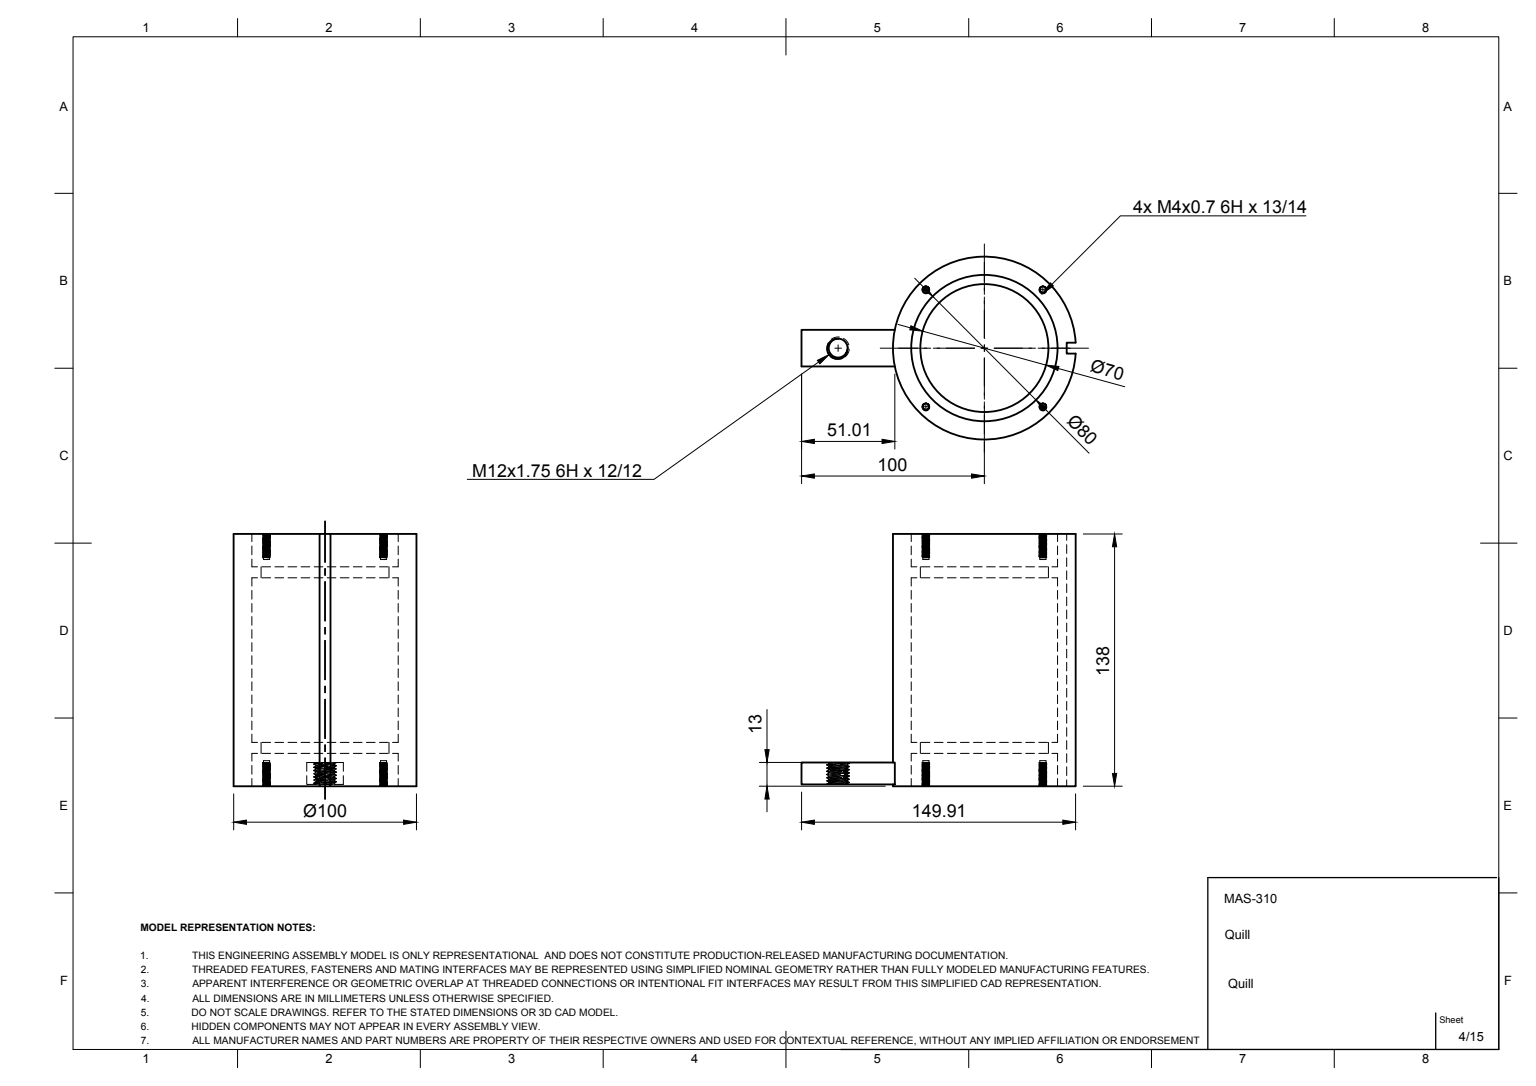
ISO-10303-21;
HEADER;
/* Generated by software containing ST-Developer
 * from STEP Tools, Inc. (www.steptools.com) 
 */

FILE_DESCRIPTION(
/* description */ ('Independent30mm screw-fed quill/spindle unit with16mm straight tool s
ocket, radial set screw, native reusable open ball bearings, retained 
inner/outer race stacks, keyed quill guide and M12x1.75 fine feed. Ext
ernal moving drive and tool not included. Ideal cage orbital links; in
dividual ball spin, force and preload not simulated. No drilling capac
ity, runout, speed, torque, load, life or machine safety rating.'),
/* implementation_level */ '2;1');

FILE_NAME(
/* name */ 'Quill.step',
/* time_stamp */ '2026-11-08T18:59:42-08:00',
/* author */ (''),
/* organization */ (''),
/* preprocessor_version */ 'ST-DEVELOPER v20.2',
/* originating_system */ 'Autodesk Translation Framework v15.17.0.0',
/* authorisation */ '');

FILE_SCHEMA (('AUTOMOTIVE_DESIGN { 1 0 10303 214 3 1 1 }'));
ENDSEC;

DATA;
#10=MECHANICAL_DESIGN_GEOMETRIC_PRESENTATION_REPRESENTATION('',(#1593),#63898);
#240=B_SPLINE_SURFACE_WITH_KNOTS('',3,3,((#31744,#31745,#31746,#31747,#31748,
#31749,#31750,#31751,#31752,#31753,#31754,#31755,#31756,#31757,#31758,#31759,
#31760,#31761,#31762,#31763,#31764,#31765,#31766,#31767,#31768,#31769,#31770,
#31771,#31772,#31773,#31774,#31775,#31776,#31777,#31778,#31779,#31780,#31781,
#31782,#31783,#31784,#31785,#31786,#31787,#31788,#31789,#31790,#31791,#31792,
#31793,#31794,#31795,#31796,#31797,#31798,#31799,#31800,#31801,#31802,#31803,
#31804,#31805,#31806,#31807,#31808,#31809,#31810,#31811,#31812,#31813,#31814,
#31815,#31816,#31817,#31818,#31819,#31820,#31821,#31822,#31823,#31824,#31825,
#31826,#31827,#31828,#31829,#31830,#31831,#31832,#31833,#31834,#31835,#31836,
#31837,#31838,#31839,#31840,#31841,#31842,#31843,#31844,#31845,#31846,#31847,
#31848,#31849,#31850,#31851,#31852,#31853,#31854,#31855,#31856,#31857,#31858,
#31859,#31860,#31861,#31862,#31863,#31864,#31865),(#31866,#31867,#31868,
#31869,#31870,#31871,#31872,#31873,#31874,#31875,#31876,#31877,#31878,#31879,
#31880,#31881,#31882,#31883,#31884,#31885,#31886,#31887,#31888,#31889,#31890,
#31891,#31892,#31893,#31894,#31895,#31896,#31897,#31898,#31899,#31900,#31901,
#31902,#31903,#31904,#31905,#31906,#31907,#31908,#31909,#31910,#31911,#31912,
#31913,#31914,#31915,#31916,#31917,#31918,#31919,#31920,#31921,#31922,#31923,
#31924,#31925,#31926,#31927,#31928,#31929,#31930,#31931,#31932,#31933,#31934,
#31935,#31936,#31937,#31938,#31939,#31940,#31941,#31942,#31943,#31944,#31945,
#31946,#31947,#31948,#31949,#31950,#31951,#31952,#31953,#31954,#31955,#31956,
#31957,#31958,#31959,#31960,#31961,#31962,#31963,#31964,#31965,#31966,#31967,
#31968,#31969,#31970,#31971,#31972,#31973,#31974,#31975,#31976,#31977,#31978,
#31979,#31980,#31981,#31982,#31983,#31984,#31985,#31986,#31987),(#31988,
#31989,#31990,#31991,#31992,#31993,#31994,#31995,#31996,#31997,#31998,#31999,
#32000,#32001,#32002,#32003,#32004,#32005,#32006,#32007,#32008,#32009,#32010,
#32011,#32012,#32013,#32014,#32015,#32016,#32017,#32018,#32019,#32020,#32021,
#32022,#32023,#32024,#32025,#32026,#32027,#32028,#32029,#32030,#32031,#32032,
#32033,#32034,#32035,#32036,#32037,#32038,#32039,#32040,#32041,#32042,#32043,
#32044,#32045,#32046,#32047,#32048,#32049,#32050,#32051,#32052,#32053,#32054,
#32055,#32056,#32057,#32058,#32059,#32060,#32061,#32062,#32063,#32064,#32065,
#32066,#32067,#32068,#32069,#32070,#32071,#32072,#32073,#32074,#32075,#32076,
#32077,#32078,#32079,#32080,#32081,#32082,#32083,#32084,#32085,#32086,#32087,
#32088,#32089,#32090,#32091,#32092,#32093,#32094,#32095,#32096,#32097,#32098,
#32099,#32100,#32101,#32102,#32103,#32104,#32105,#32106,#32107,#32108,#32109),
(#32110,#32111,#32112,#32113,#32114,#32115,#32116,#32117,#32118,#32119,
#32120,#32121,#32122,#32123,#32124,#32125,#32126,#32127,#32128,#32129,#32130,
#32131,#32132,#32133,#32134,#32135,#32136,#32137,#32138,#32139,#32140,#32141,
#32142,#32143,#32144,#32145,#32146,#32147,#32148,#32149,#32150,#32151,#32152,
#32153,#32154,#32155,#32156,#32157,#32158,#32159,#32160,#32161,#32162,#32163,
#32164,#32165,#32166,#32167,#32168,#32169,#32170,#32171,#32172,#32173,#32174,
#32175,#32176,#32177,#32178,#32179,#32180,#32181,#32182,#32183,#32184,#32185,
#32186,#32187,#32188,#32189,#32190,#32191,#32192,#32193,#32194,#32195,#32196,
#32197,#32198,#32199,#32200,#32201,#32202,#32203,#32204,#32205,#32206,#32207,
#32208,#32209,#32210,#32211,#32212,#32213,#32214,#32215,#32216,#32217,#32218,
#32219,#32220,#32221,#32222,#32223,#32224,#32225,#32226,#32227,#32228,#32229,
#32230,#32231)),.UNSPECIFIED.,.F.,.F.,.F.,(4,4),(4,1,1,1,1,1,1,1,1,1,1,
1,1,1,1,1,1,1,1,1,1,1,1,1,1,1,1,1,1,1,1,1,1,1,1,1,1,1,1,1,1,1,1,1,1,1,1,
1,1,1,1,1,1,1,1,1,1,1,1,1,1,1,1,1,1,1,1,1,1,1,1,1,1,1,1,1,1,1,1,1,1,1,1,
1,1,1,1,1,1,1,1,1,1,1,1,1,1,1,1,1,1,1,1,1,1,1,1,1,1,1,1,1,1,1,1,1,1,1,1,
4),(0.,0.0448889834294937),(11.8615800042573,12.8590786597078,13.8565773151583,
14.8540759706088,15.8515746260593,16.8490732815098,17.8465719369603,18.8440705924108,
19.8415692478613,20.8390679033118,21.8365665587623,22.8340652142128,23.8315638696633,
24.8290625251138,25.8265611805643,26.8240598360148,27.8215584914653,28.8190571469158,
29.8165558023663,30.8140544578168,31.8115531132673,32.8090517687178,33.8065504241683,
34.8040490796188,35.8015477350693,36.7990463905198,37.7965450459703,38.7940437014208,
39.7915423568713,40.7890410123218,41.7865396677723,42.7840383232228,43.7815369786733,
44.7790356341238,45.7765342895743,46.7740329450248,47.7715316004753,48.7690302559258,
49.7665289113763,50.7640275668268,51.7615262222773,52.7590248777278,53.7565235331783,
54.7540221886288,55.7515208440793,56.7490194995298,57.7465181549803,58.7440168104308,
59.7415154658813,60.7390141213318,61.7365127767823,62.7340114322328,63.7315100876833,
64.7290087431338,65.7265073985843,66.7240060540348,67.7215047094853,68.7190033649358,
69.7165020203863,70.7140006758368,71.7114993312873,72.7089979867378,73.7064966421883,
74.7039952976388,75.7014939530893,76.6989926085398,77.6964912639903,78.6939899194408,
79.6914885748913,80.6889872303418,81.6864858857923,82.6839845412428,83.6814831966933,
84.6789818521438,85.6764805075943,86.6739791630448,87.6714778184953,88.6689764739458,
89.6664751293963,90.6639737848468,91.6614724402973,92.6589710957478,93.6564697511983,
94.6539684066488,95.6514670620993,96.6489657175498,97.6464643730003,98.6439630284508,
99.6414616839013,100.638960339352,101.636458994802,102.633957650253,103.631456305703,
104.628954961154,105.626453616604,106.623952272055,107.621450927505,108.618949582956,
109.616448238406,110.613946893857,111.611445549307,112.608944204758,113.606442860208,
114.603941515659,115.601440171109,116.59893882656,117.59643748201,118.593936137461,
119.591434792911,120.588933448362,121.586432103812,122.583930759263,123.581429414713,
124.578928070164,125.576426725614,126.573925381065,127.571424036515,128.568922691966,
129.566421347416,130.563920002867),.UNSPECIFIED.);
#241=B_SPLINE_SURFACE_WITH_KNOTS('',3,3,((#32339,#32340,#32341,#32342,#32343,
#32344,#32345,#32346,#32347,#32348,#32349,#32350,#32351,#32352,#32353,#32354,
#32355,#32356,#32357,#32358,#32359,#32360,#32361,#32362,#32363,#32364,#32365,
#32366,#32367,#32368,#32369,#32370,#32371,#32372,#32373,#32374,#32375,#32376,
#32377,#32378,#32379,#32380,#32381,#32382,#32383,#32384,#32385,#32386,#32387,
#32388,#32389,#32390,#32391,#32392,#32393,#32394,#32395,#32396,#32397,#32398,
#32399,#32400,#32401,#32402,#32403,#32404,#32405,#32406,#32407,#32408,#32409,
#32410,#32411,#32412,#32413,#32414,#32415,#32416,#32417,#32418,#32419,#32420,
#32421,#32422,#32423,#32424,#32425,#32426,#32427,#32428,#32429,#32430,#32431,
#32432,#32433,#32434,#32435,#32436,#32437,#32438,#32439,#32440,#32441,#32442,
#32443,#32444,#32445,#32446,#32447,#32448,#32449,#32450,#32451,#32452,#32453,
#32454,#32455,#32456,#32457,#32458,#32459,#32460),(#32461,#32462,#32463,
#32464,#32465,#32466,#32467,#32468,#32469,#32470,#32471,#32472,#32473,#32474,
#32475,#32476,#32477,#32478,#32479,#32480,#32481,#32482,#32483,#32484,#32485,
#32486,#32487,#32488,#32489,#32490,#32491,#32492,#32493,#32494,#32495,#32496,
#32497,#32498,#32499,#32500,#32501,#32502,#32503,#32504,#32505,#32506,#32507,
#32508,#32509,#32510,#32511,#32512,#32513,#32514,#32515,#32516,#32517,#32518,
#32519,#32520,#32521,#32522,#32523,#32524,#32525,#32526,#32527,#32528,#32529,
#32530,#32531,#32532,#32533,#32534,#32535,#32536,#32537,#32538,#32539,#32540,
#32541,#32542,#32543,#32544,#32545,#32546,#32547,#32548,#32549,#32550,#32551,
#32552,#32553,#32554,#32555,#32556,#32557,#32558,#32559,#32560,#32561,#32562,
#32563,#32564,#32565,#32566,#32567,#32568,#32569,#32570,#32571,#32572,#32573,
#32574,#32575,#32576,#32577,#32578,#32579,#32580,#32581,#32582),(#32583,
#32584,#32585,#32586,#32587,#32588,#32589,#32590,#32591,#32592,#32593,#32594,
#32595,#32596,#32597,#32598,#32599,#32600,#32601,#32602,#32603,#32604,#32605,
#32606,#32607,#32608,#32609,#32610,#32611,#32612,#32613,#32614,#32615,#32616,
#32617,#32618,#32619,#32620,#32621,#32622,#32623,#32624,#32625,#32626,#32627,
#32628,#32629,#32630,#32631,#32632,#32633,#32634,#32635,#32636,#32637,#32638,
#32639,#32640,#32641,#32642,#32643,#32644,#32645,#32646,#32647,#32648,#32649,
#32650,#32651,#32652,#32653,#32654,#32655,#32656,#32657,#32658,#32659,#32660,
#32661,#32662,#32663,#32664,#32665,#32666,#32667,#32668,#32669,#32670,#32671,
#32672,#32673,#32674,#32675,#32676,#32677,#32678,#32679,#32680,#32681,#32682,
#32683,#32684,#32685,#32686,#32687,#32688,#32689,#32690,#32691,#32692,#32693,
#32694,#32695,#32696,#32697,#32698,#32699,#32700,#32701,#32702,#32703,#32704),
(#32705,#32706,#32707,#32708,#32709,#32710,#32711,#32712,#32713,#32714,
#32715,#32716,#32717,#32718,#32719,#32720,#32721,#32722,#32723,#32724,#32725,
#32726,#32727,#32728,#32729,#32730,#32731,#32732,#32733,#32734,#32735,#32736,
#32737,#32738,#32739,#32740,#32741,#32742,#32743,#32744,#32745,#32746,#32747,
#32748,#32749,#32750,#32751,#32752,#32753,#32754,#32755,#32756,#32757,#32758,
#32759,#32760,#32761,#32762,#32763,#32764,#32765,#32766,#32767,#32768,#32769,
#32770,#32771,#32772,#32773,#32774,#32775,#32776,#32777,#32778,#32779,#32780,
#32781,#32782,#32783,#32784,#32785,#32786,#32787,#32788,#32789,#32790,#32791,
#32792,#32793,#32794,#32795,#32796,#32797,#32798,#32799,#32800,#32801,#32802,
#32803,#32804,#32805,#32806,#32807,#32808,#32809,#32810,#32811,#32812,#32813,
#32814,#32815,#32816,#32817,#32818,#32819,#32820,#32821,#32822,#32823,#32824,
#32825,#32826)),.UNSPECIFIED.,.F.,.F.,.F.,(4,4),(4,1,1,1,1,1,1,1,1,1,1,
1,1,1,1,1,1,1,1,1,1,1,1,1,1,1,1,1,1,1,1,1,1,1,1,1,1,1,1,1,1,1,1,1,1,1,1,
1,1,1,1,1,1,1,1,1,1,1,1,1,1,1,1,1,1,1,1,1,1,1,1,1,1,1,1,1,1,1,1,1,1,1,1,
1,1,1,1,1,1,1,1,1,1,1,1,1,1,1,1,1,1,1,1,1,1,1,1,1,1,1,1,1,1,1,1,1,1,1,1,
4),(0.,0.0448889834294937),(14.3981410127776,15.3956396682281,16.3931383236786,
17.3906369791291,18.3881356345796,19.3856342900301,20.3831329454806,21.3806316009311,
22.3781302563816,23.3756289118321,24.3731275672826,25.3706262227331,26.3681248781836,
27.3656235336341,28.3631221890846,29.3606208445351,30.3581194999856,31.3556181554361,
32.3531168108866,33.3506154663371,34.3481141217876,35.3456127772381,36.3431114326886,
37.3406100881391,38.3381087435896,39.3356073990401,40.3331060544906,41.3306047099411,
42.3281033653916,43.3256020208421,44.3231006762926,45.3205993317431,46.3180979871936,
47.3155966426441,48.3130952980946,49.3105939535451,50.3080926089956,51.3055912644461,
52.3030899198966,53.3005885753471,54.2980872307976,55.2955858862481,56.2930845416986,
57.2905831971491,58.2880818525996,59.2855805080501,60.2830791635006,61.2805778189511,
62.2780764744016,63.2755751298521,64.2730737853026,65.2705724407531,66.2680710962036,
67.2655697516541,68.2630684071046,69.2605670625551,70.2580657180056,71.2555643734561,
72.2530630289066,73.2505616843571,74.2480603398076,75.2455589952581,76.2430576507086,
77.2405563061591,78.2380549616096,79.2355536170601,80.2330522725106,81.2305509279611,
82.2280495834116,83.2255482388621,84.2230468943126,85.2205455497631,86.2180442052136,
87.2155428606641,88.2130415161146,89.2105401715651,90.2080388270156,91.2055374824661,
92.2030361379166,93.2005347933671,94.1980334488176,95.1955321042681,96.1930307597186,
97.1905294151691,98.1880280706196,99.1855267260701,100.183025381521,101.180524036971,
102.178022692422,103.175521347872,104.173020003323,105.170518658773,106.168017314224,
107.165515969674,108.163014625125,109.160513280575,110.158011936026,111.155510591476,
112.153009246927,113.150507902377,114.148006557828,115.145505213278,116.143003868729,
117.140502524179,118.13800117963,119.13549983508,120.132998490531,121.130497145981,
122.127995801432,123.125494456882,124.122993112333,125.120491767783,126.117990423234,
127.115489078684,128.112987734135,129.110486389585,130.107985045036,131.105483700486,
132.102982355937,133.100481011387),.UNSPECIFIED.);
#242=B_SPLINE_SURFACE_WITH_KNOTS('',3,3,((#33131,#33132,#33133,#33134,#33135,
#33136,#33137,#33138,#33139,#33140,#33141,#33142,#33143,#33144,#33145,#33146,
#33147,#33148,#33149,#33150,#33151,#33152,#33153,#33154,#33155,#33156,#33157,
#33158,#33159,#33160,#33161,#33162,#33163,#33164,#33165,#33166,#33167,#33168,
#33169,#33170,#33171,#33172,#33173,#33174,#33175,#33176,#33177,#33178,#33179,
#33180,#33181,#33182,#33183,#33184,#33185,#33186,#33187,#33188,#33189,#33190,
#33191,#33192,#33193,#33194,#33195,#33196,#33197,#33198,#33199,#33200,#33201,
#33202,#33203,#33204,#33205,#33206,#33207,#33208,#33209,#33210,#33211,#33212,
#33213,#33214,#33215,#33216,#33217,#33218,#33219,#33220,#33221,#33222,#33223,
#33224,#33225,#33226,#33227,#33228,#33229,#33230,#33231,#33232,#33233,#33234,
#33235,#33236,#33237,#33238,#33239,#33240,#33241,#33242,#33243,#33244,#33245,
#33246,#33247,#33248,#33249,#33250,#33251,#33252),(#33253,#33254,#33255,
#33256,#33257,#33258,#33259,#33260,#33261,#33262,#33263,#33264,#33265,#33266,
#33267,#33268,#33269,#33270,#33271,#33272,#33273,#33274,#33275,#33276,#33277,
#33278,#33279,#33280,#33281,#33282,#33283,#33284,#33285,#33286,#33287,#33288,
#33289,#33290,#33291,#33292,#33293,#33294,#33295,#33296,#33297,#33298,#33299,
#33300,#33301,#33302,#33303,#33304,#33305,#33306,#33307,#33308,#33309,#33310,
#33311,#33312,#33313,#33314,#33315,#33316,#33317,#33318,#33319,#33320,#33321,
#33322,#33323,#33324,#33325,#33326,#33327,#33328,#33329,#33330,#33331,#33332,
#33333,#33334,#33335,#33336,#33337,#33338,#33339,#33340,#33341,#33342,#33343,
#33344,#33345,#33346,#33347,#33348,#33349,#33350,#33351,#33352,#33353,#33354,
#33355,#33356,#33357,#33358,#33359,#33360,#33361,#33362,#33363,#33364,#33365,
#33366,#33367,#33368,#33369,#33370,#33371,#33372,#33373,#33374),(#33375,
#33376,#33377,#33378,#33379,#33380,#33381,#33382,#33383,#33384,#33385,#33386,
#33387,#33388,#33389,#33390,#33391,#33392,#33393,#33394,#33395,#33396,#33397,
#33398,#33399,#33400,#33401,#33402,#33403,#33404,#33405,#33406,#33407,#33408,
#33409,#33410,#33411,#33412,#33413,#33414,#33415,#33416,#33417,#33418,#33419,
#33420,#33421,#33422,#33423,#33424,#33425,#33426,#33427,#33428,#33429,#33430,
#33431,#33432,#33433,#33434,#33435,#33436,#33437,#33438,#33439,#33440,#33441,
#33442,#33443,#33444,#33445,#33446,#33447,#33448,#33449,#33450,#33451,#33452,
#33453,#33454,#33455,#33456,#33457,#33458,#33459,#33460,#33461,#33462,#33463,
#33464,#33465,#33466,#33467,#33468,#33469,#33470,#33471,#33472,#33473,#33474,
#33475,#33476,#33477,#33478,#33479,#33480,#33481,#33482,#33483,#33484,#33485,
#33486,#33487,#33488,#33489,#33490,#33491,#33492,#33493,#33494,#33495,#33496),
(#33497,#33498,#33499,#33500,#33501,#33502,#33503,#33504,#33505,#33506,
#33507,#33508,#33509,#33510,#33511,#33512,#33513,#33514,#33515,#33516,#33517,
#33518,#33519,#33520,#33521,#33522,#33523,#33524,#33525,#33526,#33527,#33528,
#33529,#33530,#33531,#33532,#33533,#33534,#33535,#33536,#33537,#33538,#33539,
#33540,#33541,#33542,#33543,#33544,#33545,#33546,#33547,#33548,#33549,#33550,
#33551,#33552,#33553,#33554,#33555,#33556,#33557,#33558,#33559,#33560,#33561,
#33562,#33563,#33564,#33565,#33566,#33567,#33568,#33569,#33570,#33571,#33572,
#33573,#33574,#33575,#33576,#33577,#33578,#33579,#33580,#33581,#33582,#33583,
#33584,#33585,#33586,#33587,#33588,#33589,#33590,#33591,#33592,#33593,#33594,
#33595,#33596,#33597,#33598,#33599,#33600,#33601,#33602,#33603,#33604,#33605,
#33606,#33607,#33608,#33609,#33610,#33611,#33612,#33613,#33614,#33615,#33616,
#33617,#33618)),.UNSPECIFIED.,.F.,.F.,.F.,(4,4),(4,1,1,1,1,1,1,1,1,1,1,
1,1,1,1,1,1,1,1,1,1,1,1,1,1,1,1,1,1,1,1,1,1,1,1,1,1,1,1,1,1,1,1,1,1,1,1,
1,1,1,1,1,1,1,1,1,1,1,1,1,1,1,1,1,1,1,1,1,1,1,1,1,1,1,1,1,1,1,1,1,1,1,1,
1,1,1,1,1,1,1,1,1,1,1,1,1,1,1,1,1,1,1,1,1,1,1,1,1,1,1,1,1,1,1,1,1,1,1,1,
4),(0.,0.0448889834294937),(11.8615800042567,12.8590786597072,13.8565773151577,
14.8540759706082,15.8515746260587,16.8490732815092,17.8465719369597,18.8440705924102,
19.8415692478607,20.8390679033112,21.8365665587617,22.8340652142122,23.8315638696627,
24.8290625251132,25.8265611805637,26.8240598360142,27.8215584914647,28.8190571469152,
29.8165558023657,30.8140544578162,31.8115531132667,32.8090517687172,33.8065504241677,
34.8040490796182,35.8015477350687,36.7990463905192,37.7965450459697,38.7940437014202,
39.7915423568707,40.7890410123212,41.7865396677717,42.7840383232222,43.7815369786727,
44.7790356341232,45.7765342895737,46.7740329450242,47.7715316004747,48.7690302559252,
49.7665289113757,50.7640275668262,51.7615262222767,52.7590248777272,53.7565235331777,
54.7540221886282,55.7515208440787,56.7490194995292,57.7465181549797,58.7440168104302,
59.7415154658807,60.7390141213312,61.7365127767817,62.7340114322322,63.7315100876827,
64.7290087431332,65.7265073985837,66.7240060540342,67.7215047094847,68.7190033649352,
69.7165020203857,70.7140006758362,71.7114993312867,72.7089979867372,73.7064966421877,
74.7039952976382,75.7014939530887,76.6989926085392,77.6964912639897,78.6939899194402,
79.6914885748907,80.6889872303412,81.6864858857917,82.6839845412422,83.6814831966927,
84.6789818521432,85.6764805075937,86.6739791630442,87.6714778184947,88.6689764739452,
89.6664751293957,90.6639737848462,91.6614724402967,92.6589710957472,93.6564697511977,
94.6539684066482,95.6514670620987,96.6489657175492,97.6464643729997,98.6439630284502,
99.6414616839007,100.638960339351,101.636458994802,102.633957650252,103.631456305703,
104.628954961153,105.626453616604,106.623952272054,107.621450927505,108.618949582955,
109.616448238406,110.613946893856,111.611445549307,112.608944204757,113.606442860208,
114.603941515658,115.601440171109,116.598938826559,117.59643748201,118.59393613746,
119.591434792911,120.588933448361,121.586432103812,122.583930759262,123.581429414713,
124.578928070163,125.576426725614,126.573925381064,127.571424036515,128.568922691965,
129.566421347416,130.563920002866),.UNSPECIFIED.);
#243=B_SPLINE_SURFACE_WITH_KNOTS('',3,3,((#33726,#33727,#33728,#33729,#33730,
#33731,#33732,#33733,#33734,#33735,#33736,#33737,#33738,#33739,#33740,#33741,
#33742,#33743,#33744,#33745,#33746,#33747,#33748,#33749,#33750,#33751,#33752,
#33753,#33754,#33755,#33756,#33757,#33758,#33759,#33760,#33761,#33762,#33763,
#33764,#33765,#33766,#33767,#33768,#33769,#33770,#33771,#33772,#33773,#33774,
#33775,#33776,#33777,#33778,#33779,#33780,#33781,#33782,#33783,#33784,#33785,
#33786,#33787,#33788,#33789,#33790,#33791,#33792,#33793,#33794,#33795,#33796,
#33797,#33798,#33799,#33800,#33801,#33802,#33803,#33804,#33805,#33806,#33807,
#33808,#33809,#33810,#33811,#33812,#33813,#33814,#33815,#33816,#33817,#33818,
#33819,#33820,#33821,#33822,#33823,#33824,#33825,#33826,#33827,#33828,#33829,
#33830,#33831,#33832,#33833,#33834,#33835,#33836,#33837,#33838,#33839,#33840,
#33841,#33842,#33843,#33844,#33845,#33846,#33847),(#33848,#33849,#33850,
#33851,#33852,#33853,#33854,#33855,#33856,#33857,#33858,#33859,#33860,#33861,
#33862,#33863,#33864,#33865,#33866,#33867,#33868,#33869,#33870,#33871,#33872,
#33873,#33874,#33875,#33876,#33877,#33878,#33879,#33880,#33881,#33882,#33883,
#33884,#33885,#33886,#33887,#33888,#33889,#33890,#33891,#33892,#33893,#33894,
#33895,#33896,#33897,#33898,#33899,#33900,#33901,#33902,#33903,#33904,#33905,
#33906,#33907,#33908,#33909,#33910,#33911,#33912,#33913,#33914,#33915,#33916,
#33917,#33918,#33919,#33920,#33921,#33922,#33923,#33924,#33925,#33926,#33927,
#33928,#33929,#33930,#33931,#33932,#33933,#33934,#33935,#33936,#33937,#33938,
#33939,#33940,#33941,#33942,#33943,#33944,#33945,#33946,#33947,#33948,#33949,
#33950,#33951,#33952,#33953,#33954,#33955,#33956,#33957,#33958,#33959,#33960,
#33961,#33962,#33963,#33964,#33965,#33966,#33967,#33968,#33969),(#33970,
#33971,#33972,#33973,#33974,#33975,#33976,#33977,#33978,#33979,#33980,#33981,
#33982,#33983,#33984,#33985,#33986,#33987,#33988,#33989,#33990,#33991,#33992,
#33993,#33994,#33995,#33996,#33997,#33998,#33999,#34000,#34001,#34002,#34003,
#34004,#34005,#34006,#34007,#34008,#34009,#34010,#34011,#34012,#34013,#34014,
#34015,#34016,#34017,#34018,#34019,#34020,#34021,#34022,#34023,#34024,#34025,
#34026,#34027,#34028,#34029,#34030,#34031,#34032,#34033,#34034,#34035,#34036,
#34037,#34038,#34039,#34040,#34041,#34042,#34043,#34044,#34045,#34046,#34047,
#34048,#34049,#34050,#34051,#34052,#34053,#34054,#34055,#34056,#34057,#34058,
#34059,#34060,#34061,#34062,#34063,#34064,#34065,#34066,#34067,#34068,#34069,
#34070,#34071,#34072,#34073,#34074,#34075,#34076,#34077,#34078,#34079,#34080,
#34081,#34082,#34083,#34084,#34085,#34086,#34087,#34088,#34089,#34090,#34091),
(#34092,#34093,#34094,#34095,#34096,#34097,#34098,#34099,#34100,#34101,
#34102,#34103,#34104,#34105,#34106,#34107,#34108,#34109,#34110,#34111,#34112,
#34113,#34114,#34115,#34116,#34117,#34118,#34119,#34120,#34121,#34122,#34123,
#34124,#34125,#34126,#34127,#34128,#34129,#34130,#34131,#34132,#34133,#34134,
#34135,#34136,#34137,#34138,#34139,#34140,#34141,#34142,#34143,#34144,#34145,
#34146,#34147,#34148,#34149,#34150,#34151,#34152,#34153,#34154,#34155,#34156,
#34157,#34158,#34159,#34160,#34161,#34162,#34163,#34164,#34165,#34166,#34167,
#34168,#34169,#34170,#34171,#34172,#34173,#34174,#34175,#34176,#34177,#34178,
#34179,#34180,#34181,#34182,#34183,#34184,#34185,#34186,#34187,#34188,#34189,
#34190,#34191,#34192,#34193,#34194,#34195,#34196,#34197,#34198,#34199,#34200,
#34201,#34202,#34203,#34204,#34205,#34206,#34207,#34208,#34209,#34210,#34211,
#34212,#34213)),.UNSPECIFIED.,.F.,.F.,.F.,(4,4),(4,1,1,1,1,1,1,1,1,1,1,
1,1,1,1,1,1,1,1,1,1,1,1,1,1,1,1,1,1,1,1,1,1,1,1,1,1,1,1,1,1,1,1,1,1,1,1,
1,1,1,1,1,1,1,1,1,1,1,1,1,1,1,1,1,1,1,1,1,1,1,1,1,1,1,1,1,1,1,1,1,1,1,1,
1,1,1,1,1,1,1,1,1,1,1,1,1,1,1,1,1,1,1,1,1,1,1,1,1,1,1,1,1,1,1,1,1,1,1,1,
4),(0.,0.0448889834294937),(14.398141012777,15.3956396682275,16.393138323678,
17.3906369791285,18.388135634579,19.3856342900295,20.38313294548,21.3806316009305,
22.378130256381,23.3756289118315,24.373127567282,25.3706262227325,26.368124878183,
27.3656235336335,28.363122189084,29.3606208445345,30.358119499985,31.3556181554355,
32.353116810886,33.3506154663365,34.348114121787,35.3456127772375,36.343111432688,
37.3406100881385,38.338108743589,39.3356073990395,40.33310605449,41.3306047099405,
42.328103365391,43.3256020208415,44.323100676292,45.3205993317425,46.318097987193,
47.3155966426435,48.313095298094,49.3105939535445,50.308092608995,51.3055912644455,
52.303089919896,53.3005885753465,54.298087230797,55.2955858862475,56.293084541698,
57.2905831971485,58.288081852599,59.2855805080495,60.2830791635,61.2805778189505,
62.278076474401,63.2755751298515,64.273073785302,65.2705724407525,66.268071096203,
67.2655697516535,68.263068407104,69.2605670625545,70.258065718005,71.2555643734555,
72.253063028906,73.2505616843565,74.248060339807,75.2455589952575,76.243057650708,
77.2405563061585,78.238054961609,79.2355536170595,80.23305227251,81.2305509279605,
82.228049583411,83.2255482388615,84.223046894312,85.2205455497625,86.218044205213,
87.2155428606635,88.213041516114,89.2105401715645,90.208038827015,91.2055374824655,
92.203036137916,93.2005347933665,94.198033448817,95.1955321042675,96.193030759718,
97.1905294151685,98.1880280706191,99.1855267260696,100.18302538152,101.180524036971,
102.178022692421,103.175521347872,104.173020003322,105.170518658773,106.168017314223,
107.165515969674,108.163014625124,109.160513280575,110.158011936025,111.155510591476,
112.153009246926,113.150507902377,114.148006557827,115.145505213278,116.143003868728,
117.140502524179,118.138001179629,119.13549983508,120.13299849053,121.130497145981,
122.127995801431,123.125494456882,124.122993112332,125.120491767783,126.117990423233,
127.115489078684,128.112987734134,129.110486389585,130.107985045035,131.105483700486,
132.102982355936,133.100481011387),.UNSPECIFIED.);
#244=B_SPLINE_SURFACE_WITH_KNOTS('',3,3,((#34518,#34519,#34520,#34521,#34522,
#34523,#34524,#34525,#34526,#34527,#34528,#34529,#34530,#34531,#34532,#34533,
#34534,#34535,#34536,#34537,#34538,#34539,#34540,#34541,#34542,#34543,#34544,
#34545,#34546,#34547,#34548,#34549,#34550,#34551,#34552,#34553,#34554,#34555,
#34556,#34557,#34558,#34559,#34560,#34561,#34562,#34563,#34564,#34565,#34566,
#34567,#34568,#34569,#34570,#34571,#34572,#34573,#34574,#34575,#34576,#34577,
#34578,#34579,#34580,#34581,#34582,#34583,#34584,#34585,#34586,#34587,#34588,
#34589,#34590,#34591,#34592,#34593,#34594,#34595,#34596,#34597,#34598,#34599,
#34600,#34601,#34602,#34603,#34604,#34605,#34606,#34607,#34608,#34609,#34610,
#34611,#34612,#34613,#34614,#34615,#34616,#34617,#34618,#34619,#34620,#34621,
#34622,#34623,#34624,#34625,#34626,#34627,#34628,#34629,#34630,#34631,#34632,
#34633,#34634,#34635,#34636,#34637,#34638,#34639),(#34640,#34641,#34642,
#34643,#34644,#34645,#34646,#34647,#34648,#34649,#34650,#34651,#34652,#34653,
#34654,#34655,#34656,#34657,#34658,#34659,#34660,#34661,#34662,#34663,#34664,
#34665,#34666,#34667,#34668,#34669,#34670,#34671,#34672,#34673,#34674,#34675,
#34676,#34677,#34678,#34679,#34680,#34681,#34682,#34683,#34684,#34685,#34686,
#34687,#34688,#34689,#34690,#34691,#34692,#34693,#34694,#34695,#34696,#34697,
#34698,#34699,#34700,#34701,#34702,#34703,#34704,#34705,#34706,#34707,#34708,
#34709,#34710,#34711,#34712,#34713,#34714,#34715,#34716,#34717,#34718,#34719,
#34720,#34721,#34722,#34723,#34724,#34725,#34726,#34727,#34728,#34729,#34730,
#34731,#34732,#34733,#34734,#34735,#34736,#34737,#34738,#34739,#34740,#34741,
#34742,#34743,#34744,#34745,#34746,#34747,#34748,#34749,#34750,#34751,#34752,
#34753,#34754,#34755,#34756,#34757,#34758,#34759,#34760,#34761),(#34762,
#34763,#34764,#34765,#34766,#34767,#34768,#34769,#34770,#34771,#34772,#34773,
#34774,#34775,#34776,#34777,#34778,#34779,#34780,#34781,#34782,#34783,#34784,
#34785,#34786,#34787,#34788,#34789,#34790,#34791,#34792,#34793,#34794,#34795,
#34796,#34797,#34798,#34799,#34800,#34801,#34802,#34803,#34804,#34805,#34806,
#34807,#34808,#34809,#34810,#34811,#34812,#34813,#34814,#34815,#34816,#34817,
#34818,#34819,#34820,#34821,#34822,#34823,#34824,#34825,#34826,#34827,#34828,
#34829,#34830,#34831,#34832,#34833,#34834,#34835,#34836,#34837,#34838,#34839,
#34840,#34841,#34842,#34843,#34844,#34845,#34846,#34847,#34848,#34849,#34850,
#34851,#34852,#34853,#34854,#34855,#34856,#34857,#34858,#34859,#34860,#34861,
#34862,#34863,#34864,#34865,#34866,#34867,#34868,#34869,#34870,#34871,#34872,
#34873,#34874,#34875,#34876,#34877,#34878,#34879,#34880,#34881,#34882,#34883),
(#34884,#34885,#34886,#34887,#34888,#34889,#34890,#34891,#34892,#34893,
#34894,#34895,#34896,#34897,#34898,#34899,#34900,#34901,#34902,#34903,#34904,
#34905,#34906,#34907,#34908,#34909,#34910,#34911,#34912,#34913,#34914,#34915,
#34916,#34917,#34918,#34919,#34920,#34921,#34922,#34923,#34924,#34925,#34926,
#34927,#34928,#34929,#34930,#34931,#34932,#34933,#34934,#34935,#34936,#34937,
#34938,#34939,#34940,#34941,#34942,#34943,#34944,#34945,#34946,#34947,#34948,
#34949,#34950,#34951,#34952,#34953,#34954,#34955,#34956,#34957,#34958,#34959,
#34960,#34961,#34962,#34963,#34964,#34965,#34966,#34967,#34968,#34969,#34970,
#34971,#34972,#34973,#34974,#34975,#34976,#34977,#34978,#34979,#34980,#34981,
#34982,#34983,#34984,#34985,#34986,#34987,#34988,#34989,#34990,#34991,#34992,
#34993,#34994,#34995,#34996,#34997,#34998,#34999,#35000,#35001,#35002,#35003,
#35004,#35005)),.UNSPECIFIED.,.F.,.F.,.F.,(4,4),(4,1,1,1,1,1,1,1,1,1,1,
1,1,1,1,1,1,1,1,1,1,1,1,1,1,1,1,1,1,1,1,1,1,1,1,1,1,1,1,1,1,1,1,1,1,1,1,
1,1,1,1,1,1,1,1,1,1,1,1,1,1,1,1,1,1,1,1,1,1,1,1,1,1,1,1,1,1,1,1,1,1,1,1,
1,1,1,1,1,1,1,1,1,1,1,1,1,1,1,1,1,1,1,1,1,1,1,1,1,1,1,1,1,1,1,1,1,1,1,1,
4),(0.,0.0448889834294937),(11.861580004257,12.8590786597075,13.856577315158,
14.8540759706085,15.851574626059,16.8490732815095,17.84657193696,18.8440705924105,
19.841569247861,20.8390679033115,21.836566558762,22.8340652142125,23.831563869663,
24.8290625251135,25.826561180564,26.8240598360145,27.821558491465,28.8190571469155,
29.816555802366,30.8140544578165,31.811553113267,32.8090517687175,33.806550424168,
34.8040490796185,35.801547735069,36.7990463905195,37.79654504597,38.7940437014205,
39.791542356871,40.7890410123215,41.786539667772,42.7840383232225,43.781536978673,
44.7790356341235,45.776534289574,46.7740329450245,47.771531600475,48.7690302559255,
49.766528911376,50.7640275668265,51.761526222277,52.7590248777275,53.756523533178,
54.7540221886285,55.751520844079,56.7490194995295,57.74651815498,58.7440168104305,
59.741515465881,60.7390141213315,61.736512776782,62.7340114322325,63.731510087683,
64.7290087431335,65.726507398584,66.7240060540345,67.721504709485,68.7190033649355,
69.716502020386,70.7140006758365,71.711499331287,72.7089979867375,73.706496642188,
74.7039952976385,75.701493953089,76.6989926085395,77.69649126399,78.6939899194405,
79.691488574891,80.6889872303415,81.686485885792,82.6839845412425,83.681483196693,
84.6789818521435,85.676480507594,86.6739791630445,87.671477818495,88.6689764739455,
89.666475129396,90.6639737848465,91.661472440297,92.6589710957475,93.656469751198,
94.6539684066485,95.651467062099,96.6489657175495,97.646464373,98.6439630284505,
99.641461683901,100.638960339352,101.636458994802,102.633957650253,103.631456305703,
104.628954961154,105.626453616604,106.623952272055,107.621450927505,108.618949582956,
109.616448238406,110.613946893857,111.611445549307,112.608944204758,113.606442860208,
114.603941515659,115.601440171109,116.59893882656,117.59643748201,118.593936137461,
119.591434792911,120.588933448362,121.586432103812,122.583930759263,123.581429414713,
124.578928070164,125.576426725614,126.573925381065,127.571424036515,128.568922691966,
129.566421347416,130.563920002867),.UNSPECIFIED.);
#245=B_SPLINE_SURFACE_WITH_KNOTS('',3,3,((#35113,#35114,#35115,#35116,#35117,
#35118,#35119,#35120,#35121,#35122,#35123,#35124,#35125,#35126,#35127,#35128,
#35129,#35130,#35131,#35132,#35133,#35134,#35135,#35136,#35137,#35138,#35139,
#35140,#35141,#35142,#35143,#35144,#35145,#35146,#35147,#35148,#35149,#35150,
#35151,#35152,#35153,#35154,#35155,#35156,#35157,#35158,#35159,#35160,#35161,
#35162,#35163,#35164,#35165,#35166,#35167,#35168,#35169,#35170,#35171,#35172,
#35173,#35174,#35175,#35176,#35177,#35178,#35179,#35180,#35181,#35182,#35183,
#35184,#35185,#35186,#35187,#35188,#35189,#35190,#35191,#35192,#35193,#35194,
#35195,#35196,#35197,#35198,#35199,#35200,#35201,#35202,#35203,#35204,#35205,
#35206,#35207,#35208,#35209,#35210,#35211,#35212,#35213,#35214,#35215,#35216,
#35217,#35218,#35219,#35220,#35221,#35222,#35223,#35224,#35225,#35226,#35227,
#35228,#35229,#35230,#35231,#35232,#35233,#35234),(#35235,#35236,#35237,
#35238,#35239,#35240,#35241,#35242,#35243,#35244,#35245,#35246,#35247,#35248,
#35249,#35250,#35251,#35252,#35253,#35254,#35255,#35256,#35257,#35258,#35259,
#35260,#35261,#35262,#35263,#35264,#35265,#35266,#35267,#35268,#35269,#35270,
#35271,#35272,#35273,#35274,#35275,#35276,#35277,#35278,#35279,#35280,#35281,
#35282,#35283,#35284,#35285,#35286,#35287,#35288,#35289,#35290,#35291,#35292,
#35293,#35294,#35295,#35296,#35297,#35298,#35299,#35300,#35301,#35302,#35303,
#35304,#35305,#35306,#35307,#35308,#35309,#35310,#35311,#35312,#35313,#35314,
#35315,#35316,#35317,#35318,#35319,#35320,#35321,#35322,#35323,#35324,#35325,
#35326,#35327,#35328,#35329,#35330,#35331,#35332,#35333,#35334,#35335,#35336,
#35337,#35338,#35339,#35340,#35341,#35342,#35343,#35344,#35345,#35346,#35347,
#35348,#35349,#35350,#35351,#35352,#35353,#35354,#35355,#35356),(#35357,
#35358,#35359,#35360,#35361,#35362,#35363,#35364,#35365,#35366,#35367,#35368,
#35369,#35370,#35371,#35372,#35373,#35374,#35375,#35376,#35377,#35378,#35379,
#35380,#35381,#35382,#35383,#35384,#35385,#35386,#35387,#35388,#35389,#35390,
#35391,#35392,#35393,#35394,#35395,#35396,#35397,#35398,#35399,#35400,#35401,
#35402,#35403,#35404,#35405,#35406,#35407,#35408,#35409,#35410,#35411,#35412,
#35413,#35414,#35415,#35416,#35417,#35418,#35419,#35420,#35421,#35422,#35423,
#35424,#35425,#35426,#35427,#35428,#35429,#35430,#35431,#35432,#35433,#35434,
#35435,#35436,#35437,#35438,#35439,#35440,#35441,#35442,#35443,#35444,#35445,
#35446,#35447,#35448,#35449,#35450,#35451,#35452,#35453,#35454,#35455,#35456,
#35457,#35458,#35459,#35460,#35461,#35462,#35463,#35464,#35465,#35466,#35467,
#35468,#35469,#35470,#35471,#35472,#35473,#35474,#35475,#35476,#35477,#35478),
(#35479,#35480,#35481,#35482,#35483,#35484,#35485,#35486,#35487,#35488,
#35489,#35490,#35491,#35492,#35493,#35494,#35495,#35496,#35497,#35498,#35499,
#35500,#35501,#35502,#35503,#35504,#35505,#35506,#35507,#35508,#35509,#35510,
#35511,#35512,#35513,#35514,#35515,#35516,#35517,#35518,#35519,#35520,#35521,
#35522,#35523,#35524,#35525,#35526,#35527,#35528,#35529,#35530,#35531,#35532,
#35533,#35534,#35535,#35536,#35537,#35538,#35539,#35540,#35541,#35542,#35543,
#35544,#35545,#35546,#35547,#35548,#35549,#35550,#35551,#35552,#35553,#35554,
#35555,#35556,#35557,#35558,#35559,#35560,#35561,#35562,#35563,#35564,#35565,
#35566,#35567,#35568,#35569,#35570,#35571,#35572,#35573,#35574,#35575,#35576,
#35577,#35578,#35579,#35580,#35581,#35582,#35583,#35584,#35585,#35586,#35587,
#35588,#35589,#35590,#35591,#35592,#35593,#35594,#35595,#35596,#35597,#35598,
#35599,#35600)),.UNSPECIFIED.,.F.,.F.,.F.,(4,4),(4,1,1,1,1,1,1,1,1,1,1,
1,1,1,1,1,1,1,1,1,1,1,1,1,1,1,1,1,1,1,1,1,1,1,1,1,1,1,1,1,1,1,1,1,1,1,1,
1,1,1,1,1,1,1,1,1,1,1,1,1,1,1,1,1,1,1,1,1,1,1,1,1,1,1,1,1,1,1,1,1,1,1,1,
1,1,1,1,1,1,1,1,1,1,1,1,1,1,1,1,1,1,1,1,1,1,1,1,1,1,1,1,1,1,1,1,1,1,1,1,
4),(0.,0.0448889834294937),(14.3981410127773,15.3956396682278,16.3931383236783,
17.3906369791288,18.3881356345793,19.3856342900298,20.3831329454803,21.3806316009308,
22.3781302563813,23.3756289118318,24.3731275672823,25.3706262227328,26.3681248781833,
27.3656235336338,28.3631221890843,29.3606208445348,30.3581194999853,31.3556181554358,
32.3531168108863,33.3506154663368,34.3481141217873,35.3456127772378,36.3431114326883,
37.3406100881388,38.3381087435893,39.3356073990398,40.3331060544903,41.3306047099408,
42.3281033653913,43.3256020208418,44.3231006762923,45.3205993317428,46.3180979871933,
47.3155966426438,48.3130952980943,49.3105939535448,50.3080926089953,51.3055912644458,
52.3030899198963,53.3005885753468,54.2980872307973,55.2955858862478,56.2930845416983,
57.2905831971488,58.2880818525993,59.2855805080498,60.2830791635003,61.2805778189508,
62.2780764744013,63.2755751298518,64.2730737853023,65.2705724407528,66.2680710962033,
67.2655697516538,68.2630684071043,69.2605670625549,70.2580657180054,71.2555643734559,
72.2530630289064,73.2505616843569,74.2480603398074,75.2455589952579,76.2430576507084,
77.2405563061589,78.2380549616094,79.2355536170598,80.2330522725103,81.2305509279608,
82.2280495834113,83.2255482388618,84.2230468943123,85.2205455497629,86.2180442052134,
87.2155428606639,88.2130415161144,89.2105401715649,90.2080388270154,91.2055374824659,
92.2030361379164,93.2005347933669,94.1980334488174,95.1955321042679,96.1930307597184,
97.1905294151689,98.1880280706194,99.1855267260699,100.18302538152,101.180524036971,
102.178022692421,103.175521347872,104.173020003322,105.170518658773,106.168017314223,
107.165515969674,108.163014625124,109.160513280575,110.158011936025,111.155510591476,
112.153009246926,113.150507902377,114.148006557827,115.145505213278,116.143003868728,
117.140502524179,118.138001179629,119.13549983508,120.13299849053,121.130497145981,
122.127995801431,123.125494456882,124.122993112332,125.120491767783,126.117990423233,
127.115489078684,128.112987734134,129.110486389585,130.107985045035,131.105483700486,
132.102982355936,133.100481011387),.UNSPECIFIED.);
#246=B_SPLINE_SURFACE_WITH_KNOTS('',3,3,((#35905,#35906,#35907,#35908,#35909,
#35910,#35911,#35912,#35913,#35914,#35915,#35916,#35917,#35918,#35919,#35920,
#35921,#35922,#35923,#35924,#35925,#35926,#35927,#35928,#35929,#35930,#35931,
#35932,#35933,#35934,#35935,#35936,#35937,#35938,#35939,#35940,#35941,#35942,
#35943,#35944,#35945,#35946,#35947,#35948,#35949,#35950,#35951,#35952,#35953,
#35954,#35955,#35956,#35957,#35958,#35959,#35960,#35961,#35962,#35963,#35964,
#35965,#35966,#35967,#35968,#35969,#35970,#35971,#35972,#35973,#35974,#35975,
#35976,#35977,#35978,#35979,#35980,#35981,#35982,#35983,#35984,#35985,#35986,
#35987,#35988,#35989,#35990,#35991,#35992,#35993,#35994,#35995,#35996,#35997,
#35998,#35999,#36000,#36001,#36002,#36003,#36004,#36005,#36006,#36007,#36008,
#36009,#36010,#36011,#36012,#36013,#36014,#36015,#36016,#36017,#36018,#36019,
#36020,#36021,#36022,#36023,#36024,#36025,#36026),(#36027,#36028,#36029,
#36030,#36031,#36032,#36033,#36034,#36035,#36036,#36037,#36038,#36039,#36040,
#36041,#36042,#36043,#36044,#36045,#36046,#36047,#36048,#36049,#36050,#36051,
#36052,#36053,#36054,#36055,#36056,#36057,#36058,#36059,#36060,#36061,#36062,
#36063,#36064,#36065,#36066,#36067,#36068,#36069,#36070,#36071,#36072,#36073,
#36074,#36075,#36076,#36077,#36078,#36079,#36080,#36081,#36082,#36083,#36084,
#36085,#36086,#36087,#36088,#36089,#36090,#36091,#36092,#36093,#36094,#36095,
#36096,#36097,#36098,#36099,#36100,#36101,#36102,#36103,#36104,#36105,#36106,
#36107,#36108,#36109,#36110,#36111,#36112,#36113,#36114,#36115,#36116,#36117,
#36118,#36119,#36120,#36121,#36122,#36123,#36124,#36125,#36126,#36127,#36128,
#36129,#36130,#36131,#36132,#36133,#36134,#36135,#36136,#36137,#36138,#36139,
#36140,#36141,#36142,#36143,#36144,#36145,#36146,#36147,#36148),(#36149,
#36150,#36151,#36152,#36153,#36154,#36155,#36156,#36157,#36158,#36159,#36160,
#36161,#36162,#36163,#36164,#36165,#36166,#36167,#36168,#36169,#36170,#36171,
#36172,#36173,#36174,#36175,#36176,#36177,#36178,#36179,#36180,#36181,#36182,
#36183,#36184,#36185,#36186,#36187,#36188,#36189,#36190,#36191,#36192,#36193,
#36194,#36195,#36196,#36197,#36198,#36199,#36200,#36201,#36202,#36203,#36204,
#36205,#36206,#36207,#36208,#36209,#36210,#36211,#36212,#36213,#36214,#36215,
#36216,#36217,#36218,#36219,#36220,#36221,#36222,#36223,#36224,#36225,#36226,
#36227,#36228,#36229,#36230,#36231,#36232,#36233,#36234,#36235,#36236,#36237,
#36238,#36239,#36240,#36241,#36242,#36243,#36244,#36245,#36246,#36247,#36248,
#36249,#36250,#36251,#36252,#36253,#36254,#36255,#36256,#36257,#36258,#36259,
#36260,#36261,#36262,#36263,#36264,#36265,#36266,#36267,#36268,#36269,#36270),
(#36271,#36272,#36273,#36274,#36275,#36276,#36277,#36278,#36279,#36280,
#36281,#36282,#36283,#36284,#36285,#36286,#36287,#36288,#36289,#36290,#36291,
#36292,#36293,#36294,#36295,#36296,#36297,#36298,#36299,#36300,#36301,#36302,
#36303,#36304,#36305,#36306,#36307,#36308,#36309,#36310,#36311,#36312,#36313,
#36314,#36315,#36316,#36317,#36318,#36319,#36320,#36321,#36322,#36323,#36324,
#36325,#36326,#36327,#36328,#36329,#36330,#36331,#36332,#36333,#36334,#36335,
#36336,#36337,#36338,#36339,#36340,#36341,#36342,#36343,#36344,#36345,#36346,
#36347,#36348,#36349,#36350,#36351,#36352,#36353,#36354,#36355,#36356,#36357,
#36358,#36359,#36360,#36361,#36362,#36363,#36364,#36365,#36366,#36367,#36368,
#36369,#36370,#36371,#36372,#36373,#36374,#36375,#36376,#36377,#36378,#36379,
#36380,#36381,#36382,#36383,#36384,#36385,#36386,#36387,#36388,#36389,#36390,
#36391,#36392)),.UNSPECIFIED.,.F.,.F.,.F.,(4,4),(4,1,1,1,1,1,1,1,1,1,1,
1,1,1,1,1,1,1,1,1,1,1,1,1,1,1,1,1,1,1,1,1,1,1,1,1,1,1,1,1,1,1,1,1,1,1,1,
1,1,1,1,1,1,1,1,1,1,1,1,1,1,1,1,1,1,1,1,1,1,1,1,1,1,1,1,1,1,1,1,1,1,1,1,
1,1,1,1,1,1,1,1,1,1,1,1,1,1,1,1,1,1,1,1,1,1,1,1,1,1,1,1,1,1,1,1,1,1,1,1,
4),(0.,0.0448889834294937),(11.861580004257,12.8590786597075,13.856577315158,
14.8540759706085,15.851574626059,16.8490732815095,17.84657193696,18.8440705924105,
19.841569247861,20.8390679033115,21.836566558762,22.8340652142125,23.831563869663,
24.8290625251135,25.826561180564,26.8240598360145,27.821558491465,28.8190571469155,
29.816555802366,30.8140544578165,31.811553113267,32.8090517687175,33.806550424168,
34.8040490796185,35.801547735069,36.7990463905195,37.79654504597,38.7940437014205,
39.791542356871,40.7890410123215,41.786539667772,42.7840383232225,43.781536978673,
44.7790356341235,45.776534289574,46.7740329450245,47.771531600475,48.7690302559255,
49.766528911376,50.7640275668265,51.761526222277,52.7590248777275,53.756523533178,
54.7540221886285,55.751520844079,56.7490194995295,57.74651815498,58.7440168104305,
59.741515465881,60.7390141213315,61.736512776782,62.7340114322325,63.731510087683,
64.7290087431335,65.726507398584,66.7240060540345,67.721504709485,68.7190033649355,
69.716502020386,70.7140006758365,71.711499331287,72.7089979867375,73.706496642188,
74.7039952976385,75.701493953089,76.6989926085395,77.69649126399,78.6939899194405,
79.691488574891,80.6889872303415,81.686485885792,82.6839845412425,83.681483196693,
84.6789818521435,85.676480507594,86.6739791630445,87.671477818495,88.6689764739455,
89.666475129396,90.6639737848465,91.661472440297,92.6589710957475,93.656469751198,
94.6539684066485,95.651467062099,96.6489657175495,97.646464373,98.6439630284505,
99.641461683901,100.638960339352,101.636458994802,102.633957650253,103.631456305703,
104.628954961154,105.626453616604,106.623952272055,107.621450927505,108.618949582956,
109.616448238406,110.613946893857,111.611445549307,112.608944204758,113.606442860208,
114.603941515659,115.601440171109,116.59893882656,117.59643748201,118.593936137461,
119.591434792911,120.588933448362,121.586432103812,122.583930759263,123.581429414713,
124.578928070164,125.576426725614,126.573925381065,127.571424036515,128.568922691966,
129.566421347416,130.563920002867),.UNSPECIFIED.);
#247=B_SPLINE_SURFACE_WITH_KNOTS('',3,3,((#36500,#36501,#36502,#36503,#36504,
#36505,#36506,#36507,#36508,#36509,#36510,#36511,#36512,#36513,#36514,#36515,
#36516,#36517,#36518,#36519,#36520,#36521,#36522,#36523,#36524,#36525,#36526,
#36527,#36528,#36529,#36530,#36531,#36532,#36533,#36534,#36535,#36536,#36537,
#36538,#36539,#36540,#36541,#36542,#36543,#36544,#36545,#36546,#36547,#36548,
#36549,#36550,#36551,#36552,#36553,#36554,#36555,#36556,#36557,#36558,#36559,
#36560,#36561,#36562,#36563,#36564,#36565,#36566,#36567,#36568,#36569,#36570,
#36571,#36572,#36573,#36574,#36575,#36576,#36577,#36578,#36579,#36580,#36581,
#36582,#36583,#36584,#36585,#36586,#36587,#36588,#36589,#36590,#36591,#36592,
#36593,#36594,#36595,#36596,#36597,#36598,#36599,#36600,#36601,#36602,#36603,
#36604,#36605,#36606,#36607,#36608,#36609,#36610,#36611,#36612,#36613,#36614,
#36615,#36616,#36617,#36618,#36619,#36620,#36621),(#36622,#36623,#36624,
#36625,#36626,#36627,#36628,#36629,#36630,#36631,#36632,#36633,#36634,#36635,
#36636,#36637,#36638,#36639,#36640,#36641,#36642,#36643,#36644,#36645,#36646,
#36647,#36648,#36649,#36650,#36651,#36652,#36653,#36654,#36655,#36656,#36657,
#36658,#36659,#36660,#36661,#36662,#36663,#36664,#36665,#36666,#36667,#36668,
#36669,#36670,#36671,#36672,#36673,#36674,#36675,#36676,#36677,#36678,#36679,
#36680,#36681,#36682,#36683,#36684,#36685,#36686,#36687,#36688,#36689,#36690,
#36691,#36692,#36693,#36694,#36695,#36696,#36697,#36698,#36699,#36700,#36701,
#36702,#36703,#36704,#36705,#36706,#36707,#36708,#36709,#36710,#36711,#36712,
#36713,#36714,#36715,#36716,#36717,#36718,#36719,#36720,#36721,#36722,#36723,
#36724,#36725,#36726,#36727,#36728,#36729,#36730,#36731,#36732,#36733,#36734,
#36735,#36736,#36737,#36738,#36739,#36740,#36741,#36742,#36743),(#36744,
#36745,#36746,#36747,#36748,#36749,#36750,#36751,#36752,#36753,#36754,#36755,
#36756,#36757,#36758,#36759,#36760,#36761,#36762,#36763,#36764,#36765,#36766,
#36767,#36768,#36769,#36770,#36771,#36772,#36773,#36774,#36775,#36776,#36777,
#36778,#36779,#36780,#36781,#36782,#36783,#36784,#36785,#36786,#36787,#36788,
#36789,#36790,#36791,#36792,#36793,#36794,#36795,#36796,#36797,#36798,#36799,
#36800,#36801,#36802,#36803,#36804,#36805,#36806,#36807,#36808,#36809,#36810,
#36811,#36812,#36813,#36814,#36815,#36816,#36817,#36818,#36819,#36820,#36821,
#36822,#36823,#36824,#36825,#36826,#36827,#36828,#36829,#36830,#36831,#36832,
#36833,#36834,#36835,#36836,#36837,#36838,#36839,#36840,#36841,#36842,#36843,
#36844,#36845,#36846,#36847,#36848,#36849,#36850,#36851,#36852,#36853,#36854,
#36855,#36856,#36857,#36858,#36859,#36860,#36861,#36862,#36863,#36864,#36865),
(#36866,#36867,#36868,#36869,#36870,#36871,#36872,#36873,#36874,#36875,
#36876,#36877,#36878,#36879,#36880,#36881,#36882,#36883,#36884,#36885,#36886,
#36887,#36888,#36889,#36890,#36891,#36892,#36893,#36894,#36895,#36896,#36897,
#36898,#36899,#36900,#36901,#36902,#36903,#36904,#36905,#36906,#36907,#36908,
#36909,#36910,#36911,#36912,#36913,#36914,#36915,#36916,#36917,#36918,#36919,
#36920,#36921,#36922,#36923,#36924,#36925,#36926,#36927,#36928,#36929,#36930,
#36931,#36932,#36933,#36934,#36935,#36936,#36937,#36938,#36939,#36940,#36941,
#36942,#36943,#36944,#36945,#36946,#36947,#36948,#36949,#36950,#36951,#36952,
#36953,#36954,#36955,#36956,#36957,#36958,#36959,#36960,#36961,#36962,#36963,
#36964,#36965,#36966,#36967,#36968,#36969,#36970,#36971,#36972,#36973,#36974,
#36975,#36976,#36977,#36978,#36979,#36980,#36981,#36982,#36983,#36984,#36985,
#36986,#36987)),.UNSPECIFIED.,.F.,.F.,.F.,(4,4),(4,1,1,1,1,1,1,1,1,1,1,
1,1,1,1,1,1,1,1,1,1,1,1,1,1,1,1,1,1,1,1,1,1,1,1,1,1,1,1,1,1,1,1,1,1,1,1,
1,1,1,1,1,1,1,1,1,1,1,1,1,1,1,1,1,1,1,1,1,1,1,1,1,1,1,1,1,1,1,1,1,1,1,1,
1,1,1,1,1,1,1,1,1,1,1,1,1,1,1,1,1,1,1,1,1,1,1,1,1,1,1,1,1,1,1,1,1,1,1,1,
4),(0.,0.0448889834294937),(14.3981410127773,15.3956396682278,16.3931383236783,
17.3906369791288,18.3881356345793,19.3856342900298,20.3831329454803,21.3806316009308,
22.3781302563813,23.3756289118318,24.3731275672823,25.3706262227328,26.3681248781833,
27.3656235336338,28.3631221890843,29.3606208445348,30.3581194999853,31.3556181554358,
32.3531168108863,33.3506154663368,34.3481141217873,35.3456127772378,36.3431114326883,
37.3406100881388,38.3381087435893,39.3356073990398,40.3331060544903,41.3306047099408,
42.3281033653913,43.3256020208418,44.3231006762923,45.3205993317428,46.3180979871933,
47.3155966426438,48.3130952980943,49.3105939535448,50.3080926089953,51.3055912644458,
52.3030899198963,53.3005885753468,54.2980872307973,55.2955858862478,56.2930845416983,
57.2905831971488,58.2880818525993,59.2855805080498,60.2830791635003,61.2805778189508,
62.2780764744013,63.2755751298518,64.2730737853023,65.2705724407528,66.2680710962033,
67.2655697516538,68.2630684071043,69.2605670625549,70.2580657180054,71.2555643734559,
72.2530630289064,73.2505616843569,74.2480603398074,75.2455589952579,76.2430576507084,
77.2405563061589,78.2380549616094,79.2355536170598,80.2330522725103,81.2305509279608,
82.2280495834113,83.2255482388618,84.2230468943123,85.2205455497629,86.2180442052134,
87.2155428606639,88.2130415161144,89.2105401715649,90.2080388270154,91.2055374824659,
92.2030361379164,93.2005347933669,94.1980334488174,95.1955321042679,96.1930307597184,
97.1905294151689,98.1880280706194,99.1855267260699,100.18302538152,101.180524036971,
102.178022692421,103.175521347872,104.173020003322,105.170518658773,106.168017314223,
107.165515969674,108.163014625124,109.160513280575,110.158011936025,111.155510591476,
112.153009246926,113.150507902377,114.148006557827,115.145505213278,116.143003868728,
117.140502524179,118.138001179629,119.13549983508,120.13299849053,121.130497145981,
122.127995801431,123.125494456882,124.122993112332,125.120491767783,126.117990423233,
127.115489078684,128.112987734134,129.110486389585,130.107985045035,131.105483700486,
132.102982355936,133.100481011387),.UNSPECIFIED.);
#248=B_SPLINE_SURFACE_WITH_KNOTS('',3,3,((#37296,#37297,#37298,#37299,#37300,
#37301,#37302,#37303,#37304,#37305,#37306,#37307,#37308,#37309,#37310,#37311,
#37312,#37313,#37314,#37315,#37316,#37317,#37318,#37319,#37320,#37321,#37322,
#37323,#37324,#37325,#37326,#37327,#37328,#37329,#37330,#37331,#37332,#37333,
#37334,#37335,#37336,#37337,#37338,#37339,#37340,#37341,#37342,#37343,#37344,
#37345,#37346,#37347,#37348,#37349,#37350,#37351,#37352,#37353,#37354,#37355,
#37356,#37357,#37358,#37359,#37360,#37361,#37362,#37363,#37364,#37365,#37366,
#37367,#37368,#37369,#37370,#37371,#37372,#37373,#37374,#37375,#37376,#37377,
#37378,#37379,#37380,#37381,#37382,#37383,#37384,#37385,#37386,#37387,#37388,
#37389,#37390,#37391,#37392,#37393,#37394,#37395,#37396,#37397,#37398,#37399,
#37400,#37401,#37402,#37403,#37404,#37405,#37406,#37407,#37408,#37409,#37410,
#37411,#37412,#37413,#37414,#37415,#37416,#37417),(#37418,#37419,#37420,
#37421,#37422,#37423,#37424,#37425,#37426,#37427,#37428,#37429,#37430,#37431,
#37432,#37433,#37434,#37435,#37436,#37437,#37438,#37439,#37440,#37441,#37442,
#37443,#37444,#37445,#37446,#37447,#37448,#37449,#37450,#37451,#37452,#37453,
#37454,#37455,#37456,#37457,#37458,#37459,#37460,#37461,#37462,#37463,#37464,
#37465,#37466,#37467,#37468,#37469,#37470,#37471,#37472,#37473,#37474,#37475,
#37476,#37477,#37478,#37479,#37480,#37481,#37482,#37483,#37484,#37485,#37486,
#37487,#37488,#37489,#37490,#37491,#37492,#37493,#37494,#37495,#37496,#37497,
#37498,#37499,#37500,#37501,#37502,#37503,#37504,#37505,#37506,#37507,#37508,
#37509,#37510,#37511,#37512,#37513,#37514,#37515,#37516,#37517,#37518,#37519,
#37520,#37521,#37522,#37523,#37524,#37525,#37526,#37527,#37528,#37529,#37530,
#37531,#37532,#37533,#37534,#37535,#37536,#37537,#37538,#37539),(#37540,
#37541,#37542,#37543,#37544,#37545,#37546,#37547,#37548,#37549,#37550,#37551,
#37552,#37553,#37554,#37555,#37556,#37557,#37558,#37559,#37560,#37561,#37562,
#37563,#37564,#37565,#37566,#37567,#37568,#37569,#37570,#37571,#37572,#37573,
#37574,#37575,#37576,#37577,#37578,#37579,#37580,#37581,#37582,#37583,#37584,
#37585,#37586,#37587,#37588,#37589,#37590,#37591,#37592,#37593,#37594,#37595,
#37596,#37597,#37598,#37599,#37600,#37601,#37602,#37603,#37604,#37605,#37606,
#37607,#37608,#37609,#37610,#37611,#37612,#37613,#37614,#37615,#37616,#37617,
#37618,#37619,#37620,#37621,#37622,#37623,#37624,#37625,#37626,#37627,#37628,
#37629,#37630,#37631,#37632,#37633,#37634,#37635,#37636,#37637,#37638,#37639,
#37640,#37641,#37642,#37643,#37644,#37645,#37646,#37647,#37648,#37649,#37650,
#37651,#37652,#37653,#37654,#37655,#37656,#37657,#37658,#37659,#37660,#37661),
(#37662,#37663,#37664,#37665,#37666,#37667,#37668,#37669,#37670,#37671,
#37672,#37673,#37674,#37675,#37676,#37677,#37678,#37679,#37680,#37681,#37682,
#37683,#37684,#37685,#37686,#37687,#37688,#37689,#37690,#37691,#37692,#37693,
#37694,#37695,#37696,#37697,#37698,#37699,#37700,#37701,#37702,#37703,#37704,
#37705,#37706,#37707,#37708,#37709,#37710,#37711,#37712,#37713,#37714,#37715,
#37716,#37717,#37718,#37719,#37720,#37721,#37722,#37723,#37724,#37725,#37726,
#37727,#37728,#37729,#37730,#37731,#37732,#37733,#37734,#37735,#37736,#37737,
#37738,#37739,#37740,#37741,#37742,#37743,#37744,#37745,#37746,#37747,#37748,
#37749,#37750,#37751,#37752,#37753,#37754,#37755,#37756,#37757,#37758,#37759,
#37760,#37761,#37762,#37763,#37764,#37765,#37766,#37767,#37768,#37769,#37770,
#37771,#37772,#37773,#37774,#37775,#37776,#37777,#37778,#37779,#37780,#37781,
#37782,#37783)),.UNSPECIFIED.,.F.,.F.,.F.,(4,4),(4,1,1,1,1,1,1,1,1,1,1,
1,1,1,1,1,1,1,1,1,1,1,1,1,1,1,1,1,1,1,1,1,1,1,1,1,1,1,1,1,1,1,1,1,1,1,1,
1,1,1,1,1,1,1,1,1,1,1,1,1,1,1,1,1,1,1,1,1,1,1,1,1,1,1,1,1,1,1,1,1,1,1,1,
1,1,1,1,1,1,1,1,1,1,1,1,1,1,1,1,1,1,1,1,1,1,1,1,1,1,1,1,1,1,1,1,1,1,1,1,
4),(0.,0.0448889834294937),(11.8615800042567,12.8590786597072,13.8565773151577,
14.8540759706082,15.8515746260587,16.8490732815092,17.8465719369597,18.8440705924102,
19.8415692478607,20.8390679033112,21.8365665587617,22.8340652142122,23.8315638696627,
24.8290625251132,25.8265611805637,26.8240598360142,27.8215584914647,28.8190571469152,
29.8165558023657,30.8140544578162,31.8115531132667,32.8090517687172,33.8065504241677,
34.8040490796182,35.8015477350687,36.7990463905192,37.7965450459697,38.7940437014202,
39.7915423568707,40.7890410123212,41.7865396677717,42.7840383232222,43.7815369786727,
44.7790356341232,45.7765342895737,46.7740329450242,47.7715316004747,48.7690302559252,
49.7665289113757,50.7640275668262,51.7615262222767,52.7590248777272,53.7565235331777,
54.7540221886282,55.7515208440787,56.7490194995292,57.7465181549797,58.7440168104302,
59.7415154658807,60.7390141213312,61.7365127767817,62.7340114322322,63.7315100876827,
64.7290087431332,65.7265073985837,66.7240060540342,67.7215047094847,68.7190033649352,
69.7165020203857,70.7140006758362,71.7114993312867,72.7089979867372,73.7064966421877,
74.7039952976382,75.7014939530887,76.6989926085392,77.6964912639897,78.6939899194402,
79.6914885748908,80.6889872303413,81.6864858857918,82.6839845412423,83.6814831966928,
84.6789818521433,85.6764805075938,86.6739791630443,87.6714778184948,88.6689764739453,
89.6664751293958,90.6639737848463,91.6614724402968,92.6589710957473,93.6564697511978,
94.6539684066483,95.6514670620988,96.6489657175493,97.6464643729998,98.6439630284503,
99.6414616839008,100.638960339351,101.636458994802,102.633957650252,103.631456305703,
104.628954961153,105.626453616604,106.623952272054,107.621450927505,108.618949582955,
109.616448238406,110.613946893856,111.611445549307,112.608944204757,113.606442860208,
114.603941515658,115.601440171109,116.598938826559,117.59643748201,118.59393613746,
119.591434792911,120.588933448361,121.586432103812,122.583930759262,123.581429414713,
124.578928070163,125.576426725614,126.573925381064,127.571424036515,128.568922691965,
129.566421347416,130.563920002866),.UNSPECIFIED.);
#249=B_SPLINE_SURFACE_WITH_KNOTS('',3,3,((#37891,#37892,#37893,#37894,#37895,
#37896,#37897,#37898,#37899,#37900,#37901,#37902,#37903,#37904,#37905,#37906,
#37907,#37908,#37909,#37910,#37911,#37912,#37913,#37914,#37915,#37916,#37917,
#37918,#37919,#37920,#37921,#37922,#37923,#37924,#37925,#37926,#37927,#37928,
#37929,#37930,#37931,#37932,#37933,#37934,#37935,#37936,#37937,#37938,#37939,
#37940,#37941,#37942,#37943,#37944,#37945,#37946,#37947,#37948,#37949,#37950,
#37951,#37952,#37953,#37954,#37955,#37956,#37957,#37958,#37959,#37960,#37961,
#37962,#37963,#37964,#37965,#37966,#37967,#37968,#37969,#37970,#37971,#37972,
#37973,#37974,#37975,#37976,#37977,#37978,#37979,#37980,#37981,#37982,#37983,
#37984,#37985,#37986,#37987,#37988,#37989,#37990,#37991,#37992,#37993,#37994,
#37995,#37996,#37997,#37998,#37999,#38000,#38001,#38002,#38003,#38004,#38005,
#38006,#38007,#38008,#38009,#38010,#38011,#38012),(#38013,#38014,#38015,
#38016,#38017,#38018,#38019,#38020,#38021,#38022,#38023,#38024,#38025,#38026,
#38027,#38028,#38029,#38030,#38031,#38032,#38033,#38034,#38035,#38036,#38037,
#38038,#38039,#38040,#38041,#38042,#38043,#38044,#38045,#38046,#38047,#38048,
#38049,#38050,#38051,#38052,#38053,#38054,#38055,#38056,#38057,#38058,#38059,
#38060,#38061,#38062,#38063,#38064,#38065,#38066,#38067,#38068,#38069,#38070,
#38071,#38072,#38073,#38074,#38075,#38076,#38077,#38078,#38079,#38080,#38081,
#38082,#38083,#38084,#38085,#38086,#38087,#38088,#38089,#38090,#38091,#38092,
#38093,#38094,#38095,#38096,#38097,#38098,#38099,#38100,#38101,#38102,#38103,
#38104,#38105,#38106,#38107,#38108,#38109,#38110,#38111,#38112,#38113,#38114,
#38115,#38116,#38117,#38118,#38119,#38120,#38121,#38122,#38123,#38124,#38125,
#38126,#38127,#38128,#38129,#38130,#38131,#38132,#38133,#38134),(#38135,
#38136,#38137,#38138,#38139,#38140,#38141,#38142,#38143,#38144,#38145,#38146,
#38147,#38148,#38149,#38150,#38151,#38152,#38153,#38154,#38155,#38156,#38157,
#38158,#38159,#38160,#38161,#38162,#38163,#38164,#38165,#38166,#38167,#38168,
#38169,#38170,#38171,#38172,#38173,#38174,#38175,#38176,#38177,#38178,#38179,
#38180,#38181,#38182,#38183,#38184,#38185,#38186,#38187,#38188,#38189,#38190,
#38191,#38192,#38193,#38194,#38195,#38196,#38197,#38198,#38199,#38200,#38201,
#38202,#38203,#38204,#38205,#38206,#38207,#38208,#38209,#38210,#38211,#38212,
#38213,#38214,#38215,#38216,#38217,#38218,#38219,#38220,#38221,#38222,#38223,
#38224,#38225,#38226,#38227,#38228,#38229,#38230,#38231,#38232,#38233,#38234,
#38235,#38236,#38237,#38238,#38239,#38240,#38241,#38242,#38243,#38244,#38245,
#38246,#38247,#38248,#38249,#38250,#38251,#38252,#38253,#38254,#38255,#38256),
(#38257,#38258,#38259,#38260,#38261,#38262,#38263,#38264,#38265,#38266,
#38267,#38268,#38269,#38270,#38271,#38272,#38273,#38274,#38275,#38276,#38277,
#38278,#38279,#38280,#38281,#38282,#38283,#38284,#38285,#38286,#38287,#38288,
#38289,#38290,#38291,#38292,#38293,#38294,#38295,#38296,#38297,#38298,#38299,
#38300,#38301,#38302,#38303,#38304,#38305,#38306,#38307,#38308,#38309,#38310,
#38311,#38312,#38313,#38314,#38315,#38316,#38317,#38318,#38319,#38320,#38321,
#38322,#38323,#38324,#38325,#38326,#38327,#38328,#38329,#38330,#38331,#38332,
#38333,#38334,#38335,#38336,#38337,#38338,#38339,#38340,#38341,#38342,#38343,
#38344,#38345,#38346,#38347,#38348,#38349,#38350,#38351,#38352,#38353,#38354,
#38355,#38356,#38357,#38358,#38359,#38360,#38361,#38362,#38363,#38364,#38365,
#38366,#38367,#38368,#38369,#38370,#38371,#38372,#38373,#38374,#38375,#38376,
#38377,#38378)),.UNSPECIFIED.,.F.,.F.,.F.,(4,4),(4,1,1,1,1,1,1,1,1,1,1,
1,1,1,1,1,1,1,1,1,1,1,1,1,1,1,1,1,1,1,1,1,1,1,1,1,1,1,1,1,1,1,1,1,1,1,1,
1,1,1,1,1,1,1,1,1,1,1,1,1,1,1,1,1,1,1,1,1,1,1,1,1,1,1,1,1,1,1,1,1,1,1,1,
1,1,1,1,1,1,1,1,1,1,1,1,1,1,1,1,1,1,1,1,1,1,1,1,1,1,1,1,1,1,1,1,1,1,1,1,
4),(0.,0.0448889834294937),(14.3981410127769,15.3956396682274,16.3931383236779,
17.3906369791284,18.3881356345789,19.3856342900294,20.3831329454799,21.3806316009304,
22.3781302563809,23.3756289118314,24.3731275672819,25.3706262227324,26.3681248781829,
27.3656235336334,28.3631221890839,29.3606208445344,30.3581194999849,31.3556181554354,
32.3531168108859,33.3506154663364,34.3481141217869,35.3456127772374,36.3431114326879,
37.3406100881384,38.3381087435889,39.3356073990394,40.3331060544899,41.3306047099404,
42.3281033653909,43.3256020208414,44.3231006762919,45.3205993317424,46.3180979871929,
47.3155966426434,48.3130952980939,49.3105939535444,50.3080926089949,51.3055912644454,
52.3030899198959,53.3005885753464,54.2980872307969,55.2955858862474,56.2930845416979,
57.2905831971484,58.2880818525989,59.2855805080494,60.2830791634999,61.2805778189504,
62.2780764744009,63.2755751298514,64.2730737853019,65.2705724407524,66.2680710962029,
67.2655697516534,68.2630684071039,69.2605670625544,70.2580657180049,71.2555643734554,
72.2530630289059,73.2505616843565,74.248060339807,75.2455589952575,76.243057650708,
77.2405563061585,78.238054961609,79.2355536170595,80.23305227251,81.2305509279605,
82.228049583411,83.2255482388615,84.223046894312,85.2205455497625,86.218044205213,
87.2155428606635,88.213041516114,89.2105401715645,90.208038827015,91.2055374824655,
92.203036137916,93.2005347933665,94.198033448817,95.1955321042675,96.193030759718,
97.1905294151685,98.188028070619,99.1855267260695,100.18302538152,101.18052403697,
102.178022692421,103.175521347871,104.173020003322,105.170518658772,106.168017314223,
107.165515969673,108.163014625124,109.160513280574,110.158011936025,111.155510591476,
112.153009246926,113.150507902377,114.148006557827,115.145505213278,116.143003868728,
117.140502524179,118.138001179629,119.13549983508,120.13299849053,121.130497145981,
122.127995801431,123.125494456882,124.122993112332,125.120491767783,126.117990423233,
127.115489078684,128.112987734134,129.110486389585,130.107985045035,131.105483700486,
132.102982355936,133.100481011387),.UNSPECIFIED.);
#250=B_SPLINE_SURFACE_WITH_KNOTS('',3,3,((#38683,#38684,#38685,#38686,#38687,
#38688,#38689,#38690,#38691,#38692,#38693,#38694,#38695,#38696,#38697,#38698,
#38699,#38700,#38701,#38702,#38703,#38704,#38705,#38706,#38707,#38708,#38709,
#38710,#38711,#38712,#38713,#38714,#38715,#38716,#38717,#38718,#38719,#38720,
#38721,#38722,#38723,#38724,#38725,#38726,#38727,#38728,#38729,#38730,#38731,
#38732,#38733,#38734,#38735,#38736,#38737,#38738,#38739,#38740,#38741,#38742,
#38743,#38744,#38745,#38746,#38747,#38748,#38749,#38750,#38751,#38752,#38753,
#38754,#38755,#38756,#38757,#38758,#38759,#38760,#38761,#38762,#38763,#38764,
#38765,#38766,#38767,#38768,#38769,#38770,#38771,#38772,#38773,#38774,#38775,
#38776,#38777,#38778,#38779,#38780,#38781,#38782,#38783,#38784,#38785,#38786,
#38787,#38788,#38789,#38790,#38791,#38792,#38793,#38794,#38795,#38796,#38797,
#38798,#38799,#38800,#38801,#38802,#38803,#38804),(#38805,#38806,#38807,
#38808,#38809,#38810,#38811,#38812,#38813,#38814,#38815,#38816,#38817,#38818,
#38819,#38820,#38821,#38822,#38823,#38824,#38825,#38826,#38827,#38828,#38829,
#38830,#38831,#38832,#38833,#38834,#38835,#38836,#38837,#38838,#38839,#38840,
#38841,#38842,#38843,#38844,#38845,#38846,#38847,#38848,#38849,#38850,#38851,
#38852,#38853,#38854,#38855,#38856,#38857,#38858,#38859,#38860,#38861,#38862,
#38863,#38864,#38865,#38866,#38867,#38868,#38869,#38870,#38871,#38872,#38873,
#38874,#38875,#38876,#38877,#38878,#38879,#38880,#38881,#38882,#38883,#38884,
#38885,#38886,#38887,#38888,#38889,#38890,#38891,#38892,#38893,#38894,#38895,
#38896,#38897,#38898,#38899,#38900,#38901,#38902,#38903,#38904,#38905,#38906,
#38907,#38908,#38909,#38910,#38911,#38912,#38913,#38914,#38915,#38916,#38917,
#38918,#38919,#38920,#38921,#38922,#38923,#38924,#38925,#38926),(#38927,
#38928,#38929,#38930,#38931,#38932,#38933,#38934,#38935,#38936,#38937,#38938,
#38939,#38940,#38941,#38942,#38943,#38944,#38945,#38946,#38947,#38948,#38949,
#38950,#38951,#38952,#38953,#38954,#38955,#38956,#38957,#38958,#38959,#38960,
#38961,#38962,#38963,#38964,#38965,#38966,#38967,#38968,#38969,#38970,#38971,
#38972,#38973,#38974,#38975,#38976,#38977,#38978,#38979,#38980,#38981,#38982,
#38983,#38984,#38985,#38986,#38987,#38988,#38989,#38990,#38991,#38992,#38993,
#38994,#38995,#38996,#38997,#38998,#38999,#39000,#39001,#39002,#39003,#39004,
#39005,#39006,#39007,#39008,#39009,#39010,#39011,#39012,#39013,#39014,#39015,
#39016,#39017,#39018,#39019,#39020,#39021,#39022,#39023,#39024,#39025,#39026,
#39027,#39028,#39029,#39030,#39031,#39032,#39033,#39034,#39035,#39036,#39037,
#39038,#39039,#39040,#39041,#39042,#39043,#39044,#39045,#39046,#39047,#39048),
(#39049,#39050,#39051,#39052,#39053,#39054,#39055,#39056,#39057,#39058,
#39059,#39060,#39061,#39062,#39063,#39064,#39065,#39066,#39067,#39068,#39069,
#39070,#39071,#39072,#39073,#39074,#39075,#39076,#39077,#39078,#39079,#39080,
#39081,#39082,#39083,#39084,#39085,#39086,#39087,#39088,#39089,#39090,#39091,
#39092,#39093,#39094,#39095,#39096,#39097,#39098,#39099,#39100,#39101,#39102,
#39103,#39104,#39105,#39106,#39107,#39108,#39109,#39110,#39111,#39112,#39113,
#39114,#39115,#39116,#39117,#39118,#39119,#39120,#39121,#39122,#39123,#39124,
#39125,#39126,#39127,#39128,#39129,#39130,#39131,#39132,#39133,#39134,#39135,
#39136,#39137,#39138,#39139,#39140,#39141,#39142,#39143,#39144,#39145,#39146,
#39147,#39148,#39149,#39150,#39151,#39152,#39153,#39154,#39155,#39156,#39157,
#39158,#39159,#39160,#39161,#39162,#39163,#39164,#39165,#39166,#39167,#39168,
#39169,#39170)),.UNSPECIFIED.,.F.,.F.,.F.,(4,4),(4,1,1,1,1,1,1,1,1,1,1,
1,1,1,1,1,1,1,1,1,1,1,1,1,1,1,1,1,1,1,1,1,1,1,1,1,1,1,1,1,1,1,1,1,1,1,1,
1,1,1,1,1,1,1,1,1,1,1,1,1,1,1,1,1,1,1,1,1,1,1,1,1,1,1,1,1,1,1,1,1,1,1,1,
1,1,1,1,1,1,1,1,1,1,1,1,1,1,1,1,1,1,1,1,1,1,1,1,1,1,1,1,1,1,1,1,1,1,1,1,
4),(0.,0.0448889834294937),(11.8615800042567,12.8590786597072,13.8565773151577,
14.8540759706082,15.8515746260587,16.8490732815092,17.8465719369597,18.8440705924102,
19.8415692478607,20.8390679033112,21.8365665587617,22.8340652142122,23.8315638696627,
24.8290625251132,25.8265611805637,26.8240598360142,27.8215584914647,28.8190571469152,
29.8165558023657,30.8140544578162,31.8115531132667,32.8090517687172,33.8065504241677,
34.8040490796182,35.8015477350687,36.7990463905192,37.7965450459697,38.7940437014202,
39.7915423568707,40.7890410123212,41.7865396677717,42.7840383232222,43.7815369786727,
44.7790356341232,45.7765342895737,46.7740329450242,47.7715316004747,48.7690302559252,
49.7665289113757,50.7640275668262,51.7615262222767,52.7590248777272,53.7565235331777,
54.7540221886282,55.7515208440787,56.7490194995292,57.7465181549797,58.7440168104302,
59.7415154658807,60.7390141213312,61.7365127767817,62.7340114322322,63.7315100876827,
64.7290087431332,65.7265073985837,66.7240060540342,67.7215047094847,68.7190033649352,
69.7165020203857,70.7140006758362,71.7114993312867,72.7089979867372,73.7064966421877,
74.7039952976382,75.7014939530887,76.6989926085392,77.6964912639897,78.6939899194402,
79.6914885748908,80.6889872303413,81.6864858857918,82.6839845412423,83.6814831966928,
84.6789818521433,85.6764805075938,86.6739791630443,87.6714778184948,88.6689764739453,
89.6664751293958,90.6639737848463,91.6614724402968,92.6589710957473,93.6564697511978,
94.6539684066483,95.6514670620988,96.6489657175493,97.6464643729998,98.6439630284503,
99.6414616839008,100.638960339351,101.636458994802,102.633957650252,103.631456305703,
104.628954961153,105.626453616604,106.623952272054,107.621450927505,108.618949582955,
109.616448238406,110.613946893856,111.611445549307,112.608944204757,113.606442860208,
114.603941515658,115.601440171109,116.598938826559,117.59643748201,118.59393613746,
119.591434792911,120.588933448361,121.586432103812,122.583930759262,123.581429414713,
124.578928070163,125.576426725614,126.573925381064,127.571424036515,128.568922691965,
129.566421347416,130.563920002866),.UNSPECIFIED.);
#251=B_SPLINE_SURFACE_WITH_KNOTS('',3,3,((#39278,#39279,#39280,#39281,#39282,
#39283,#39284,#39285,#39286,#39287,#39288,#39289,#39290,#39291,#39292,#39293,
#39294,#39295,#39296,#39297,#39298,#39299,#39300,#39301,#39302,#39303,#39304,
#39305,#39306,#39307,#39308,#39309,#39310,#39311,#39312,#39313,#39314,#39315,
#39316,#39317,#39318,#39319,#39320,#39321,#39322,#39323,#39324,#39325,#39326,
#39327,#39328,#39329,#39330,#39331,#39332,#39333,#39334,#39335,#39336,#39337,
#39338,#39339,#39340,#39341,#39342,#39343,#39344,#39345,#39346,#39347,#39348,
#39349,#39350,#39351,#39352,#39353,#39354,#39355,#39356,#39357,#39358,#39359,
#39360,#39361,#39362,#39363,#39364,#39365,#39366,#39367,#39368,#39369,#39370,
#39371,#39372,#39373,#39374,#39375,#39376,#39377,#39378,#39379,#39380,#39381,
#39382,#39383,#39384,#39385,#39386,#39387,#39388,#39389,#39390,#39391,#39392,
#39393,#39394,#39395,#39396,#39397,#39398,#39399),(#39400,#39401,#39402,
#39403,#39404,#39405,#39406,#39407,#39408,#39409,#39410,#39411,#39412,#39413,
#39414,#39415,#39416,#39417,#39418,#39419,#39420,#39421,#39422,#39423,#39424,
#39425,#39426,#39427,#39428,#39429,#39430,#39431,#39432,#39433,#39434,#39435,
#39436,#39437,#39438,#39439,#39440,#39441,#39442,#39443,#39444,#39445,#39446,
#39447,#39448,#39449,#39450,#39451,#39452,#39453,#39454,#39455,#39456,#39457,
#39458,#39459,#39460,#39461,#39462,#39463,#39464,#39465,#39466,#39467,#39468,
#39469,#39470,#39471,#39472,#39473,#39474,#39475,#39476,#39477,#39478,#39479,
#39480,#39481,#39482,#39483,#39484,#39485,#39486,#39487,#39488,#39489,#39490,
#39491,#39492,#39493,#39494,#39495,#39496,#39497,#39498,#39499,#39500,#39501,
#39502,#39503,#39504,#39505,#39506,#39507,#39508,#39509,#39510,#39511,#39512,
#39513,#39514,#39515,#39516,#39517,#39518,#39519,#39520,#39521),(#39522,
#39523,#39524,#39525,#39526,#39527,#39528,#39529,#39530,#39531,#39532,#39533,
#39534,#39535,#39536,#39537,#39538,#39539,#39540,#39541,#39542,#39543,#39544,
#39545,#39546,#39547,#39548,#39549,#39550,#39551,#39552,#39553,#39554,#39555,
#39556,#39557,#39558,#39559,#39560,#39561,#39562,#39563,#39564,#39565,#39566,
#39567,#39568,#39569,#39570,#39571,#39572,#39573,#39574,#39575,#39576,#39577,
#39578,#39579,#39580,#39581,#39582,#39583,#39584,#39585,#39586,#39587,#39588,
#39589,#39590,#39591,#39592,#39593,#39594,#39595,#39596,#39597,#39598,#39599,
#39600,#39601,#39602,#39603,#39604,#39605,#39606,#39607,#39608,#39609,#39610,
#39611,#39612,#39613,#39614,#39615,#39616,#39617,#39618,#39619,#39620,#39621,
#39622,#39623,#39624,#39625,#39626,#39627,#39628,#39629,#39630,#39631,#39632,
#39633,#39634,#39635,#39636,#39637,#39638,#39639,#39640,#39641,#39642,#39643),
(#39644,#39645,#39646,#39647,#39648,#39649,#39650,#39651,#39652,#39653,
#39654,#39655,#39656,#39657,#39658,#39659,#39660,#39661,#39662,#39663,#39664,
#39665,#39666,#39667,#39668,#39669,#39670,#39671,#39672,#39673,#39674,#39675,
#39676,#39677,#39678,#39679,#39680,#39681,#39682,#39683,#39684,#39685,#39686,
#39687,#39688,#39689,#39690,#39691,#39692,#39693,#39694,#39695,#39696,#39697,
#39698,#39699,#39700,#39701,#39702,#39703,#39704,#39705,#39706,#39707,#39708,
#39709,#39710,#39711,#39712,#39713,#39714,#39715,#39716,#39717,#39718,#39719,
#39720,#39721,#39722,#39723,#39724,#39725,#39726,#39727,#39728,#39729,#39730,
#39731,#39732,#39733,#39734,#39735,#39736,#39737,#39738,#39739,#39740,#39741,
#39742,#39743,#39744,#39745,#39746,#39747,#39748,#39749,#39750,#39751,#39752,
#39753,#39754,#39755,#39756,#39757,#39758,#39759,#39760,#39761,#39762,#39763,
#39764,#39765)),.UNSPECIFIED.,.F.,.F.,.F.,(4,4),(4,1,1,1,1,1,1,1,1,1,1,
1,1,1,1,1,1,1,1,1,1,1,1,1,1,1,1,1,1,1,1,1,1,1,1,1,1,1,1,1,1,1,1,1,1,1,1,
1,1,1,1,1,1,1,1,1,1,1,1,1,1,1,1,1,1,1,1,1,1,1,1,1,1,1,1,1,1,1,1,1,1,1,1,
1,1,1,1,1,1,1,1,1,1,1,1,1,1,1,1,1,1,1,1,1,1,1,1,1,1,1,1,1,1,1,1,1,1,1,1,
4),(0.,0.0448889834294937),(14.3981410127769,15.3956396682274,16.3931383236779,
17.3906369791284,18.3881356345789,19.3856342900294,20.3831329454799,21.3806316009304,
22.3781302563809,23.3756289118314,24.3731275672819,25.3706262227324,26.3681248781829,
27.3656235336334,28.3631221890839,29.3606208445344,30.3581194999849,31.3556181554354,
32.3531168108859,33.3506154663364,34.3481141217869,35.3456127772374,36.3431114326879,
37.3406100881384,38.3381087435889,39.3356073990394,40.3331060544899,41.3306047099404,
42.3281033653909,43.3256020208414,44.3231006762919,45.3205993317424,46.3180979871929,
47.3155966426434,48.3130952980939,49.3105939535444,50.3080926089949,51.3055912644454,
52.3030899198959,53.3005885753464,54.2980872307969,55.2955858862474,56.2930845416979,
57.2905831971484,58.2880818525989,59.2855805080494,60.2830791634999,61.2805778189504,
62.2780764744009,63.2755751298514,64.2730737853019,65.2705724407524,66.2680710962029,
67.2655697516534,68.2630684071039,69.2605670625544,70.2580657180049,71.2555643734554,
72.2530630289059,73.2505616843565,74.248060339807,75.2455589952575,76.243057650708,
77.2405563061585,78.238054961609,79.2355536170595,80.23305227251,81.2305509279605,
82.228049583411,83.2255482388615,84.223046894312,85.2205455497625,86.218044205213,
87.2155428606635,88.213041516114,89.2105401715645,90.208038827015,91.2055374824655,
92.203036137916,93.2005347933665,94.198033448817,95.1955321042675,96.193030759718,
97.1905294151685,98.188028070619,99.1855267260695,100.18302538152,101.18052403697,
102.178022692421,103.175521347871,104.173020003322,105.170518658772,106.168017314223,
107.165515969673,108.163014625124,109.160513280574,110.158011936025,111.155510591476,
112.153009246926,113.150507902377,114.148006557827,115.145505213278,116.143003868728,
117.140502524179,118.138001179629,119.13549983508,120.13299849053,121.130497145981,
122.127995801431,123.125494456882,124.122993112332,125.120491767783,126.117990423233,
127.115489078684,128.112987734134,129.110486389585,130.107985045035,131.105483700486,
132.102982355936,133.100481011387),.UNSPECIFIED.);
#252=B_SPLINE_SURFACE_WITH_KNOTS('',3,3,((#40070,#40071,#40072,#40073,#40074,
#40075,#40076,#40077,#40078,#40079,#40080,#40081,#40082,#40083,#40084,#40085,
#40086,#40087,#40088,#40089,#40090,#40091,#40092,#40093,#40094,#40095,#40096,
#40097,#40098,#40099,#40100,#40101,#40102,#40103,#40104,#40105,#40106,#40107,
#40108,#40109,#40110,#40111,#40112,#40113,#40114,#40115,#40116,#40117,#40118,
#40119,#40120,#40121,#40122,#40123,#40124,#40125,#40126,#40127,#40128,#40129,
#40130,#40131,#40132,#40133,#40134,#40135,#40136,#40137,#40138,#40139,#40140,
#40141,#40142,#40143,#40144,#40145,#40146,#40147,#40148,#40149,#40150,#40151,
#40152,#40153,#40154,#40155,#40156,#40157,#40158,#40159,#40160,#40161,#40162,
#40163,#40164,#40165,#40166,#40167,#40168,#40169,#40170,#40171,#40172,#40173,
#40174,#40175,#40176,#40177,#40178,#40179,#40180,#40181,#40182,#40183,#40184,
#40185,#40186,#40187,#40188,#40189,#40190,#40191),(#40192,#40193,#40194,
#40195,#40196,#40197,#40198,#40199,#40200,#40201,#40202,#40203,#40204,#40205,
#40206,#40207,#40208,#40209,#40210,#40211,#40212,#40213,#40214,#40215,#40216,
#40217,#40218,#40219,#40220,#40221,#40222,#40223,#40224,#40225,#40226,#40227,
#40228,#40229,#40230,#40231,#40232,#40233,#40234,#40235,#40236,#40237,#40238,
#40239,#40240,#40241,#40242,#40243,#40244,#40245,#40246,#40247,#40248,#40249,
#40250,#40251,#40252,#40253,#40254,#40255,#40256,#40257,#40258,#40259,#40260,
#40261,#40262,#40263,#40264,#40265,#40266,#40267,#40268,#40269,#40270,#40271,
#40272,#40273,#40274,#40275,#40276,#40277,#40278,#40279,#40280,#40281,#40282,
#40283,#40284,#40285,#40286,#40287,#40288,#40289,#40290,#40291,#40292,#40293,
#40294,#40295,#40296,#40297,#40298,#40299,#40300,#40301,#40302,#40303,#40304,
#40305,#40306,#40307,#40308,#40309,#40310,#40311,#40312,#40313),(#40314,
#40315,#40316,#40317,#40318,#40319,#40320,#40321,#40322,#40323,#40324,#40325,
#40326,#40327,#40328,#40329,#40330,#40331,#40332,#40333,#40334,#40335,#40336,
#40337,#40338,#40339,#40340,#40341,#40342,#40343,#40344,#40345,#40346,#40347,
#40348,#40349,#40350,#40351,#40352,#40353,#40354,#40355,#40356,#40357,#40358,
#40359,#40360,#40361,#40362,#40363,#40364,#40365,#40366,#40367,#40368,#40369,
#40370,#40371,#40372,#40373,#40374,#40375,#40376,#40377,#40378,#40379,#40380,
#40381,#40382,#40383,#40384,#40385,#40386,#40387,#40388,#40389,#40390,#40391,
#40392,#40393,#40394,#40395,#40396,#40397,#40398,#40399,#40400,#40401,#40402,
#40403,#40404,#40405,#40406,#40407,#40408,#40409,#40410,#40411,#40412,#40413,
#40414,#40415,#40416,#40417,#40418,#40419,#40420,#40421,#40422,#40423,#40424,
#40425,#40426,#40427,#40428,#40429,#40430,#40431,#40432,#40433,#40434,#40435),
(#40436,#40437,#40438,#40439,#40440,#40441,#40442,#40443,#40444,#40445,
#40446,#40447,#40448,#40449,#40450,#40451,#40452,#40453,#40454,#40455,#40456,
#40457,#40458,#40459,#40460,#40461,#40462,#40463,#40464,#40465,#40466,#40467,
#40468,#40469,#40470,#40471,#40472,#40473,#40474,#40475,#40476,#40477,#40478,
#40479,#40480,#40481,#40482,#40483,#40484,#40485,#40486,#40487,#40488,#40489,
#40490,#40491,#40492,#40493,#40494,#40495,#40496,#40497,#40498,#40499,#40500,
#40501,#40502,#40503,#40504,#40505,#40506,#40507,#40508,#40509,#40510,#40511,
#40512,#40513,#40514,#40515,#40516,#40517,#40518,#40519,#40520,#40521,#40522,
#40523,#40524,#40525,#40526,#40527,#40528,#40529,#40530,#40531,#40532,#40533,
#40534,#40535,#40536,#40537,#40538,#40539,#40540,#40541,#40542,#40543,#40544,
#40545,#40546,#40547,#40548,#40549,#40550,#40551,#40552,#40553,#40554,#40555,
#40556,#40557)),.UNSPECIFIED.,.F.,.F.,.F.,(4,4),(4,1,1,1,1,1,1,1,1,1,1,
1,1,1,1,1,1,1,1,1,1,1,1,1,1,1,1,1,1,1,1,1,1,1,1,1,1,1,1,1,1,1,1,1,1,1,1,
1,1,1,1,1,1,1,1,1,1,1,1,1,1,1,1,1,1,1,1,1,1,1,1,1,1,1,1,1,1,1,1,1,1,1,1,
1,1,1,1,1,1,1,1,1,1,1,1,1,1,1,1,1,1,1,1,1,1,1,1,1,1,1,1,1,1,1,1,1,1,1,1,
4),(0.,0.0448889834294937),(11.8615800042567,12.8590786597072,13.8565773151577,
14.8540759706082,15.8515746260587,16.8490732815092,17.8465719369597,18.8440705924102,
19.8415692478607,20.8390679033112,21.8365665587617,22.8340652142122,23.8315638696627,
24.8290625251132,25.8265611805637,26.8240598360142,27.8215584914647,28.8190571469152,
29.8165558023657,30.8140544578162,31.8115531132667,32.8090517687172,33.8065504241677,
34.8040490796182,35.8015477350687,36.7990463905192,37.7965450459697,38.7940437014202,
39.7915423568707,40.7890410123212,41.7865396677717,42.7840383232222,43.7815369786727,
44.7790356341232,45.7765342895737,46.7740329450242,47.7715316004747,48.7690302559252,
49.7665289113757,50.7640275668262,51.7615262222767,52.7590248777272,53.7565235331777,
54.7540221886282,55.7515208440787,56.7490194995292,57.7465181549797,58.7440168104302,
59.7415154658807,60.7390141213312,61.7365127767817,62.7340114322322,63.7315100876827,
64.7290087431332,65.7265073985837,66.7240060540342,67.7215047094847,68.7190033649352,
69.7165020203857,70.7140006758362,71.7114993312867,72.7089979867372,73.7064966421877,
74.7039952976382,75.7014939530887,76.6989926085392,77.6964912639897,78.6939899194402,
79.6914885748908,80.6889872303413,81.6864858857918,82.6839845412423,83.6814831966928,
84.6789818521433,85.6764805075938,86.6739791630443,87.6714778184948,88.6689764739453,
89.6664751293958,90.6639737848463,91.6614724402968,92.6589710957473,93.6564697511978,
94.6539684066483,95.6514670620988,96.6489657175493,97.6464643729998,98.6439630284503,
99.6414616839008,100.638960339351,101.636458994802,102.633957650252,103.631456305703,
104.628954961153,105.626453616604,106.623952272054,107.621450927505,108.618949582955,
109.616448238406,110.613946893856,111.611445549307,112.608944204757,113.606442860208,
114.603941515658,115.601440171109,116.598938826559,117.59643748201,118.59393613746,
119.591434792911,120.588933448361,121.586432103812,122.583930759262,123.581429414713,
124.578928070163,125.576426725614,126.573925381064,127.571424036515,128.568922691965,
129.566421347416,130.563920002866),.UNSPECIFIED.);
#253=B_SPLINE_SURFACE_WITH_KNOTS('',3,3,((#40665,#40666,#40667,#40668,#40669,
#40670,#40671,#40672,#40673,#40674,#40675,#40676,#40677,#40678,#40679,#40680,
#40681,#40682,#40683,#40684,#40685,#40686,#40687,#40688,#40689,#40690,#40691,
#40692,#40693,#40694,#40695,#40696,#40697,#40698,#40699,#40700,#40701,#40702,
#40703,#40704,#40705,#40706,#40707,#40708,#40709,#40710,#40711,#40712,#40713,
#40714,#40715,#40716,#40717,#40718,#40719,#40720,#40721,#40722,#40723,#40724,
#40725,#40726,#40727,#40728,#40729,#40730,#40731,#40732,#40733,#40734,#40735,
#40736,#40737,#40738,#40739,#40740,#40741,#40742,#40743,#40744,#40745,#40746,
#40747,#40748,#40749,#40750,#40751,#40752,#40753,#40754,#40755,#40756,#40757,
#40758,#40759,#40760,#40761,#40762,#40763,#40764,#40765,#40766,#40767,#40768,
#40769,#40770,#40771,#40772,#40773,#40774,#40775,#40776,#40777,#40778,#40779,
#40780,#40781,#40782,#40783,#40784,#40785,#40786),(#40787,#40788,#40789,
#40790,#40791,#40792,#40793,#40794,#40795,#40796,#40797,#40798,#40799,#40800,
#40801,#40802,#40803,#40804,#40805,#40806,#40807,#40808,#40809,#40810,#40811,
#40812,#40813,#40814,#40815,#40816,#40817,#40818,#40819,#40820,#40821,#40822,
#40823,#40824,#40825,#40826,#40827,#40828,#40829,#40830,#40831,#40832,#40833,
#40834,#40835,#40836,#40837,#40838,#40839,#40840,#40841,#40842,#40843,#40844,
#40845,#40846,#40847,#40848,#40849,#40850,#40851,#40852,#40853,#40854,#40855,
#40856,#40857,#40858,#40859,#40860,#40861,#40862,#40863,#40864,#40865,#40866,
#40867,#40868,#40869,#40870,#40871,#40872,#40873,#40874,#40875,#40876,#40877,
#40878,#40879,#40880,#40881,#40882,#40883,#40884,#40885,#40886,#40887,#40888,
#40889,#40890,#40891,#40892,#40893,#40894,#40895,#40896,#40897,#40898,#40899,
#40900,#40901,#40902,#40903,#40904,#40905,#40906,#40907,#40908),(#40909,
#40910,#40911,#40912,#40913,#40914,#40915,#40916,#40917,#40918,#40919,#40920,
#40921,#40922,#40923,#40924,#40925,#40926,#40927,#40928,#40929,#40930,#40931,
#40932,#40933,#40934,#40935,#40936,#40937,#40938,#40939,#40940,#40941,#40942,
#40943,#40944,#40945,#40946,#40947,#40948,#40949,#40950,#40951,#40952,#40953,
#40954,#40955,#40956,#40957,#40958,#40959,#40960,#40961,#40962,#40963,#40964,
#40965,#40966,#40967,#40968,#40969,#40970,#40971,#40972,#40973,#40974,#40975,
#40976,#40977,#40978,#40979,#40980,#40981,#40982,#40983,#40984,#40985,#40986,
#40987,#40988,#40989,#40990,#40991,#40992,#40993,#40994,#40995,#40996,#40997,
#40998,#40999,#41000,#41001,#41002,#41003,#41004,#41005,#41006,#41007,#41008,
#41009,#41010,#41011,#41012,#41013,#41014,#41015,#41016,#41017,#41018,#41019,
#41020,#41021,#41022,#41023,#41024,#41025,#41026,#41027,#41028,#41029,#41030),
(#41031,#41032,#41033,#41034,#41035,#41036,#41037,#41038,#41039,#41040,
#41041,#41042,#41043,#41044,#41045,#41046,#41047,#41048,#41049,#41050,#41051,
#41052,#41053,#41054,#41055,#41056,#41057,#41058,#41059,#41060,#41061,#41062,
#41063,#41064,#41065,#41066,#41067,#41068,#41069,#41070,#41071,#41072,#41073,
#41074,#41075,#41076,#41077,#41078,#41079,#41080,#41081,#41082,#41083,#41084,
#41085,#41086,#41087,#41088,#41089,#41090,#41091,#41092,#41093,#41094,#41095,
#41096,#41097,#41098,#41099,#41100,#41101,#41102,#41103,#41104,#41105,#41106,
#41107,#41108,#41109,#41110,#41111,#41112,#41113,#41114,#41115,#41116,#41117,
#41118,#41119,#41120,#41121,#41122,#41123,#41124,#41125,#41126,#41127,#41128,
#41129,#41130,#41131,#41132,#41133,#41134,#41135,#41136,#41137,#41138,#41139,
#41140,#41141,#41142,#41143,#41144,#41145,#41146,#41147,#41148,#41149,#41150,
#41151,#41152)),.UNSPECIFIED.,.F.,.F.,.F.,(4,4),(4,1,1,1,1,1,1,1,1,1,1,
1,1,1,1,1,1,1,1,1,1,1,1,1,1,1,1,1,1,1,1,1,1,1,1,1,1,1,1,1,1,1,1,1,1,1,1,
1,1,1,1,1,1,1,1,1,1,1,1,1,1,1,1,1,1,1,1,1,1,1,1,1,1,1,1,1,1,1,1,1,1,1,1,
1,1,1,1,1,1,1,1,1,1,1,1,1,1,1,1,1,1,1,1,1,1,1,1,1,1,1,1,1,1,1,1,1,1,1,1,
4),(0.,0.0448889834294937),(14.3981410127769,15.3956396682274,16.3931383236779,
17.3906369791284,18.3881356345789,19.3856342900294,20.3831329454799,21.3806316009304,
22.3781302563809,23.3756289118314,24.3731275672819,25.3706262227324,26.3681248781829,
27.3656235336334,28.3631221890839,29.3606208445344,30.3581194999849,31.3556181554354,
32.3531168108859,33.3506154663364,34.3481141217869,35.3456127772374,36.3431114326879,
37.3406100881384,38.3381087435889,39.3356073990394,40.3331060544899,41.3306047099404,
42.3281033653909,43.3256020208414,44.3231006762919,45.3205993317424,46.3180979871929,
47.3155966426434,48.3130952980939,49.3105939535444,50.3080926089949,51.3055912644454,
52.3030899198959,53.3005885753464,54.2980872307969,55.2955858862474,56.2930845416979,
57.2905831971484,58.2880818525989,59.2855805080494,60.2830791634999,61.2805778189504,
62.2780764744009,63.2755751298514,64.2730737853019,65.2705724407524,66.2680710962029,
67.2655697516534,68.2630684071039,69.2605670625544,70.2580657180049,71.2555643734554,
72.2530630289059,73.2505616843565,74.248060339807,75.2455589952575,76.243057650708,
77.2405563061585,78.238054961609,79.2355536170595,80.23305227251,81.2305509279605,
82.228049583411,83.2255482388615,84.223046894312,85.2205455497625,86.218044205213,
87.2155428606635,88.213041516114,89.2105401715645,90.208038827015,91.2055374824655,
92.203036137916,93.2005347933665,94.198033448817,95.1955321042675,96.193030759718,
97.1905294151685,98.188028070619,99.1855267260695,100.18302538152,101.18052403697,
102.178022692421,103.175521347871,104.173020003322,105.170518658772,106.168017314223,
107.165515969673,108.163014625124,109.160513280574,110.158011936025,111.155510591476,
112.153009246926,113.150507902377,114.148006557827,115.145505213278,116.143003868728,
117.140502524179,118.138001179629,119.13549983508,120.13299849053,121.130497145981,
122.127995801431,123.125494456882,124.122993112332,125.120491767783,126.117990423233,
127.115489078684,128.112987734134,129.110486389585,130.107985045035,131.105483700486,
132.102982355936,133.100481011387),.UNSPECIFIED.);
#254=B_SPLINE_SURFACE_WITH_KNOTS('',3,3,((#41457,#41458,#41459,#41460,#41461,
#41462,#41463,#41464,#41465,#41466,#41467,#41468,#41469,#41470,#41471,#41472,
#41473,#41474,#41475,#41476,#41477,#41478,#41479,#41480,#41481,#41482,#41483,
#41484,#41485,#41486,#41487,#41488,#41489,#41490,#41491,#41492,#41493,#41494,
#41495,#41496,#41497,#41498,#41499,#41500,#41501,#41502,#41503,#41504,#41505,
#41506,#41507,#41508,#41509,#41510,#41511,#41512,#41513,#41514,#41515,#41516,
#41517,#41518,#41519,#41520,#41521,#41522,#41523,#41524,#41525,#41526,#41527,
#41528,#41529,#41530,#41531,#41532,#41533,#41534,#41535,#41536,#41537,#41538,
#41539,#41540,#41541,#41542,#41543,#41544,#41545,#41546,#41547,#41548,#41549,
#41550,#41551,#41552,#41553,#41554,#41555,#41556,#41557,#41558,#41559,#41560,
#41561,#41562,#41563,#41564,#41565,#41566,#41567,#41568,#41569,#41570,#41571,
#41572,#41573,#41574,#41575,#41576,#41577,#41578),(#41579,#41580,#41581,
#41582,#41583,#41584,#41585,#41586,#41587,#41588,#41589,#41590,#41591,#41592,
#41593,#41594,#41595,#41596,#41597,#41598,#41599,#41600,#41601,#41602,#41603,
#41604,#41605,#41606,#41607,#41608,#41609,#41610,#41611,#41612,#41613,#41614,
#41615,#41616,#41617,#41618,#41619,#41620,#41621,#41622,#41623,#41624,#41625,
#41626,#41627,#41628,#41629,#41630,#41631,#41632,#41633,#41634,#41635,#41636,
#41637,#41638,#41639,#41640,#41641,#41642,#41643,#41644,#41645,#41646,#41647,
#41648,#41649,#41650,#41651,#41652,#41653,#41654,#41655,#41656,#41657,#41658,
#41659,#41660,#41661,#41662,#41663,#41664,#41665,#41666,#41667,#41668,#41669,
#41670,#41671,#41672,#41673,#41674,#41675,#41676,#41677,#41678,#41679,#41680,
#41681,#41682,#41683,#41684,#41685,#41686,#41687,#41688,#41689,#41690,#41691,
#41692,#41693,#41694,#41695,#41696,#41697,#41698,#41699,#41700),(#41701,
#41702,#41703,#41704,#41705,#41706,#41707,#41708,#41709,#41710,#41711,#41712,
#41713,#41714,#41715,#41716,#41717,#41718,#41719,#41720,#41721,#41722,#41723,
#41724,#41725,#41726,#41727,#41728,#41729,#41730,#41731,#41732,#41733,#41734,
#41735,#41736,#41737,#41738,#41739,#41740,#41741,#41742,#41743,#41744,#41745,
#41746,#41747,#41748,#41749,#41750,#41751,#41752,#41753,#41754,#41755,#41756,
#41757,#41758,#41759,#41760,#41761,#41762,#41763,#41764,#41765,#41766,#41767,
#41768,#41769,#41770,#41771,#41772,#41773,#41774,#41775,#41776,#41777,#41778,
#41779,#41780,#41781,#41782,#41783,#41784,#41785,#41786,#41787,#41788,#41789,
#41790,#41791,#41792,#41793,#41794,#41795,#41796,#41797,#41798,#41799,#41800,
#41801,#41802,#41803,#41804,#41805,#41806,#41807,#41808,#41809,#41810,#41811,
#41812,#41813,#41814,#41815,#41816,#41817,#41818,#41819,#41820,#41821,#41822),
(#41823,#41824,#41825,#41826,#41827,#41828,#41829,#41830,#41831,#41832,
#41833,#41834,#41835,#41836,#41837,#41838,#41839,#41840,#41841,#41842,#41843,
#41844,#41845,#41846,#41847,#41848,#41849,#41850,#41851,#41852,#41853,#41854,
#41855,#41856,#41857,#41858,#41859,#41860,#41861,#41862,#41863,#41864,#41865,
#41866,#41867,#41868,#41869,#41870,#41871,#41872,#41873,#41874,#41875,#41876,
#41877,#41878,#41879,#41880,#41881,#41882,#41883,#41884,#41885,#41886,#41887,
#41888,#41889,#41890,#41891,#41892,#41893,#41894,#41895,#41896,#41897,#41898,
#41899,#41900,#41901,#41902,#41903,#41904,#41905,#41906,#41907,#41908,#41909,
#41910,#41911,#41912,#41913,#41914,#41915,#41916,#41917,#41918,#41919,#41920,
#41921,#41922,#41923,#41924,#41925,#41926,#41927,#41928,#41929,#41930,#41931,
#41932,#41933,#41934,#41935,#41936,#41937,#41938,#41939,#41940,#41941,#41942,
#41943,#41944)),.UNSPECIFIED.,.F.,.F.,.F.,(4,4),(4,1,1,1,1,1,1,1,1,1,1,
1,1,1,1,1,1,1,1,1,1,1,1,1,1,1,1,1,1,1,1,1,1,1,1,1,1,1,1,1,1,1,1,1,1,1,1,
1,1,1,1,1,1,1,1,1,1,1,1,1,1,1,1,1,1,1,1,1,1,1,1,1,1,1,1,1,1,1,1,1,1,1,1,
1,1,1,1,1,1,1,1,1,1,1,1,1,1,1,1,1,1,1,1,1,1,1,1,1,1,1,1,1,1,1,1,1,1,1,1,
4),(0.,0.0448889834294937),(11.8615800042567,12.8590786597072,13.8565773151577,
14.8540759706082,15.8515746260587,16.8490732815092,17.8465719369597,18.8440705924102,
19.8415692478607,20.8390679033112,21.8365665587617,22.8340652142122,23.8315638696627,
24.8290625251132,25.8265611805637,26.8240598360142,27.8215584914647,28.8190571469152,
29.8165558023657,30.8140544578162,31.8115531132667,32.8090517687172,33.8065504241677,
34.8040490796182,35.8015477350687,36.7990463905192,37.7965450459697,38.7940437014202,
39.7915423568707,40.7890410123212,41.7865396677717,42.7840383232222,43.7815369786727,
44.7790356341232,45.7765342895737,46.7740329450242,47.7715316004747,48.7690302559252,
49.7665289113757,50.7640275668262,51.7615262222767,52.7590248777272,53.7565235331777,
54.7540221886282,55.7515208440787,56.7490194995292,57.7465181549797,58.7440168104302,
59.7415154658807,60.7390141213312,61.7365127767817,62.7340114322322,63.7315100876827,
64.7290087431332,65.7265073985837,66.7240060540342,67.7215047094847,68.7190033649352,
69.7165020203857,70.7140006758362,71.7114993312867,72.7089979867372,73.7064966421877,
74.7039952976382,75.7014939530887,76.6989926085392,77.6964912639897,78.6939899194402,
79.6914885748908,80.6889872303413,81.6864858857918,82.6839845412423,83.6814831966928,
84.6789818521433,85.6764805075938,86.6739791630443,87.6714778184948,88.6689764739453,
89.6664751293958,90.6639737848463,91.6614724402968,92.6589710957473,93.6564697511978,
94.6539684066483,95.6514670620988,96.6489657175493,97.6464643729998,98.6439630284503,
99.6414616839008,100.638960339351,101.636458994802,102.633957650252,103.631456305703,
104.628954961153,105.626453616604,106.623952272054,107.621450927505,108.618949582955,
109.616448238406,110.613946893856,111.611445549307,112.608944204757,113.606442860208,
114.603941515658,115.601440171109,116.598938826559,117.59643748201,118.59393613746,
119.591434792911,120.588933448361,121.586432103812,122.583930759262,123.581429414713,
124.578928070163,125.576426725614,126.573925381064,127.571424036515,128.568922691965,
129.566421347416,130.563920002866),.UNSPECIFIED.);
#255=B_SPLINE_SURFACE_WITH_KNOTS('',3,3,((#42052,#42053,#42054,#42055,#42056,
#42057,#42058,#42059,#42060,#42061,#42062,#42063,#42064,#42065,#42066,#42067,
#42068,#42069,#42070,#42071,#42072,#42073,#42074,#42075,#42076,#42077,#42078,
#42079,#42080,#42081,#42082,#42083,#42084,#42085,#42086,#42087,#42088,#42089,
#42090,#42091,#42092,#42093,#42094,#42095,#42096,#42097,#42098,#42099,#42100,
#42101,#42102,#42103,#42104,#42105,#42106,#42107,#42108,#42109,#42110,#42111,
#42112,#42113,#42114,#42115,#42116,#42117,#42118,#42119,#42120,#42121,#42122,
#42123,#42124,#42125,#42126,#42127,#42128,#42129,#42130,#42131,#42132,#42133,
#42134,#42135,#42136,#42137,#42138,#42139,#42140,#42141,#42142,#42143,#42144,
#42145,#42146,#42147,#42148,#42149,#42150,#42151,#42152,#42153,#42154,#42155,
#42156,#42157,#42158,#42159,#42160,#42161,#42162,#42163,#42164,#42165,#42166,
#42167,#42168,#42169,#42170,#42171,#42172,#42173),(#42174,#42175,#42176,
#42177,#42178,#42179,#42180,#42181,#42182,#42183,#42184,#42185,#42186,#42187,
#42188,#42189,#42190,#42191,#42192,#42193,#42194,#42195,#42196,#42197,#42198,
#42199,#42200,#42201,#42202,#42203,#42204,#42205,#42206,#42207,#42208,#42209,
#42210,#42211,#42212,#42213,#42214,#42215,#42216,#42217,#42218,#42219,#42220,
#42221,#42222,#42223,#42224,#42225,#42226,#42227,#42228,#42229,#42230,#42231,
#42232,#42233,#42234,#42235,#42236,#42237,#42238,#42239,#42240,#42241,#42242,
#42243,#42244,#42245,#42246,#42247,#42248,#42249,#42250,#42251,#42252,#42253,
#42254,#42255,#42256,#42257,#42258,#42259,#42260,#42261,#42262,#42263,#42264,
#42265,#42266,#42267,#42268,#42269,#42270,#42271,#42272,#42273,#42274,#42275,
#42276,#42277,#42278,#42279,#42280,#42281,#42282,#42283,#42284,#42285,#42286,
#42287,#42288,#42289,#42290,#42291,#42292,#42293,#42294,#42295),(#42296,
#42297,#42298,#42299,#42300,#42301,#42302,#42303,#42304,#42305,#42306,#42307,
#42308,#42309,#42310,#42311,#42312,#42313,#42314,#42315,#42316,#42317,#42318,
#42319,#42320,#42321,#42322,#42323,#42324,#42325,#42326,#42327,#42328,#42329,
#42330,#42331,#42332,#42333,#42334,#42335,#42336,#42337,#42338,#42339,#42340,
#42341,#42342,#42343,#42344,#42345,#42346,#42347,#42348,#42349,#42350,#42351,
#42352,#42353,#42354,#42355,#42356,#42357,#42358,#42359,#42360,#42361,#42362,
#42363,#42364,#42365,#42366,#42367,#42368,#42369,#42370,#42371,#42372,#42373,
#42374,#42375,#42376,#42377,#42378,#42379,#42380,#42381,#42382,#42383,#42384,
#42385,#42386,#42387,#42388,#42389,#42390,#42391,#42392,#42393,#42394,#42395,
#42396,#42397,#42398,#42399,#42400,#42401,#42402,#42403,#42404,#42405,#42406,
#42407,#42408,#42409,#42410,#42411,#42412,#42413,#42414,#42415,#42416,#42417),
(#42418,#42419,#42420,#42421,#42422,#42423,#42424,#42425,#42426,#42427,
#42428,#42429,#42430,#42431,#42432,#42433,#42434,#42435,#42436,#42437,#42438,
#42439,#42440,#42441,#42442,#42443,#42444,#42445,#42446,#42447,#42448,#42449,
#42450,#42451,#42452,#42453,#42454,#42455,#42456,#42457,#42458,#42459,#42460,
#42461,#42462,#42463,#42464,#42465,#42466,#42467,#42468,#42469,#42470,#42471,
#42472,#42473,#42474,#42475,#42476,#42477,#42478,#42479,#42480,#42481,#42482,
#42483,#42484,#42485,#42486,#42487,#42488,#42489,#42490,#42491,#42492,#42493,
#42494,#42495,#42496,#42497,#42498,#42499,#42500,#42501,#42502,#42503,#42504,
#42505,#42506,#42507,#42508,#42509,#42510,#42511,#42512,#42513,#42514,#42515,
#42516,#42517,#42518,#42519,#42520,#42521,#42522,#42523,#42524,#42525,#42526,
#42527,#42528,#42529,#42530,#42531,#42532,#42533,#42534,#42535,#42536,#42537,
#42538,#42539)),.UNSPECIFIED.,.F.,.F.,.F.,(4,4),(4,1,1,1,1,1,1,1,1,1,1,
1,1,1,1,1,1,1,1,1,1,1,1,1,1,1,1,1,1,1,1,1,1,1,1,1,1,1,1,1,1,1,1,1,1,1,1,
1,1,1,1,1,1,1,1,1,1,1,1,1,1,1,1,1,1,1,1,1,1,1,1,1,1,1,1,1,1,1,1,1,1,1,1,
1,1,1,1,1,1,1,1,1,1,1,1,1,1,1,1,1,1,1,1,1,1,1,1,1,1,1,1,1,1,1,1,1,1,1,1,
4),(0.,0.0448889834294937),(14.3981410127769,15.3956396682274,16.3931383236779,
17.3906369791284,18.3881356345789,19.3856342900294,20.3831329454799,21.3806316009304,
22.3781302563809,23.3756289118314,24.3731275672819,25.3706262227324,26.3681248781829,
27.3656235336334,28.3631221890839,29.3606208445344,30.3581194999849,31.3556181554354,
32.3531168108859,33.3506154663364,34.3481141217869,35.3456127772374,36.3431114326879,
37.3406100881384,38.3381087435889,39.3356073990394,40.3331060544899,41.3306047099404,
42.3281033653909,43.3256020208414,44.3231006762919,45.3205993317424,46.3180979871929,
47.3155966426434,48.3130952980939,49.3105939535444,50.3080926089949,51.3055912644454,
52.3030899198959,53.3005885753464,54.2980872307969,55.2955858862474,56.2930845416979,
57.2905831971484,58.2880818525989,59.2855805080494,60.2830791634999,61.2805778189504,
62.2780764744009,63.2755751298514,64.2730737853019,65.2705724407524,66.2680710962029,
67.2655697516534,68.2630684071039,69.2605670625544,70.2580657180049,71.2555643734554,
72.2530630289059,73.2505616843565,74.248060339807,75.2455589952575,76.243057650708,
77.2405563061585,78.238054961609,79.2355536170595,80.23305227251,81.2305509279605,
82.228049583411,83.2255482388615,84.223046894312,85.2205455497625,86.218044205213,
87.2155428606635,88.213041516114,89.2105401715645,90.208038827015,91.2055374824655,
92.203036137916,93.2005347933665,94.198033448817,95.1955321042675,96.193030759718,
97.1905294151685,98.188028070619,99.1855267260695,100.18302538152,101.18052403697,
102.178022692421,103.175521347871,104.173020003322,105.170518658772,106.168017314223,
107.165515969673,108.163014625124,109.160513280574,110.158011936025,111.155510591476,
112.153009246926,113.150507902377,114.148006557827,115.145505213278,116.143003868728,
117.140502524179,118.138001179629,119.13549983508,120.13299849053,121.130497145981,
122.127995801431,123.125494456882,124.122993112332,125.120491767783,126.117990423233,
127.115489078684,128.112987734134,129.110486389585,130.107985045035,131.105483700486,
132.102982355936,133.100481011387),.UNSPECIFIED.);
#256=B_SPLINE_SURFACE_WITH_KNOTS('',3,3,((#42712,#42713,#42714,#42715,#42716,
#42717,#42718,#42719,#42720,#42721,#42722,#42723,#42724,#42725,#42726,#42727,
#42728,#42729,#42730,#42731,#42732,#42733,#42734,#42735,#42736,#42737,#42738,
#42739,#42740,#42741,#42742,#42743,#42744,#42745,#42746,#42747,#42748,#42749,
#42750,#42751,#42752,#42753,#42754,#42755,#42756,#42757,#42758,#42759,#42760,
#42761,#42762,#42763,#42764,#42765,#42766,#42767,#42768,#42769,#42770,#42771,
#42772,#42773,#42774,#42775,#42776,#42777,#42778,#42779,#42780,#42781,#42782,
#42783,#42784,#42785,#42786,#42787,#42788,#42789,#42790,#42791,#42792,#42793,
#42794,#42795,#42796,#42797,#42798,#42799,#42800,#42801,#42802,#42803,#42804,
#42805,#42806),(#42807,#42808,#42809,#42810,#42811,#42812,#42813,#42814,
#42815,#42816,#42817,#42818,#42819,#42820,#42821,#42822,#42823,#42824,#42825,
#42826,#42827,#42828,#42829,#42830,#42831,#42832,#42833,#42834,#42835,#42836,
#42837,#42838,#42839,#42840,#42841,#42842,#42843,#42844,#42845,#42846,#42847,
#42848,#42849,#42850,#42851,#42852,#42853,#42854,#42855,#42856,#42857,#42858,
#42859,#42860,#42861,#42862,#42863,#42864,#42865,#42866,#42867,#42868,#42869,
#42870,#42871,#42872,#42873,#42874,#42875,#42876,#42877,#42878,#42879,#42880,
#42881,#42882,#42883,#42884,#42885,#42886,#42887,#42888,#42889,#42890,#42891,
#42892,#42893,#42894,#42895,#42896,#42897,#42898,#42899,#42900,#42901),
(#42902,#42903,#42904,#42905,#42906,#42907,#42908,#42909,#42910,#42911,
#42912,#42913,#42914,#42915,#42916,#42917,#42918,#42919,#42920,#42921,#42922,
#42923,#42924,#42925,#42926,#42927,#42928,#42929,#42930,#42931,#42932,#42933,
#42934,#42935,#42936,#42937,#42938,#42939,#42940,#42941,#42942,#42943,#42944,
#42945,#42946,#42947,#42948,#42949,#42950,#42951,#42952,#42953,#42954,#42955,
#42956,#42957,#42958,#42959,#42960,#42961,#42962,#42963,#42964,#42965,#42966,
#42967,#42968,#42969,#42970,#42971,#42972,#42973,#42974,#42975,#42976,#42977,
#42978,#42979,#42980,#42981,#42982,#42983,#42984,#42985,#42986,#42987,#42988,
#42989,#42990,#42991,#42992,#42993,#42994,#42995,#42996),(#42997,#42998,
#42999,#43000,#43001,#43002,#43003,#43004,#43005,#43006,#43007,#43008,#43009,
#43010,#43011,#43012,#43013,#43014,#43015,#43016,#43017,#43018,#43019,#43020,
#43021,#43022,#43023,#43024,#43025,#43026,#43027,#43028,#43029,#43030,#43031,
#43032,#43033,#43034,#43035,#43036,#43037,#43038,#43039,#43040,#43041,#43042,
#43043,#43044,#43045,#43046,#43047,#43048,#43049,#43050,#43051,#43052,#43053,
#43054,#43055,#43056,#43057,#43058,#43059,#43060,#43061,#43062,#43063,#43064,
#43065,#43066,#43067,#43068,#43069,#43070,#43071,#43072,#43073,#43074,#43075,
#43076,#43077,#43078,#43079,#43080,#43081,#43082,#43083,#43084,#43085,#43086,
#43087,#43088,#43089,#43090,#43091)),.UNSPECIFIED.,.F.,.F.,.F.,(4,4),(4,
1,1,1,1,1,1,1,1,1,1,1,1,1,1,1,1,1,1,1,1,1,1,1,1,1,1,1,1,1,1,1,1,1,1,1,1,
1,1,1,1,1,1,1,1,1,1,1,1,1,1,1,1,1,1,1,1,1,1,1,1,1,1,1,1,1,1,1,1,1,1,1,1,
1,1,1,1,1,1,1,1,1,1,1,1,1,1,1,1,1,1,1,4),(0.,0.112756507572734),(11.8517336648509,
12.3420477881087,12.8323619113665,13.3226760346243,13.812990157882,14.3033042811398,
14.7936184043976,15.2839325276554,15.7742466509132,16.264560774171,16.7548748974288,
17.2451890206866,17.7355031439444,18.2258172672022,18.71613139046,19.2064455137178,
19.6967596369755,20.1870737602333,20.6773878834911,21.1677020067489,21.6580161300067,
22.1483302532645,22.6386443765223,23.1289584997801,23.6192726230379,24.1095867462957,
24.5999008695535,25.0902149928113,25.5805291160691,26.0708432393268,26.5611573625846,
27.0514714858424,27.5417856091002,28.032099732358,28.5224138556158,29.0127279788736,
29.5030421021314,29.9933562253892,30.483670348647,30.9739844719048,31.4642985951626,
31.9546127184203,32.4449268416781,32.9352409649359,33.4255550881937,33.9158692114515,
34.4061833347093,34.8964974579671,35.3868115812249,35.8771257044827,36.3674398277405,
36.8577539509983,37.3480680742561,37.8383821975139,38.3286963207716,38.8190104440294,
39.3093245672872,39.799638690545,40.2899528138028,40.7802669370606,41.2705810603184,
41.7608951835762,42.251209306834,42.7415234300918,43.2318375533496,43.7221516766074,
44.2124657998651,44.7027799231229,45.1930940463807,45.6834081696385,46.1737222928963,
46.6640364161541,47.1543505394119,47.6446646626697,48.1349787859275,48.6252929091853,
49.1156070324431,49.6059211557009,50.0962352789586,50.5865494022164,51.0768635254742,
51.567177648732,52.0574917719898,52.5478058952476,53.0381200185054,53.5284341417632,
54.018748265021,54.5090623882788,54.9993765115366,55.4896906347944,55.9800047580521,
56.4703188813099,56.9606330045677),.UNSPECIFIED.);
#257=B_SPLINE_SURFACE_WITH_KNOTS('',3,3,((#43365,#43366,#43367,#43368,#43369,
#43370,#43371,#43372,#43373,#43374,#43375,#43376,#43377,#43378,#43379,#43380,
#43381,#43382,#43383,#43384,#43385,#43386,#43387,#43388,#43389,#43390,#43391,
#43392,#43393,#43394,#43395,#43396,#43397,#43398,#43399,#43400,#43401,#43402,
#43403,#43404,#43405,#43406,#43407,#43408,#43409,#43410,#43411,#43412,#43413,
#43414,#43415,#43416,#43417,#43418,#43419,#43420,#43421,#43422,#43423,#43424,
#43425,#43426,#43427,#43428,#43429,#43430,#43431,#43432,#43433,#43434,#43435,
#43436,#43437,#43438,#43439,#43440,#43441,#43442,#43443,#43444,#43445,#43446,
#43447,#43448,#43449,#43450,#43451,#43452,#43453,#43454,#43455,#43456,#43457,
#43458,#43459),(#43460,#43461,#43462,#43463,#43464,#43465,#43466,#43467,
#43468,#43469,#43470,#43471,#43472,#43473,#43474,#43475,#43476,#43477,#43478,
#43479,#43480,#43481,#43482,#43483,#43484,#43485,#43486,#43487,#43488,#43489,
#43490,#43491,#43492,#43493,#43494,#43495,#43496,#43497,#43498,#43499,#43500,
#43501,#43502,#43503,#43504,#43505,#43506,#43507,#43508,#43509,#43510,#43511,
#43512,#43513,#43514,#43515,#43516,#43517,#43518,#43519,#43520,#43521,#43522,
#43523,#43524,#43525,#43526,#43527,#43528,#43529,#43530,#43531,#43532,#43533,
#43534,#43535,#43536,#43537,#43538,#43539,#43540,#43541,#43542,#43543,#43544,
#43545,#43546,#43547,#43548,#43549,#43550,#43551,#43552,#43553,#43554),
(#43555,#43556,#43557,#43558,#43559,#43560,#43561,#43562,#43563,#43564,
#43565,#43566,#43567,#43568,#43569,#43570,#43571,#43572,#43573,#43574,#43575,
#43576,#43577,#43578,#43579,#43580,#43581,#43582,#43583,#43584,#43585,#43586,
#43587,#43588,#43589,#43590,#43591,#43592,#43593,#43594,#43595,#43596,#43597,
#43598,#43599,#43600,#43601,#43602,#43603,#43604,#43605,#43606,#43607,#43608,
#43609,#43610,#43611,#43612,#43613,#43614,#43615,#43616,#43617,#43618,#43619,
#43620,#43621,#43622,#43623,#43624,#43625,#43626,#43627,#43628,#43629,#43630,
#43631,#43632,#43633,#43634,#43635,#43636,#43637,#43638,#43639,#43640,#43641,
#43642,#43643,#43644,#43645,#43646,#43647,#43648,#43649),(#43650,#43651,
#43652,#43653,#43654,#43655,#43656,#43657,#43658,#43659,#43660,#43661,#43662,
#43663,#43664,#43665,#43666,#43667,#43668,#43669,#43670,#43671,#43672,#43673,
#43674,#43675,#43676,#43677,#43678,#43679,#43680,#43681,#43682,#43683,#43684,
#43685,#43686,#43687,#43688,#43689,#43690,#43691,#43692,#43693,#43694,#43695,
#43696,#43697,#43698,#43699,#43700,#43701,#43702,#43703,#43704,#43705,#43706,
#43707,#43708,#43709,#43710,#43711,#43712,#43713,#43714,#43715,#43716,#43717,
#43718,#43719,#43720,#43721,#43722,#43723,#43724,#43725,#43726,#43727,#43728,
#43729,#43730,#43731,#43732,#43733,#43734,#43735,#43736,#43737,#43738,#43739,
#43740,#43741,#43742,#43743,#43744)),.UNSPECIFIED.,.F.,.F.,.F.,(4,4),(4,
1,1,1,1,1,1,1,1,1,1,1,1,1,1,1,1,1,1,1,1,1,1,1,1,1,1,1,1,1,1,1,1,1,1,1,1,
1,1,1,1,1,1,1,1,1,1,1,1,1,1,1,1,1,1,1,1,1,1,1,1,1,1,1,1,1,1,1,1,1,1,1,1,
1,1,1,1,1,1,1,1,1,1,1,1,1,1,1,1,1,1,1,4),(0.,0.112756507572734),(14.3984001269719,
14.8887142502297,15.3790283734874,15.8693424967452,16.359656620003,16.8499707432608,
17.3402848665186,17.8305989897764,18.3209131130342,18.811227236292,19.3015413595498,
19.7918554828076,20.2821696060654,20.7724837293232,21.2627978525809,21.7531119758387,
22.2434260990965,22.7337402223543,23.2240543456121,23.7143684688699,24.2046825921277,
24.6949967153855,25.1853108386433,25.6756249619011,26.1659390851589,26.6562532084167,
27.1465673316744,27.6368814549322,28.12719557819,28.6175097014478,29.1078238247056,
29.5981379479634,30.0884520712212,30.578766194479,31.0690803177368,31.5593944409946,
32.0497085642524,32.5400226875101,33.0303368107679,33.5206509340257,34.0109650572835,
34.5012791805413,34.9915933037991,35.4819074270569,35.9722215503147,36.4625356735725,
36.9528497968303,37.4431639200881,37.9334780433459,38.4237921666036,38.9141062898614,
39.4044204131192,39.894734536377,40.3850486596348,40.8753627828926,41.3656769061504,
41.8559910294082,42.346305152666,42.8366192759238,43.3269333991816,43.8172475224394,
44.3075616456971,44.7978757689549,45.2881898922127,45.7785040154705,46.2688181387283,
46.7591322619861,47.2494463852439,47.7397605085017,48.2300746317595,48.7203887550173,
49.2107028782751,49.7010170015329,50.1913311247907,50.6816452480484,51.1719593713062,
51.662273494564,52.1525876178218,52.6429017410796,53.1332158643374,53.6235299875952,
54.113844110853,54.6041582341108,55.0944723573686,55.5847864806264,56.0751006038842,
56.5654147271419,57.0557288503997,57.5460429736575,58.0363570969153,58.5266712201731,
59.0169853434309,59.5072994666887),.UNSPECIFIED.);
#266=B_SPLINE_CURVE_WITH_KNOTS('',3,(#20089,#20090,#20091,#20092,#20093,
#20094,#20095,#20096,#20097,#20098,#20099,#20100,#20101),.UNSPECIFIED.,
 .F.,.F.,(4,3,3,3,4),(-43.0846992492315,-42.6573287234279,-42.1670146001701,
-41.6767004769123,-41.5553414461756),.UNSPECIFIED.);
#267=B_SPLINE_CURVE_WITH_KNOTS('',3,(#20107,#20108,#20109,#20110,#20111,
#20112,#20113,#20114,#20115,#20116,#20117,#20118,#20119,#20120,#20121,#20122,
#20123,#20124,#20125,#20126,#20127,#20128,#20129,#20130,#20131,#20132,#20133,
#20134,#20135,#20136,#20137,#20138,#20139,#20140,#20141,#20142,#20143,#20144,
#20145,#20146),.UNSPECIFIED.,.F.,.F.,(4,3,3,3,3,3,3,3,3,3,3,3,3,4),(39.0086749840546,
39.2251298606233,39.7154439838811,40.2057581071389,40.6960722303967,41.1863863536545,
41.6767004769123,42.1670146001701,42.6573287234279,43.1476428466857,43.6379569699435,
44.1282710932012,44.618585216459,45.1088993397168),.UNSPECIFIED.);
#268=B_SPLINE_CURVE_WITH_KNOTS('',3,(#20148,#20149,#20150,#20151,#20152,
#20153,#20154,#20155,#20156,#20157,#20158,#20159,#20160,#20161,#20162,#20163,
#20164,#20165,#20166,#20167,#20168,#20169,#20170,#20171,#20172,#20173,#20174,
#20175,#20176,#20177,#20178,#20179,#20180,#20181,#20182,#20183,#20184,#20185,
#20186,#20187,#20188,#20189,#20190),.UNSPECIFIED.,.F.,.F.,(4,3,3,3,3,3,
3,3,3,3,3,3,3,3,4),(-41.5553414461756,-41.1863863536545,-40.6960722303967,
-40.2057581071389,-39.7154439838811,-39.2251298606233,-38.7348157373656,
-38.2445016141078,-37.75418749085,-37.2638733675922,-36.7735592443344,-36.2832451210766,
-35.7929309978188,-35.302616874561,-35.272156138996),.UNSPECIFIED.);
#269=B_SPLINE_CURVE_WITH_KNOTS('',3,(#20195,#20196,#20197,#20198,#20199,
#20200,#20201,#20202,#20203,#20204,#20205,#20206,#20207,#20208,#20209,#20210,
#20211,#20212,#20213,#20214,#20215,#20216,#20217,#20218,#20219,#20220,#20221,
#20222,#20223,#20224,#20225,#20226,#20227,#20228,#20229,#20230,#20231,#20232,
#20233,#20234,#20235,#20236,#20237),.UNSPECIFIED.,.F.,.F.,(4,3,3,3,3,3,
3,3,3,3,3,3,3,3,4),(32.725489676875,32.851046258272,33.3413603815298,33.8316745047876,
34.3219886280454,34.8123027513032,35.302616874561,35.7929309978188,36.2832451210766,
36.7735592443344,37.2638733675922,37.75418749085,38.2445016141078,38.7348157373655,
39.0086749840546),.UNSPECIFIED.);
#270=B_SPLINE_CURVE_WITH_KNOTS('',3,(#20238,#20239,#20240,#20241,#20242,
#20243,#20244,#20245,#20246,#20247,#20248,#20249,#20250,#20251,#20252,#20253,
#20254,#20255,#20256,#20257,#20258,#20259,#20260,#20261,#20262,#20263,#20264,
#20265,#20266,#20267,#20268,#20269,#20270,#20271,#20272,#20273,#20274,#20275,
#20276,#20277),.UNSPECIFIED.,.F.,.F.,(4,3,3,3,3,3,3,3,3,3,3,3,3,4),(-35.272156138996,
-34.8123027513032,-34.3219886280454,-33.8316745047876,-33.3413603815298,
-32.851046258272,-32.3607321350143,-31.8704180117565,-31.3801038884987,
-30.8897897652409,-30.3994756419831,-29.9091615187253,-29.4188473954675,
-28.9889708318164),.UNSPECIFIED.);
#271=B_SPLINE_CURVE_WITH_KNOTS('',3,(#20282,#20283,#20284,#20285,#20286,
#20287,#20288,#20289,#20290,#20291,#20292,#20293,#20294,#20295,#20296,#20297,
#20298,#20299,#20300,#20301,#20302,#20303,#20304,#20305,#20306,#20307,#20308,
#20309,#20310,#20311,#20312,#20313,#20314,#20315,#20316,#20317,#20318,#20319,
#20320,#20321,#20322,#20323,#20324),.UNSPECIFIED.,.F.,.F.,(4,3,3,3,3,3,
3,3,3,3,3,3,3,3,4),(26.4423043696954,26.4769626559207,26.9672767791785,
27.4575909024363,27.9479050256941,28.4382191489519,28.9285332722097,29.4188473954675,
29.9091615187253,30.3994756419831,30.8897897652409,31.3801038884987,31.8704180117565,
32.3607321350143,32.725489676875),.UNSPECIFIED.);
#272=B_SPLINE_CURVE_WITH_KNOTS('',3,(#20325,#20326,#20327,#20328,#20329,
#20330,#20331,#20332,#20333,#20334,#20335,#20336,#20337,#20338,#20339,#20340,
#20341,#20342,#20343,#20344,#20345,#20346,#20347,#20348,#20349,#20350,#20351,
#20352,#20353,#20354,#20355,#20356,#20357,#20358,#20359,#20360,#20361,#20362,
#20363,#20364,#20365,#20366,#20367),.UNSPECIFIED.,.F.,.F.,(4,3,3,3,3,3,
3,3,3,3,3,3,3,3,4),(-28.9889708318164,-28.9285332722097,-28.4382191489519,
-27.9479050256941,-27.4575909024363,-26.9672767791785,-26.4769626559208,
-25.986648532663,-25.4963344094052,-25.0060202861474,-24.5157061628896,
-24.0253920396318,-23.535077916374,-23.0447637931162,-22.7057855246369),
 .UNSPECIFIED.);
#273=B_SPLINE_CURVE_WITH_KNOTS('',3,(#20372,#20373,#20374,#20375,#20376,
#20377,#20378,#20379,#20380,#20381,#20382,#20383,#20384,#20385,#20386,#20387,
#20388,#20389,#20390,#20391,#20392,#20393,#20394,#20395,#20396,#20397,#20398,
#20399,#20400,#20401,#20402,#20403,#20404,#20405,#20406,#20407,#20408,#20409,
#20410,#20411),.UNSPECIFIED.,.F.,.F.,(4,3,3,3,3,3,3,3,3,3,3,3,3,4),(20.1591190625159,
20.5931931768272,21.083507300085,21.5738214233428,22.0641355466006,22.5544496698584,
23.0447637931162,23.535077916374,24.0253920396318,24.5157061628896,25.0060202861474,
25.4963344094052,25.986648532663,26.4423043696954),.UNSPECIFIED.);
#274=B_SPLINE_CURVE_WITH_KNOTS('',3,(#20412,#20413,#20414,#20415,#20416,
#20417,#20418,#20419,#20420,#20421,#20422,#20423,#20424,#20425,#20426,#20427,
#20428,#20429,#20430,#20431,#20432,#20433,#20434,#20435,#20436,#20437,#20438,
#20439,#20440,#20441,#20442,#20443,#20444,#20445,#20446,#20447,#20448,#20449,
#20450,#20451,#20452,#20453,#20454),.UNSPECIFIED.,.F.,.F.,(4,3,3,3,3,3,
3,3,3,3,3,3,3,3,4),(-22.7057855246369,-22.5544496698584,-22.0641355466006,
-21.5738214233428,-21.083507300085,-20.5931931768273,-20.1028790535695,
-19.6125649303117,-19.1222508070539,-18.6319366837961,-18.1416225605383,
-17.6513084372805,-17.1609943140227,-16.6706801907649,-16.4226002174572),
 .UNSPECIFIED.);
#275=B_SPLINE_CURVE_WITH_KNOTS('',3,(#20459,#20460,#20461,#20462,#20463,
#20464,#20465,#20466,#20467,#20468,#20469,#20470,#20471,#20472,#20473,#20474,
#20475,#20476,#20477,#20478,#20479,#20480,#20481,#20482,#20483,#20484,#20485,
#20486,#20487,#20488,#20489,#20490,#20491,#20492,#20493,#20494,#20495,#20496,
#20497,#20498,#20499,#20500,#20501),.UNSPECIFIED.,.F.,.F.,(4,3,3,3,3,3,
3,3,3,3,3,3,3,3,4),(13.8759337553363,14.219109574476,14.7094236977338,15.1997378209915,
15.6900519442493,16.1803660675071,16.6706801907649,17.1609943140227,17.6513084372805,
18.1416225605383,18.6319366837961,19.1222508070539,19.6125649303117,20.1028790535695,
20.1591190625159),.UNSPECIFIED.);
#276=B_SPLINE_CURVE_WITH_KNOTS('',3,(#20502,#20503,#20504,#20505,#20506,
#20507,#20508,#20509,#20510,#20511,#20512,#20513,#20514,#20515,#20516,#20517,
#20518,#20519,#20520,#20521,#20522,#20523,#20524,#20525,#20526,#20527,#20528,
#20529,#20530,#20531,#20532,#20533,#20534,#20535,#20536,#20537,#20538,#20539,
#20540,#20541,#20542,#20543,#20544),.UNSPECIFIED.,.F.,.F.,(4,3,3,3,3,3,
3,3,3,3,3,3,3,3,4),(-16.4226002174572,-16.1803660675071,-15.6900519442493,
-15.1997378209915,-14.7094236977338,-14.219109574476,-13.7287954512182,
-13.2384813279604,-12.7481672047026,-12.2578530814448,-11.767538958187,
-11.2772248349292,-10.7869107116714,-10.2965965884136,-10.1394149102777),
 .UNSPECIFIED.);
#277=B_SPLINE_CURVE_WITH_KNOTS('',3,(#20550,#20551,#20552,#20553,#20554,
#20555,#20556,#20557,#20558,#20559,#20560,#20561,#20562,#20563,#20564,#20565,
#20566,#20567,#20568,#20569,#20570,#20571,#20572,#20573,#20574),
 .UNSPECIFIED.,.F.,.F.,(4,3,3,3,3,3,3,3,4),(-3.85622960309808,-3.43219886280454,
-2.94188473954675,-2.45157061628896,-1.96125649303117,-1.47094236977338,
-0.980628246515584,-0.490314123257793,0.),.UNSPECIFIED.);
#278=B_SPLINE_CURVE_WITH_KNOTS('',3,(#20577,#20578,#20579,#20580,#20581,
#20582,#20583,#20584,#20585,#20586,#20587,#20588,#20589,#20590,#20591,#20592,
#20593,#20594,#20595,#20596,#20597,#20598,#20599,#20600,#20601,#20602,#20603,
#20604,#20605,#20606,#20607,#20608,#20609,#20610,#20611,#20612,#20613),
 .UNSPECIFIED.,.F.,.F.,(4,3,3,3,3,3,3,3,3,3,3,3,4),(2.02420009048538,2.45157061628896,
2.94188473954675,3.43219886280454,3.92251298606233,4.41282710932012,4.90314123257792,
5.39345535583571,5.8837694790935,6.37408360235129,6.86439772560908,7.35471184886687,
7.59274844815668),.UNSPECIFIED.);
#279=B_SPLINE_CURVE_WITH_KNOTS('',3,(#20619,#20620,#20621,#20622,#20623,
#20624,#20625,#20626,#20627,#20628,#20629),.UNSPECIFIED.,.F.,.F.,(4,1,1,
1,1,1,1,1,4),(53.4070751110265,53.5284341417632,54.018748265021,54.5090623882788,
54.9993765115366,55.4896906347944,55.9800047580521,56.4703188813099,56.9606330045677),
 .UNSPECIFIED.);
#280=B_SPLINE_CURVE_WITH_KNOTS('',3,(#20632,#20633,#20634,#20635,#20636,
#20637,#20638,#20639,#20640,#20641,#20642,#20643),.UNSPECIFIED.,.F.,.F.,
(4,1,1,1,1,1,1,1,1,4),(53.4070751110265,53.6235299875952,54.113844110853,
54.6041582341108,55.0944723573686,55.5847864806264,56.0751006038842,56.5654147271419,
57.0557288503997,57.4830993762033),.UNSPECIFIED.);
#281=B_SPLINE_CURVE_WITH_KNOTS('',3,(#20648,#20649,#20650,#20651,#20652,
#20653,#20654,#20655,#20656,#20657,#20658,#20659,#20660,#20661,#20662,#20663,
#20664),.UNSPECIFIED.,.F.,.F.,(4,1,1,1,1,1,1,1,1,1,1,1,1,1,4),(47.1238898038469,
47.1543505394119,47.6446646626697,48.1349787859275,48.6252929091853,49.1156070324431,
49.6059211557009,50.0962352789586,50.5865494022164,51.0768635254742,51.567177648732,
52.0574917719898,52.5478058952476,53.0381200185054,53.4070751110265),
 .UNSPECIFIED.);
#282=B_SPLINE_CURVE_WITH_KNOTS('',3,(#20665,#20666,#20667,#20668,#20669,
#20670,#20671,#20672,#20673,#20674,#20675,#20676,#20677,#20678,#20679,#20680,
#20681),.UNSPECIFIED.,.F.,.F.,(4,1,1,1,1,1,1,1,1,1,1,1,1,1,4),(47.1238898038469,
47.2494463852439,47.7397605085017,48.2300746317595,48.7203887550173,49.2107028782751,
49.7010170015329,50.1913311247907,50.6816452480484,51.1719593713062,51.662273494564,
52.1525876178218,52.6429017410796,53.1332158643374,53.4070751110265),
 .UNSPECIFIED.);
#283=B_SPLINE_CURVE_WITH_KNOTS('',3,(#20686,#20687,#20688,#20689,#20690,
#20691,#20692,#20693,#20694,#20695,#20696,#20697,#20698,#20699,#20700,#20701),
 .UNSPECIFIED.,.F.,.F.,(4,1,1,1,1,1,1,1,1,1,1,1,1,4),(40.8407044966673,
41.2705810603184,41.7608951835762,42.251209306834,42.7415234300918,43.2318375533496,
43.7221516766074,44.2124657998651,44.7027799231229,45.1930940463807,45.6834081696385,
46.1737222928963,46.6640364161541,47.1238898038469),.UNSPECIFIED.);
#284=B_SPLINE_CURVE_WITH_KNOTS('',3,(#20702,#20703,#20704,#20705,#20706,
#20707,#20708,#20709,#20710,#20711,#20712,#20713,#20714,#20715,#20716,#20717,
#20718),.UNSPECIFIED.,.F.,.F.,(4,1,1,1,1,1,1,1,1,1,1,1,1,1,4),(40.8407044966673,
40.8753627828926,41.3656769061504,41.8559910294082,42.346305152666,42.8366192759238,
43.3269333991816,43.8172475224394,44.3075616456971,44.7978757689549,45.2881898922127,
45.7785040154705,46.2688181387283,46.7591322619861,47.1238898038469),
 .UNSPECIFIED.);
#285=B_SPLINE_CURVE_WITH_KNOTS('',3,(#20723,#20724,#20725,#20726,#20727,
#20728,#20729,#20730,#20731,#20732,#20733,#20734,#20735,#20736,#20737,#20738,
#20739),.UNSPECIFIED.,.F.,.F.,(4,1,1,1,1,1,1,1,1,1,1,1,1,1,4),(34.5575191894877,
34.8964974579671,35.3868115812249,35.8771257044827,36.3674398277405,36.8577539509983,
37.3480680742561,37.8383821975139,38.3286963207716,38.8190104440294,39.3093245672872,
39.799638690545,40.2899528138028,40.7802669370606,40.8407044966673),
 .UNSPECIFIED.);
#286=B_SPLINE_CURVE_WITH_KNOTS('',3,(#20740,#20741,#20742,#20743,#20744,
#20745,#20746,#20747,#20748,#20749,#20750,#20751,#20752,#20753,#20754,#20755),
 .UNSPECIFIED.,.F.,.F.,(4,1,1,1,1,1,1,1,1,1,1,1,1,4),(34.5575191894877,
34.9915933037991,35.4819074270569,35.9722215503147,36.4625356735725,36.9528497968303,
37.4431639200881,37.9334780433459,38.4237921666036,38.9141062898614,39.4044204131192,
39.894734536377,40.3850486596348,40.8407044966673),.UNSPECIFIED.);
#287=B_SPLINE_CURVE_WITH_KNOTS('',3,(#20760,#20761,#20762,#20763,#20764,
#20765,#20766,#20767,#20768,#20769,#20770,#20771,#20772,#20773,#20774,#20775,
#20776),.UNSPECIFIED.,.F.,.F.,(4,1,1,1,1,1,1,1,1,1,1,1,1,1,4),(28.2743338823081,
28.5224138556158,29.0127279788736,29.5030421021314,29.9933562253892,30.483670348647,
30.9739844719048,31.4642985951626,31.9546127184203,32.4449268416781,32.9352409649359,
33.4255550881937,33.9158692114515,34.4061833347093,34.5575191894877),
 .UNSPECIFIED.);
#288=B_SPLINE_CURVE_WITH_KNOTS('',3,(#20777,#20778,#20779,#20780,#20781,
#20782,#20783,#20784,#20785,#20786,#20787,#20788,#20789,#20790,#20791,#20792,
#20793),.UNSPECIFIED.,.F.,.F.,(4,1,1,1,1,1,1,1,1,1,1,1,1,1,4),(28.2743338823081,
28.6175097014478,29.1078238247056,29.5981379479634,30.0884520712212,30.578766194479,
31.0690803177368,31.5593944409946,32.0497085642524,32.5400226875101,33.0303368107679,
33.5206509340257,34.0109650572835,34.5012791805413,34.5575191894877),
 .UNSPECIFIED.);
#289=B_SPLINE_CURVE_WITH_KNOTS('',3,(#20798,#20799,#20800,#20801,#20802,
#20803,#20804,#20805,#20806,#20807,#20808,#20809,#20810,#20811,#20812,#20813,
#20814),.UNSPECIFIED.,.F.,.F.,(4,1,1,1,1,1,1,1,1,1,1,1,1,1,4),(21.9911485751285,
22.1483302532645,22.6386443765223,23.1289584997801,23.6192726230379,24.1095867462957,
24.5999008695535,25.0902149928113,25.5805291160691,26.0708432393268,26.5611573625846,
27.0514714858424,27.5417856091002,28.032099732358,28.2743338823081),
 .UNSPECIFIED.);
#290=B_SPLINE_CURVE_WITH_KNOTS('',3,(#20815,#20816,#20817,#20818,#20819,
#20820,#20821,#20822,#20823,#20824,#20825,#20826,#20827,#20828,#20829,#20830,
#20831),.UNSPECIFIED.,.F.,.F.,(4,1,1,1,1,1,1,1,1,1,1,1,1,1,4),(21.9911485751285,
22.2434260990965,22.7337402223543,23.2240543456121,23.7143684688699,24.2046825921277,
24.6949967153855,25.1853108386433,25.6756249619011,26.1659390851589,26.6562532084167,
27.1465673316744,27.6368814549322,28.12719557819,28.2743338823081),
 .UNSPECIFIED.);
#291=B_SPLINE_CURVE_WITH_KNOTS('',3,(#20837,#20838,#20839,#20840,#20841,
#20842),.UNSPECIFIED.,.F.,.F.,(4,1,1,4),(14.3984001269719,14.8887142502297,
15.3790283734874,15.7079632679489),.UNSPECIFIED.);
#292=B_SPLINE_CURVE_WITH_KNOTS('',3,(#20845,#20846,#20847,#20848,#20849,
#20850,#20851),.UNSPECIFIED.,.F.,.F.,(4,1,1,1,4),(13.8759337553363,14.3033042811398,
14.7936184043976,15.2839325276554,15.7079632679489),.UNSPECIFIED.);
#293=B_SPLINE_CURVE_WITH_KNOTS('',3,(#20857,#20858,#20859,#20860,#20861,
#20862,#20863,#20864,#20865,#20866,#20867,#20868,#20869,#20870,#20871,#20872),
 .UNSPECIFIED.,.F.,.F.,(4,3,3,3,3,4),(114.407157784405,114.712345376808,
115.709844032258,116.707342687709,117.704841343159,118.70233999861),
 .UNSPECIFIED.);
#294=B_SPLINE_CURVE_WITH_KNOTS('',3,(#20880,#20881,#20882,#20883,#20884,
#20885,#20886,#20887,#20888,#20889,#20890,#20891,#20892,#20893,#20894,#20895,
#20896,#20897,#20898,#20899,#20900,#20901),.UNSPECIFIED.,.F.,.F.,(4,3,3,
3,3,3,3,4),(-116.687727133335,-115.709844032258,-114.712345376808,-113.714846721357,
-112.717348065907,-111.719849410456,-110.722350755006,-110.660533485745),
 .UNSPECIFIED.);
#295=B_SPLINE_CURVE_WITH_KNOTS('',3,(#20906,#20907,#20908,#20909,#20910,
#20911,#20912,#20913,#20914,#20915,#20916,#20917,#20918,#20919,#20920,#20921,
#20922,#20923,#20924,#20925,#20926,#20927),.UNSPECIFIED.,.F.,.F.,(4,3,3,
3,3,3,3,4),(108.123972477225,108.727353444105,109.724852099555,110.722350755006,
111.719849410456,112.717348065907,113.714846721357,114.407157784405),
 .UNSPECIFIED.);
#296=B_SPLINE_CURVE_WITH_KNOTS('',3,(#20928,#20929,#20930,#20931,#20932,
#20933,#20934,#20935,#20936,#20937,#20938,#20939,#20940,#20941,#20942,#20943,
#20944,#20945,#20946,#20947,#20948,#20949),.UNSPECIFIED.,.F.,.F.,(4,3,3,
3,3,3,3,4),(-110.660533485745,-109.724852099555,-108.727353444105,-107.729854788654,
-106.732356133204,-105.734857477753,-104.737358822303,-104.377348178566),
 .UNSPECIFIED.);
#297=B_SPLINE_CURVE_WITH_KNOTS('',3,(#20954,#20955,#20956,#20957,#20958,
#20959,#20960,#20961,#20962,#20963,#20964,#20965,#20966,#20967,#20968,#20969,
#20970,#20971,#20972,#20973,#20974,#20975),.UNSPECIFIED.,.F.,.F.,(4,3,3,
3,3,3,3,4),(101.840787170045,102.742361511402,103.739860166852,104.737358822303,
105.734857477753,106.732356133204,107.729854788654,108.123972477225),
 .UNSPECIFIED.);
#298=B_SPLINE_CURVE_WITH_KNOTS('',3,(#20976,#20977,#20978,#20979,#20980,
#20981,#20982,#20983,#20984,#20985,#20986,#20987,#20988,#20989,#20990,#20991,
#20992,#20993,#20994,#20995,#20996,#20997),.UNSPECIFIED.,.F.,.F.,(4,3,3,
3,3,3,3,4),(-104.377348178566,-103.739860166852,-102.742361511402,-101.744862855951,
-100.747364200501,-99.7498655450501,-98.7523668895996,-98.094162871386),
 .UNSPECIFIED.);
#299=B_SPLINE_CURVE_WITH_KNOTS('',3,(#21002,#21003,#21004,#21005,#21006,
#21007,#21008,#21009,#21010,#21011,#21012,#21013,#21014,#21015,#21016,#21017,
#21018,#21019,#21020,#21021,#21022,#21023,#21024,#21025,#21026),
 .UNSPECIFIED.,.F.,.F.,(4,3,3,3,3,3,3,3,4),(95.5576018628658,95.7598709232481,
96.7573695786986,97.7548682341491,98.7523668895996,99.7498655450502,100.747364200501,
101.744862855951,101.840787170045),.UNSPECIFIED.);
#300=B_SPLINE_CURVE_WITH_KNOTS('',3,(#21027,#21028,#21029,#21030,#21031,
#21032,#21033,#21034,#21035,#21036,#21037,#21038,#21039,#21040,#21041,#21042,
#21043,#21044,#21045,#21046,#21047,#21048),.UNSPECIFIED.,.F.,.F.,(4,3,3,
3,3,3,3,4),(-98.094162871386,-97.7548682341491,-96.7573695786986,-95.7598709232481,
-94.7623722677976,-93.7648736123471,-92.7673749568966,-91.8109775642064),
 .UNSPECIFIED.);
#301=B_SPLINE_CURVE_WITH_KNOTS('',3,(#21053,#21054,#21055,#21056,#21057,
#21058,#21059,#21060,#21061,#21062,#21063,#21064,#21065,#21066,#21067,#21068,
#21069,#21070,#21071,#21072,#21073,#21074),.UNSPECIFIED.,.F.,.F.,(4,3,3,
3,3,3,3,4),(89.2744165556862,89.7748789905451,90.7723776459956,91.7698763014461,
92.7673749568966,93.7648736123471,94.7623722677976,95.5576018628658),
 .UNSPECIFIED.);
#302=B_SPLINE_CURVE_WITH_KNOTS('',3,(#21075,#21076,#21077,#21078,#21079,
#21080,#21081,#21082,#21083,#21084,#21085,#21086,#21087,#21088,#21089,#21090,
#21091,#21092,#21093,#21094,#21095,#21096,#21097,#21098,#21099),
 .UNSPECIFIED.,.F.,.F.,(4,3,3,3,3,3,3,3,4),(-91.8109775642064,-91.7698763014461,
-90.7723776459956,-89.7748789905451,-88.7773803350946,-87.7798816796441,
-86.7823830241936,-85.7848843687431,-85.5277922570269),.UNSPECIFIED.);
#303=B_SPLINE_CURVE_WITH_KNOTS('',3,(#21104,#21105,#21106,#21107,#21108,
#21109,#21110,#21111,#21112,#21113,#21114,#21115,#21116,#21117,#21118,#21119,
#21120,#21121,#21122,#21123,#21124,#21125),.UNSPECIFIED.,.F.,.F.,(4,3,3,
3,3,3,3,4),(82.9912312485066,83.7898870578421,84.7873857132926,85.7848843687431,
86.7823830241936,87.7798816796441,88.7773803350946,89.2744165556862),
 .UNSPECIFIED.);
#304=B_SPLINE_CURVE_WITH_KNOTS('',3,(#21126,#21127,#21128,#21129,#21130,
#21131,#21132,#21133,#21134,#21135,#21136,#21137,#21138,#21139,#21140,#21141,
#21142,#21143,#21144,#21145,#21146,#21147),.UNSPECIFIED.,.F.,.F.,(4,3,3,
3,3,3,3,4),(-85.5277922570269,-84.7873857132926,-83.7898870578422,-82.7923884023916,
-81.7948897469411,-80.7973910914906,-79.7998924360401,-79.2446069498473),
 .UNSPECIFIED.);
#305=B_SPLINE_CURVE_WITH_KNOTS('',3,(#21152,#21153,#21154,#21155,#21156,
#21157,#21158,#21159,#21160,#21161,#21162,#21163,#21164,#21165,#21166,#21167,
#21168,#21169,#21170,#21171,#21172,#21173,#21174,#21175,#21176),
 .UNSPECIFIED.,.F.,.F.,(4,3,3,3,3,3,3,3,4),(76.708045941327,76.8073964696886,
77.8048951251391,78.8023937805896,79.7998924360401,80.7973910914906,81.7948897469411,
82.7923884023916,82.9912312485066),.UNSPECIFIED.);
#306=B_SPLINE_CURVE_WITH_KNOTS('',3,(#21177,#21178,#21179,#21180,#21181,
#21182,#21183,#21184,#21185,#21186,#21187,#21188,#21189,#21190,#21191,#21192,
#21193,#21194,#21195,#21196,#21197,#21198),.UNSPECIFIED.,.F.,.F.,(4,3,3,
3,3,3,3,4),(-79.2446069498473,-78.8023937805896,-77.8048951251391,-76.8073964696886,
-75.8098978142381,-74.8123991587876,-73.8149005033371,-72.9614216426677),
 .UNSPECIFIED.);
#307=B_SPLINE_CURVE_WITH_KNOTS('',3,(#21203,#21204,#21205,#21206,#21207,
#21208,#21209,#21210,#21211,#21212,#21213,#21214,#21215,#21216,#21217,#21218,
#21219,#21220,#21221,#21222,#21223,#21224),.UNSPECIFIED.,.F.,.F.,(4,3,3,
3,3,3,3,4),(70.4248606341474,70.8224045369856,71.8199031924361,72.8174018478866,
73.8149005033371,74.8123991587876,75.8098978142381,76.708045941327),
 .UNSPECIFIED.);
#308=B_SPLINE_CURVE_WITH_KNOTS('',3,(#21225,#21226,#21227,#21228,#21229,
#21230,#21231,#21232,#21233,#21234,#21235,#21236,#21237,#21238,#21239,#21240,
#21241,#21242,#21243,#21244,#21245,#21246,#21247,#21248,#21249),
 .UNSPECIFIED.,.F.,.F.,(4,3,3,3,3,3,3,3,4),(-72.9614216426677,-72.8174018478866,
-71.8199031924361,-70.8224045369856,-69.8249058815351,-68.8274072260846,
-67.8299085706341,-66.8324099151836,-66.6782363354882),.UNSPECIFIED.);
#309=B_SPLINE_CURVE_WITH_KNOTS('',3,(#21254,#21255,#21256,#21257,#21258,
#21259,#21260,#21261,#21262,#21263,#21264,#21265,#21266,#21267,#21268,#21269,
#21270,#21271,#21272,#21273,#21274,#21275),.UNSPECIFIED.,.F.,.F.,(4,3,3,
3,3,3,3,4),(64.1416753269678,64.8374126042826,65.8349112597331,66.8324099151836,
67.8299085706341,68.8274072260846,69.8249058815351,70.4248606341474),
 .UNSPECIFIED.);
#310=B_SPLINE_CURVE_WITH_KNOTS('',3,(#21276,#21277,#21278,#21279,#21280,
#21281,#21282,#21283,#21284,#21285,#21286,#21287,#21288,#21289,#21290,#21291,
#21292,#21293,#21294,#21295,#21296,#21297),.UNSPECIFIED.,.F.,.F.,(4,3,3,
3,3,3,3,4),(-66.6782363354882,-65.8349112597331,-64.8374126042826,-63.8399139488321,
-62.8424152933816,-61.8449166379311,-60.8474179824806,-60.3950510283085),
 .UNSPECIFIED.);
#311=B_SPLINE_CURVE_WITH_KNOTS('',3,(#21302,#21303,#21304,#21305,#21306,
#21307,#21308,#21309,#21310,#21311,#21312,#21313,#21314,#21315,#21316,#21317,
#21318,#21319,#21320,#21321,#21322,#21323),.UNSPECIFIED.,.F.,.F.,(4,3,3,
3,3,3,3,4),(57.8584900197882,58.8524206715796,59.8499193270301,60.8474179824806,
61.8449166379311,62.8424152933816,63.8399139488321,64.1416753269678),
 .UNSPECIFIED.);
#312=B_SPLINE_CURVE_WITH_KNOTS('',3,(#21324,#21325,#21326,#21327,#21328,
#21329,#21330,#21331,#21332,#21333,#21334,#21335,#21336,#21337,#21338,#21339,
#21340,#21341,#21342,#21343,#21344,#21345),.UNSPECIFIED.,.F.,.F.,(4,3,3,
3,3,3,3,4),(-60.3950510283085,-59.8499193270301,-58.8524206715796,-57.8549220161291,
-56.8574233606786,-55.8599247052281,-54.8624260497776,-54.1118657211289),
 .UNSPECIFIED.);
#313=B_SPLINE_CURVE_WITH_KNOTS('',3,(#21350,#21351,#21352,#21353,#21354,
#21355,#21356,#21357,#21358,#21359,#21360,#21361,#21362,#21363,#21364,#21365,
#21366,#21367,#21368,#21369,#21370,#21371,#21372,#21373,#21374),
 .UNSPECIFIED.,.F.,.F.,(4,3,3,3,3,3,3,3,4),(51.5753047126086,51.8699300834261,
52.8674287388766,53.8649273943271,54.8624260497776,55.8599247052281,56.8574233606786,
57.8549220161291,57.8584900197882),.UNSPECIFIED.);
#314=B_SPLINE_CURVE_WITH_KNOTS('',3,(#21375,#21376,#21377,#21378,#21379,
#21380,#21381,#21382,#21383,#21384,#21385,#21386,#21387,#21388,#21389,#21390,
#21391,#21392,#21393,#21394,#21395,#21396,#21397,#21398,#21399),
 .UNSPECIFIED.,.F.,.F.,(4,3,3,3,3,3,3,3,4),(-54.1118657211289,-53.8649273943271,
-52.8674287388766,-51.8699300834261,-50.8724314279756,-49.8749327725251,
-48.8774341170746,-47.8799354616241,-47.8286804139493),.UNSPECIFIED.);
#315=B_SPLINE_CURVE_WITH_KNOTS('',3,(#21404,#21405,#21406,#21407,#21408,
#21409,#21410,#21411,#21412,#21413,#21414,#21415,#21416,#21417,#21418,#21419,
#21420,#21421,#21422,#21423,#21424,#21425),.UNSPECIFIED.,.F.,.F.,(4,3,3,
3,3,3,3,4),(45.292119405429,45.8849381507231,46.8824368061736,47.8799354616241,
48.8774341170746,49.8749327725251,50.8724314279756,51.5753047126086),
 .UNSPECIFIED.);
#316=B_SPLINE_CURVE_WITH_KNOTS('',3,(#21426,#21427,#21428,#21429,#21430,
#21431,#21432,#21433,#21434,#21435,#21436,#21437,#21438,#21439,#21440,#21441,
#21442,#21443,#21444,#21445,#21446,#21447),.UNSPECIFIED.,.F.,.F.,(4,3,3,
3,3,3,3,4),(-47.8286804139493,-46.8824368061736,-45.8849381507231,-44.8874394952726,
-43.8899408398221,-42.8924421843716,-41.8949435289211,-41.5454951067697),
 .UNSPECIFIED.);
#317=B_SPLINE_CURVE_WITH_KNOTS('',3,(#21452,#21453,#21454,#21455,#21456,
#21457,#21458,#21459,#21460,#21461,#21462,#21463,#21464,#21465,#21466,#21467,
#21468,#21469,#21470,#21471,#21472,#21473),.UNSPECIFIED.,.F.,.F.,(4,3,3,
3,3,3,3,4),(39.0089340982495,39.8999462180201,40.8974448734706,41.8949435289211,
42.8924421843716,43.8899408398221,44.8874394952726,45.292119405429),
 .UNSPECIFIED.);
#318=B_SPLINE_CURVE_WITH_KNOTS('',3,(#21474,#21475,#21476,#21477,#21478,
#21479,#21480,#21481,#21482,#21483,#21484,#21485,#21486,#21487,#21488,#21489,
#21490,#21491,#21492,#21493,#21494,#21495),.UNSPECIFIED.,.F.,.F.,(4,3,3,
3,3,3,3,4),(-41.5454951067697,-40.8974448734706,-39.8999462180201,-38.9024475625696,
-37.9049489071191,-36.9074502516685,-35.909951596218,-35.2623097995902),
 .UNSPECIFIED.);
#319=B_SPLINE_CURVE_WITH_KNOTS('',3,(#21500,#21501,#21502,#21503,#21504,
#21505,#21506,#21507,#21508,#21509,#21510,#21511,#21512,#21513,#21514,#21515,
#21516,#21517,#21518,#21519,#21520,#21521,#21522,#21523,#21524),
 .UNSPECIFIED.,.F.,.F.,(4,3,3,3,3,3,3,3,4),(32.7257487910699,32.9174556298666,
33.9149542853171,34.9124529407676,35.9099515962181,36.9074502516685,37.9049489071191,
38.9024475625696,39.0089340982495),.UNSPECIFIED.);
#320=B_SPLINE_CURVE_WITH_KNOTS('',3,(#21525,#21526,#21527,#21528,#21529,
#21530,#21531,#21532,#21533,#21534,#21535,#21536,#21537,#21538,#21539,#21540,
#21541,#21542,#21543,#21544,#21545,#21546),.UNSPECIFIED.,.F.,.F.,(4,3,3,
3,3,3,3,4),(-35.2623097995902,-34.9124529407676,-33.9149542853171,-32.9174556298665,
-31.919956974416,-30.9224583189655,-29.9249596635151,-28.9791244924106),
 .UNSPECIFIED.);
#321=B_SPLINE_CURVE_WITH_KNOTS('',3,(#21551,#21552,#21553,#21554,#21555,
#21556,#21557,#21558,#21559,#21560,#21561,#21562,#21563,#21564,#21565,#21566,
#21567,#21568,#21569,#21570,#21571,#21572),.UNSPECIFIED.,.F.,.F.,(4,3,3,
3,3,3,3,4),(26.4425634838902,26.9324636971635,27.929962352614,28.9274610080645,
29.924959663515,30.9224583189655,31.9199569744161,32.7257487910699),
 .UNSPECIFIED.);
#322=B_SPLINE_CURVE_WITH_KNOTS('',3,(#21573,#21574,#21575,#21576,#21577,
#21578,#21579,#21580,#21581,#21582,#21583,#21584,#21585,#21586,#21587,#21588,
#21589,#21590,#21591,#21592,#21593,#21594,#21595,#21596,#21597),
 .UNSPECIFIED.,.F.,.F.,(4,3,3,3,3,3,3,3,4),(-28.9791244924106,-28.9274610080645,
-27.929962352614,-26.9324636971635,-25.934965041713,-24.9374663862625,-23.939967730812,
-22.9424690753615,-22.6959391852309),.UNSPECIFIED.);
#323=B_SPLINE_CURVE_WITH_KNOTS('',3,(#21602,#21603,#21604,#21605,#21606,
#21607,#21608,#21609,#21610,#21611,#21612,#21613,#21614,#21615,#21616,#21617,
#21618,#21619,#21620,#21621,#21622,#21623),.UNSPECIFIED.,.F.,.F.,(4,3,3,
3,3,3,3,4),(20.1593781767107,20.9474717644605,21.944970419911,22.9424690753615,
23.939967730812,24.9374663862625,25.934965041713,26.4425634838902),
 .UNSPECIFIED.);
#324=B_SPLINE_CURVE_WITH_KNOTS('',3,(#21624,#21625,#21626,#21627,#21628,
#21629,#21630,#21631,#21632,#21633,#21634,#21635,#21636,#21637,#21638,#21639,
#21640,#21641,#21642,#21643,#21644,#21645),.UNSPECIFIED.,.F.,.F.,(4,3,3,
3,3,3,3,4),(-22.6959391852309,-21.944970419911,-20.9474717644605,-19.94997310901,
-18.9524744535595,-17.954975798109,-16.9574771426585,-16.4127538780514),
 .UNSPECIFIED.);
#325=B_SPLINE_CURVE_WITH_KNOTS('',3,(#21650,#21651,#21652,#21653,#21654,
#21655,#21656,#21657,#21658,#21659,#21660,#21661,#21662,#21663,#21664,#21665,
#21666,#21667,#21668,#21669,#21670,#21671,#21672,#21673,#21674),
 .UNSPECIFIED.,.F.,.F.,(4,3,3,3,3,3,3,3,4),(13.8761928695311,13.964981176307,
14.9624798317575,15.959978487208,16.9574771426585,17.954975798109,18.9524744535595,
19.94997310901,20.1593781767107),.UNSPECIFIED.);
#326=B_SPLINE_CURVE_WITH_KNOTS('',3,(#21675,#21676,#21677,#21678,#21679,
#21680,#21681,#21682,#21683,#21684,#21685,#21686,#21687,#21688,#21689,#21690,
#21691,#21692,#21693,#21694,#21695,#21696),.UNSPECIFIED.,.F.,.F.,(4,3,3,
3,3,3,3,4),(-16.4127538780514,-15.959978487208,-14.9624798317575,-13.964981176307,
-12.9674825208565,-11.969983865406,-10.9724852099555,-10.1295685708718),
 .UNSPECIFIED.);
#327=B_SPLINE_CURVE_WITH_KNOTS('',3,(#21702,#21703,#21704,#21705,#21706,
#21707,#21708,#21709,#21710,#21711,#21712,#21713,#21714),.UNSPECIFIED.,
 .F.,.F.,(4,3,3,3,4),(-3.84638326369218,-2.9924959663515,-1.994997310901,
-0.997498655450501,0.),.UNSPECIFIED.);
#328=B_SPLINE_CURVE_WITH_KNOTS('',3,(#21717,#21718,#21719,#21720,#21721,
#21722,#21723,#21724,#21725,#21726,#21727,#21728,#21729,#21730,#21731,#21732,
#21733,#21734,#21735),.UNSPECIFIED.,.F.,.F.,(4,3,3,3,3,3,4),(2.01461286527449,
2.9924959663515,3.989994621802,4.98749327725251,5.98499193270301,6.98249058815351,
7.59300756235149),.UNSPECIFIED.);
#329=B_SPLINE_CURVE_WITH_KNOTS('',3,(#21741,#21742,#21743,#21744,#21745),
 .UNSPECIFIED.,.F.,.F.,(4,1,4),(128.805298797182,129.566421347416,130.563920002866),
 .UNSPECIFIED.);
#330=B_SPLINE_CURVE_WITH_KNOTS('',3,(#21748,#21749,#21750,#21751,#21752,
#21753),.UNSPECIFIED.,.F.,.F.,(4,1,1,4),(128.805298797182,129.110486389585,
130.107985045035,131.085868146112),.UNSPECIFIED.);
#331=B_SPLINE_CURVE_WITH_KNOTS('',3,(#21758,#21759,#21760,#21761,#21762,
#21763,#21764,#21765,#21766,#21767,#21768),.UNSPECIFIED.,.F.,.F.,(4,1,1,
1,1,1,1,1,4),(122.522113490002,122.583930759262,123.581429414713,124.578928070163,
125.576426725614,126.573925381064,127.571424036515,128.568922691965,128.805298797182),
 .UNSPECIFIED.);
#332=B_SPLINE_CURVE_WITH_KNOTS('',3,(#21769,#21770,#21771,#21772,#21773,
#21774,#21775,#21776,#21777,#21778),.UNSPECIFIED.,.F.,.F.,(4,1,1,1,1,1,
1,4),(122.522113490002,123.125494456882,124.122993112332,125.120491767783,
126.117990423233,127.115489078684,128.112987734134,128.805298797182),
 .UNSPECIFIED.);
#333=B_SPLINE_CURVE_WITH_KNOTS('',3,(#21783,#21784,#21785,#21786,#21787,
#21788,#21789,#21790,#21791,#21792),.UNSPECIFIED.,.F.,.F.,(4,1,1,1,1,1,
1,4),(116.238928182822,116.598938826559,117.59643748201,118.59393613746,
119.591434792911,120.588933448361,121.586432103812,122.522113490002),
 .UNSPECIFIED.);
#334=B_SPLINE_CURVE_WITH_KNOTS('',3,(#21793,#21794,#21795,#21796,#21797,
#21798,#21799,#21800,#21801,#21802),.UNSPECIFIED.,.F.,.F.,(4,1,1,1,1,1,
1,4),(116.238928182822,117.140502524179,118.138001179629,119.13549983508,
120.13299849053,121.130497145981,122.127995801431,122.522113490002),
 .UNSPECIFIED.);
#335=B_SPLINE_CURVE_WITH_KNOTS('',3,(#21807,#21808,#21809,#21810,#21811,
#21812,#21813,#21814,#21815,#21816),.UNSPECIFIED.,.F.,.F.,(4,1,1,1,1,1,
1,4),(109.955742875643,110.613946893856,111.611445549307,112.608944204757,
113.606442860208,114.603941515658,115.601440171109,116.238928182822),
 .UNSPECIFIED.);
#336=B_SPLINE_CURVE_WITH_KNOTS('',3,(#21817,#21818,#21819,#21820,#21821,
#21822,#21823,#21824,#21825,#21826,#21827),.UNSPECIFIED.,.F.,.F.,(4,1,1,
1,1,1,1,1,4),(109.955742875643,110.158011936025,111.155510591476,112.153009246926,
113.150507902377,114.148006557827,115.145505213278,116.143003868728,116.238928182822),
 .UNSPECIFIED.);
#337=B_SPLINE_CURVE_WITH_KNOTS('',3,(#21832,#21833,#21834,#21835,#21836,
#21837,#21838,#21839,#21840,#21841),.UNSPECIFIED.,.F.,.F.,(4,1,1,1,1,1,
1,4),(103.672557568463,104.628954961153,105.626453616604,106.623952272054,
107.621450927505,108.618949582955,109.616448238406,109.955742875643),
 .UNSPECIFIED.);
#338=B_SPLINE_CURVE_WITH_KNOTS('',3,(#21842,#21843,#21844,#21845,#21846,
#21847,#21848,#21849,#21850,#21851),.UNSPECIFIED.,.F.,.F.,(4,1,1,1,1,1,
1,4),(103.672557568463,104.173020003322,105.170518658772,106.168017314223,
107.165515969673,108.163014625124,109.160513280574,109.955742875643),
 .UNSPECIFIED.);
#339=B_SPLINE_CURVE_WITH_KNOTS('',3,(#21856,#21857,#21858,#21859,#21860,
#21861,#21862,#21863,#21864,#21865,#21866),.UNSPECIFIED.,.F.,.F.,(4,1,1,
1,1,1,1,1,4),(97.3893722612835,97.6464643729998,98.6439630284503,99.6414616839008,
100.638960339351,101.636458994802,102.633957650252,103.631456305703,103.672557568463),
 .UNSPECIFIED.);
#340=B_SPLINE_CURVE_WITH_KNOTS('',3,(#21867,#21868,#21869,#21870,#21871,
#21872,#21873,#21874,#21875,#21876),.UNSPECIFIED.,.F.,.F.,(4,1,1,1,1,1,
1,4),(97.3893722612835,98.188028070619,99.1855267260695,100.18302538152,
101.18052403697,102.178022692421,103.175521347871,103.672557568463),
 .UNSPECIFIED.);
#341=B_SPLINE_CURVE_WITH_KNOTS('',3,(#21881,#21882,#21883,#21884,#21885,
#21886,#21887,#21888,#21889,#21890),.UNSPECIFIED.,.F.,.F.,(4,1,1,1,1,1,
1,4),(91.106186954104,91.6614724402968,92.6589710957473,93.6564697511978,
94.6539684066483,95.6514670620988,96.6489657175493,97.3893722612835),
 .UNSPECIFIED.);
#342=B_SPLINE_CURVE_WITH_KNOTS('',3,(#21891,#21892,#21893,#21894,#21895,
#21896,#21897,#21898,#21899,#21900,#21901),.UNSPECIFIED.,.F.,.F.,(4,1,1,
1,1,1,1,1,4),(91.106186954104,91.2055374824655,92.203036137916,93.2005347933665,
94.198033448817,95.1955321042675,96.193030759718,97.1905294151685,97.3893722612835),
 .UNSPECIFIED.);
#343=B_SPLINE_CURVE_WITH_KNOTS('',3,(#21906,#21907,#21908,#21909,#21910,
#21911,#21912,#21913,#21914,#21915),.UNSPECIFIED.,.F.,.F.,(4,1,1,1,1,1,
1,4),(84.8230016469244,85.6764805075938,86.6739791630443,87.6714778184948,
88.6689764739453,89.6664751293958,90.6639737848463,91.106186954104),
 .UNSPECIFIED.);
#344=B_SPLINE_CURVE_WITH_KNOTS('',3,(#21916,#21917,#21918,#21919,#21920,
#21921,#21922,#21923,#21924,#21925),.UNSPECIFIED.,.F.,.F.,(4,1,1,1,1,1,
1,4),(84.8230016469244,85.2205455497625,86.218044205213,87.2155428606635,
88.213041516114,89.2105401715645,90.208038827015,91.106186954104),
 .UNSPECIFIED.);
#345=B_SPLINE_CURVE_WITH_KNOTS('',3,(#21930,#21931,#21932,#21933,#21934,
#21935,#21936,#21937,#21938,#21939,#21940),.UNSPECIFIED.,.F.,.F.,(4,1,1,
1,1,1,1,1,4),(78.5398163397448,78.6939899194402,79.6914885748908,80.6889872303413,
81.6864858857918,82.6839845412423,83.6814831966928,84.6789818521433,84.8230016469244),
 .UNSPECIFIED.);
#346=B_SPLINE_CURVE_WITH_KNOTS('',3,(#21941,#21942,#21943,#21944,#21945,
#21946,#21947,#21948,#21949,#21950),.UNSPECIFIED.,.F.,.F.,(4,1,1,1,1,1,
1,4),(78.5398163397448,79.2355536170595,80.23305227251,81.2305509279605,
82.228049583411,83.2255482388615,84.223046894312,84.8230016469244),
 .UNSPECIFIED.);
#347=B_SPLINE_CURVE_WITH_KNOTS('',3,(#21955,#21956,#21957,#21958,#21959,
#21960,#21961,#21962,#21963,#21964),.UNSPECIFIED.,.F.,.F.,(4,1,1,1,1,1,
1,4),(72.2566310325652,72.7089979867372,73.7064966421877,74.7039952976382,
75.7014939530887,76.6989926085392,77.6964912639897,78.5398163397448),
 .UNSPECIFIED.);
#348=B_SPLINE_CURVE_WITH_KNOTS('',3,(#21965,#21966,#21967,#21968,#21969,
#21970,#21971,#21972,#21973,#21974),.UNSPECIFIED.,.F.,.F.,(4,1,1,1,1,1,
1,4),(72.2566310325652,73.2505616843565,74.248060339807,75.2455589952575,
76.243057650708,77.2405563061585,78.238054961609,78.5398163397448),
 .UNSPECIFIED.);
#349=B_SPLINE_CURVE_WITH_KNOTS('',3,(#21979,#21980,#21981,#21982,#21983,
#21984,#21985,#21986,#21987,#21988),.UNSPECIFIED.,.F.,.F.,(4,1,1,1,1,1,
1,4),(65.9734457253856,66.7240060540342,67.7215047094847,68.7190033649352,
69.7165020203857,70.7140006758362,71.7114993312867,72.2566310325652),
 .UNSPECIFIED.);
#350=B_SPLINE_CURVE_WITH_KNOTS('',3,(#21989,#21990,#21991,#21992,#21993,
#21994,#21995,#21996,#21997,#21998,#21999),.UNSPECIFIED.,.F.,.F.,(4,1,1,
1,1,1,1,1,4),(65.9734457253856,66.2680710962029,67.2655697516534,68.2630684071039,
69.2605670625544,70.2580657180049,71.2555643734554,72.2530630289059,72.2566310325652),
 .UNSPECIFIED.);
#351=B_SPLINE_CURVE_WITH_KNOTS('',3,(#22004,#22005,#22006,#22007,#22008,
#22009,#22010,#22011,#22012,#22013,#22014),.UNSPECIFIED.,.F.,.F.,(4,1,1,
1,1,1,1,1,4),(59.690260418206,59.7415154658807,60.7390141213312,61.7365127767817,
62.7340114322322,63.7315100876827,64.7290087431332,65.7265073985837,65.9734457253856),
 .UNSPECIFIED.);
#352=B_SPLINE_CURVE_WITH_KNOTS('',3,(#22015,#22016,#22017,#22018,#22019,
#22020,#22021,#22022,#22023,#22024),.UNSPECIFIED.,.F.,.F.,(4,1,1,1,1,1,
1,4),(59.690260418206,60.2830791634999,61.2805778189504,62.2780764744009,
63.2755751298514,64.2730737853019,65.2705724407524,65.9734457253856),
 .UNSPECIFIED.);
#353=B_SPLINE_CURVE_WITH_KNOTS('',3,(#22029,#22030,#22031,#22032,#22033,
#22034,#22035,#22036,#22037,#22038),.UNSPECIFIED.,.F.,.F.,(4,1,1,1,1,1,
1,4),(53.4070751110264,53.7565235331777,54.7540221886282,55.7515208440787,
56.7490194995292,57.7465181549797,58.7440168104302,59.690260418206),
 .UNSPECIFIED.);
#354=B_SPLINE_CURVE_WITH_KNOTS('',3,(#22039,#22040,#22041,#22042,#22043,
#22044,#22045,#22046,#22047,#22048),.UNSPECIFIED.,.F.,.F.,(4,1,1,1,1,1,
1,4),(53.4070751110264,54.2980872307969,55.2955858862474,56.2930845416979,
57.2905831971484,58.2880818525989,59.2855805080494,59.690260418206),
 .UNSPECIFIED.);
#355=B_SPLINE_CURVE_WITH_KNOTS('',3,(#22053,#22054,#22055,#22056,#22057,
#22058,#22059,#22060,#22061,#22062),.UNSPECIFIED.,.F.,.F.,(4,1,1,1,1,1,
1,4),(47.1238898038468,47.7715316004747,48.7690302559252,49.7665289113757,
50.7640275668262,51.7615262222767,52.7590248777272,53.4070751110264),
 .UNSPECIFIED.);
#356=B_SPLINE_CURVE_WITH_KNOTS('',3,(#22063,#22064,#22065,#22066,#22067,
#22068,#22069,#22070,#22071,#22072,#22073),.UNSPECIFIED.,.F.,.F.,(4,1,1,
1,1,1,1,1,4),(47.1238898038468,47.3155966426434,48.3130952980939,49.3105939535444,
50.3080926089949,51.3055912644454,52.3030899198959,53.3005885753464,53.4070751110264),
 .UNSPECIFIED.);
#357=B_SPLINE_CURVE_WITH_KNOTS('',3,(#22078,#22079,#22080,#22081,#22082,
#22083,#22084,#22085,#22086,#22087),.UNSPECIFIED.,.F.,.F.,(4,1,1,1,1,1,
1,4),(40.8407044966672,41.7865396677717,42.7840383232222,43.7815369786727,
44.7790356341232,45.7765342895737,46.7740329450242,47.1238898038468),
 .UNSPECIFIED.);
#358=B_SPLINE_CURVE_WITH_KNOTS('',3,(#22088,#22089,#22090,#22091,#22092,
#22093,#22094,#22095,#22096,#22097),.UNSPECIFIED.,.F.,.F.,(4,1,1,1,1,1,
1,4),(40.8407044966672,41.3306047099404,42.3281033653909,43.3256020208414,
44.3231006762919,45.3205993317424,46.3180979871929,47.1238898038468),
 .UNSPECIFIED.);
#359=B_SPLINE_CURVE_WITH_KNOTS('',3,(#22102,#22103,#22104,#22105,#22106,
#22107,#22108,#22109,#22110,#22111,#22112),.UNSPECIFIED.,.F.,.F.,(4,1,1,
1,1,1,1,1,4),(34.5575191894877,34.8040490796182,35.8015477350687,36.7990463905192,
37.7965450459697,38.7940437014202,39.7915423568707,40.7890410123212,40.8407044966672),
 .UNSPECIFIED.);
#360=B_SPLINE_CURVE_WITH_KNOTS('',3,(#22113,#22114,#22115,#22116,#22117,
#22118,#22119,#22120,#22121,#22122),.UNSPECIFIED.,.F.,.F.,(4,1,1,1,1,1,
1,4),(34.5575191894877,35.3456127772374,36.3431114326879,37.3406100881384,
38.3381087435889,39.3356073990394,40.3331060544899,40.8407044966672),
 .UNSPECIFIED.);
#361=B_SPLINE_CURVE_WITH_KNOTS('',3,(#22127,#22128,#22129,#22130,#22131,
#22132,#22133,#22134,#22135,#22136),.UNSPECIFIED.,.F.,.F.,(4,1,1,1,1,1,
1,4),(28.2743338823081,28.8190571469152,29.8165558023657,30.8140544578162,
31.8115531132667,32.8090517687172,33.8065504241677,34.5575191894877),
 .UNSPECIFIED.);
#362=B_SPLINE_CURVE_WITH_KNOTS('',3,(#22137,#22138,#22139,#22140,#22141,
#22142,#22143,#22144,#22145,#22146,#22147),.UNSPECIFIED.,.F.,.F.,(4,1,1,
1,1,1,1,1,4),(28.2743338823081,28.3631221890839,29.3606208445344,30.3581194999849,
31.3556181554354,32.3531168108859,33.3506154663364,34.3481141217869,34.5575191894877),
 .UNSPECIFIED.);
#363=B_SPLINE_CURVE_WITH_KNOTS('',3,(#22152,#22153,#22154,#22155,#22156,
#22157,#22158,#22159,#22160,#22161),.UNSPECIFIED.,.F.,.F.,(4,1,1,1,1,1,
1,4),(21.9911485751284,22.8340652142122,23.8315638696627,24.8290625251132,
25.8265611805637,26.8240598360142,27.8215584914647,28.2743338823081),
 .UNSPECIFIED.);
#364=B_SPLINE_CURVE_WITH_KNOTS('',3,(#22162,#22163,#22164,#22165,#22166,
#22167,#22168,#22169,#22170,#22171),.UNSPECIFIED.,.F.,.F.,(4,1,1,1,1,1,
1,4),(21.9911485751284,22.3781302563809,23.3756289118314,24.3731275672819,
25.3706262227324,26.3681248781829,27.3656235336334,28.2743338823081),
 .UNSPECIFIED.);
#365=B_SPLINE_CURVE_WITH_KNOTS('',3,(#22177,#22178,#22179,#22180,#22181),
 .UNSPECIFIED.,.F.,.F.,(4,1,4),(14.3981410127769,15.3956396682274,15.7079632679489),
 .UNSPECIFIED.);
#366=B_SPLINE_CURVE_WITH_KNOTS('',3,(#22184,#22185,#22186,#22187,#22188),
 .UNSPECIFIED.,.F.,.F.,(4,1,4),(13.8761928695311,14.8540759706082,15.7079632679489),
 .UNSPECIFIED.);
#367=B_SPLINE_CURVE_WITH_KNOTS('',3,(#22194,#22195,#22196,#22197,#22198,
#22199,#22200,#22201,#22202,#22203,#22204,#22205,#22206,#22207,#22208,#22209),
 .UNSPECIFIED.,.F.,.F.,(4,3,3,3,3,4),(114.407157784405,114.712345376808,
115.709844032258,116.707342687709,117.704841343159,118.70233999861),
 .UNSPECIFIED.);
#368=B_SPLINE_CURVE_WITH_KNOTS('',3,(#22217,#22218,#22219,#22220,#22221,
#22222,#22223,#22224,#22225,#22226,#22227,#22228,#22229,#22230,#22231,#22232,
#22233,#22234,#22235,#22236,#22237,#22238),.UNSPECIFIED.,.F.,.F.,(4,3,3,
3,3,3,3,4),(-116.687727133335,-115.709844032258,-114.712345376808,-113.714846721357,
-112.717348065907,-111.719849410456,-110.722350755006,-110.660533485745),
 .UNSPECIFIED.);
#369=B_SPLINE_CURVE_WITH_KNOTS('',3,(#22243,#22244,#22245,#22246,#22247,
#22248,#22249,#22250,#22251,#22252,#22253,#22254,#22255,#22256,#22257,#22258,
#22259,#22260,#22261,#22262,#22263,#22264),.UNSPECIFIED.,.F.,.F.,(4,3,3,
3,3,3,3,4),(108.123972477225,108.727353444105,109.724852099555,110.722350755006,
111.719849410456,112.717348065907,113.714846721357,114.407157784405),
 .UNSPECIFIED.);
#370=B_SPLINE_CURVE_WITH_KNOTS('',3,(#22265,#22266,#22267,#22268,#22269,
#22270,#22271,#22272,#22273,#22274,#22275,#22276,#22277,#22278,#22279,#22280,
#22281,#22282,#22283,#22284,#22285,#22286),.UNSPECIFIED.,.F.,.F.,(4,3,3,
3,3,3,3,4),(-110.660533485745,-109.724852099555,-108.727353444105,-107.729854788654,
-106.732356133204,-105.734857477753,-104.737358822303,-104.377348178566),
 .UNSPECIFIED.);
#371=B_SPLINE_CURVE_WITH_KNOTS('',3,(#22291,#22292,#22293,#22294,#22295,
#22296,#22297,#22298,#22299,#22300,#22301,#22302,#22303,#22304,#22305,#22306,
#22307,#22308,#22309,#22310,#22311,#22312),.UNSPECIFIED.,.F.,.F.,(4,3,3,
3,3,3,3,4),(101.840787170045,102.742361511402,103.739860166852,104.737358822303,
105.734857477753,106.732356133204,107.729854788654,108.123972477225),
 .UNSPECIFIED.);
#372=B_SPLINE_CURVE_WITH_KNOTS('',3,(#22313,#22314,#22315,#22316,#22317,
#22318,#22319,#22320,#22321,#22322,#22323,#22324,#22325,#22326,#22327,#22328,
#22329,#22330,#22331,#22332,#22333,#22334),.UNSPECIFIED.,.F.,.F.,(4,3,3,
3,3,3,3,4),(-104.377348178566,-103.739860166852,-102.742361511402,-101.744862855951,
-100.747364200501,-99.7498655450501,-98.7523668895996,-98.094162871386),
 .UNSPECIFIED.);
#373=B_SPLINE_CURVE_WITH_KNOTS('',3,(#22339,#22340,#22341,#22342,#22343,
#22344,#22345,#22346,#22347,#22348,#22349,#22350,#22351,#22352,#22353,#22354,
#22355,#22356,#22357,#22358,#22359,#22360,#22361,#22362,#22363),
 .UNSPECIFIED.,.F.,.F.,(4,3,3,3,3,3,3,3,4),(95.5576018628657,95.7598709232481,
96.7573695786986,97.7548682341491,98.7523668895996,99.7498655450501,100.747364200501,
101.744862855951,101.840787170045),.UNSPECIFIED.);
#374=B_SPLINE_CURVE_WITH_KNOTS('',3,(#22364,#22365,#22366,#22367,#22368,
#22369,#22370,#22371,#22372,#22373,#22374,#22375,#22376,#22377,#22378,#22379,
#22380,#22381,#22382,#22383,#22384,#22385),.UNSPECIFIED.,.F.,.F.,(4,3,3,
3,3,3,3,4),(-98.094162871386,-97.7548682341491,-96.7573695786986,-95.7598709232481,
-94.7623722677976,-93.7648736123471,-92.7673749568966,-91.8109775642064),
 .UNSPECIFIED.);
#375=B_SPLINE_CURVE_WITH_KNOTS('',3,(#22390,#22391,#22392,#22393,#22394,
#22395,#22396,#22397,#22398,#22399,#22400,#22401,#22402,#22403,#22404,#22405,
#22406,#22407,#22408,#22409,#22410,#22411),.UNSPECIFIED.,.F.,.F.,(4,3,3,
3,3,3,3,4),(89.2744165556862,89.7748789905451,90.7723776459956,91.7698763014461,
92.7673749568966,93.7648736123471,94.7623722677976,95.5576018628657),
 .UNSPECIFIED.);
#376=B_SPLINE_CURVE_WITH_KNOTS('',3,(#22412,#22413,#22414,#22415,#22416,
#22417,#22418,#22419,#22420,#22421,#22422,#22423,#22424,#22425,#22426,#22427,
#22428,#22429,#22430,#22431,#22432,#22433,#22434,#22435,#22436),
 .UNSPECIFIED.,.F.,.F.,(4,3,3,3,3,3,3,3,4),(-91.8109775642064,-91.7698763014461,
-90.7723776459956,-89.7748789905451,-88.7773803350946,-87.7798816796441,
-86.7823830241936,-85.7848843687431,-85.5277922570269),.UNSPECIFIED.);
#377=B_SPLINE_CURVE_WITH_KNOTS('',3,(#22441,#22442,#22443,#22444,#22445,
#22446,#22447,#22448,#22449,#22450,#22451,#22452,#22453,#22454,#22455,#22456,
#22457,#22458,#22459,#22460,#22461,#22462),.UNSPECIFIED.,.F.,.F.,(4,3,3,
3,3,3,3,4),(82.9912312485066,83.7898870578421,84.7873857132926,85.7848843687431,
86.7823830241936,87.7798816796441,88.7773803350946,89.2744165556862),
 .UNSPECIFIED.);
#378=B_SPLINE_CURVE_WITH_KNOTS('',3,(#22463,#22464,#22465,#22466,#22467,
#22468,#22469,#22470,#22471,#22472,#22473,#22474,#22475,#22476,#22477,#22478,
#22479,#22480,#22481,#22482,#22483,#22484),.UNSPECIFIED.,.F.,.F.,(4,3,3,
3,3,3,3,4),(-85.5277922570269,-84.7873857132926,-83.7898870578422,-82.7923884023916,
-81.7948897469411,-80.7973910914906,-79.7998924360401,-79.2446069498473),
 .UNSPECIFIED.);
#379=B_SPLINE_CURVE_WITH_KNOTS('',3,(#22489,#22490,#22491,#22492,#22493,
#22494,#22495,#22496,#22497,#22498,#22499,#22500,#22501,#22502,#22503,#22504,
#22505,#22506,#22507,#22508,#22509,#22510,#22511,#22512,#22513),
 .UNSPECIFIED.,.F.,.F.,(4,3,3,3,3,3,3,3,4),(76.708045941327,76.8073964696886,
77.8048951251391,78.8023937805896,79.7998924360401,80.7973910914906,81.7948897469411,
82.7923884023916,82.9912312485066),.UNSPECIFIED.);
#380=B_SPLINE_CURVE_WITH_KNOTS('',3,(#22514,#22515,#22516,#22517,#22518,
#22519,#22520,#22521,#22522,#22523,#22524,#22525,#22526,#22527,#22528,#22529,
#22530,#22531,#22532,#22533,#22534,#22535),.UNSPECIFIED.,.F.,.F.,(4,3,3,
3,3,3,3,4),(-79.2446069498473,-78.8023937805896,-77.8048951251391,-76.8073964696886,
-75.8098978142381,-74.8123991587876,-73.8149005033371,-72.9614216426677),
 .UNSPECIFIED.);
#381=B_SPLINE_CURVE_WITH_KNOTS('',3,(#22540,#22541,#22542,#22543,#22544,
#22545,#22546,#22547,#22548,#22549,#22550,#22551,#22552,#22553,#22554,#22555,
#22556,#22557,#22558,#22559,#22560,#22561),.UNSPECIFIED.,.F.,.F.,(4,3,3,
3,3,3,3,4),(70.4248606341474,70.8224045369856,71.8199031924361,72.8174018478866,
73.8149005033371,74.8123991587876,75.8098978142381,76.708045941327),
 .UNSPECIFIED.);
#382=B_SPLINE_CURVE_WITH_KNOTS('',3,(#22562,#22563,#22564,#22565,#22566,
#22567,#22568,#22569,#22570,#22571,#22572,#22573,#22574,#22575,#22576,#22577,
#22578,#22579,#22580,#22581,#22582,#22583,#22584,#22585,#22586),
 .UNSPECIFIED.,.F.,.F.,(4,3,3,3,3,3,3,3,4),(-72.9614216426677,-72.8174018478866,
-71.8199031924361,-70.8224045369856,-69.8249058815351,-68.8274072260846,
-67.8299085706341,-66.8324099151836,-66.6782363354882),.UNSPECIFIED.);
#383=B_SPLINE_CURVE_WITH_KNOTS('',3,(#22591,#22592,#22593,#22594,#22595,
#22596,#22597,#22598,#22599,#22600,#22601,#22602,#22603,#22604,#22605,#22606,
#22607,#22608,#22609,#22610,#22611,#22612),.UNSPECIFIED.,.F.,.F.,(4,3,3,
3,3,3,3,4),(64.1416753269678,64.8374126042826,65.8349112597331,66.8324099151836,
67.8299085706341,68.8274072260846,69.8249058815351,70.4248606341474),
 .UNSPECIFIED.);
#384=B_SPLINE_CURVE_WITH_KNOTS('',3,(#22613,#22614,#22615,#22616,#22617,
#22618,#22619,#22620,#22621,#22622,#22623,#22624,#22625,#22626,#22627,#22628,
#22629,#22630,#22631,#22632,#22633,#22634),.UNSPECIFIED.,.F.,.F.,(4,3,3,
3,3,3,3,4),(-66.6782363354882,-65.8349112597331,-64.8374126042826,-63.8399139488321,
-62.8424152933816,-61.8449166379311,-60.8474179824806,-60.3950510283085),
 .UNSPECIFIED.);
#385=B_SPLINE_CURVE_WITH_KNOTS('',3,(#22639,#22640,#22641,#22642,#22643,
#22644,#22645,#22646,#22647,#22648,#22649,#22650,#22651,#22652,#22653,#22654,
#22655,#22656,#22657,#22658,#22659,#22660),.UNSPECIFIED.,.F.,.F.,(4,3,3,
3,3,3,3,4),(57.8584900197882,58.8524206715796,59.8499193270301,60.8474179824806,
61.8449166379311,62.8424152933816,63.8399139488321,64.1416753269678),
 .UNSPECIFIED.);
#386=B_SPLINE_CURVE_WITH_KNOTS('',3,(#22661,#22662,#22663,#22664,#22665,
#22666,#22667,#22668,#22669,#22670,#22671,#22672,#22673,#22674,#22675,#22676,
#22677,#22678,#22679,#22680,#22681,#22682),.UNSPECIFIED.,.F.,.F.,(4,3,3,
3,3,3,3,4),(-60.3950510283085,-59.8499193270301,-58.8524206715796,-57.8549220161291,
-56.8574233606786,-55.8599247052281,-54.8624260497776,-54.1118657211289),
 .UNSPECIFIED.);
#387=B_SPLINE_CURVE_WITH_KNOTS('',3,(#22687,#22688,#22689,#22690,#22691,
#22692,#22693,#22694,#22695,#22696,#22697,#22698,#22699,#22700,#22701,#22702,
#22703,#22704,#22705,#22706,#22707,#22708,#22709,#22710,#22711),
 .UNSPECIFIED.,.F.,.F.,(4,3,3,3,3,3,3,3,4),(51.5753047126086,51.8699300834261,
52.8674287388766,53.8649273943271,54.8624260497776,55.8599247052281,56.8574233606786,
57.8549220161291,57.8584900197882),.UNSPECIFIED.);
#388=B_SPLINE_CURVE_WITH_KNOTS('',3,(#22712,#22713,#22714,#22715,#22716,
#22717,#22718,#22719,#22720,#22721,#22722,#22723,#22724,#22725,#22726,#22727,
#22728,#22729,#22730,#22731,#22732,#22733,#22734,#22735,#22736),
 .UNSPECIFIED.,.F.,.F.,(4,3,3,3,3,3,3,3,4),(-54.1118657211289,-53.8649273943271,
-52.8674287388766,-51.8699300834261,-50.8724314279756,-49.8749327725251,
-48.8774341170746,-47.8799354616241,-47.8286804139493),.UNSPECIFIED.);
#389=B_SPLINE_CURVE_WITH_KNOTS('',3,(#22741,#22742,#22743,#22744,#22745,
#22746,#22747,#22748,#22749,#22750,#22751,#22752,#22753,#22754,#22755,#22756,
#22757,#22758,#22759,#22760,#22761,#22762),.UNSPECIFIED.,.F.,.F.,(4,3,3,
3,3,3,3,4),(45.292119405429,45.8849381507231,46.8824368061736,47.8799354616241,
48.8774341170746,49.8749327725251,50.8724314279756,51.5753047126086),
 .UNSPECIFIED.);
#390=B_SPLINE_CURVE_WITH_KNOTS('',3,(#22763,#22764,#22765,#22766,#22767,
#22768,#22769,#22770,#22771,#22772,#22773,#22774,#22775,#22776,#22777,#22778,
#22779,#22780,#22781,#22782,#22783,#22784),.UNSPECIFIED.,.F.,.F.,(4,3,3,
3,3,3,3,4),(-47.8286804139493,-46.8824368061736,-45.8849381507231,-44.8874394952726,
-43.8899408398221,-42.8924421843716,-41.8949435289211,-41.5454951067697),
 .UNSPECIFIED.);
#391=B_SPLINE_CURVE_WITH_KNOTS('',3,(#22789,#22790,#22791,#22792,#22793,
#22794,#22795,#22796,#22797,#22798,#22799,#22800,#22801,#22802,#22803,#22804,
#22805,#22806,#22807,#22808,#22809,#22810),.UNSPECIFIED.,.F.,.F.,(4,3,3,
3,3,3,3,4),(39.0089340982494,39.8999462180201,40.8974448734706,41.8949435289211,
42.8924421843716,43.8899408398221,44.8874394952726,45.292119405429),
 .UNSPECIFIED.);
#392=B_SPLINE_CURVE_WITH_KNOTS('',3,(#22811,#22812,#22813,#22814,#22815,
#22816,#22817,#22818,#22819,#22820,#22821,#22822,#22823,#22824,#22825,#22826,
#22827,#22828,#22829,#22830,#22831,#22832),.UNSPECIFIED.,.F.,.F.,(4,3,3,
3,3,3,3,4),(-41.5454951067697,-40.8974448734706,-39.8999462180201,-38.9024475625696,
-37.9049489071191,-36.9074502516685,-35.909951596218,-35.2623097995902),
 .UNSPECIFIED.);
#393=B_SPLINE_CURVE_WITH_KNOTS('',3,(#22837,#22838,#22839,#22840,#22841,
#22842,#22843,#22844,#22845,#22846,#22847,#22848,#22849,#22850,#22851,#22852,
#22853,#22854,#22855,#22856,#22857,#22858,#22859,#22860,#22861),
 .UNSPECIFIED.,.F.,.F.,(4,3,3,3,3,3,3,3,4),(32.7257487910699,32.9174556298666,
33.9149542853171,34.9124529407676,35.9099515962181,36.9074502516685,37.9049489071191,
38.9024475625696,39.0089340982494),.UNSPECIFIED.);
#394=B_SPLINE_CURVE_WITH_KNOTS('',3,(#22862,#22863,#22864,#22865,#22866,
#22867,#22868,#22869,#22870,#22871,#22872,#22873,#22874,#22875,#22876,#22877,
#22878,#22879,#22880,#22881,#22882,#22883),.UNSPECIFIED.,.F.,.F.,(4,3,3,
3,3,3,3,4),(-35.2623097995902,-34.9124529407676,-33.9149542853171,-32.9174556298665,
-31.919956974416,-30.9224583189655,-29.9249596635151,-28.9791244924106),
 .UNSPECIFIED.);
#395=B_SPLINE_CURVE_WITH_KNOTS('',3,(#22888,#22889,#22890,#22891,#22892,
#22893,#22894,#22895,#22896,#22897,#22898,#22899,#22900,#22901,#22902,#22903,
#22904,#22905,#22906,#22907,#22908,#22909),.UNSPECIFIED.,.F.,.F.,(4,3,3,
3,3,3,3,4),(26.4425634838902,26.9324636971635,27.929962352614,28.9274610080645,
29.924959663515,30.9224583189655,31.9199569744161,32.7257487910699),
 .UNSPECIFIED.);
#396=B_SPLINE_CURVE_WITH_KNOTS('',3,(#22910,#22911,#22912,#22913,#22914,
#22915,#22916,#22917,#22918,#22919,#22920,#22921,#22922,#22923,#22924,#22925,
#22926,#22927,#22928,#22929,#22930,#22931,#22932,#22933,#22934),
 .UNSPECIFIED.,.F.,.F.,(4,3,3,3,3,3,3,3,4),(-28.9791244924106,-28.9274610080645,
-27.929962352614,-26.9324636971635,-25.934965041713,-24.9374663862625,-23.939967730812,
-22.9424690753615,-22.6959391852309),.UNSPECIFIED.);
#397=B_SPLINE_CURVE_WITH_KNOTS('',3,(#22939,#22940,#22941,#22942,#22943,
#22944,#22945,#22946,#22947,#22948,#22949,#22950,#22951,#22952,#22953,#22954,
#22955,#22956,#22957,#22958,#22959,#22960),.UNSPECIFIED.,.F.,.F.,(4,3,3,
3,3,3,3,4),(20.1593781767106,20.9474717644605,21.944970419911,22.9424690753615,
23.939967730812,24.9374663862625,25.934965041713,26.4425634838902),
 .UNSPECIFIED.);
#398=B_SPLINE_CURVE_WITH_KNOTS('',3,(#22961,#22962,#22963,#22964,#22965,
#22966,#22967,#22968,#22969,#22970,#22971,#22972,#22973,#22974,#22975,#22976,
#22977,#22978,#22979,#22980,#22981,#22982),.UNSPECIFIED.,.F.,.F.,(4,3,3,
3,3,3,3,4),(-22.6959391852309,-21.944970419911,-20.9474717644605,-19.94997310901,
-18.9524744535595,-17.954975798109,-16.9574771426585,-16.4127538780514),
 .UNSPECIFIED.);
#399=B_SPLINE_CURVE_WITH_KNOTS('',3,(#22987,#22988,#22989,#22990,#22991,
#22992,#22993,#22994,#22995,#22996,#22997,#22998,#22999,#23000,#23001,#23002,
#23003,#23004,#23005,#23006,#23007,#23008,#23009,#23010,#23011),
 .UNSPECIFIED.,.F.,.F.,(4,3,3,3,3,3,3,3,4),(13.8761928695311,13.964981176307,
14.9624798317575,15.959978487208,16.9574771426585,17.954975798109,18.9524744535595,
19.94997310901,20.1593781767106),.UNSPECIFIED.);
#400=B_SPLINE_CURVE_WITH_KNOTS('',3,(#23012,#23013,#23014,#23015,#23016,
#23017,#23018,#23019,#23020,#23021,#23022,#23023,#23024,#23025,#23026,#23027,
#23028,#23029,#23030,#23031,#23032,#23033),.UNSPECIFIED.,.F.,.F.,(4,3,3,
3,3,3,3,4),(-16.4127538780514,-15.959978487208,-14.9624798317575,-13.964981176307,
-12.9674825208565,-11.969983865406,-10.9724852099555,-10.1295685708718),
 .UNSPECIFIED.);
#401=B_SPLINE_CURVE_WITH_KNOTS('',3,(#23039,#23040,#23041,#23042,#23043,
#23044,#23045,#23046,#23047,#23048,#23049,#23050,#23051),.UNSPECIFIED.,
 .F.,.F.,(4,3,3,3,4),(-3.84638326369218,-2.9924959663515,-1.994997310901,
-0.997498655450501,0.),.UNSPECIFIED.);
#402=B_SPLINE_CURVE_WITH_KNOTS('',3,(#23054,#23055,#23056,#23057,#23058,
#23059,#23060,#23061,#23062,#23063,#23064,#23065,#23066,#23067,#23068,#23069,
#23070,#23071,#23072),.UNSPECIFIED.,.F.,.F.,(4,3,3,3,3,3,4),(2.01461286527449,
2.99249596635151,3.98999462180201,4.98749327725251,5.98499193270301,6.98249058815351,
7.59300756235149),.UNSPECIFIED.);
#403=B_SPLINE_CURVE_WITH_KNOTS('',3,(#23078,#23079,#23080,#23081,#23082),
 .UNSPECIFIED.,.F.,.F.,(4,1,4),(128.805298797182,129.566421347416,130.563920002866),
 .UNSPECIFIED.);
#404=B_SPLINE_CURVE_WITH_KNOTS('',3,(#23085,#23086,#23087,#23088,#23089,
#23090),.UNSPECIFIED.,.F.,.F.,(4,1,1,4),(128.805298797182,129.110486389585,
130.107985045035,131.085868146112),.UNSPECIFIED.);
#405=B_SPLINE_CURVE_WITH_KNOTS('',3,(#23095,#23096,#23097,#23098,#23099,
#23100,#23101,#23102,#23103,#23104,#23105),.UNSPECIFIED.,.F.,.F.,(4,1,1,
1,1,1,1,1,4),(122.522113490002,122.583930759262,123.581429414713,124.578928070163,
125.576426725614,126.573925381064,127.571424036515,128.568922691965,128.805298797182),
 .UNSPECIFIED.);
#406=B_SPLINE_CURVE_WITH_KNOTS('',3,(#23106,#23107,#23108,#23109,#23110,
#23111,#23112,#23113,#23114,#23115),.UNSPECIFIED.,.F.,.F.,(4,1,1,1,1,1,
1,4),(122.522113490002,123.125494456882,124.122993112332,125.120491767783,
126.117990423233,127.115489078684,128.112987734134,128.805298797182),
 .UNSPECIFIED.);
#407=B_SPLINE_CURVE_WITH_KNOTS('',3,(#23120,#23121,#23122,#23123,#23124,
#23125,#23126,#23127,#23128,#23129),.UNSPECIFIED.,.F.,.F.,(4,1,1,1,1,1,
1,4),(116.238928182822,116.598938826559,117.59643748201,118.59393613746,
119.591434792911,120.588933448361,121.586432103812,122.522113490002),
 .UNSPECIFIED.);
#408=B_SPLINE_CURVE_WITH_KNOTS('',3,(#23130,#23131,#23132,#23133,#23134,
#23135,#23136,#23137,#23138,#23139),.UNSPECIFIED.,.F.,.F.,(4,1,1,1,1,1,
1,4),(116.238928182822,117.140502524179,118.138001179629,119.13549983508,
120.13299849053,121.130497145981,122.127995801431,122.522113490002),
 .UNSPECIFIED.);
#409=B_SPLINE_CURVE_WITH_KNOTS('',3,(#23144,#23145,#23146,#23147,#23148,
#23149,#23150,#23151,#23152,#23153),.UNSPECIFIED.,.F.,.F.,(4,1,1,1,1,1,
1,4),(109.955742875643,110.613946893856,111.611445549307,112.608944204757,
113.606442860208,114.603941515658,115.601440171109,116.238928182822),
 .UNSPECIFIED.);
#410=B_SPLINE_CURVE_WITH_KNOTS('',3,(#23154,#23155,#23156,#23157,#23158,
#23159,#23160,#23161,#23162,#23163,#23164),.UNSPECIFIED.,.F.,.F.,(4,1,1,
1,1,1,1,1,4),(109.955742875643,110.158011936025,111.155510591476,112.153009246926,
113.150507902377,114.148006557827,115.145505213278,116.143003868728,116.238928182822),
 .UNSPECIFIED.);
#411=B_SPLINE_CURVE_WITH_KNOTS('',3,(#23169,#23170,#23171,#23172,#23173,
#23174,#23175,#23176,#23177,#23178),.UNSPECIFIED.,.F.,.F.,(4,1,1,1,1,1,
1,4),(103.672557568463,104.628954961153,105.626453616604,106.623952272054,
107.621450927505,108.618949582955,109.616448238406,109.955742875643),
 .UNSPECIFIED.);
#412=B_SPLINE_CURVE_WITH_KNOTS('',3,(#23179,#23180,#23181,#23182,#23183,
#23184,#23185,#23186,#23187,#23188),.UNSPECIFIED.,.F.,.F.,(4,1,1,1,1,1,
1,4),(103.672557568463,104.173020003322,105.170518658772,106.168017314223,
107.165515969673,108.163014625124,109.160513280574,109.955742875643),
 .UNSPECIFIED.);
#413=B_SPLINE_CURVE_WITH_KNOTS('',3,(#23193,#23194,#23195,#23196,#23197,
#23198,#23199,#23200,#23201,#23202,#23203),.UNSPECIFIED.,.F.,.F.,(4,1,1,
1,1,1,1,1,4),(97.3893722612835,97.6464643729998,98.6439630284503,99.6414616839008,
100.638960339351,101.636458994802,102.633957650252,103.631456305703,103.672557568463),
 .UNSPECIFIED.);
#414=B_SPLINE_CURVE_WITH_KNOTS('',3,(#23204,#23205,#23206,#23207,#23208,
#23209,#23210,#23211,#23212,#23213),.UNSPECIFIED.,.F.,.F.,(4,1,1,1,1,1,
1,4),(97.3893722612835,98.188028070619,99.1855267260695,100.18302538152,
101.18052403697,102.178022692421,103.175521347871,103.672557568463),
 .UNSPECIFIED.);
#415=B_SPLINE_CURVE_WITH_KNOTS('',3,(#23218,#23219,#23220,#23221,#23222,
#23223,#23224,#23225,#23226,#23227),.UNSPECIFIED.,.F.,.F.,(4,1,1,1,1,1,
1,4),(91.1061869541039,91.6614724402968,92.6589710957473,93.6564697511978,
94.6539684066483,95.6514670620988,96.6489657175493,97.3893722612835),
 .UNSPECIFIED.);
#416=B_SPLINE_CURVE_WITH_KNOTS('',3,(#23228,#23229,#23230,#23231,#23232,
#23233,#23234,#23235,#23236,#23237,#23238),.UNSPECIFIED.,.F.,.F.,(4,1,1,
1,1,1,1,1,4),(91.106186954104,91.2055374824655,92.203036137916,93.2005347933665,
94.198033448817,95.1955321042675,96.193030759718,97.1905294151685,97.3893722612835),
 .UNSPECIFIED.);
#417=B_SPLINE_CURVE_WITH_KNOTS('',3,(#23243,#23244,#23245,#23246,#23247,
#23248,#23249,#23250,#23251,#23252),.UNSPECIFIED.,.F.,.F.,(4,1,1,1,1,1,
1,4),(84.8230016469243,85.6764805075938,86.6739791630443,87.6714778184948,
88.6689764739453,89.6664751293958,90.6639737848463,91.1061869541039),
 .UNSPECIFIED.);
#418=B_SPLINE_CURVE_WITH_KNOTS('',3,(#23253,#23254,#23255,#23256,#23257,
#23258,#23259,#23260,#23261,#23262),.UNSPECIFIED.,.F.,.F.,(4,1,1,1,1,1,
1,4),(84.8230016469244,85.2205455497625,86.218044205213,87.2155428606635,
88.213041516114,89.2105401715645,90.208038827015,91.106186954104),
 .UNSPECIFIED.);
#419=B_SPLINE_CURVE_WITH_KNOTS('',3,(#23267,#23268,#23269,#23270,#23271,
#23272,#23273,#23274,#23275,#23276,#23277),.UNSPECIFIED.,.F.,.F.,(4,1,1,
1,1,1,1,1,4),(78.5398163397448,78.6939899194402,79.6914885748908,80.6889872303413,
81.6864858857918,82.6839845412423,83.6814831966928,84.6789818521433,84.8230016469243),
 .UNSPECIFIED.);
#420=B_SPLINE_CURVE_WITH_KNOTS('',3,(#23278,#23279,#23280,#23281,#23282,
#23283,#23284,#23285,#23286,#23287),.UNSPECIFIED.,.F.,.F.,(4,1,1,1,1,1,
1,4),(78.5398163397448,79.2355536170595,80.23305227251,81.2305509279605,
82.228049583411,83.2255482388615,84.223046894312,84.8230016469244),
 .UNSPECIFIED.);
#421=B_SPLINE_CURVE_WITH_KNOTS('',3,(#23292,#23293,#23294,#23295,#23296,
#23297,#23298,#23299,#23300,#23301),.UNSPECIFIED.,.F.,.F.,(4,1,1,1,1,1,
1,4),(72.2566310325652,72.7089979867372,73.7064966421877,74.7039952976382,
75.7014939530887,76.6989926085392,77.6964912639897,78.5398163397448),
 .UNSPECIFIED.);
#422=B_SPLINE_CURVE_WITH_KNOTS('',3,(#23302,#23303,#23304,#23305,#23306,
#23307,#23308,#23309,#23310,#23311),.UNSPECIFIED.,.F.,.F.,(4,1,1,1,1,1,
1,4),(72.2566310325652,73.2505616843565,74.248060339807,75.2455589952575,
76.243057650708,77.2405563061585,78.238054961609,78.5398163397448),
 .UNSPECIFIED.);
#423=B_SPLINE_CURVE_WITH_KNOTS('',3,(#23316,#23317,#23318,#23319,#23320,
#23321,#23322,#23323,#23324,#23325),.UNSPECIFIED.,.F.,.F.,(4,1,1,1,1,1,
1,4),(65.9734457253856,66.7240060540342,67.7215047094847,68.7190033649352,
69.7165020203857,70.7140006758362,71.7114993312867,72.2566310325652),
 .UNSPECIFIED.);
#424=B_SPLINE_CURVE_WITH_KNOTS('',3,(#23326,#23327,#23328,#23329,#23330,
#23331,#23332,#23333,#23334,#23335,#23336),.UNSPECIFIED.,.F.,.F.,(4,1,1,
1,1,1,1,1,4),(65.9734457253856,66.2680710962029,67.2655697516534,68.2630684071039,
69.2605670625544,70.2580657180049,71.2555643734554,72.2530630289059,72.2566310325652),
 .UNSPECIFIED.);
#425=B_SPLINE_CURVE_WITH_KNOTS('',3,(#23341,#23342,#23343,#23344,#23345,
#23346,#23347,#23348,#23349,#23350,#23351),.UNSPECIFIED.,.F.,.F.,(4,1,1,
1,1,1,1,1,4),(59.690260418206,59.7415154658807,60.7390141213312,61.7365127767817,
62.7340114322322,63.7315100876827,64.7290087431332,65.7265073985837,65.9734457253856),
 .UNSPECIFIED.);
#426=B_SPLINE_CURVE_WITH_KNOTS('',3,(#23352,#23353,#23354,#23355,#23356,
#23357,#23358,#23359,#23360,#23361),.UNSPECIFIED.,.F.,.F.,(4,1,1,1,1,1,
1,4),(59.690260418206,60.2830791634999,61.2805778189504,62.2780764744009,
63.2755751298514,64.2730737853019,65.2705724407524,65.9734457253856),
 .UNSPECIFIED.);
#427=B_SPLINE_CURVE_WITH_KNOTS('',3,(#23366,#23367,#23368,#23369,#23370,
#23371,#23372,#23373,#23374,#23375),.UNSPECIFIED.,.F.,.F.,(4,1,1,1,1,1,
1,4),(53.4070751110263,53.7565235331777,54.7540221886282,55.7515208440787,
56.7490194995292,57.7465181549797,58.7440168104302,59.690260418206),
 .UNSPECIFIED.);
#428=B_SPLINE_CURVE_WITH_KNOTS('',3,(#23376,#23377,#23378,#23379,#23380,
#23381,#23382,#23383,#23384,#23385),.UNSPECIFIED.,.F.,.F.,(4,1,1,1,1,1,
1,4),(53.4070751110264,54.2980872307969,55.2955858862474,56.2930845416979,
57.2905831971484,58.2880818525989,59.2855805080494,59.690260418206),
 .UNSPECIFIED.);
#429=B_SPLINE_CURVE_WITH_KNOTS('',3,(#23390,#23391,#23392,#23393,#23394,
#23395,#23396,#23397,#23398,#23399),.UNSPECIFIED.,.F.,.F.,(4,1,1,1,1,1,
1,4),(47.1238898038468,47.7715316004747,48.7690302559252,49.7665289113757,
50.7640275668262,51.7615262222767,52.7590248777272,53.4070751110263),
 .UNSPECIFIED.);
#430=B_SPLINE_CURVE_WITH_KNOTS('',3,(#23400,#23401,#23402,#23403,#23404,
#23405,#23406,#23407,#23408,#23409,#23410),.UNSPECIFIED.,.F.,.F.,(4,1,1,
1,1,1,1,1,4),(47.1238898038468,47.3155966426434,48.3130952980939,49.3105939535444,
50.3080926089949,51.3055912644454,52.3030899198959,53.3005885753464,53.4070751110264),
 .UNSPECIFIED.);
#431=B_SPLINE_CURVE_WITH_KNOTS('',3,(#23415,#23416,#23417,#23418,#23419,
#23420,#23421,#23422,#23423,#23424),.UNSPECIFIED.,.F.,.F.,(4,1,1,1,1,1,
1,4),(40.8407044966672,41.7865396677717,42.7840383232222,43.7815369786727,
44.7790356341232,45.7765342895737,46.7740329450242,47.1238898038468),
 .UNSPECIFIED.);
#432=B_SPLINE_CURVE_WITH_KNOTS('',3,(#23425,#23426,#23427,#23428,#23429,
#23430,#23431,#23432,#23433,#23434),.UNSPECIFIED.,.F.,.F.,(4,1,1,1,1,1,
1,4),(40.8407044966672,41.3306047099404,42.3281033653909,43.3256020208414,
44.3231006762919,45.3205993317424,46.3180979871929,47.1238898038468),
 .UNSPECIFIED.);
#433=B_SPLINE_CURVE_WITH_KNOTS('',3,(#23439,#23440,#23441,#23442,#23443,
#23444,#23445,#23446,#23447,#23448,#23449),.UNSPECIFIED.,.F.,.F.,(4,1,1,
1,1,1,1,1,4),(34.5575191894876,34.8040490796182,35.8015477350687,36.7990463905192,
37.7965450459697,38.7940437014202,39.7915423568707,40.7890410123212,40.8407044966672),
 .UNSPECIFIED.);
#434=B_SPLINE_CURVE_WITH_KNOTS('',3,(#23450,#23451,#23452,#23453,#23454,
#23455,#23456,#23457,#23458,#23459),.UNSPECIFIED.,.F.,.F.,(4,1,1,1,1,1,
1,4),(34.5575191894877,35.3456127772374,36.3431114326879,37.3406100881384,
38.3381087435889,39.3356073990394,40.3331060544899,40.8407044966672),
 .UNSPECIFIED.);
#435=B_SPLINE_CURVE_WITH_KNOTS('',3,(#23464,#23465,#23466,#23467,#23468,
#23469,#23470,#23471,#23472,#23473),.UNSPECIFIED.,.F.,.F.,(4,1,1,1,1,1,
1,4),(28.2743338823081,28.8190571469152,29.8165558023657,30.8140544578162,
31.8115531132667,32.8090517687172,33.8065504241677,34.5575191894876),
 .UNSPECIFIED.);
#436=B_SPLINE_CURVE_WITH_KNOTS('',3,(#23474,#23475,#23476,#23477,#23478,
#23479,#23480,#23481,#23482,#23483,#23484),.UNSPECIFIED.,.F.,.F.,(4,1,1,
1,1,1,1,1,4),(28.2743338823081,28.3631221890839,29.3606208445344,30.3581194999849,
31.3556181554354,32.3531168108859,33.3506154663364,34.3481141217869,34.5575191894877),
 .UNSPECIFIED.);
#437=B_SPLINE_CURVE_WITH_KNOTS('',3,(#23489,#23490,#23491,#23492,#23493,
#23494,#23495,#23496,#23497,#23498),.UNSPECIFIED.,.F.,.F.,(4,1,1,1,1,1,
1,4),(21.9911485751284,22.8340652142122,23.8315638696627,24.8290625251132,
25.8265611805637,26.8240598360142,27.8215584914647,28.2743338823081),
 .UNSPECIFIED.);
#438=B_SPLINE_CURVE_WITH_KNOTS('',3,(#23499,#23500,#23501,#23502,#23503,
#23504,#23505,#23506,#23507,#23508),.UNSPECIFIED.,.F.,.F.,(4,1,1,1,1,1,
1,4),(21.9911485751284,22.3781302563809,23.3756289118314,24.3731275672819,
25.3706262227324,26.3681248781829,27.3656235336334,28.2743338823081),
 .UNSPECIFIED.);
#439=B_SPLINE_CURVE_WITH_KNOTS('',3,(#23514,#23515,#23516,#23517,#23518),
 .UNSPECIFIED.,.F.,.F.,(4,1,4),(14.3981410127769,15.3956396682274,15.7079632679489),
 .UNSPECIFIED.);
#440=B_SPLINE_CURVE_WITH_KNOTS('',3,(#23521,#23522,#23523,#23524,#23525),
 .UNSPECIFIED.,.F.,.F.,(4,1,4),(13.8761928695311,14.8540759706082,15.7079632679488),
 .UNSPECIFIED.);
#441=B_SPLINE_CURVE_WITH_KNOTS('',3,(#23531,#23532,#23533,#23534,#23535,
#23536,#23537,#23538,#23539,#23540,#23541,#23542,#23543,#23544,#23545,#23546),
 .UNSPECIFIED.,.F.,.F.,(4,3,3,3,3,4),(114.407157784405,114.712345376808,
115.709844032258,116.707342687709,117.704841343159,118.70233999861),
 .UNSPECIFIED.);
#442=B_SPLINE_CURVE_WITH_KNOTS('',3,(#23554,#23555,#23556,#23557,#23558,
#23559,#23560,#23561,#23562,#23563,#23564,#23565,#23566,#23567,#23568,#23569,
#23570,#23571,#23572,#23573,#23574,#23575),.UNSPECIFIED.,.F.,.F.,(4,3,3,
3,3,3,3,4),(-116.687727133335,-115.709844032258,-114.712345376808,-113.714846721357,
-112.717348065907,-111.719849410456,-110.722350755006,-110.660533485745),
 .UNSPECIFIED.);
#443=B_SPLINE_CURVE_WITH_KNOTS('',3,(#23580,#23581,#23582,#23583,#23584,
#23585,#23586,#23587,#23588,#23589,#23590,#23591,#23592,#23593,#23594,#23595,
#23596,#23597,#23598,#23599,#23600,#23601),.UNSPECIFIED.,.F.,.F.,(4,3,3,
3,3,3,3,4),(108.123972477225,108.727353444105,109.724852099555,110.722350755006,
111.719849410456,112.717348065907,113.714846721357,114.407157784405),
 .UNSPECIFIED.);
#444=B_SPLINE_CURVE_WITH_KNOTS('',3,(#23602,#23603,#23604,#23605,#23606,
#23607,#23608,#23609,#23610,#23611,#23612,#23613,#23614,#23615,#23616,#23617,
#23618,#23619,#23620,#23621,#23622,#23623),.UNSPECIFIED.,.F.,.F.,(4,3,3,
3,3,3,3,4),(-110.660533485745,-109.724852099555,-108.727353444105,-107.729854788654,
-106.732356133204,-105.734857477753,-104.737358822303,-104.377348178566),
 .UNSPECIFIED.);
#445=B_SPLINE_CURVE_WITH_KNOTS('',3,(#23628,#23629,#23630,#23631,#23632,
#23633,#23634,#23635,#23636,#23637,#23638,#23639,#23640,#23641,#23642,#23643,
#23644,#23645,#23646,#23647,#23648,#23649),.UNSPECIFIED.,.F.,.F.,(4,3,3,
3,3,3,3,4),(101.840787170045,102.742361511402,103.739860166852,104.737358822303,
105.734857477753,106.732356133204,107.729854788654,108.123972477225),
 .UNSPECIFIED.);
#446=B_SPLINE_CURVE_WITH_KNOTS('',3,(#23650,#23651,#23652,#23653,#23654,
#23655,#23656,#23657,#23658,#23659,#23660,#23661,#23662,#23663,#23664,#23665,
#23666,#23667,#23668,#23669,#23670,#23671),.UNSPECIFIED.,.F.,.F.,(4,3,3,
3,3,3,3,4),(-104.377348178566,-103.739860166852,-102.742361511402,-101.744862855951,
-100.747364200501,-99.7498655450501,-98.7523668895996,-98.094162871386),
 .UNSPECIFIED.);
#447=B_SPLINE_CURVE_WITH_KNOTS('',3,(#23676,#23677,#23678,#23679,#23680,
#23681,#23682,#23683,#23684,#23685,#23686,#23687,#23688,#23689,#23690,#23691,
#23692,#23693,#23694,#23695,#23696,#23697,#23698,#23699,#23700),
 .UNSPECIFIED.,.F.,.F.,(4,3,3,3,3,3,3,3,4),(95.5576018628657,95.7598709232481,
96.7573695786986,97.7548682341491,98.7523668895996,99.7498655450501,100.747364200501,
101.744862855951,101.840787170045),.UNSPECIFIED.);
#448=B_SPLINE_CURVE_WITH_KNOTS('',3,(#23701,#23702,#23703,#23704,#23705,
#23706,#23707,#23708,#23709,#23710,#23711,#23712,#23713,#23714,#23715,#23716,
#23717,#23718,#23719,#23720,#23721,#23722),.UNSPECIFIED.,.F.,.F.,(4,3,3,
3,3,3,3,4),(-98.094162871386,-97.7548682341491,-96.7573695786986,-95.7598709232481,
-94.7623722677976,-93.7648736123471,-92.7673749568966,-91.8109775642064),
 .UNSPECIFIED.);
#449=B_SPLINE_CURVE_WITH_KNOTS('',3,(#23727,#23728,#23729,#23730,#23731,
#23732,#23733,#23734,#23735,#23736,#23737,#23738,#23739,#23740,#23741,#23742,
#23743,#23744,#23745,#23746,#23747,#23748),.UNSPECIFIED.,.F.,.F.,(4,3,3,
3,3,3,3,4),(89.2744165556862,89.7748789905451,90.7723776459956,91.7698763014461,
92.7673749568966,93.7648736123471,94.7623722677976,95.5576018628657),
 .UNSPECIFIED.);
#450=B_SPLINE_CURVE_WITH_KNOTS('',3,(#23749,#23750,#23751,#23752,#23753,
#23754,#23755,#23756,#23757,#23758,#23759,#23760,#23761,#23762,#23763,#23764,
#23765,#23766,#23767,#23768,#23769,#23770,#23771,#23772,#23773),
 .UNSPECIFIED.,.F.,.F.,(4,3,3,3,3,3,3,3,4),(-91.8109775642064,-91.7698763014461,
-90.7723776459956,-89.7748789905451,-88.7773803350946,-87.7798816796441,
-86.7823830241936,-85.7848843687431,-85.5277922570269),.UNSPECIFIED.);
#451=B_SPLINE_CURVE_WITH_KNOTS('',3,(#23778,#23779,#23780,#23781,#23782,
#23783,#23784,#23785,#23786,#23787,#23788,#23789,#23790,#23791,#23792,#23793,
#23794,#23795,#23796,#23797,#23798,#23799),.UNSPECIFIED.,.F.,.F.,(4,3,3,
3,3,3,3,4),(82.9912312485066,83.7898870578421,84.7873857132926,85.7848843687431,
86.7823830241936,87.7798816796441,88.7773803350946,89.2744165556862),
 .UNSPECIFIED.);
#452=B_SPLINE_CURVE_WITH_KNOTS('',3,(#23800,#23801,#23802,#23803,#23804,
#23805,#23806,#23807,#23808,#23809,#23810,#23811,#23812,#23813,#23814,#23815,
#23816,#23817,#23818,#23819,#23820,#23821),.UNSPECIFIED.,.F.,.F.,(4,3,3,
3,3,3,3,4),(-85.5277922570269,-84.7873857132926,-83.7898870578422,-82.7923884023916,
-81.7948897469411,-80.7973910914906,-79.7998924360401,-79.2446069498473),
 .UNSPECIFIED.);
#453=B_SPLINE_CURVE_WITH_KNOTS('',3,(#23826,#23827,#23828,#23829,#23830,
#23831,#23832,#23833,#23834,#23835,#23836,#23837,#23838,#23839,#23840,#23841,
#23842,#23843,#23844,#23845,#23846,#23847,#23848,#23849,#23850),
 .UNSPECIFIED.,.F.,.F.,(4,3,3,3,3,3,3,3,4),(76.708045941327,76.8073964696886,
77.8048951251391,78.8023937805896,79.7998924360401,80.7973910914906,81.7948897469411,
82.7923884023916,82.9912312485066),.UNSPECIFIED.);
#454=B_SPLINE_CURVE_WITH_KNOTS('',3,(#23851,#23852,#23853,#23854,#23855,
#23856,#23857,#23858,#23859,#23860,#23861,#23862,#23863,#23864,#23865,#23866,
#23867,#23868,#23869,#23870,#23871,#23872),.UNSPECIFIED.,.F.,.F.,(4,3,3,
3,3,3,3,4),(-79.2446069498473,-78.8023937805896,-77.8048951251391,-76.8073964696886,
-75.8098978142381,-74.8123991587876,-73.8149005033371,-72.9614216426677),
 .UNSPECIFIED.);
#455=B_SPLINE_CURVE_WITH_KNOTS('',3,(#23877,#23878,#23879,#23880,#23881,
#23882,#23883,#23884,#23885,#23886,#23887,#23888,#23889,#23890,#23891,#23892,
#23893,#23894,#23895,#23896,#23897,#23898),.UNSPECIFIED.,.F.,.F.,(4,3,3,
3,3,3,3,4),(70.4248606341474,70.8224045369856,71.8199031924361,72.8174018478866,
73.8149005033371,74.8123991587876,75.8098978142381,76.708045941327),
 .UNSPECIFIED.);
#456=B_SPLINE_CURVE_WITH_KNOTS('',3,(#23899,#23900,#23901,#23902,#23903,
#23904,#23905,#23906,#23907,#23908,#23909,#23910,#23911,#23912,#23913,#23914,
#23915,#23916,#23917,#23918,#23919,#23920,#23921,#23922,#23923),
 .UNSPECIFIED.,.F.,.F.,(4,3,3,3,3,3,3,3,4),(-72.9614216426677,-72.8174018478866,
-71.8199031924361,-70.8224045369856,-69.8249058815351,-68.8274072260846,
-67.8299085706341,-66.8324099151836,-66.6782363354882),.UNSPECIFIED.);
#457=B_SPLINE_CURVE_WITH_KNOTS('',3,(#23928,#23929,#23930,#23931,#23932,
#23933,#23934,#23935,#23936,#23937,#23938,#23939,#23940,#23941,#23942,#23943,
#23944,#23945,#23946,#23947,#23948,#23949),.UNSPECIFIED.,.F.,.F.,(4,3,3,
3,3,3,3,4),(64.1416753269678,64.8374126042826,65.8349112597331,66.8324099151836,
67.8299085706341,68.8274072260846,69.8249058815351,70.4248606341474),
 .UNSPECIFIED.);
#458=B_SPLINE_CURVE_WITH_KNOTS('',3,(#23950,#23951,#23952,#23953,#23954,
#23955,#23956,#23957,#23958,#23959,#23960,#23961,#23962,#23963,#23964,#23965,
#23966,#23967,#23968,#23969,#23970,#23971),.UNSPECIFIED.,.F.,.F.,(4,3,3,
3,3,3,3,4),(-66.6782363354882,-65.8349112597331,-64.8374126042826,-63.8399139488321,
-62.8424152933816,-61.8449166379311,-60.8474179824806,-60.3950510283085),
 .UNSPECIFIED.);
#459=B_SPLINE_CURVE_WITH_KNOTS('',3,(#23976,#23977,#23978,#23979,#23980,
#23981,#23982,#23983,#23984,#23985,#23986,#23987,#23988,#23989,#23990,#23991,
#23992,#23993,#23994,#23995,#23996,#23997),.UNSPECIFIED.,.F.,.F.,(4,3,3,
3,3,3,3,4),(57.8584900197882,58.8524206715796,59.8499193270301,60.8474179824806,
61.8449166379311,62.8424152933816,63.8399139488321,64.1416753269678),
 .UNSPECIFIED.);
#460=B_SPLINE_CURVE_WITH_KNOTS('',3,(#23998,#23999,#24000,#24001,#24002,
#24003,#24004,#24005,#24006,#24007,#24008,#24009,#24010,#24011,#24012,#24013,
#24014,#24015,#24016,#24017,#24018,#24019),.UNSPECIFIED.,.F.,.F.,(4,3,3,
3,3,3,3,4),(-60.3950510283085,-59.8499193270301,-58.8524206715796,-57.8549220161291,
-56.8574233606786,-55.8599247052281,-54.8624260497776,-54.1118657211289),
 .UNSPECIFIED.);
#461=B_SPLINE_CURVE_WITH_KNOTS('',3,(#24024,#24025,#24026,#24027,#24028,
#24029,#24030,#24031,#24032,#24033,#24034,#24035,#24036,#24037,#24038,#24039,
#24040,#24041,#24042,#24043,#24044,#24045,#24046,#24047,#24048),
 .UNSPECIFIED.,.F.,.F.,(4,3,3,3,3,3,3,3,4),(51.5753047126086,51.8699300834261,
52.8674287388766,53.8649273943271,54.8624260497776,55.8599247052281,56.8574233606786,
57.8549220161291,57.8584900197882),.UNSPECIFIED.);
#462=B_SPLINE_CURVE_WITH_KNOTS('',3,(#24049,#24050,#24051,#24052,#24053,
#24054,#24055,#24056,#24057,#24058,#24059,#24060,#24061,#24062,#24063,#24064,
#24065,#24066,#24067,#24068,#24069,#24070,#24071,#24072,#24073),
 .UNSPECIFIED.,.F.,.F.,(4,3,3,3,3,3,3,3,4),(-54.1118657211289,-53.8649273943271,
-52.8674287388766,-51.8699300834261,-50.8724314279756,-49.8749327725251,
-48.8774341170746,-47.8799354616241,-47.8286804139493),.UNSPECIFIED.);
#463=B_SPLINE_CURVE_WITH_KNOTS('',3,(#24078,#24079,#24080,#24081,#24082,
#24083,#24084,#24085,#24086,#24087,#24088,#24089,#24090,#24091,#24092,#24093,
#24094,#24095,#24096,#24097,#24098,#24099),.UNSPECIFIED.,.F.,.F.,(4,3,3,
3,3,3,3,4),(45.292119405429,45.8849381507231,46.8824368061736,47.8799354616241,
48.8774341170746,49.8749327725251,50.8724314279756,51.5753047126086),
 .UNSPECIFIED.);
#464=B_SPLINE_CURVE_WITH_KNOTS('',3,(#24100,#24101,#24102,#24103,#24104,
#24105,#24106,#24107,#24108,#24109,#24110,#24111,#24112,#24113,#24114,#24115,
#24116,#24117,#24118,#24119,#24120,#24121),.UNSPECIFIED.,.F.,.F.,(4,3,3,
3,3,3,3,4),(-47.8286804139493,-46.8824368061736,-45.8849381507231,-44.8874394952726,
-43.8899408398221,-42.8924421843716,-41.8949435289211,-41.5454951067697),
 .UNSPECIFIED.);
#465=B_SPLINE_CURVE_WITH_KNOTS('',3,(#24126,#24127,#24128,#24129,#24130,
#24131,#24132,#24133,#24134,#24135,#24136,#24137,#24138,#24139,#24140,#24141,
#24142,#24143,#24144,#24145,#24146,#24147),.UNSPECIFIED.,.F.,.F.,(4,3,3,
3,3,3,3,4),(39.0089340982494,39.8999462180201,40.8974448734706,41.8949435289211,
42.8924421843716,43.8899408398221,44.8874394952726,45.292119405429),
 .UNSPECIFIED.);
#466=B_SPLINE_CURVE_WITH_KNOTS('',3,(#24148,#24149,#24150,#24151,#24152,
#24153,#24154,#24155,#24156,#24157,#24158,#24159,#24160,#24161,#24162,#24163,
#24164,#24165,#24166,#24167,#24168,#24169),.UNSPECIFIED.,.F.,.F.,(4,3,3,
3,3,3,3,4),(-41.5454951067697,-40.8974448734706,-39.8999462180201,-38.9024475625696,
-37.9049489071191,-36.9074502516685,-35.909951596218,-35.2623097995902),
 .UNSPECIFIED.);
#467=B_SPLINE_CURVE_WITH_KNOTS('',3,(#24174,#24175,#24176,#24177,#24178,
#24179,#24180,#24181,#24182,#24183,#24184,#24185,#24186,#24187,#24188,#24189,
#24190,#24191,#24192,#24193,#24194,#24195,#24196,#24197,#24198),
 .UNSPECIFIED.,.F.,.F.,(4,3,3,3,3,3,3,3,4),(32.7257487910699,32.9174556298665,
33.9149542853171,34.9124529407676,35.9099515962181,36.9074502516685,37.904948907119,
38.9024475625696,39.0089340982494),.UNSPECIFIED.);
#468=B_SPLINE_CURVE_WITH_KNOTS('',3,(#24199,#24200,#24201,#24202,#24203,
#24204,#24205,#24206,#24207,#24208,#24209,#24210,#24211,#24212,#24213,#24214,
#24215,#24216,#24217,#24218,#24219,#24220),.UNSPECIFIED.,.F.,.F.,(4,3,3,
3,3,3,3,4),(-35.2623097995902,-34.9124529407676,-33.9149542853171,-32.9174556298665,
-31.919956974416,-30.9224583189655,-29.9249596635151,-28.9791244924106),
 .UNSPECIFIED.);
#469=B_SPLINE_CURVE_WITH_KNOTS('',3,(#24225,#24226,#24227,#24228,#24229,
#24230,#24231,#24232,#24233,#24234,#24235,#24236,#24237,#24238,#24239,#24240,
#24241,#24242,#24243,#24244,#24245,#24246),.UNSPECIFIED.,.F.,.F.,(4,3,3,
3,3,3,3,4),(26.4425634838902,26.9324636971635,27.929962352614,28.9274610080645,
29.924959663515,30.9224583189655,31.919956974416,32.7257487910699),
 .UNSPECIFIED.);
#470=B_SPLINE_CURVE_WITH_KNOTS('',3,(#24247,#24248,#24249,#24250,#24251,
#24252,#24253,#24254,#24255,#24256,#24257,#24258,#24259,#24260,#24261,#24262,
#24263,#24264,#24265,#24266,#24267,#24268,#24269,#24270,#24271),
 .UNSPECIFIED.,.F.,.F.,(4,3,3,3,3,3,3,3,4),(-28.9791244924106,-28.9274610080645,
-27.929962352614,-26.9324636971635,-25.934965041713,-24.9374663862625,-23.939967730812,
-22.9424690753615,-22.6959391852309),.UNSPECIFIED.);
#471=B_SPLINE_CURVE_WITH_KNOTS('',3,(#24276,#24277,#24278,#24279,#24280,
#24281,#24282,#24283,#24284,#24285,#24286,#24287,#24288,#24289,#24290,#24291,
#24292,#24293,#24294,#24295,#24296,#24297),.UNSPECIFIED.,.F.,.F.,(4,3,3,
3,3,3,3,4),(20.1593781767106,20.9474717644605,21.944970419911,22.9424690753615,
23.939967730812,24.9374663862625,25.934965041713,26.4425634838902),
 .UNSPECIFIED.);
#472=B_SPLINE_CURVE_WITH_KNOTS('',3,(#24298,#24299,#24300,#24301,#24302,
#24303,#24304,#24305,#24306,#24307,#24308,#24309,#24310,#24311,#24312,#24313,
#24314,#24315,#24316,#24317,#24318,#24319),.UNSPECIFIED.,.F.,.F.,(4,3,3,
3,3,3,3,4),(-22.6959391852309,-21.944970419911,-20.9474717644605,-19.94997310901,
-18.9524744535595,-17.954975798109,-16.9574771426585,-16.4127538780514),
 .UNSPECIFIED.);
#473=B_SPLINE_CURVE_WITH_KNOTS('',3,(#24324,#24325,#24326,#24327,#24328,
#24329,#24330,#24331,#24332,#24333,#24334,#24335,#24336,#24337,#24338,#24339,
#24340,#24341,#24342,#24343,#24344,#24345,#24346,#24347,#24348),
 .UNSPECIFIED.,.F.,.F.,(4,3,3,3,3,3,3,3,4),(13.8761928695311,13.964981176307,
14.9624798317575,15.959978487208,16.9574771426585,17.954975798109,18.9524744535595,
19.94997310901,20.1593781767106),.UNSPECIFIED.);
#474=B_SPLINE_CURVE_WITH_KNOTS('',3,(#24349,#24350,#24351,#24352,#24353,
#24354,#24355,#24356,#24357,#24358,#24359,#24360,#24361,#24362,#24363,#24364,
#24365,#24366,#24367,#24368,#24369,#24370),.UNSPECIFIED.,.F.,.F.,(4,3,3,
3,3,3,3,4),(-16.4127538780514,-15.959978487208,-14.9624798317575,-13.964981176307,
-12.9674825208565,-11.969983865406,-10.9724852099555,-10.1295685708718),
 .UNSPECIFIED.);
#475=B_SPLINE_CURVE_WITH_KNOTS('',3,(#24376,#24377,#24378,#24379,#24380,
#24381,#24382,#24383,#24384,#24385,#24386,#24387,#24388),.UNSPECIFIED.,
 .F.,.F.,(4,3,3,3,4),(-3.84638326369218,-2.9924959663515,-1.994997310901,
-0.997498655450501,0.),.UNSPECIFIED.);
#476=B_SPLINE_CURVE_WITH_KNOTS('',3,(#24391,#24392,#24393,#24394,#24395,
#24396,#24397,#24398,#24399,#24400,#24401,#24402,#24403,#24404,#24405,#24406,
#24407,#24408,#24409),.UNSPECIFIED.,.F.,.F.,(4,3,3,3,3,3,4),(2.01461286527449,
2.99249596635151,3.98999462180201,4.98749327725251,5.98499193270301,6.98249058815351,
7.59300756235149),.UNSPECIFIED.);
#477=B_SPLINE_CURVE_WITH_KNOTS('',3,(#24415,#24416,#24417,#24418,#24419),
 .UNSPECIFIED.,.F.,.F.,(4,1,4),(128.805298797182,129.566421347416,130.563920002866),
 .UNSPECIFIED.);
#478=B_SPLINE_CURVE_WITH_KNOTS('',3,(#24422,#24423,#24424,#24425,#24426,
#24427),.UNSPECIFIED.,.F.,.F.,(4,1,1,4),(128.805298797182,129.110486389585,
130.107985045035,131.085868146112),.UNSPECIFIED.);
#479=B_SPLINE_CURVE_WITH_KNOTS('',3,(#24432,#24433,#24434,#24435,#24436,
#24437,#24438,#24439,#24440,#24441,#24442),.UNSPECIFIED.,.F.,.F.,(4,1,1,
1,1,1,1,1,4),(122.522113490002,122.583930759262,123.581429414713,124.578928070163,
125.576426725614,126.573925381064,127.571424036515,128.568922691965,128.805298797182),
 .UNSPECIFIED.);
#480=B_SPLINE_CURVE_WITH_KNOTS('',3,(#24443,#24444,#24445,#24446,#24447,
#24448,#24449,#24450,#24451,#24452),.UNSPECIFIED.,.F.,.F.,(4,1,1,1,1,1,
1,4),(122.522113490002,123.125494456882,124.122993112332,125.120491767783,
126.117990423233,127.115489078684,128.112987734134,128.805298797182),
 .UNSPECIFIED.);
#481=B_SPLINE_CURVE_WITH_KNOTS('',3,(#24457,#24458,#24459,#24460,#24461,
#24462,#24463,#24464,#24465,#24466),.UNSPECIFIED.,.F.,.F.,(4,1,1,1,1,1,
1,4),(116.238928182822,116.598938826559,117.59643748201,118.59393613746,
119.591434792911,120.588933448361,121.586432103812,122.522113490002),
 .UNSPECIFIED.);
#482=B_SPLINE_CURVE_WITH_KNOTS('',3,(#24467,#24468,#24469,#24470,#24471,
#24472,#24473,#24474,#24475,#24476),.UNSPECIFIED.,.F.,.F.,(4,1,1,1,1,1,
1,4),(116.238928182822,117.140502524179,118.138001179629,119.13549983508,
120.13299849053,121.130497145981,122.127995801431,122.522113490002),
 .UNSPECIFIED.);
#483=B_SPLINE_CURVE_WITH_KNOTS('',3,(#24481,#24482,#24483,#24484,#24485,
#24486,#24487,#24488,#24489,#24490),.UNSPECIFIED.,.F.,.F.,(4,1,1,1,1,1,
1,4),(109.955742875643,110.613946893856,111.611445549307,112.608944204757,
113.606442860208,114.603941515658,115.601440171109,116.238928182822),
 .UNSPECIFIED.);
#484=B_SPLINE_CURVE_WITH_KNOTS('',3,(#24491,#24492,#24493,#24494,#24495,
#24496,#24497,#24498,#24499,#24500,#24501),.UNSPECIFIED.,.F.,.F.,(4,1,1,
1,1,1,1,1,4),(109.955742875643,110.158011936025,111.155510591476,112.153009246926,
113.150507902377,114.148006557827,115.145505213278,116.143003868728,116.238928182822),
 .UNSPECIFIED.);
#485=B_SPLINE_CURVE_WITH_KNOTS('',3,(#24506,#24507,#24508,#24509,#24510,
#24511,#24512,#24513,#24514,#24515),.UNSPECIFIED.,.F.,.F.,(4,1,1,1,1,1,
1,4),(103.672557568463,104.628954961153,105.626453616604,106.623952272054,
107.621450927505,108.618949582955,109.616448238406,109.955742875643),
 .UNSPECIFIED.);
#486=B_SPLINE_CURVE_WITH_KNOTS('',3,(#24516,#24517,#24518,#24519,#24520,
#24521,#24522,#24523,#24524,#24525),.UNSPECIFIED.,.F.,.F.,(4,1,1,1,1,1,
1,4),(103.672557568463,104.173020003322,105.170518658772,106.168017314223,
107.165515969673,108.163014625124,109.160513280574,109.955742875643),
 .UNSPECIFIED.);
#487=B_SPLINE_CURVE_WITH_KNOTS('',3,(#24530,#24531,#24532,#24533,#24534,
#24535,#24536,#24537,#24538,#24539,#24540),.UNSPECIFIED.,.F.,.F.,(4,1,1,
1,1,1,1,1,4),(97.3893722612835,97.6464643729998,98.6439630284503,99.6414616839008,
100.638960339351,101.636458994802,102.633957650252,103.631456305703,103.672557568463),
 .UNSPECIFIED.);
#488=B_SPLINE_CURVE_WITH_KNOTS('',3,(#24541,#24542,#24543,#24544,#24545,
#24546,#24547,#24548,#24549,#24550),.UNSPECIFIED.,.F.,.F.,(4,1,1,1,1,1,
1,4),(97.3893722612835,98.188028070619,99.1855267260695,100.18302538152,
101.18052403697,102.178022692421,103.175521347871,103.672557568463),
 .UNSPECIFIED.);
#489=B_SPLINE_CURVE_WITH_KNOTS('',3,(#24555,#24556,#24557,#24558,#24559,
#24560,#24561,#24562,#24563,#24564),.UNSPECIFIED.,.F.,.F.,(4,1,1,1,1,1,
1,4),(91.1061869541039,91.6614724402968,92.6589710957473,93.6564697511978,
94.6539684066483,95.6514670620988,96.6489657175493,97.3893722612835),
 .UNSPECIFIED.);
#490=B_SPLINE_CURVE_WITH_KNOTS('',3,(#24565,#24566,#24567,#24568,#24569,
#24570,#24571,#24572,#24573,#24574,#24575),.UNSPECIFIED.,.F.,.F.,(4,1,1,
1,1,1,1,1,4),(91.106186954104,91.2055374824655,92.203036137916,93.2005347933665,
94.198033448817,95.1955321042675,96.193030759718,97.1905294151685,97.3893722612835),
 .UNSPECIFIED.);
#491=B_SPLINE_CURVE_WITH_KNOTS('',3,(#24580,#24581,#24582,#24583,#24584,
#24585,#24586,#24587,#24588,#24589),.UNSPECIFIED.,.F.,.F.,(4,1,1,1,1,1,
1,4),(84.8230016469243,85.6764805075938,86.6739791630443,87.6714778184948,
88.6689764739453,89.6664751293958,90.6639737848463,91.1061869541039),
 .UNSPECIFIED.);
#492=B_SPLINE_CURVE_WITH_KNOTS('',3,(#24590,#24591,#24592,#24593,#24594,
#24595,#24596,#24597,#24598,#24599),.UNSPECIFIED.,.F.,.F.,(4,1,1,1,1,1,
1,4),(84.8230016469244,85.2205455497625,86.218044205213,87.2155428606635,
88.213041516114,89.2105401715645,90.208038827015,91.106186954104),
 .UNSPECIFIED.);
#493=B_SPLINE_CURVE_WITH_KNOTS('',3,(#24604,#24605,#24606,#24607,#24608,
#24609,#24610,#24611,#24612,#24613,#24614),.UNSPECIFIED.,.F.,.F.,(4,1,1,
1,1,1,1,1,4),(78.5398163397448,78.6939899194402,79.6914885748908,80.6889872303413,
81.6864858857918,82.6839845412423,83.6814831966928,84.6789818521433,84.8230016469243),
 .UNSPECIFIED.);
#494=B_SPLINE_CURVE_WITH_KNOTS('',3,(#24615,#24616,#24617,#24618,#24619,
#24620,#24621,#24622,#24623,#24624),.UNSPECIFIED.,.F.,.F.,(4,1,1,1,1,1,
1,4),(78.5398163397448,79.2355536170595,80.23305227251,81.2305509279605,
82.228049583411,83.2255482388615,84.223046894312,84.8230016469244),
 .UNSPECIFIED.);
#495=B_SPLINE_CURVE_WITH_KNOTS('',3,(#24629,#24630,#24631,#24632,#24633,
#24634,#24635,#24636,#24637,#24638),.UNSPECIFIED.,.F.,.F.,(4,1,1,1,1,1,
1,4),(72.2566310325652,72.7089979867372,73.7064966421877,74.7039952976382,
75.7014939530887,76.6989926085392,77.6964912639897,78.5398163397448),
 .UNSPECIFIED.);
#496=B_SPLINE_CURVE_WITH_KNOTS('',3,(#24639,#24640,#24641,#24642,#24643,
#24644,#24645,#24646,#24647,#24648),.UNSPECIFIED.,.F.,.F.,(4,1,1,1,1,1,
1,4),(72.2566310325652,73.2505616843565,74.248060339807,75.2455589952575,
76.243057650708,77.2405563061585,78.238054961609,78.5398163397448),
 .UNSPECIFIED.);
#497=B_SPLINE_CURVE_WITH_KNOTS('',3,(#24653,#24654,#24655,#24656,#24657,
#24658,#24659,#24660,#24661,#24662),.UNSPECIFIED.,.F.,.F.,(4,1,1,1,1,1,
1,4),(65.9734457253856,66.7240060540342,67.7215047094847,68.7190033649352,
69.7165020203857,70.7140006758362,71.7114993312867,72.2566310325652),
 .UNSPECIFIED.);
#498=B_SPLINE_CURVE_WITH_KNOTS('',3,(#24663,#24664,#24665,#24666,#24667,
#24668,#24669,#24670,#24671,#24672,#24673),.UNSPECIFIED.,.F.,.F.,(4,1,1,
1,1,1,1,1,4),(65.9734457253856,66.2680710962029,67.2655697516534,68.2630684071039,
69.2605670625544,70.2580657180049,71.2555643734554,72.2530630289059,72.2566310325652),
 .UNSPECIFIED.);
#499=B_SPLINE_CURVE_WITH_KNOTS('',3,(#24678,#24679,#24680,#24681,#24682,
#24683,#24684,#24685,#24686,#24687,#24688),.UNSPECIFIED.,.F.,.F.,(4,1,1,
1,1,1,1,1,4),(59.690260418206,59.7415154658807,60.7390141213312,61.7365127767817,
62.7340114322322,63.7315100876827,64.7290087431332,65.7265073985837,65.9734457253856),
 .UNSPECIFIED.);
#500=B_SPLINE_CURVE_WITH_KNOTS('',3,(#24689,#24690,#24691,#24692,#24693,
#24694,#24695,#24696,#24697,#24698),.UNSPECIFIED.,.F.,.F.,(4,1,1,1,1,1,
1,4),(59.690260418206,60.2830791634999,61.2805778189504,62.2780764744009,
63.2755751298514,64.2730737853019,65.2705724407524,65.9734457253856),
 .UNSPECIFIED.);
#501=B_SPLINE_CURVE_WITH_KNOTS('',3,(#24703,#24704,#24705,#24706,#24707,
#24708,#24709,#24710,#24711,#24712),.UNSPECIFIED.,.F.,.F.,(4,1,1,1,1,1,
1,4),(53.4070751110263,53.7565235331777,54.7540221886282,55.7515208440787,
56.7490194995292,57.7465181549797,58.7440168104302,59.690260418206),
 .UNSPECIFIED.);
#502=B_SPLINE_CURVE_WITH_KNOTS('',3,(#24713,#24714,#24715,#24716,#24717,
#24718,#24719,#24720,#24721,#24722),.UNSPECIFIED.,.F.,.F.,(4,1,1,1,1,1,
1,4),(53.4070751110264,54.2980872307969,55.2955858862474,56.2930845416979,
57.2905831971484,58.2880818525989,59.2855805080494,59.690260418206),
 .UNSPECIFIED.);
#503=B_SPLINE_CURVE_WITH_KNOTS('',3,(#24727,#24728,#24729,#24730,#24731,
#24732,#24733,#24734,#24735,#24736),.UNSPECIFIED.,.F.,.F.,(4,1,1,1,1,1,
1,4),(47.1238898038468,47.7715316004747,48.7690302559252,49.7665289113757,
50.7640275668262,51.7615262222767,52.7590248777272,53.4070751110263),
 .UNSPECIFIED.);
#504=B_SPLINE_CURVE_WITH_KNOTS('',3,(#24737,#24738,#24739,#24740,#24741,
#24742,#24743,#24744,#24745,#24746,#24747),.UNSPECIFIED.,.F.,.F.,(4,1,1,
1,1,1,1,1,4),(47.1238898038468,47.3155966426434,48.3130952980939,49.3105939535444,
50.3080926089949,51.3055912644454,52.3030899198959,53.3005885753464,53.4070751110264),
 .UNSPECIFIED.);
#505=B_SPLINE_CURVE_WITH_KNOTS('',3,(#24752,#24753,#24754,#24755,#24756,
#24757,#24758,#24759,#24760,#24761),.UNSPECIFIED.,.F.,.F.,(4,1,1,1,1,1,
1,4),(40.8407044966672,41.7865396677717,42.7840383232222,43.7815369786727,
44.7790356341232,45.7765342895737,46.7740329450242,47.1238898038468),
 .UNSPECIFIED.);
#506=B_SPLINE_CURVE_WITH_KNOTS('',3,(#24762,#24763,#24764,#24765,#24766,
#24767,#24768,#24769,#24770,#24771),.UNSPECIFIED.,.F.,.F.,(4,1,1,1,1,1,
1,4),(40.8407044966672,41.3306047099404,42.3281033653909,43.3256020208414,
44.3231006762919,45.3205993317424,46.3180979871929,47.1238898038468),
 .UNSPECIFIED.);
#507=B_SPLINE_CURVE_WITH_KNOTS('',3,(#24776,#24777,#24778,#24779,#24780,
#24781,#24782,#24783,#24784,#24785,#24786),.UNSPECIFIED.,.F.,.F.,(4,1,1,
1,1,1,1,1,4),(34.5575191894876,34.8040490796182,35.8015477350687,36.7990463905192,
37.7965450459697,38.7940437014202,39.7915423568707,40.7890410123212,40.8407044966672),
 .UNSPECIFIED.);
#508=B_SPLINE_CURVE_WITH_KNOTS('',3,(#24787,#24788,#24789,#24790,#24791,
#24792,#24793,#24794,#24795,#24796),.UNSPECIFIED.,.F.,.F.,(4,1,1,1,1,1,
1,4),(34.5575191894877,35.3456127772374,36.3431114326879,37.3406100881384,
38.3381087435889,39.3356073990394,40.3331060544899,40.8407044966672),
 .UNSPECIFIED.);
#509=B_SPLINE_CURVE_WITH_KNOTS('',3,(#24801,#24802,#24803,#24804,#24805,
#24806,#24807,#24808,#24809,#24810),.UNSPECIFIED.,.F.,.F.,(4,1,1,1,1,1,
1,4),(28.2743338823081,28.8190571469152,29.8165558023657,30.8140544578162,
31.8115531132667,32.8090517687172,33.8065504241677,34.5575191894876),
 .UNSPECIFIED.);
#510=B_SPLINE_CURVE_WITH_KNOTS('',3,(#24811,#24812,#24813,#24814,#24815,
#24816,#24817,#24818,#24819,#24820,#24821),.UNSPECIFIED.,.F.,.F.,(4,1,1,
1,1,1,1,1,4),(28.2743338823081,28.3631221890839,29.3606208445344,30.3581194999849,
31.3556181554354,32.3531168108859,33.3506154663364,34.3481141217869,34.5575191894877),
 .UNSPECIFIED.);
#511=B_SPLINE_CURVE_WITH_KNOTS('',3,(#24826,#24827,#24828,#24829,#24830,
#24831,#24832,#24833,#24834,#24835),.UNSPECIFIED.,.F.,.F.,(4,1,1,1,1,1,
1,4),(21.9911485751284,22.8340652142122,23.8315638696627,24.8290625251132,
25.8265611805637,26.8240598360142,27.8215584914647,28.2743338823081),
 .UNSPECIFIED.);
#512=B_SPLINE_CURVE_WITH_KNOTS('',3,(#24836,#24837,#24838,#24839,#24840,
#24841,#24842,#24843,#24844,#24845),.UNSPECIFIED.,.F.,.F.,(4,1,1,1,1,1,
1,4),(21.9911485751284,22.3781302563809,23.3756289118314,24.3731275672819,
25.3706262227324,26.3681248781829,27.3656235336334,28.2743338823081),
 .UNSPECIFIED.);
#513=B_SPLINE_CURVE_WITH_KNOTS('',3,(#24851,#24852,#24853,#24854,#24855),
 .UNSPECIFIED.,.F.,.F.,(4,1,4),(14.3981410127769,15.3956396682274,15.7079632679489),
 .UNSPECIFIED.);
#514=B_SPLINE_CURVE_WITH_KNOTS('',3,(#24858,#24859,#24860,#24861,#24862),
 .UNSPECIFIED.,.F.,.F.,(4,1,4),(13.8761928695311,14.8540759706082,15.7079632679488),
 .UNSPECIFIED.);
#515=B_SPLINE_CURVE_WITH_KNOTS('',3,(#24868,#24869,#24870,#24871,#24872,
#24873,#24874,#24875,#24876,#24877,#24878,#24879,#24880,#24881,#24882,#24883),
 .UNSPECIFIED.,.F.,.F.,(4,3,3,3,3,4),(114.407157784405,114.712345376808,
115.709844032258,116.707342687709,117.704841343159,118.70233999861),
 .UNSPECIFIED.);
#516=B_SPLINE_CURVE_WITH_KNOTS('',3,(#24891,#24892,#24893,#24894,#24895,
#24896,#24897,#24898,#24899,#24900,#24901,#24902,#24903,#24904,#24905,#24906,
#24907,#24908,#24909,#24910,#24911,#24912),.UNSPECIFIED.,.F.,.F.,(4,3,3,
3,3,3,3,4),(-116.687727133335,-115.709844032258,-114.712345376808,-113.714846721357,
-112.717348065907,-111.719849410456,-110.722350755006,-110.660533485745),
 .UNSPECIFIED.);
#517=B_SPLINE_CURVE_WITH_KNOTS('',3,(#24917,#24918,#24919,#24920,#24921,
#24922,#24923,#24924,#24925,#24926,#24927,#24928,#24929,#24930,#24931,#24932,
#24933,#24934,#24935,#24936,#24937,#24938),.UNSPECIFIED.,.F.,.F.,(4,3,3,
3,3,3,3,4),(108.123972477225,108.727353444105,109.724852099555,110.722350755006,
111.719849410456,112.717348065907,113.714846721357,114.407157784405),
 .UNSPECIFIED.);
#518=B_SPLINE_CURVE_WITH_KNOTS('',3,(#24939,#24940,#24941,#24942,#24943,
#24944,#24945,#24946,#24947,#24948,#24949,#24950,#24951,#24952,#24953,#24954,
#24955,#24956,#24957,#24958,#24959,#24960),.UNSPECIFIED.,.F.,.F.,(4,3,3,
3,3,3,3,4),(-110.660533485745,-109.724852099555,-108.727353444105,-107.729854788654,
-106.732356133204,-105.734857477753,-104.737358822303,-104.377348178566),
 .UNSPECIFIED.);
#519=B_SPLINE_CURVE_WITH_KNOTS('',3,(#24965,#24966,#24967,#24968,#24969,
#24970,#24971,#24972,#24973,#24974,#24975,#24976,#24977,#24978,#24979,#24980,
#24981,#24982,#24983,#24984,#24985,#24986),.UNSPECIFIED.,.F.,.F.,(4,3,3,
3,3,3,3,4),(101.840787170045,102.742361511402,103.739860166852,104.737358822303,
105.734857477753,106.732356133204,107.729854788654,108.123972477225),
 .UNSPECIFIED.);
#520=B_SPLINE_CURVE_WITH_KNOTS('',3,(#24987,#24988,#24989,#24990,#24991,
#24992,#24993,#24994,#24995,#24996,#24997,#24998,#24999,#25000,#25001,#25002,
#25003,#25004,#25005,#25006,#25007,#25008),.UNSPECIFIED.,.F.,.F.,(4,3,3,
3,3,3,3,4),(-104.377348178566,-103.739860166852,-102.742361511402,-101.744862855951,
-100.747364200501,-99.7498655450501,-98.7523668895996,-98.094162871386),
 .UNSPECIFIED.);
#521=B_SPLINE_CURVE_WITH_KNOTS('',3,(#25013,#25014,#25015,#25016,#25017,
#25018,#25019,#25020,#25021,#25022,#25023,#25024,#25025,#25026,#25027,#25028,
#25029,#25030,#25031,#25032,#25033,#25034,#25035,#25036,#25037),
 .UNSPECIFIED.,.F.,.F.,(4,3,3,3,3,3,3,3,4),(95.5576018628657,95.7598709232481,
96.7573695786986,97.7548682341491,98.7523668895996,99.7498655450501,100.747364200501,
101.744862855951,101.840787170045),.UNSPECIFIED.);
#522=B_SPLINE_CURVE_WITH_KNOTS('',3,(#25038,#25039,#25040,#25041,#25042,
#25043,#25044,#25045,#25046,#25047,#25048,#25049,#25050,#25051,#25052,#25053,
#25054,#25055,#25056,#25057,#25058,#25059),.UNSPECIFIED.,.F.,.F.,(4,3,3,
3,3,3,3,4),(-98.094162871386,-97.7548682341491,-96.7573695786986,-95.7598709232481,
-94.7623722677976,-93.7648736123471,-92.7673749568966,-91.8109775642064),
 .UNSPECIFIED.);
#523=B_SPLINE_CURVE_WITH_KNOTS('',3,(#25064,#25065,#25066,#25067,#25068,
#25069,#25070,#25071,#25072,#25073,#25074,#25075,#25076,#25077,#25078,#25079,
#25080,#25081,#25082,#25083,#25084,#25085),.UNSPECIFIED.,.F.,.F.,(4,3,3,
3,3,3,3,4),(89.2744165556862,89.7748789905451,90.7723776459956,91.7698763014461,
92.7673749568966,93.7648736123471,94.7623722677976,95.5576018628657),
 .UNSPECIFIED.);
#524=B_SPLINE_CURVE_WITH_KNOTS('',3,(#25086,#25087,#25088,#25089,#25090,
#25091,#25092,#25093,#25094,#25095,#25096,#25097,#25098,#25099,#25100,#25101,
#25102,#25103,#25104,#25105,#25106,#25107,#25108,#25109,#25110),
 .UNSPECIFIED.,.F.,.F.,(4,3,3,3,3,3,3,3,4),(-91.8109775642064,-91.7698763014461,
-90.7723776459956,-89.7748789905451,-88.7773803350946,-87.7798816796441,
-86.7823830241936,-85.7848843687431,-85.5277922570269),.UNSPECIFIED.);
#525=B_SPLINE_CURVE_WITH_KNOTS('',3,(#25115,#25116,#25117,#25118,#25119,
#25120,#25121,#25122,#25123,#25124,#25125,#25126,#25127,#25128,#25129,#25130,
#25131,#25132,#25133,#25134,#25135,#25136),.UNSPECIFIED.,.F.,.F.,(4,3,3,
3,3,3,3,4),(82.9912312485066,83.7898870578421,84.7873857132926,85.7848843687431,
86.7823830241936,87.7798816796441,88.7773803350946,89.2744165556862),
 .UNSPECIFIED.);
#526=B_SPLINE_CURVE_WITH_KNOTS('',3,(#25137,#25138,#25139,#25140,#25141,
#25142,#25143,#25144,#25145,#25146,#25147,#25148,#25149,#25150,#25151,#25152,
#25153,#25154,#25155,#25156,#25157,#25158),.UNSPECIFIED.,.F.,.F.,(4,3,3,
3,3,3,3,4),(-85.5277922570269,-84.7873857132926,-83.7898870578422,-82.7923884023916,
-81.7948897469411,-80.7973910914906,-79.7998924360401,-79.2446069498473),
 .UNSPECIFIED.);
#527=B_SPLINE_CURVE_WITH_KNOTS('',3,(#25163,#25164,#25165,#25166,#25167,
#25168,#25169,#25170,#25171,#25172,#25173,#25174,#25175,#25176,#25177,#25178,
#25179,#25180,#25181,#25182,#25183,#25184,#25185,#25186,#25187),
 .UNSPECIFIED.,.F.,.F.,(4,3,3,3,3,3,3,3,4),(76.708045941327,76.8073964696886,
77.8048951251391,78.8023937805896,79.7998924360401,80.7973910914906,81.7948897469411,
82.7923884023916,82.9912312485066),.UNSPECIFIED.);
#528=B_SPLINE_CURVE_WITH_KNOTS('',3,(#25188,#25189,#25190,#25191,#25192,
#25193,#25194,#25195,#25196,#25197,#25198,#25199,#25200,#25201,#25202,#25203,
#25204,#25205,#25206,#25207,#25208,#25209),.UNSPECIFIED.,.F.,.F.,(4,3,3,
3,3,3,3,4),(-79.2446069498473,-78.8023937805896,-77.8048951251391,-76.8073964696886,
-75.8098978142381,-74.8123991587876,-73.8149005033371,-72.9614216426677),
 .UNSPECIFIED.);
#529=B_SPLINE_CURVE_WITH_KNOTS('',3,(#25214,#25215,#25216,#25217,#25218,
#25219,#25220,#25221,#25222,#25223,#25224,#25225,#25226,#25227,#25228,#25229,
#25230,#25231,#25232,#25233,#25234,#25235),.UNSPECIFIED.,.F.,.F.,(4,3,3,
3,3,3,3,4),(70.4248606341474,70.8224045369856,71.8199031924361,72.8174018478866,
73.8149005033371,74.8123991587876,75.8098978142381,76.708045941327),
 .UNSPECIFIED.);
#530=B_SPLINE_CURVE_WITH_KNOTS('',3,(#25236,#25237,#25238,#25239,#25240,
#25241,#25242,#25243,#25244,#25245,#25246,#25247,#25248,#25249,#25250,#25251,
#25252,#25253,#25254,#25255,#25256,#25257,#25258,#25259,#25260),
 .UNSPECIFIED.,.F.,.F.,(4,3,3,3,3,3,3,3,4),(-72.9614216426677,-72.8174018478866,
-71.8199031924361,-70.8224045369856,-69.8249058815351,-68.8274072260846,
-67.8299085706341,-66.8324099151836,-66.6782363354882),.UNSPECIFIED.);
#531=B_SPLINE_CURVE_WITH_KNOTS('',3,(#25265,#25266,#25267,#25268,#25269,
#25270,#25271,#25272,#25273,#25274,#25275,#25276,#25277,#25278,#25279,#25280,
#25281,#25282,#25283,#25284,#25285,#25286),.UNSPECIFIED.,.F.,.F.,(4,3,3,
3,3,3,3,4),(64.1416753269678,64.8374126042826,65.8349112597331,66.8324099151836,
67.8299085706341,68.8274072260846,69.8249058815351,70.4248606341474),
 .UNSPECIFIED.);
#532=B_SPLINE_CURVE_WITH_KNOTS('',3,(#25287,#25288,#25289,#25290,#25291,
#25292,#25293,#25294,#25295,#25296,#25297,#25298,#25299,#25300,#25301,#25302,
#25303,#25304,#25305,#25306,#25307,#25308),.UNSPECIFIED.,.F.,.F.,(4,3,3,
3,3,3,3,4),(-66.6782363354882,-65.8349112597331,-64.8374126042826,-63.8399139488321,
-62.8424152933816,-61.8449166379311,-60.8474179824806,-60.3950510283085),
 .UNSPECIFIED.);
#533=B_SPLINE_CURVE_WITH_KNOTS('',3,(#25313,#25314,#25315,#25316,#25317,
#25318,#25319,#25320,#25321,#25322,#25323,#25324,#25325,#25326,#25327,#25328,
#25329,#25330,#25331,#25332,#25333,#25334),.UNSPECIFIED.,.F.,.F.,(4,3,3,
3,3,3,3,4),(57.8584900197882,58.8524206715796,59.8499193270301,60.8474179824806,
61.8449166379311,62.8424152933816,63.8399139488321,64.1416753269678),
 .UNSPECIFIED.);
#534=B_SPLINE_CURVE_WITH_KNOTS('',3,(#25335,#25336,#25337,#25338,#25339,
#25340,#25341,#25342,#25343,#25344,#25345,#25346,#25347,#25348,#25349,#25350,
#25351,#25352,#25353,#25354,#25355,#25356),.UNSPECIFIED.,.F.,.F.,(4,3,3,
3,3,3,3,4),(-60.3950510283085,-59.8499193270301,-58.8524206715796,-57.8549220161291,
-56.8574233606786,-55.8599247052281,-54.8624260497776,-54.1118657211289),
 .UNSPECIFIED.);
#535=B_SPLINE_CURVE_WITH_KNOTS('',3,(#25361,#25362,#25363,#25364,#25365,
#25366,#25367,#25368,#25369,#25370,#25371,#25372,#25373,#25374,#25375,#25376,
#25377,#25378,#25379,#25380,#25381,#25382,#25383,#25384,#25385),
 .UNSPECIFIED.,.F.,.F.,(4,3,3,3,3,3,3,3,4),(51.5753047126086,51.8699300834261,
52.8674287388766,53.8649273943271,54.8624260497776,55.8599247052281,56.8574233606786,
57.8549220161291,57.8584900197882),.UNSPECIFIED.);
#536=B_SPLINE_CURVE_WITH_KNOTS('',3,(#25386,#25387,#25388,#25389,#25390,
#25391,#25392,#25393,#25394,#25395,#25396,#25397,#25398,#25399,#25400,#25401,
#25402,#25403,#25404,#25405,#25406,#25407,#25408,#25409,#25410),
 .UNSPECIFIED.,.F.,.F.,(4,3,3,3,3,3,3,3,4),(-54.1118657211289,-53.8649273943271,
-52.8674287388766,-51.8699300834261,-50.8724314279756,-49.8749327725251,
-48.8774341170746,-47.8799354616241,-47.8286804139493),.UNSPECIFIED.);
#537=B_SPLINE_CURVE_WITH_KNOTS('',3,(#25415,#25416,#25417,#25418,#25419,
#25420,#25421,#25422,#25423,#25424,#25425,#25426,#25427,#25428,#25429,#25430,
#25431,#25432,#25433,#25434,#25435,#25436),.UNSPECIFIED.,.F.,.F.,(4,3,3,
3,3,3,3,4),(45.292119405429,45.8849381507231,46.8824368061736,47.8799354616241,
48.8774341170746,49.8749327725251,50.8724314279756,51.5753047126086),
 .UNSPECIFIED.);
#538=B_SPLINE_CURVE_WITH_KNOTS('',3,(#25437,#25438,#25439,#25440,#25441,
#25442,#25443,#25444,#25445,#25446,#25447,#25448,#25449,#25450,#25451,#25452,
#25453,#25454,#25455,#25456,#25457,#25458),.UNSPECIFIED.,.F.,.F.,(4,3,3,
3,3,3,3,4),(-47.8286804139493,-46.8824368061736,-45.8849381507231,-44.8874394952726,
-43.8899408398221,-42.8924421843716,-41.8949435289211,-41.5454951067697),
 .UNSPECIFIED.);
#539=B_SPLINE_CURVE_WITH_KNOTS('',3,(#25463,#25464,#25465,#25466,#25467,
#25468,#25469,#25470,#25471,#25472,#25473,#25474,#25475,#25476,#25477,#25478,
#25479,#25480,#25481,#25482,#25483,#25484),.UNSPECIFIED.,.F.,.F.,(4,3,3,
3,3,3,3,4),(39.0089340982494,39.8999462180201,40.8974448734706,41.8949435289211,
42.8924421843716,43.8899408398221,44.8874394952726,45.292119405429),
 .UNSPECIFIED.);
#540=B_SPLINE_CURVE_WITH_KNOTS('',3,(#25485,#25486,#25487,#25488,#25489,
#25490,#25491,#25492,#25493,#25494,#25495,#25496,#25497,#25498,#25499,#25500,
#25501,#25502,#25503,#25504,#25505,#25506),.UNSPECIFIED.,.F.,.F.,(4,3,3,
3,3,3,3,4),(-41.5454951067697,-40.8974448734706,-39.8999462180201,-38.9024475625696,
-37.9049489071191,-36.9074502516685,-35.909951596218,-35.2623097995902),
 .UNSPECIFIED.);
#541=B_SPLINE_CURVE_WITH_KNOTS('',3,(#25511,#25512,#25513,#25514,#25515,
#25516,#25517,#25518,#25519,#25520,#25521,#25522,#25523,#25524,#25525,#25526,
#25527,#25528,#25529,#25530,#25531,#25532,#25533,#25534,#25535),
 .UNSPECIFIED.,.F.,.F.,(4,3,3,3,3,3,3,3,4),(32.7257487910699,32.9174556298665,
33.9149542853171,34.9124529407676,35.9099515962181,36.9074502516685,37.904948907119,
38.9024475625696,39.0089340982494),.UNSPECIFIED.);
#542=B_SPLINE_CURVE_WITH_KNOTS('',3,(#25536,#25537,#25538,#25539,#25540,
#25541,#25542,#25543,#25544,#25545,#25546,#25547,#25548,#25549,#25550,#25551,
#25552,#25553,#25554,#25555,#25556,#25557),.UNSPECIFIED.,.F.,.F.,(4,3,3,
3,3,3,3,4),(-35.2623097995902,-34.9124529407676,-33.9149542853171,-32.9174556298665,
-31.919956974416,-30.9224583189655,-29.9249596635151,-28.9791244924106),
 .UNSPECIFIED.);
#543=B_SPLINE_CURVE_WITH_KNOTS('',3,(#25562,#25563,#25564,#25565,#25566,
#25567,#25568,#25569,#25570,#25571,#25572,#25573,#25574,#25575,#25576,#25577,
#25578,#25579,#25580,#25581,#25582,#25583),.UNSPECIFIED.,.F.,.F.,(4,3,3,
3,3,3,3,4),(26.4425634838902,26.9324636971635,27.929962352614,28.9274610080645,
29.924959663515,30.9224583189655,31.919956974416,32.7257487910699),
 .UNSPECIFIED.);
#544=B_SPLINE_CURVE_WITH_KNOTS('',3,(#25584,#25585,#25586,#25587,#25588,
#25589,#25590,#25591,#25592,#25593,#25594,#25595,#25596,#25597,#25598,#25599,
#25600,#25601,#25602,#25603,#25604,#25605,#25606,#25607,#25608),
 .UNSPECIFIED.,.F.,.F.,(4,3,3,3,3,3,3,3,4),(-28.9791244924106,-28.9274610080645,
-27.929962352614,-26.9324636971635,-25.934965041713,-24.9374663862625,-23.939967730812,
-22.9424690753615,-22.6959391852309),.UNSPECIFIED.);
#545=B_SPLINE_CURVE_WITH_KNOTS('',3,(#25613,#25614,#25615,#25616,#25617,
#25618,#25619,#25620,#25621,#25622,#25623,#25624,#25625,#25626,#25627,#25628,
#25629,#25630,#25631,#25632,#25633,#25634),.UNSPECIFIED.,.F.,.F.,(4,3,3,
3,3,3,3,4),(20.1593781767106,20.9474717644605,21.944970419911,22.9424690753615,
23.939967730812,24.9374663862625,25.934965041713,26.4425634838902),
 .UNSPECIFIED.);
#546=B_SPLINE_CURVE_WITH_KNOTS('',3,(#25635,#25636,#25637,#25638,#25639,
#25640,#25641,#25642,#25643,#25644,#25645,#25646,#25647,#25648,#25649,#25650,
#25651,#25652,#25653,#25654,#25655,#25656),.UNSPECIFIED.,.F.,.F.,(4,3,3,
3,3,3,3,4),(-22.6959391852309,-21.944970419911,-20.9474717644605,-19.94997310901,
-18.9524744535595,-17.954975798109,-16.9574771426585,-16.4127538780514),
 .UNSPECIFIED.);
#547=B_SPLINE_CURVE_WITH_KNOTS('',3,(#25661,#25662,#25663,#25664,#25665,
#25666,#25667,#25668,#25669,#25670,#25671,#25672,#25673,#25674,#25675,#25676,
#25677,#25678,#25679,#25680,#25681,#25682,#25683,#25684,#25685),
 .UNSPECIFIED.,.F.,.F.,(4,3,3,3,3,3,3,3,4),(13.8761928695311,13.964981176307,
14.9624798317575,15.959978487208,16.9574771426585,17.954975798109,18.9524744535595,
19.94997310901,20.1593781767106),.UNSPECIFIED.);
#548=B_SPLINE_CURVE_WITH_KNOTS('',3,(#25686,#25687,#25688,#25689,#25690,
#25691,#25692,#25693,#25694,#25695,#25696,#25697,#25698,#25699,#25700,#25701,
#25702,#25703,#25704,#25705,#25706,#25707),.UNSPECIFIED.,.F.,.F.,(4,3,3,
3,3,3,3,4),(-16.4127538780514,-15.959978487208,-14.9624798317575,-13.964981176307,
-12.9674825208565,-11.969983865406,-10.9724852099555,-10.1295685708718),
 .UNSPECIFIED.);
#549=B_SPLINE_CURVE_WITH_KNOTS('',3,(#25713,#25714,#25715,#25716,#25717,
#25718,#25719,#25720,#25721,#25722,#25723,#25724,#25725),.UNSPECIFIED.,
 .F.,.F.,(4,3,3,3,4),(-3.84638326369218,-2.9924959663515,-1.994997310901,
-0.997498655450501,0.),.UNSPECIFIED.);
#550=B_SPLINE_CURVE_WITH_KNOTS('',3,(#25728,#25729,#25730,#25731,#25732,
#25733,#25734,#25735,#25736,#25737,#25738,#25739,#25740,#25741,#25742,#25743,
#25744,#25745,#25746),.UNSPECIFIED.,.F.,.F.,(4,3,3,3,3,3,4),(2.01461286527449,
2.99249596635151,3.98999462180201,4.98749327725251,5.98499193270301,6.98249058815351,
7.59300756235149),.UNSPECIFIED.);
#551=B_SPLINE_CURVE_WITH_KNOTS('',3,(#25752,#25753,#25754,#25755,#25756),
 .UNSPECIFIED.,.F.,.F.,(4,1,4),(128.805298797182,129.566421347416,130.563920002866),
 .UNSPECIFIED.);
#552=B_SPLINE_CURVE_WITH_KNOTS('',3,(#25759,#25760,#25761,#25762,#25763,
#25764),.UNSPECIFIED.,.F.,.F.,(4,1,1,4),(128.805298797182,129.110486389585,
130.107985045035,131.085868146112),.UNSPECIFIED.);
#553=B_SPLINE_CURVE_WITH_KNOTS('',3,(#25769,#25770,#25771,#25772,#25773,
#25774,#25775,#25776,#25777,#25778,#25779),.UNSPECIFIED.,.F.,.F.,(4,1,1,
1,1,1,1,1,4),(122.522113490002,122.583930759262,123.581429414713,124.578928070163,
125.576426725614,126.573925381064,127.571424036515,128.568922691965,128.805298797182),
 .UNSPECIFIED.);
#554=B_SPLINE_CURVE_WITH_KNOTS('',3,(#25780,#25781,#25782,#25783,#25784,
#25785,#25786,#25787,#25788,#25789),.UNSPECIFIED.,.F.,.F.,(4,1,1,1,1,1,
1,4),(122.522113490002,123.125494456882,124.122993112332,125.120491767783,
126.117990423233,127.115489078684,128.112987734134,128.805298797182),
 .UNSPECIFIED.);
#555=B_SPLINE_CURVE_WITH_KNOTS('',3,(#25794,#25795,#25796,#25797,#25798,
#25799,#25800,#25801,#25802,#25803),.UNSPECIFIED.,.F.,.F.,(4,1,1,1,1,1,
1,4),(116.238928182822,116.598938826559,117.59643748201,118.59393613746,
119.591434792911,120.588933448361,121.586432103812,122.522113490002),
 .UNSPECIFIED.);
#556=B_SPLINE_CURVE_WITH_KNOTS('',3,(#25804,#25805,#25806,#25807,#25808,
#25809,#25810,#25811,#25812,#25813),.UNSPECIFIED.,.F.,.F.,(4,1,1,1,1,1,
1,4),(116.238928182822,117.140502524179,118.138001179629,119.13549983508,
120.13299849053,121.130497145981,122.127995801431,122.522113490002),
 .UNSPECIFIED.);
#557=B_SPLINE_CURVE_WITH_KNOTS('',3,(#25818,#25819,#25820,#25821,#25822,
#25823,#25824,#25825,#25826,#25827),.UNSPECIFIED.,.F.,.F.,(4,1,1,1,1,1,
1,4),(109.955742875643,110.613946893856,111.611445549307,112.608944204757,
113.606442860208,114.603941515658,115.601440171109,116.238928182822),
 .UNSPECIFIED.);
#558=B_SPLINE_CURVE_WITH_KNOTS('',3,(#25828,#25829,#25830,#25831,#25832,
#25833,#25834,#25835,#25836,#25837,#25838),.UNSPECIFIED.,.F.,.F.,(4,1,1,
1,1,1,1,1,4),(109.955742875643,110.158011936025,111.155510591476,112.153009246926,
113.150507902377,114.148006557827,115.145505213278,116.143003868728,116.238928182822),
 .UNSPECIFIED.);
#559=B_SPLINE_CURVE_WITH_KNOTS('',3,(#25843,#25844,#25845,#25846,#25847,
#25848,#25849,#25850,#25851,#25852),.UNSPECIFIED.,.F.,.F.,(4,1,1,1,1,1,
1,4),(103.672557568463,104.628954961153,105.626453616604,106.623952272054,
107.621450927505,108.618949582955,109.616448238406,109.955742875643),
 .UNSPECIFIED.);
#560=B_SPLINE_CURVE_WITH_KNOTS('',3,(#25853,#25854,#25855,#25856,#25857,
#25858,#25859,#25860,#25861,#25862),.UNSPECIFIED.,.F.,.F.,(4,1,1,1,1,1,
1,4),(103.672557568463,104.173020003322,105.170518658772,106.168017314223,
107.165515969673,108.163014625124,109.160513280574,109.955742875643),
 .UNSPECIFIED.);
#561=B_SPLINE_CURVE_WITH_KNOTS('',3,(#25867,#25868,#25869,#25870,#25871,
#25872,#25873,#25874,#25875,#25876,#25877),.UNSPECIFIED.,.F.,.F.,(4,1,1,
1,1,1,1,1,4),(97.3893722612835,97.6464643729998,98.6439630284503,99.6414616839008,
100.638960339351,101.636458994802,102.633957650252,103.631456305703,103.672557568463),
 .UNSPECIFIED.);
#562=B_SPLINE_CURVE_WITH_KNOTS('',3,(#25878,#25879,#25880,#25881,#25882,
#25883,#25884,#25885,#25886,#25887),.UNSPECIFIED.,.F.,.F.,(4,1,1,1,1,1,
1,4),(97.3893722612835,98.188028070619,99.1855267260695,100.18302538152,
101.18052403697,102.178022692421,103.175521347871,103.672557568463),
 .UNSPECIFIED.);
#563=B_SPLINE_CURVE_WITH_KNOTS('',3,(#25892,#25893,#25894,#25895,#25896,
#25897,#25898,#25899,#25900,#25901),.UNSPECIFIED.,.F.,.F.,(4,1,1,1,1,1,
1,4),(91.1061869541039,91.6614724402968,92.6589710957473,93.6564697511978,
94.6539684066483,95.6514670620988,96.6489657175493,97.3893722612835),
 .UNSPECIFIED.);
#564=B_SPLINE_CURVE_WITH_KNOTS('',3,(#25902,#25903,#25904,#25905,#25906,
#25907,#25908,#25909,#25910,#25911,#25912),.UNSPECIFIED.,.F.,.F.,(4,1,1,
1,1,1,1,1,4),(91.106186954104,91.2055374824655,92.203036137916,93.2005347933665,
94.198033448817,95.1955321042675,96.193030759718,97.1905294151685,97.3893722612835),
 .UNSPECIFIED.);
#565=B_SPLINE_CURVE_WITH_KNOTS('',3,(#25917,#25918,#25919,#25920,#25921,
#25922,#25923,#25924,#25925,#25926),.UNSPECIFIED.,.F.,.F.,(4,1,1,1,1,1,
1,4),(84.8230016469243,85.6764805075938,86.6739791630443,87.6714778184948,
88.6689764739453,89.6664751293958,90.6639737848463,91.1061869541039),
 .UNSPECIFIED.);
#566=B_SPLINE_CURVE_WITH_KNOTS('',3,(#25927,#25928,#25929,#25930,#25931,
#25932,#25933,#25934,#25935,#25936),.UNSPECIFIED.,.F.,.F.,(4,1,1,1,1,1,
1,4),(84.8230016469244,85.2205455497625,86.218044205213,87.2155428606635,
88.213041516114,89.2105401715645,90.208038827015,91.106186954104),
 .UNSPECIFIED.);
#567=B_SPLINE_CURVE_WITH_KNOTS('',3,(#25941,#25942,#25943,#25944,#25945,
#25946,#25947,#25948,#25949,#25950,#25951),.UNSPECIFIED.,.F.,.F.,(4,1,1,
1,1,1,1,1,4),(78.5398163397448,78.6939899194402,79.6914885748908,80.6889872303413,
81.6864858857918,82.6839845412423,83.6814831966928,84.6789818521433,84.8230016469243),
 .UNSPECIFIED.);
#568=B_SPLINE_CURVE_WITH_KNOTS('',3,(#25952,#25953,#25954,#25955,#25956,
#25957,#25958,#25959,#25960,#25961),.UNSPECIFIED.,.F.,.F.,(4,1,1,1,1,1,
1,4),(78.5398163397448,79.2355536170595,80.23305227251,81.2305509279605,
82.228049583411,83.2255482388615,84.223046894312,84.8230016469244),
 .UNSPECIFIED.);
#569=B_SPLINE_CURVE_WITH_KNOTS('',3,(#25966,#25967,#25968,#25969,#25970,
#25971,#25972,#25973,#25974,#25975),.UNSPECIFIED.,.F.,.F.,(4,1,1,1,1,1,
1,4),(72.2566310325652,72.7089979867372,73.7064966421877,74.7039952976382,
75.7014939530887,76.6989926085392,77.6964912639897,78.5398163397448),
 .UNSPECIFIED.);
#570=B_SPLINE_CURVE_WITH_KNOTS('',3,(#25976,#25977,#25978,#25979,#25980,
#25981,#25982,#25983,#25984,#25985),.UNSPECIFIED.,.F.,.F.,(4,1,1,1,1,1,
1,4),(72.2566310325652,73.2505616843565,74.248060339807,75.2455589952575,
76.243057650708,77.2405563061585,78.238054961609,78.5398163397448),
 .UNSPECIFIED.);
#571=B_SPLINE_CURVE_WITH_KNOTS('',3,(#25990,#25991,#25992,#25993,#25994,
#25995,#25996,#25997,#25998,#25999),.UNSPECIFIED.,.F.,.F.,(4,1,1,1,1,1,
1,4),(65.9734457253856,66.7240060540342,67.7215047094847,68.7190033649352,
69.7165020203857,70.7140006758362,71.7114993312867,72.2566310325652),
 .UNSPECIFIED.);
#572=B_SPLINE_CURVE_WITH_KNOTS('',3,(#26000,#26001,#26002,#26003,#26004,
#26005,#26006,#26007,#26008,#26009,#26010),.UNSPECIFIED.,.F.,.F.,(4,1,1,
1,1,1,1,1,4),(65.9734457253856,66.2680710962029,67.2655697516534,68.2630684071039,
69.2605670625544,70.2580657180049,71.2555643734554,72.2530630289059,72.2566310325652),
 .UNSPECIFIED.);
#573=B_SPLINE_CURVE_WITH_KNOTS('',3,(#26015,#26016,#26017,#26018,#26019,
#26020,#26021,#26022,#26023,#26024,#26025),.UNSPECIFIED.,.F.,.F.,(4,1,1,
1,1,1,1,1,4),(59.690260418206,59.7415154658807,60.7390141213312,61.7365127767817,
62.7340114322322,63.7315100876827,64.7290087431332,65.7265073985837,65.9734457253856),
 .UNSPECIFIED.);
#574=B_SPLINE_CURVE_WITH_KNOTS('',3,(#26026,#26027,#26028,#26029,#26030,
#26031,#26032,#26033,#26034,#26035),.UNSPECIFIED.,.F.,.F.,(4,1,1,1,1,1,
1,4),(59.690260418206,60.2830791634999,61.2805778189504,62.2780764744009,
63.2755751298514,64.2730737853019,65.2705724407524,65.9734457253856),
 .UNSPECIFIED.);
#575=B_SPLINE_CURVE_WITH_KNOTS('',3,(#26040,#26041,#26042,#26043,#26044,
#26045,#26046,#26047,#26048,#26049),.UNSPECIFIED.,.F.,.F.,(4,1,1,1,1,1,
1,4),(53.4070751110263,53.7565235331777,54.7540221886282,55.7515208440787,
56.7490194995292,57.7465181549797,58.7440168104302,59.690260418206),
 .UNSPECIFIED.);
#576=B_SPLINE_CURVE_WITH_KNOTS('',3,(#26050,#26051,#26052,#26053,#26054,
#26055,#26056,#26057,#26058,#26059),.UNSPECIFIED.,.F.,.F.,(4,1,1,1,1,1,
1,4),(53.4070751110264,54.2980872307969,55.2955858862474,56.2930845416979,
57.2905831971484,58.2880818525989,59.2855805080494,59.690260418206),
 .UNSPECIFIED.);
#577=B_SPLINE_CURVE_WITH_KNOTS('',3,(#26064,#26065,#26066,#26067,#26068,
#26069,#26070,#26071,#26072,#26073),.UNSPECIFIED.,.F.,.F.,(4,1,1,1,1,1,
1,4),(47.1238898038468,47.7715316004747,48.7690302559252,49.7665289113757,
50.7640275668262,51.7615262222767,52.7590248777272,53.4070751110263),
 .UNSPECIFIED.);
#578=B_SPLINE_CURVE_WITH_KNOTS('',3,(#26074,#26075,#26076,#26077,#26078,
#26079,#26080,#26081,#26082,#26083,#26084),.UNSPECIFIED.,.F.,.F.,(4,1,1,
1,1,1,1,1,4),(47.1238898038468,47.3155966426434,48.3130952980939,49.3105939535444,
50.3080926089949,51.3055912644454,52.3030899198959,53.3005885753464,53.4070751110264),
 .UNSPECIFIED.);
#579=B_SPLINE_CURVE_WITH_KNOTS('',3,(#26089,#26090,#26091,#26092,#26093,
#26094,#26095,#26096,#26097,#26098),.UNSPECIFIED.,.F.,.F.,(4,1,1,1,1,1,
1,4),(40.8407044966672,41.7865396677717,42.7840383232222,43.7815369786727,
44.7790356341232,45.7765342895737,46.7740329450242,47.1238898038468),
 .UNSPECIFIED.);
#580=B_SPLINE_CURVE_WITH_KNOTS('',3,(#26099,#26100,#26101,#26102,#26103,
#26104,#26105,#26106,#26107,#26108),.UNSPECIFIED.,.F.,.F.,(4,1,1,1,1,1,
1,4),(40.8407044966672,41.3306047099404,42.3281033653909,43.3256020208414,
44.3231006762919,45.3205993317424,46.3180979871929,47.1238898038468),
 .UNSPECIFIED.);
#581=B_SPLINE_CURVE_WITH_KNOTS('',3,(#26113,#26114,#26115,#26116,#26117,
#26118,#26119,#26120,#26121,#26122,#26123),.UNSPECIFIED.,.F.,.F.,(4,1,1,
1,1,1,1,1,4),(34.5575191894876,34.8040490796182,35.8015477350687,36.7990463905192,
37.7965450459697,38.7940437014202,39.7915423568707,40.7890410123212,40.8407044966672),
 .UNSPECIFIED.);
#582=B_SPLINE_CURVE_WITH_KNOTS('',3,(#26124,#26125,#26126,#26127,#26128,
#26129,#26130,#26131,#26132,#26133),.UNSPECIFIED.,.F.,.F.,(4,1,1,1,1,1,
1,4),(34.5575191894877,35.3456127772374,36.3431114326879,37.3406100881384,
38.3381087435889,39.3356073990394,40.3331060544899,40.8407044966672),
 .UNSPECIFIED.);
#583=B_SPLINE_CURVE_WITH_KNOTS('',3,(#26138,#26139,#26140,#26141,#26142,
#26143,#26144,#26145,#26146,#26147),.UNSPECIFIED.,.F.,.F.,(4,1,1,1,1,1,
1,4),(28.2743338823081,28.8190571469152,29.8165558023657,30.8140544578162,
31.8115531132667,32.8090517687172,33.8065504241677,34.5575191894876),
 .UNSPECIFIED.);
#584=B_SPLINE_CURVE_WITH_KNOTS('',3,(#26148,#26149,#26150,#26151,#26152,
#26153,#26154,#26155,#26156,#26157,#26158),.UNSPECIFIED.,.F.,.F.,(4,1,1,
1,1,1,1,1,4),(28.2743338823081,28.3631221890839,29.3606208445344,30.3581194999849,
31.3556181554354,32.3531168108859,33.3506154663364,34.3481141217869,34.5575191894877),
 .UNSPECIFIED.);
#585=B_SPLINE_CURVE_WITH_KNOTS('',3,(#26163,#26164,#26165,#26166,#26167,
#26168,#26169,#26170,#26171,#26172),.UNSPECIFIED.,.F.,.F.,(4,1,1,1,1,1,
1,4),(21.9911485751284,22.8340652142122,23.8315638696627,24.8290625251132,
25.8265611805637,26.8240598360142,27.8215584914647,28.2743338823081),
 .UNSPECIFIED.);
#586=B_SPLINE_CURVE_WITH_KNOTS('',3,(#26173,#26174,#26175,#26176,#26177,
#26178,#26179,#26180,#26181,#26182),.UNSPECIFIED.,.F.,.F.,(4,1,1,1,1,1,
1,4),(21.9911485751284,22.3781302563809,23.3756289118314,24.3731275672819,
25.3706262227324,26.3681248781829,27.3656235336334,28.2743338823081),
 .UNSPECIFIED.);
#587=B_SPLINE_CURVE_WITH_KNOTS('',3,(#26188,#26189,#26190,#26191,#26192),
 .UNSPECIFIED.,.F.,.F.,(4,1,4),(14.3981410127769,15.3956396682274,15.7079632679489),
 .UNSPECIFIED.);
#588=B_SPLINE_CURVE_WITH_KNOTS('',3,(#26195,#26196,#26197,#26198,#26199),
 .UNSPECIFIED.,.F.,.F.,(4,1,4),(13.8761928695311,14.8540759706082,15.7079632679488),
 .UNSPECIFIED.);
#589=B_SPLINE_CURVE_WITH_KNOTS('',3,(#26205,#26206,#26207,#26208,#26209,
#26210,#26211,#26212,#26213,#26214,#26215,#26216,#26217,#26218,#26219,#26220),
 .UNSPECIFIED.,.F.,.F.,(4,3,3,3,3,4),(114.407157784404,114.712345376808,
115.709844032258,116.707342687709,117.704841343159,118.702339998609),
 .UNSPECIFIED.);
#590=B_SPLINE_CURVE_WITH_KNOTS('',3,(#26228,#26229,#26230,#26231,#26232,
#26233,#26234,#26235,#26236,#26237,#26238,#26239,#26240,#26241,#26242,#26243,
#26244,#26245,#26246,#26247,#26248,#26249),.UNSPECIFIED.,.F.,.F.,(4,3,3,
3,3,3,3,4),(-116.687727133335,-115.709844032258,-114.712345376808,-113.714846721357,
-112.717348065907,-111.719849410456,-110.722350755006,-110.660533485745),
 .UNSPECIFIED.);
#591=B_SPLINE_CURVE_WITH_KNOTS('',3,(#26254,#26255,#26256,#26257,#26258,
#26259,#26260,#26261,#26262,#26263,#26264,#26265,#26266,#26267,#26268,#26269,
#26270,#26271,#26272,#26273,#26274,#26275),.UNSPECIFIED.,.F.,.F.,(4,3,3,
3,3,3,3,4),(108.123972477224,108.727353444105,109.724852099555,110.722350755006,
111.719849410456,112.717348065907,113.714846721357,114.407157784404),
 .UNSPECIFIED.);
#592=B_SPLINE_CURVE_WITH_KNOTS('',3,(#26276,#26277,#26278,#26279,#26280,
#26281,#26282,#26283,#26284,#26285,#26286,#26287,#26288,#26289,#26290,#26291,
#26292,#26293,#26294,#26295,#26296,#26297),.UNSPECIFIED.,.F.,.F.,(4,3,3,
3,3,3,3,4),(-110.660533485745,-109.724852099555,-108.727353444105,-107.729854788654,
-106.732356133204,-105.734857477753,-104.737358822303,-104.377348178565),
 .UNSPECIFIED.);
#593=B_SPLINE_CURVE_WITH_KNOTS('',3,(#26302,#26303,#26304,#26305,#26306,
#26307,#26308,#26309,#26310,#26311,#26312,#26313,#26314,#26315,#26316,#26317,
#26318,#26319,#26320,#26321,#26322,#26323),.UNSPECIFIED.,.F.,.F.,(4,3,3,
3,3,3,3,4),(101.840787170045,102.742361511402,103.739860166852,104.737358822303,
105.734857477753,106.732356133204,107.729854788654,108.123972477224),
 .UNSPECIFIED.);
#594=B_SPLINE_CURVE_WITH_KNOTS('',3,(#26324,#26325,#26326,#26327,#26328,
#26329,#26330,#26331,#26332,#26333,#26334,#26335,#26336,#26337,#26338,#26339,
#26340,#26341,#26342,#26343,#26344,#26345),.UNSPECIFIED.,.F.,.F.,(4,3,3,
3,3,3,3,4),(-104.377348178565,-103.739860166852,-102.742361511402,-101.744862855951,
-100.747364200501,-99.74986554505,-98.7523668895995,-98.0941628713858),
 .UNSPECIFIED.);
#595=B_SPLINE_CURVE_WITH_KNOTS('',3,(#26350,#26351,#26352,#26353,#26354,
#26355,#26356,#26357,#26358,#26359,#26360,#26361,#26362,#26363,#26364,#26365,
#26366,#26367,#26368,#26369,#26370,#26371,#26372,#26373,#26374),
 .UNSPECIFIED.,.F.,.F.,(4,3,3,3,3,3,3,3,4),(95.5576018628653,95.7598709232481,
96.7573695786986,97.7548682341491,98.7523668895996,99.7498655450501,100.747364200501,
101.744862855951,101.840787170045),.UNSPECIFIED.);
#596=B_SPLINE_CURVE_WITH_KNOTS('',3,(#26375,#26376,#26377,#26378,#26379,
#26380,#26381,#26382,#26383,#26384,#26385,#26386,#26387,#26388,#26389,#26390,
#26391,#26392,#26393,#26394,#26395,#26396),.UNSPECIFIED.,.F.,.F.,(4,3,3,
3,3,3,3,4),(-98.0941628713858,-97.754868234149,-96.7573695786985,-95.759870923248,
-94.7623722677975,-93.764873612347,-92.7673749568965,-91.8109775642062),
 .UNSPECIFIED.);
#597=B_SPLINE_CURVE_WITH_KNOTS('',3,(#26401,#26402,#26403,#26404,#26405,
#26406,#26407,#26408,#26409,#26410,#26411,#26412,#26413,#26414,#26415,#26416,
#26417,#26418,#26419,#26420,#26421,#26422),.UNSPECIFIED.,.F.,.F.,(4,3,3,
3,3,3,3,4),(89.2744165556857,89.774878990545,90.7723776459955,91.769876301446,
92.7673749568965,93.764873612347,94.7623722677975,95.5576018628653),
 .UNSPECIFIED.);
#598=B_SPLINE_CURVE_WITH_KNOTS('',3,(#26423,#26424,#26425,#26426,#26427,
#26428,#26429,#26430,#26431,#26432,#26433,#26434,#26435,#26436,#26437,#26438,
#26439,#26440,#26441,#26442,#26443,#26444,#26445,#26446,#26447),
 .UNSPECIFIED.,.F.,.F.,(4,3,3,3,3,3,3,3,4),(-91.8109775642062,-91.769876301446,
-90.7723776459955,-89.774878990545,-88.7773803350945,-87.779881679644,-86.7823830241935,
-85.784884368743,-85.5277922570266),.UNSPECIFIED.);
#599=B_SPLINE_CURVE_WITH_KNOTS('',3,(#26452,#26453,#26454,#26455,#26456,
#26457,#26458,#26459,#26460,#26461,#26462,#26463,#26464,#26465,#26466,#26467,
#26468,#26469,#26470,#26471,#26472,#26473),.UNSPECIFIED.,.F.,.F.,(4,3,3,
3,3,3,3,4),(82.9912312485061,83.7898870578421,84.7873857132926,85.7848843687431,
86.7823830241935,87.779881679644,88.7773803350946,89.2744165556857),
 .UNSPECIFIED.);
#600=B_SPLINE_CURVE_WITH_KNOTS('',3,(#26474,#26475,#26476,#26477,#26478,
#26479,#26480,#26481,#26482,#26483,#26484,#26485,#26486,#26487,#26488,#26489,
#26490,#26491,#26492,#26493,#26494,#26495),.UNSPECIFIED.,.F.,.F.,(4,3,3,
3,3,3,3,4),(-85.5277922570266,-84.7873857132925,-83.789887057842,-82.7923884023915,
-81.794889746941,-80.7973910914905,-79.79989243604,-79.244606949847),
 .UNSPECIFIED.);
#601=B_SPLINE_CURVE_WITH_KNOTS('',3,(#26500,#26501,#26502,#26503,#26504,
#26505,#26506,#26507,#26508,#26509,#26510,#26511,#26512,#26513,#26514,#26515,
#26516,#26517,#26518,#26519,#26520,#26521,#26522,#26523,#26524),
 .UNSPECIFIED.,.F.,.F.,(4,3,3,3,3,3,3,3,4),(76.7080459413264,76.8073964696885,
77.804895125139,78.8023937805895,79.79989243604,80.7973910914905,81.7948897469411,
82.7923884023915,82.9912312485061),.UNSPECIFIED.);
#602=B_SPLINE_CURVE_WITH_KNOTS('',3,(#26525,#26526,#26527,#26528,#26529,
#26530,#26531,#26532,#26533,#26534,#26535,#26536,#26537,#26538,#26539,#26540,
#26541,#26542,#26543,#26544,#26545,#26546),.UNSPECIFIED.,.F.,.F.,(4,3,3,
3,3,3,3,4),(-79.244606949847,-78.8023937805895,-77.804895125139,-76.8073964696885,
-75.809897814238,-74.8123991587875,-73.814900503337,-72.9614216426674),
 .UNSPECIFIED.);
#603=B_SPLINE_CURVE_WITH_KNOTS('',3,(#26551,#26552,#26553,#26554,#26555,
#26556,#26557,#26558,#26559,#26560,#26561,#26562,#26563,#26564,#26565,#26566,
#26567,#26568,#26569,#26570,#26571,#26572),.UNSPECIFIED.,.F.,.F.,(4,3,3,
3,3,3,3,4),(70.4248606341468,70.8224045369855,71.8199031924361,72.8174018478865,
73.814900503337,74.8123991587875,75.809897814238,76.7080459413264),
 .UNSPECIFIED.);
#604=B_SPLINE_CURVE_WITH_KNOTS('',3,(#26573,#26574,#26575,#26576,#26577,
#26578,#26579,#26580,#26581,#26582,#26583,#26584,#26585,#26586,#26587,#26588,
#26589,#26590,#26591,#26592,#26593,#26594,#26595,#26596,#26597),
 .UNSPECIFIED.,.F.,.F.,(4,3,3,3,3,3,3,3,4),(-72.9614216426674,-72.8174018478865,
-71.819903192436,-70.8224045369855,-69.824905881535,-68.8274072260845,-67.829908570634,
-66.8324099151835,-66.6782363354877),.UNSPECIFIED.);
#605=B_SPLINE_CURVE_WITH_KNOTS('',3,(#26602,#26603,#26604,#26605,#26606,
#26607,#26608,#26609,#26610,#26611,#26612,#26613,#26614,#26615,#26616,#26617,
#26618,#26619,#26620,#26621,#26622,#26623),.UNSPECIFIED.,.F.,.F.,(4,3,3,
3,3,3,3,4),(64.1416753269672,64.8374126042825,65.834911259733,66.8324099151835,
67.829908570634,68.8274072260845,69.824905881535,70.4248606341468),
 .UNSPECIFIED.);
#606=B_SPLINE_CURVE_WITH_KNOTS('',3,(#26624,#26625,#26626,#26627,#26628,
#26629,#26630,#26631,#26632,#26633,#26634,#26635,#26636,#26637,#26638,#26639,
#26640,#26641,#26642,#26643,#26644,#26645),.UNSPECIFIED.,.F.,.F.,(4,3,3,
3,3,3,3,4),(-66.6782363354877,-65.834911259733,-64.8374126042825,-63.839913948832,
-62.8424152933815,-61.844916637931,-60.8474179824805,-60.3950510283081),
 .UNSPECIFIED.);
#607=B_SPLINE_CURVE_WITH_KNOTS('',3,(#26650,#26651,#26652,#26653,#26654,
#26655,#26656,#26657,#26658,#26659,#26660,#26661,#26662,#26663,#26664,#26665,
#26666,#26667,#26668,#26669,#26670,#26671),.UNSPECIFIED.,.F.,.F.,(4,3,3,
3,3,3,3,4),(57.8584900197876,58.8524206715795,59.84991932703,60.8474179824805,
61.844916637931,62.8424152933815,63.839913948832,64.1416753269672),
 .UNSPECIFIED.);
#608=B_SPLINE_CURVE_WITH_KNOTS('',3,(#26672,#26673,#26674,#26675,#26676,
#26677,#26678,#26679,#26680,#26681,#26682,#26683,#26684,#26685,#26686,#26687,
#26688,#26689,#26690,#26691,#26692,#26693),.UNSPECIFIED.,.F.,.F.,(4,3,3,
3,3,3,3,4),(-60.3950510283081,-59.84991932703,-58.8524206715795,-57.854922016129,
-56.8574233606785,-55.859924705228,-54.8624260497775,-54.1118657211285),
 .UNSPECIFIED.);
#609=B_SPLINE_CURVE_WITH_KNOTS('',3,(#26698,#26699,#26700,#26701,#26702,
#26703,#26704,#26705,#26706,#26707,#26708,#26709,#26710,#26711,#26712,#26713,
#26714,#26715,#26716,#26717,#26718,#26719,#26720,#26721,#26722),
 .UNSPECIFIED.,.F.,.F.,(4,3,3,3,3,3,3,3,4),(51.5753047126083,51.869930083426,
52.8674287388765,53.864927394327,54.8624260497775,55.859924705228,56.8574233606785,
57.854922016129,57.8584900197876),.UNSPECIFIED.);
#610=B_SPLINE_CURVE_WITH_KNOTS('',3,(#26723,#26724,#26725,#26726,#26727,
#26728,#26729,#26730,#26731,#26732,#26733,#26734,#26735,#26736,#26737,#26738,
#26739,#26740,#26741,#26742,#26743,#26744,#26745,#26746,#26747),
 .UNSPECIFIED.,.F.,.F.,(4,3,3,3,3,3,3,3,4),(-54.1118657211285,-53.864927394327,
-52.8674287388765,-51.869930083426,-50.8724314279755,-49.874932772525,-48.8774341170745,
-47.879935461624,-47.8286804139489),.UNSPECIFIED.);
#611=B_SPLINE_CURVE_WITH_KNOTS('',3,(#26752,#26753,#26754,#26755,#26756,
#26757,#26758,#26759,#26760,#26761,#26762,#26763,#26764,#26765,#26766,#26767,
#26768,#26769,#26770,#26771,#26772,#26773),.UNSPECIFIED.,.F.,.F.,(4,3,3,
3,3,3,3,4),(45.2921194054287,45.884938150723,46.8824368061735,47.879935461624,
48.8774341170745,49.874932772525,50.8724314279755,51.5753047126083),
 .UNSPECIFIED.);
#612=B_SPLINE_CURVE_WITH_KNOTS('',3,(#26774,#26775,#26776,#26777,#26778,
#26779,#26780,#26781,#26782,#26783,#26784,#26785,#26786,#26787,#26788,#26789,
#26790,#26791,#26792,#26793,#26794,#26795),.UNSPECIFIED.,.F.,.F.,(4,3,3,
3,3,3,3,4),(-47.8286804139489,-46.8824368061735,-45.884938150723,-44.8874394952725,
-43.889940839822,-42.8924421843715,-41.894943528921,-41.5454951067693),
 .UNSPECIFIED.);
#613=B_SPLINE_CURVE_WITH_KNOTS('',3,(#26800,#26801,#26802,#26803,#26804,
#26805,#26806,#26807,#26808,#26809,#26810,#26811,#26812,#26813,#26814,#26815,
#26816,#26817,#26818,#26819,#26820,#26821),.UNSPECIFIED.,.F.,.F.,(4,3,3,
3,3,3,3,4),(39.0089340982491,39.89994621802,40.8974448734705,41.894943528921,
42.8924421843715,43.889940839822,44.8874394952725,45.2921194054287),
 .UNSPECIFIED.);
#614=B_SPLINE_CURVE_WITH_KNOTS('',3,(#26822,#26823,#26824,#26825,#26826,
#26827,#26828,#26829,#26830,#26831,#26832,#26833,#26834,#26835,#26836,#26837,
#26838,#26839,#26840,#26841,#26842,#26843),.UNSPECIFIED.,.F.,.F.,(4,3,3,
3,3,3,3,4),(-41.5454951067693,-40.8974448734705,-39.89994621802,-38.9024475625695,
-37.904948907119,-36.9074502516685,-35.909951596218,-35.2623097995897),
 .UNSPECIFIED.);
#615=B_SPLINE_CURVE_WITH_KNOTS('',3,(#26848,#26849,#26850,#26851,#26852,
#26853,#26854,#26855,#26856,#26857,#26858,#26859,#26860,#26861,#26862,#26863,
#26864,#26865,#26866,#26867,#26868,#26869,#26870,#26871,#26872),
 .UNSPECIFIED.,.F.,.F.,(4,3,3,3,3,3,3,3,4),(32.7257487910695,32.9174556298665,
33.914954285317,34.9124529407675,35.909951596218,36.9074502516685,37.904948907119,
38.9024475625695,39.0089340982491),.UNSPECIFIED.);
#616=B_SPLINE_CURVE_WITH_KNOTS('',3,(#26873,#26874,#26875,#26876,#26877,
#26878,#26879,#26880,#26881,#26882,#26883,#26884,#26885,#26886,#26887,#26888,
#26889,#26890,#26891,#26892,#26893,#26894),.UNSPECIFIED.,.F.,.F.,(4,3,3,
3,3,3,3,4),(-35.2623097995897,-34.9124529407675,-33.914954285317,-32.9174556298665,
-31.919956974416,-30.9224583189655,-29.924959663515,-28.9791244924101),
 .UNSPECIFIED.);
#617=B_SPLINE_CURVE_WITH_KNOTS('',3,(#26899,#26900,#26901,#26902,#26903,
#26904,#26905,#26906,#26907,#26908,#26909,#26910,#26911,#26912,#26913,#26914,
#26915,#26916,#26917,#26918,#26919,#26920),.UNSPECIFIED.,.F.,.F.,(4,3,3,
3,3,3,3,4),(26.4425634838898,26.9324636971635,27.929962352614,28.9274610080645,
29.924959663515,30.9224583189655,31.919956974416,32.7257487910695),
 .UNSPECIFIED.);
#618=B_SPLINE_CURVE_WITH_KNOTS('',3,(#26921,#26922,#26923,#26924,#26925,
#26926,#26927,#26928,#26929,#26930,#26931,#26932,#26933,#26934,#26935,#26936,
#26937,#26938,#26939,#26940,#26941,#26942,#26943,#26944,#26945),
 .UNSPECIFIED.,.F.,.F.,(4,3,3,3,3,3,3,3,4),(-28.9791244924101,-28.9274610080645,
-27.929962352614,-26.9324636971635,-25.934965041713,-24.9374663862625,-23.939967730812,
-22.9424690753615,-22.6959391852305),.UNSPECIFIED.);
#619=B_SPLINE_CURVE_WITH_KNOTS('',3,(#26950,#26951,#26952,#26953,#26954,
#26955,#26956,#26957,#26958,#26959,#26960,#26961,#26962,#26963,#26964,#26965,
#26966,#26967,#26968,#26969,#26970,#26971),.UNSPECIFIED.,.F.,.F.,(4,3,3,
3,3,3,3,4),(20.1593781767102,20.9474717644605,21.944970419911,22.9424690753615,
23.939967730812,24.9374663862625,25.934965041713,26.4425634838898),
 .UNSPECIFIED.);
#620=B_SPLINE_CURVE_WITH_KNOTS('',3,(#26972,#26973,#26974,#26975,#26976,
#26977,#26978,#26979,#26980,#26981,#26982,#26983,#26984,#26985,#26986,#26987,
#26988,#26989,#26990,#26991,#26992,#26993),.UNSPECIFIED.,.F.,.F.,(4,3,3,
3,3,3,3,4),(-22.6959391852305,-21.944970419911,-20.9474717644605,-19.94997310901,
-18.9524744535595,-17.954975798109,-16.9574771426585,-16.4127538780512),
 .UNSPECIFIED.);
#621=B_SPLINE_CURVE_WITH_KNOTS('',3,(#26998,#26999,#27000,#27001,#27002,
#27003,#27004,#27005,#27006,#27007,#27008,#27009,#27010,#27011,#27012,#27013,
#27014,#27015,#27016,#27017,#27018,#27019,#27020,#27021,#27022),
 .UNSPECIFIED.,.F.,.F.,(4,3,3,3,3,3,3,3,4),(13.8761928695306,13.964981176307,
14.9624798317575,15.959978487208,16.9574771426585,17.954975798109,18.9524744535595,
19.94997310901,20.1593781767102),.UNSPECIFIED.);
#622=B_SPLINE_CURVE_WITH_KNOTS('',3,(#27023,#27024,#27025,#27026,#27027,
#27028,#27029,#27030,#27031,#27032,#27033,#27034,#27035,#27036,#27037,#27038,
#27039,#27040,#27041,#27042,#27043,#27044),.UNSPECIFIED.,.F.,.F.,(4,3,3,
3,3,3,3,4),(-16.4127538780512,-15.959978487208,-14.9624798317575,-13.964981176307,
-12.9674825208565,-11.969983865406,-10.9724852099555,-10.1295685708716),
 .UNSPECIFIED.);
#623=B_SPLINE_CURVE_WITH_KNOTS('',3,(#27050,#27051,#27052,#27053,#27054,
#27055,#27056,#27057,#27058,#27059,#27060,#27061,#27062),.UNSPECIFIED.,
 .F.,.F.,(4,3,3,3,4),(-3.84638326369194,-2.9924959663515,-1.994997310901,
-0.997498655450502,0.),.UNSPECIFIED.);
#624=B_SPLINE_CURVE_WITH_KNOTS('',3,(#27065,#27066,#27067,#27068,#27069,
#27070,#27071,#27072,#27073,#27074,#27075,#27076,#27077,#27078,#27079,#27080,
#27081,#27082,#27083),.UNSPECIFIED.,.F.,.F.,(4,3,3,3,3,3,4),(2.01461286527449,
2.9924959663515,3.989994621802,4.9874932772525,5.984991932703,6.9824905881535,
7.59300756235101),.UNSPECIFIED.);
#625=B_SPLINE_CURVE_WITH_KNOTS('',3,(#27089,#27090,#27091,#27092,#27093),
 .UNSPECIFIED.,.F.,.F.,(4,1,4),(128.805298797181,129.566421347416,130.563920002867),
 .UNSPECIFIED.);
#626=B_SPLINE_CURVE_WITH_KNOTS('',3,(#27096,#27097,#27098,#27099,#27100,
#27101),.UNSPECIFIED.,.F.,.F.,(4,1,1,4),(128.805298797181,129.110486389585,
130.107985045035,131.085868146112),.UNSPECIFIED.);
#627=B_SPLINE_CURVE_WITH_KNOTS('',3,(#27106,#27107,#27108,#27109,#27110,
#27111,#27112,#27113,#27114,#27115,#27116),.UNSPECIFIED.,.F.,.F.,(4,1,1,
1,1,1,1,1,4),(122.522113490002,122.583930759263,123.581429414713,124.578928070164,
125.576426725614,126.573925381065,127.571424036515,128.568922691966,128.805298797181),
 .UNSPECIFIED.);
#628=B_SPLINE_CURVE_WITH_KNOTS('',3,(#27117,#27118,#27119,#27120,#27121,
#27122,#27123,#27124,#27125,#27126),.UNSPECIFIED.,.F.,.F.,(4,1,1,1,1,1,
1,4),(122.522113490002,123.125494456882,124.122993112332,125.120491767783,
126.117990423233,127.115489078684,128.112987734134,128.805298797181),
 .UNSPECIFIED.);
#629=B_SPLINE_CURVE_WITH_KNOTS('',3,(#27131,#27132,#27133,#27134,#27135,
#27136,#27137,#27138,#27139,#27140),.UNSPECIFIED.,.F.,.F.,(4,1,1,1,1,1,
1,4),(116.238928182822,116.59893882656,117.59643748201,118.593936137461,
119.591434792911,120.588933448362,121.586432103812,122.522113490002),
 .UNSPECIFIED.);
#630=B_SPLINE_CURVE_WITH_KNOTS('',3,(#27141,#27142,#27143,#27144,#27145,
#27146,#27147,#27148,#27149,#27150),.UNSPECIFIED.,.F.,.F.,(4,1,1,1,1,1,
1,4),(116.238928182823,117.140502524179,118.138001179629,119.13549983508,
120.13299849053,121.130497145981,122.127995801431,122.522113490002),
 .UNSPECIFIED.);
#631=B_SPLINE_CURVE_WITH_KNOTS('',3,(#27155,#27156,#27157,#27158,#27159,
#27160,#27161,#27162,#27163,#27164),.UNSPECIFIED.,.F.,.F.,(4,1,1,1,1,1,
1,4),(109.955742875643,110.613946893857,111.611445549307,112.608944204758,
113.606442860208,114.603941515659,115.601440171109,116.238928182822),
 .UNSPECIFIED.);
#632=B_SPLINE_CURVE_WITH_KNOTS('',3,(#27165,#27166,#27167,#27168,#27169,
#27170,#27171,#27172,#27173,#27174,#27175),.UNSPECIFIED.,.F.,.F.,(4,1,1,
1,1,1,1,1,4),(109.955742875643,110.158011936025,111.155510591476,112.153009246926,
113.150507902377,114.148006557827,115.145505213278,116.143003868728,116.238928182823),
 .UNSPECIFIED.);
#633=B_SPLINE_CURVE_WITH_KNOTS('',3,(#27180,#27181,#27182,#27183,#27184,
#27185,#27186,#27187,#27188,#27189),.UNSPECIFIED.,.F.,.F.,(4,1,1,1,1,1,
1,4),(103.672557568463,104.628954961154,105.626453616604,106.623952272055,
107.621450927505,108.618949582956,109.616448238406,109.955742875643),
 .UNSPECIFIED.);
#634=B_SPLINE_CURVE_WITH_KNOTS('',3,(#27190,#27191,#27192,#27193,#27194,
#27195,#27196,#27197,#27198,#27199),.UNSPECIFIED.,.F.,.F.,(4,1,1,1,1,1,
1,4),(103.672557568463,104.173020003322,105.170518658773,106.168017314223,
107.165515969674,108.163014625124,109.160513280575,109.955742875643),
 .UNSPECIFIED.);
#635=B_SPLINE_CURVE_WITH_KNOTS('',3,(#27204,#27205,#27206,#27207,#27208,
#27209,#27210,#27211,#27212,#27213,#27214),.UNSPECIFIED.,.F.,.F.,(4,1,1,
1,1,1,1,1,4),(97.3893722612837,97.646464373,98.6439630284505,99.641461683901,
100.638960339352,101.636458994802,102.633957650253,103.631456305703,103.672557568463),
 .UNSPECIFIED.);
#636=B_SPLINE_CURVE_WITH_KNOTS('',3,(#27215,#27216,#27217,#27218,#27219,
#27220,#27221,#27222,#27223,#27224),.UNSPECIFIED.,.F.,.F.,(4,1,1,1,1,1,
1,4),(97.3893722612837,98.1880280706194,99.1855267260699,100.18302538152,
101.180524036971,102.178022692421,103.175521347872,103.672557568463),
 .UNSPECIFIED.);
#637=B_SPLINE_CURVE_WITH_KNOTS('',3,(#27229,#27230,#27231,#27232,#27233,
#27234,#27235,#27236,#27237,#27238),.UNSPECIFIED.,.F.,.F.,(4,1,1,1,1,1,
1,4),(91.106186954104,91.661472440297,92.6589710957475,93.656469751198,
94.6539684066485,95.651467062099,96.6489657175495,97.3893722612837),
 .UNSPECIFIED.);
#638=B_SPLINE_CURVE_WITH_KNOTS('',3,(#27239,#27240,#27241,#27242,#27243,
#27244,#27245,#27246,#27247,#27248,#27249),.UNSPECIFIED.,.F.,.F.,(4,1,1,
1,1,1,1,1,4),(91.106186954104,91.2055374824659,92.2030361379164,93.2005347933669,
94.1980334488174,95.1955321042679,96.1930307597184,97.1905294151689,97.3893722612837),
 .UNSPECIFIED.);
#639=B_SPLINE_CURVE_WITH_KNOTS('',3,(#27254,#27255,#27256,#27257,#27258,
#27259,#27260,#27261,#27262,#27263),.UNSPECIFIED.,.F.,.F.,(4,1,1,1,1,1,
1,4),(84.8230016469245,85.676480507594,86.6739791630445,87.671477818495,
88.6689764739455,89.666475129396,90.6639737848465,91.106186954104),
 .UNSPECIFIED.);
#640=B_SPLINE_CURVE_WITH_KNOTS('',3,(#27264,#27265,#27266,#27267,#27268,
#27269,#27270,#27271,#27272,#27273),.UNSPECIFIED.,.F.,.F.,(4,1,1,1,1,1,
1,4),(84.8230016469245,85.2205455497629,86.2180442052134,87.2155428606639,
88.2130415161144,89.2105401715649,90.2080388270154,91.106186954104),
 .UNSPECIFIED.);
#641=B_SPLINE_CURVE_WITH_KNOTS('',3,(#27278,#27279,#27280,#27281,#27282,
#27283,#27284,#27285,#27286,#27287,#27288),.UNSPECIFIED.,.F.,.F.,(4,1,1,
1,1,1,1,1,4),(78.5398163397448,78.6939899194405,79.691488574891,80.6889872303415,
81.686485885792,82.6839845412425,83.681483196693,84.6789818521435,84.8230016469245),
 .UNSPECIFIED.);
#642=B_SPLINE_CURVE_WITH_KNOTS('',3,(#27289,#27290,#27291,#27292,#27293,
#27294,#27295,#27296,#27297,#27298),.UNSPECIFIED.,.F.,.F.,(4,1,1,1,1,1,
1,4),(78.5398163397448,79.2355536170598,80.2330522725103,81.2305509279608,
82.2280495834113,83.2255482388618,84.2230468943123,84.8230016469245),
 .UNSPECIFIED.);
#643=B_SPLINE_CURVE_WITH_KNOTS('',3,(#27303,#27304,#27305,#27306,#27307,
#27308,#27309,#27310,#27311,#27312),.UNSPECIFIED.,.F.,.F.,(4,1,1,1,1,1,
1,4),(72.2566310325652,72.7089979867375,73.706496642188,74.7039952976385,
75.701493953089,76.6989926085395,77.69649126399,78.5398163397448),
 .UNSPECIFIED.);
#644=B_SPLINE_CURVE_WITH_KNOTS('',3,(#27313,#27314,#27315,#27316,#27317,
#27318,#27319,#27320,#27321,#27322),.UNSPECIFIED.,.F.,.F.,(4,1,1,1,1,1,
1,4),(72.2566310325652,73.2505616843569,74.2480603398074,75.2455589952579,
76.2430576507084,77.2405563061589,78.2380549616094,78.5398163397448),
 .UNSPECIFIED.);
#645=B_SPLINE_CURVE_WITH_KNOTS('',3,(#27327,#27328,#27329,#27330,#27331,
#27332,#27333,#27334,#27335,#27336),.UNSPECIFIED.,.F.,.F.,(4,1,1,1,1,1,
1,4),(65.9734457253856,66.7240060540345,67.721504709485,68.7190033649355,
69.716502020386,70.7140006758365,71.711499331287,72.2566310325652),
 .UNSPECIFIED.);
#646=B_SPLINE_CURVE_WITH_KNOTS('',3,(#27337,#27338,#27339,#27340,#27341,
#27342,#27343,#27344,#27345,#27346,#27347),.UNSPECIFIED.,.F.,.F.,(4,1,1,
1,1,1,1,1,4),(65.9734457253856,66.2680710962033,67.2655697516538,68.2630684071043,
69.2605670625549,70.2580657180054,71.2555643734559,72.2530630289064,72.2566310325652),
 .UNSPECIFIED.);
#647=B_SPLINE_CURVE_WITH_KNOTS('',3,(#27352,#27353,#27354,#27355,#27356,
#27357,#27358,#27359,#27360,#27361,#27362),.UNSPECIFIED.,.F.,.F.,(4,1,1,
1,1,1,1,1,4),(59.690260418206,59.741515465881,60.7390141213315,61.736512776782,
62.7340114322325,63.731510087683,64.7290087431335,65.726507398584,65.9734457253856),
 .UNSPECIFIED.);
#648=B_SPLINE_CURVE_WITH_KNOTS('',3,(#27363,#27364,#27365,#27366,#27367,
#27368,#27369,#27370,#27371,#27372),.UNSPECIFIED.,.F.,.F.,(4,1,1,1,1,1,
1,4),(59.690260418206,60.2830791635003,61.2805778189508,62.2780764744013,
63.2755751298518,64.2730737853023,65.2705724407528,65.9734457253856),
 .UNSPECIFIED.);
#649=B_SPLINE_CURVE_WITH_KNOTS('',3,(#27377,#27378,#27379,#27380,#27381,
#27382,#27383,#27384,#27385,#27386),.UNSPECIFIED.,.F.,.F.,(4,1,1,1,1,1,
1,4),(53.4070751110264,53.756523533178,54.7540221886285,55.751520844079,
56.7490194995295,57.74651815498,58.7440168104305,59.690260418206),
 .UNSPECIFIED.);
#650=B_SPLINE_CURVE_WITH_KNOTS('',3,(#27387,#27388,#27389,#27390,#27391,
#27392,#27393,#27394,#27395,#27396),.UNSPECIFIED.,.F.,.F.,(4,1,1,1,1,1,
1,4),(53.4070751110264,54.2980872307973,55.2955858862478,56.2930845416983,
57.2905831971488,58.2880818525993,59.2855805080498,59.690260418206),
 .UNSPECIFIED.);
#651=B_SPLINE_CURVE_WITH_KNOTS('',3,(#27401,#27402,#27403,#27404,#27405,
#27406,#27407,#27408,#27409,#27410),.UNSPECIFIED.,.F.,.F.,(4,1,1,1,1,1,
1,4),(47.1238898038468,47.771531600475,48.7690302559255,49.766528911376,
50.7640275668265,51.761526222277,52.7590248777275,53.4070751110264),
 .UNSPECIFIED.);
#652=B_SPLINE_CURVE_WITH_KNOTS('',3,(#27411,#27412,#27413,#27414,#27415,
#27416,#27417,#27418,#27419,#27420,#27421),.UNSPECIFIED.,.F.,.F.,(4,1,1,
1,1,1,1,1,4),(47.1238898038468,47.3155966426438,48.3130952980943,49.3105939535448,
50.3080926089953,51.3055912644458,52.3030899198963,53.3005885753468,53.4070751110264),
 .UNSPECIFIED.);
#653=B_SPLINE_CURVE_WITH_KNOTS('',3,(#27426,#27427,#27428,#27429,#27430,
#27431,#27432,#27433,#27434,#27435),.UNSPECIFIED.,.F.,.F.,(4,1,1,1,1,1,
1,4),(40.8407044966672,41.786539667772,42.7840383232225,43.781536978673,
44.7790356341235,45.776534289574,46.7740329450245,47.1238898038468),
 .UNSPECIFIED.);
#654=B_SPLINE_CURVE_WITH_KNOTS('',3,(#27436,#27437,#27438,#27439,#27440,
#27441,#27442,#27443,#27444,#27445),.UNSPECIFIED.,.F.,.F.,(4,1,1,1,1,1,
1,4),(40.8407044966672,41.3306047099408,42.3281033653913,43.3256020208418,
44.3231006762923,45.3205993317428,46.3180979871933,47.1238898038468),
 .UNSPECIFIED.);
#655=B_SPLINE_CURVE_WITH_KNOTS('',3,(#27450,#27451,#27452,#27453,#27454,
#27455,#27456,#27457,#27458,#27459,#27460),.UNSPECIFIED.,.F.,.F.,(4,1,1,
1,1,1,1,1,4),(34.5575191894876,34.8040490796185,35.801547735069,36.7990463905195,
37.79654504597,38.7940437014205,39.791542356871,40.7890410123215,40.8407044966672),
 .UNSPECIFIED.);
#656=B_SPLINE_CURVE_WITH_KNOTS('',3,(#27461,#27462,#27463,#27464,#27465,
#27466,#27467,#27468,#27469,#27470),.UNSPECIFIED.,.F.,.F.,(4,1,1,1,1,1,
1,4),(34.5575191894876,35.3456127772378,36.3431114326883,37.3406100881388,
38.3381087435893,39.3356073990398,40.3331060544903,40.8407044966672),
 .UNSPECIFIED.);
#657=B_SPLINE_CURVE_WITH_KNOTS('',3,(#27475,#27476,#27477,#27478,#27479,
#27480,#27481,#27482,#27483,#27484),.UNSPECIFIED.,.F.,.F.,(4,1,1,1,1,1,
1,4),(28.2743338823079,28.8190571469155,29.816555802366,30.8140544578165,
31.811553113267,32.8090517687175,33.806550424168,34.5575191894876),
 .UNSPECIFIED.);
#658=B_SPLINE_CURVE_WITH_KNOTS('',3,(#27485,#27486,#27487,#27488,#27489,
#27490,#27491,#27492,#27493,#27494,#27495),.UNSPECIFIED.,.F.,.F.,(4,1,1,
1,1,1,1,1,4),(28.2743338823079,28.3631221890843,29.3606208445348,30.3581194999853,
31.3556181554358,32.3531168108863,33.3506154663368,34.3481141217873,34.5575191894876),
 .UNSPECIFIED.);
#659=B_SPLINE_CURVE_WITH_KNOTS('',3,(#27500,#27501,#27502,#27503,#27504,
#27505,#27506,#27507,#27508,#27509),.UNSPECIFIED.,.F.,.F.,(4,1,1,1,1,1,
1,4),(21.9911485751283,22.8340652142125,23.831563869663,24.8290625251135,
25.826561180564,26.8240598360145,27.821558491465,28.2743338823079),
 .UNSPECIFIED.);
#660=B_SPLINE_CURVE_WITH_KNOTS('',3,(#27510,#27511,#27512,#27513,#27514,
#27515,#27516,#27517,#27518,#27519),.UNSPECIFIED.,.F.,.F.,(4,1,1,1,1,1,
1,4),(21.9911485751283,22.3781302563813,23.3756289118318,24.3731275672823,
25.3706262227328,26.3681248781833,27.3656235336338,28.2743338823079),
 .UNSPECIFIED.);
#661=B_SPLINE_CURVE_WITH_KNOTS('',3,(#27525,#27526,#27527,#27528,#27529),
 .UNSPECIFIED.,.F.,.F.,(4,1,4),(14.3981410127773,15.3956396682278,15.707963267949),
 .UNSPECIFIED.);
#662=B_SPLINE_CURVE_WITH_KNOTS('',3,(#27532,#27533,#27534,#27535,#27536),
 .UNSPECIFIED.,.F.,.F.,(4,1,4),(13.8761928695316,14.8540759706085,15.707963267949),
 .UNSPECIFIED.);
#663=B_SPLINE_CURVE_WITH_KNOTS('',3,(#27542,#27543,#27544,#27545,#27546,
#27547,#27548,#27549,#27550,#27551,#27552,#27553,#27554,#27555,#27556,#27557),
 .UNSPECIFIED.,.F.,.F.,(4,3,3,3,3,4),(114.407157784404,114.712345376808,
115.709844032258,116.707342687709,117.704841343159,118.702339998609),
 .UNSPECIFIED.);
#664=B_SPLINE_CURVE_WITH_KNOTS('',3,(#27565,#27566,#27567,#27568,#27569,
#27570,#27571,#27572,#27573,#27574,#27575,#27576,#27577,#27578,#27579,#27580,
#27581,#27582,#27583,#27584,#27585,#27586),.UNSPECIFIED.,.F.,.F.,(4,3,3,
3,3,3,3,4),(-116.687727133335,-115.709844032258,-114.712345376808,-113.714846721357,
-112.717348065907,-111.719849410456,-110.722350755006,-110.660533485745),
 .UNSPECIFIED.);
#665=B_SPLINE_CURVE_WITH_KNOTS('',3,(#27591,#27592,#27593,#27594,#27595,
#27596,#27597,#27598,#27599,#27600,#27601,#27602,#27603,#27604,#27605,#27606,
#27607,#27608,#27609,#27610,#27611,#27612),.UNSPECIFIED.,.F.,.F.,(4,3,3,
3,3,3,3,4),(108.123972477224,108.727353444105,109.724852099555,110.722350755006,
111.719849410456,112.717348065907,113.714846721357,114.407157784404),
 .UNSPECIFIED.);
#666=B_SPLINE_CURVE_WITH_KNOTS('',3,(#27613,#27614,#27615,#27616,#27617,
#27618,#27619,#27620,#27621,#27622,#27623,#27624,#27625,#27626,#27627,#27628,
#27629,#27630,#27631,#27632,#27633,#27634),.UNSPECIFIED.,.F.,.F.,(4,3,3,
3,3,3,3,4),(-110.660533485745,-109.724852099555,-108.727353444105,-107.729854788654,
-106.732356133204,-105.734857477753,-104.737358822303,-104.377348178565),
 .UNSPECIFIED.);
#667=B_SPLINE_CURVE_WITH_KNOTS('',3,(#27639,#27640,#27641,#27642,#27643,
#27644,#27645,#27646,#27647,#27648,#27649,#27650,#27651,#27652,#27653,#27654,
#27655,#27656,#27657,#27658,#27659,#27660),.UNSPECIFIED.,.F.,.F.,(4,3,3,
3,3,3,3,4),(101.840787170045,102.742361511402,103.739860166852,104.737358822303,
105.734857477753,106.732356133204,107.729854788654,108.123972477224),
 .UNSPECIFIED.);
#668=B_SPLINE_CURVE_WITH_KNOTS('',3,(#27661,#27662,#27663,#27664,#27665,
#27666,#27667,#27668,#27669,#27670,#27671,#27672,#27673,#27674,#27675,#27676,
#27677,#27678,#27679,#27680,#27681,#27682),.UNSPECIFIED.,.F.,.F.,(4,3,3,
3,3,3,3,4),(-104.377348178565,-103.739860166852,-102.742361511402,-101.744862855951,
-100.747364200501,-99.74986554505,-98.7523668895995,-98.0941628713858),
 .UNSPECIFIED.);
#669=B_SPLINE_CURVE_WITH_KNOTS('',3,(#27687,#27688,#27689,#27690,#27691,
#27692,#27693,#27694,#27695,#27696,#27697,#27698,#27699,#27700,#27701,#27702,
#27703,#27704,#27705,#27706,#27707,#27708,#27709,#27710,#27711),
 .UNSPECIFIED.,.F.,.F.,(4,3,3,3,3,3,3,3,4),(95.5576018628653,95.759870923248,
96.7573695786985,97.754868234149,98.7523668895996,99.7498655450501,100.747364200501,
101.744862855951,101.840787170045),.UNSPECIFIED.);
#670=B_SPLINE_CURVE_WITH_KNOTS('',3,(#27712,#27713,#27714,#27715,#27716,
#27717,#27718,#27719,#27720,#27721,#27722,#27723,#27724,#27725,#27726,#27727,
#27728,#27729,#27730,#27731,#27732,#27733),.UNSPECIFIED.,.F.,.F.,(4,3,3,
3,3,3,3,4),(-98.0941628713858,-97.754868234149,-96.7573695786985,-95.759870923248,
-94.7623722677975,-93.764873612347,-92.7673749568965,-91.8109775642062),
 .UNSPECIFIED.);
#671=B_SPLINE_CURVE_WITH_KNOTS('',3,(#27738,#27739,#27740,#27741,#27742,
#27743,#27744,#27745,#27746,#27747,#27748,#27749,#27750,#27751,#27752,#27753,
#27754,#27755,#27756,#27757,#27758,#27759),.UNSPECIFIED.,.F.,.F.,(4,3,3,
3,3,3,3,4),(89.2744165556857,89.774878990545,90.7723776459955,91.769876301446,
92.7673749568965,93.764873612347,94.7623722677975,95.5576018628653),
 .UNSPECIFIED.);
#672=B_SPLINE_CURVE_WITH_KNOTS('',3,(#27760,#27761,#27762,#27763,#27764,
#27765,#27766,#27767,#27768,#27769,#27770,#27771,#27772,#27773,#27774,#27775,
#27776,#27777,#27778,#27779,#27780,#27781,#27782,#27783,#27784),
 .UNSPECIFIED.,.F.,.F.,(4,3,3,3,3,3,3,3,4),(-91.8109775642062,-91.769876301446,
-90.7723776459955,-89.774878990545,-88.7773803350945,-87.779881679644,-86.7823830241935,
-85.784884368743,-85.5277922570266),.UNSPECIFIED.);
#673=B_SPLINE_CURVE_WITH_KNOTS('',3,(#27789,#27790,#27791,#27792,#27793,
#27794,#27795,#27796,#27797,#27798,#27799,#27800,#27801,#27802,#27803,#27804,
#27805,#27806,#27807,#27808,#27809,#27810),.UNSPECIFIED.,.F.,.F.,(4,3,3,
3,3,3,3,4),(82.9912312485061,83.7898870578421,84.7873857132926,85.7848843687431,
86.7823830241935,87.779881679644,88.7773803350946,89.2744165556857),
 .UNSPECIFIED.);
#674=B_SPLINE_CURVE_WITH_KNOTS('',3,(#27811,#27812,#27813,#27814,#27815,
#27816,#27817,#27818,#27819,#27820,#27821,#27822,#27823,#27824,#27825,#27826,
#27827,#27828,#27829,#27830,#27831,#27832),.UNSPECIFIED.,.F.,.F.,(4,3,3,
3,3,3,3,4),(-85.5277922570266,-84.7873857132925,-83.789887057842,-82.7923884023915,
-81.794889746941,-80.7973910914905,-79.79989243604,-79.244606949847),
 .UNSPECIFIED.);
#675=B_SPLINE_CURVE_WITH_KNOTS('',3,(#27837,#27838,#27839,#27840,#27841,
#27842,#27843,#27844,#27845,#27846,#27847,#27848,#27849,#27850,#27851,#27852,
#27853,#27854,#27855,#27856,#27857,#27858,#27859,#27860,#27861),
 .UNSPECIFIED.,.F.,.F.,(4,3,3,3,3,3,3,3,4),(76.7080459413264,76.8073964696885,
77.804895125139,78.8023937805895,79.79989243604,80.7973910914905,81.7948897469411,
82.7923884023915,82.9912312485061),.UNSPECIFIED.);
#676=B_SPLINE_CURVE_WITH_KNOTS('',3,(#27862,#27863,#27864,#27865,#27866,
#27867,#27868,#27869,#27870,#27871,#27872,#27873,#27874,#27875,#27876,#27877,
#27878,#27879,#27880,#27881,#27882,#27883),.UNSPECIFIED.,.F.,.F.,(4,3,3,
3,3,3,3,4),(-79.244606949847,-78.8023937805895,-77.804895125139,-76.8073964696885,
-75.809897814238,-74.8123991587875,-73.814900503337,-72.9614216426674),
 .UNSPECIFIED.);
#677=B_SPLINE_CURVE_WITH_KNOTS('',3,(#27888,#27889,#27890,#27891,#27892,
#27893,#27894,#27895,#27896,#27897,#27898,#27899,#27900,#27901,#27902,#27903,
#27904,#27905,#27906,#27907,#27908,#27909),.UNSPECIFIED.,.F.,.F.,(4,3,3,
3,3,3,3,4),(70.4248606341468,70.8224045369855,71.8199031924361,72.8174018478865,
73.814900503337,74.8123991587875,75.809897814238,76.7080459413264),
 .UNSPECIFIED.);
#678=B_SPLINE_CURVE_WITH_KNOTS('',3,(#27910,#27911,#27912,#27913,#27914,
#27915,#27916,#27917,#27918,#27919,#27920,#27921,#27922,#27923,#27924,#27925,
#27926,#27927,#27928,#27929,#27930,#27931,#27932,#27933,#27934),
 .UNSPECIFIED.,.F.,.F.,(4,3,3,3,3,3,3,3,4),(-72.9614216426674,-72.8174018478865,
-71.819903192436,-70.8224045369855,-69.824905881535,-68.8274072260845,-67.829908570634,
-66.8324099151835,-66.6782363354877),.UNSPECIFIED.);
#679=B_SPLINE_CURVE_WITH_KNOTS('',3,(#27939,#27940,#27941,#27942,#27943,
#27944,#27945,#27946,#27947,#27948,#27949,#27950,#27951,#27952,#27953,#27954,
#27955,#27956,#27957,#27958,#27959,#27960),.UNSPECIFIED.,.F.,.F.,(4,3,3,
3,3,3,3,4),(64.1416753269672,64.8374126042825,65.834911259733,66.8324099151835,
67.829908570634,68.8274072260845,69.824905881535,70.4248606341468),
 .UNSPECIFIED.);
#680=B_SPLINE_CURVE_WITH_KNOTS('',3,(#27961,#27962,#27963,#27964,#27965,
#27966,#27967,#27968,#27969,#27970,#27971,#27972,#27973,#27974,#27975,#27976,
#27977,#27978,#27979,#27980,#27981,#27982),.UNSPECIFIED.,.F.,.F.,(4,3,3,
3,3,3,3,4),(-66.6782363354877,-65.834911259733,-64.8374126042825,-63.839913948832,
-62.8424152933815,-61.844916637931,-60.8474179824805,-60.3950510283081),
 .UNSPECIFIED.);
#681=B_SPLINE_CURVE_WITH_KNOTS('',3,(#27987,#27988,#27989,#27990,#27991,
#27992,#27993,#27994,#27995,#27996,#27997,#27998,#27999,#28000,#28001,#28002,
#28003,#28004,#28005,#28006,#28007,#28008),.UNSPECIFIED.,.F.,.F.,(4,3,3,
3,3,3,3,4),(57.8584900197876,58.8524206715795,59.84991932703,60.8474179824805,
61.844916637931,62.8424152933815,63.839913948832,64.1416753269672),
 .UNSPECIFIED.);
#682=B_SPLINE_CURVE_WITH_KNOTS('',3,(#28009,#28010,#28011,#28012,#28013,
#28014,#28015,#28016,#28017,#28018,#28019,#28020,#28021,#28022,#28023,#28024,
#28025,#28026,#28027,#28028,#28029,#28030),.UNSPECIFIED.,.F.,.F.,(4,3,3,
3,3,3,3,4),(-60.3950510283081,-59.84991932703,-58.8524206715795,-57.854922016129,
-56.8574233606785,-55.859924705228,-54.8624260497775,-54.1118657211285),
 .UNSPECIFIED.);
#683=B_SPLINE_CURVE_WITH_KNOTS('',3,(#28035,#28036,#28037,#28038,#28039,
#28040,#28041,#28042,#28043,#28044,#28045,#28046,#28047,#28048,#28049,#28050,
#28051,#28052,#28053,#28054,#28055,#28056,#28057,#28058,#28059),
 .UNSPECIFIED.,.F.,.F.,(4,3,3,3,3,3,3,3,4),(51.5753047126083,51.869930083426,
52.8674287388765,53.864927394327,54.8624260497775,55.859924705228,56.8574233606785,
57.854922016129,57.8584900197876),.UNSPECIFIED.);
#684=B_SPLINE_CURVE_WITH_KNOTS('',3,(#28060,#28061,#28062,#28063,#28064,
#28065,#28066,#28067,#28068,#28069,#28070,#28071,#28072,#28073,#28074,#28075,
#28076,#28077,#28078,#28079,#28080,#28081,#28082,#28083,#28084),
 .UNSPECIFIED.,.F.,.F.,(4,3,3,3,3,3,3,3,4),(-54.1118657211285,-53.864927394327,
-52.8674287388765,-51.869930083426,-50.8724314279755,-49.874932772525,-48.8774341170745,
-47.879935461624,-47.8286804139489),.UNSPECIFIED.);
#685=B_SPLINE_CURVE_WITH_KNOTS('',3,(#28089,#28090,#28091,#28092,#28093,
#28094,#28095,#28096,#28097,#28098,#28099,#28100,#28101,#28102,#28103,#28104,
#28105,#28106,#28107,#28108,#28109,#28110),.UNSPECIFIED.,.F.,.F.,(4,3,3,
3,3,3,3,4),(45.2921194054287,45.884938150723,46.8824368061735,47.879935461624,
48.8774341170745,49.874932772525,50.8724314279755,51.5753047126083),
 .UNSPECIFIED.);
#686=B_SPLINE_CURVE_WITH_KNOTS('',3,(#28111,#28112,#28113,#28114,#28115,
#28116,#28117,#28118,#28119,#28120,#28121,#28122,#28123,#28124,#28125,#28126,
#28127,#28128,#28129,#28130,#28131,#28132),.UNSPECIFIED.,.F.,.F.,(4,3,3,
3,3,3,3,4),(-47.8286804139489,-46.8824368061735,-45.884938150723,-44.8874394952725,
-43.889940839822,-42.8924421843715,-41.894943528921,-41.5454951067693),
 .UNSPECIFIED.);
#687=B_SPLINE_CURVE_WITH_KNOTS('',3,(#28137,#28138,#28139,#28140,#28141,
#28142,#28143,#28144,#28145,#28146,#28147,#28148,#28149,#28150,#28151,#28152,
#28153,#28154,#28155,#28156,#28157,#28158),.UNSPECIFIED.,.F.,.F.,(4,3,3,
3,3,3,3,4),(39.0089340982491,39.89994621802,40.8974448734705,41.894943528921,
42.8924421843715,43.889940839822,44.8874394952725,45.2921194054287),
 .UNSPECIFIED.);
#688=B_SPLINE_CURVE_WITH_KNOTS('',3,(#28159,#28160,#28161,#28162,#28163,
#28164,#28165,#28166,#28167,#28168,#28169,#28170,#28171,#28172,#28173,#28174,
#28175,#28176,#28177,#28178,#28179,#28180),.UNSPECIFIED.,.F.,.F.,(4,3,3,
3,3,3,3,4),(-41.5454951067693,-40.8974448734705,-39.89994621802,-38.9024475625695,
-37.904948907119,-36.9074502516685,-35.909951596218,-35.2623097995897),
 .UNSPECIFIED.);
#689=B_SPLINE_CURVE_WITH_KNOTS('',3,(#28185,#28186,#28187,#28188,#28189,
#28190,#28191,#28192,#28193,#28194,#28195,#28196,#28197,#28198,#28199,#28200,
#28201,#28202,#28203,#28204,#28205,#28206,#28207,#28208,#28209),
 .UNSPECIFIED.,.F.,.F.,(4,3,3,3,3,3,3,3,4),(32.7257487910695,32.9174556298665,
33.914954285317,34.9124529407675,35.909951596218,36.9074502516685,37.904948907119,
38.9024475625695,39.0089340982491),.UNSPECIFIED.);
#690=B_SPLINE_CURVE_WITH_KNOTS('',3,(#28210,#28211,#28212,#28213,#28214,
#28215,#28216,#28217,#28218,#28219,#28220,#28221,#28222,#28223,#28224,#28225,
#28226,#28227,#28228,#28229,#28230,#28231),.UNSPECIFIED.,.F.,.F.,(4,3,3,
3,3,3,3,4),(-35.2623097995897,-34.9124529407675,-33.914954285317,-32.9174556298665,
-31.919956974416,-30.9224583189655,-29.924959663515,-28.9791244924101),
 .UNSPECIFIED.);
#691=B_SPLINE_CURVE_WITH_KNOTS('',3,(#28236,#28237,#28238,#28239,#28240,
#28241,#28242,#28243,#28244,#28245,#28246,#28247,#28248,#28249,#28250,#28251,
#28252,#28253,#28254,#28255,#28256,#28257),.UNSPECIFIED.,.F.,.F.,(4,3,3,
3,3,3,3,4),(26.4425634838898,26.9324636971635,27.929962352614,28.9274610080645,
29.924959663515,30.9224583189655,31.919956974416,32.7257487910695),
 .UNSPECIFIED.);
#692=B_SPLINE_CURVE_WITH_KNOTS('',3,(#28258,#28259,#28260,#28261,#28262,
#28263,#28264,#28265,#28266,#28267,#28268,#28269,#28270,#28271,#28272,#28273,
#28274,#28275,#28276,#28277,#28278,#28279,#28280,#28281,#28282),
 .UNSPECIFIED.,.F.,.F.,(4,3,3,3,3,3,3,3,4),(-28.9791244924101,-28.9274610080645,
-27.929962352614,-26.9324636971635,-25.934965041713,-24.9374663862625,-23.939967730812,
-22.9424690753615,-22.6959391852305),.UNSPECIFIED.);
#693=B_SPLINE_CURVE_WITH_KNOTS('',3,(#28287,#28288,#28289,#28290,#28291,
#28292,#28293,#28294,#28295,#28296,#28297,#28298,#28299,#28300,#28301,#28302,
#28303,#28304,#28305,#28306,#28307,#28308),.UNSPECIFIED.,.F.,.F.,(4,3,3,
3,3,3,3,4),(20.1593781767102,20.9474717644605,21.944970419911,22.9424690753615,
23.939967730812,24.9374663862625,25.934965041713,26.4425634838898),
 .UNSPECIFIED.);
#694=B_SPLINE_CURVE_WITH_KNOTS('',3,(#28309,#28310,#28311,#28312,#28313,
#28314,#28315,#28316,#28317,#28318,#28319,#28320,#28321,#28322,#28323,#28324,
#28325,#28326,#28327,#28328,#28329,#28330),.UNSPECIFIED.,.F.,.F.,(4,3,3,
3,3,3,3,4),(-22.6959391852305,-21.944970419911,-20.9474717644605,-19.94997310901,
-18.9524744535595,-17.954975798109,-16.9574771426585,-16.4127538780512),
 .UNSPECIFIED.);
#695=B_SPLINE_CURVE_WITH_KNOTS('',3,(#28335,#28336,#28337,#28338,#28339,
#28340,#28341,#28342,#28343,#28344,#28345,#28346,#28347,#28348,#28349,#28350,
#28351,#28352,#28353,#28354,#28355,#28356,#28357,#28358,#28359),
 .UNSPECIFIED.,.F.,.F.,(4,3,3,3,3,3,3,3,4),(13.8761928695306,13.964981176307,
14.9624798317575,15.959978487208,16.9574771426585,17.954975798109,18.9524744535595,
19.94997310901,20.1593781767102),.UNSPECIFIED.);
#696=B_SPLINE_CURVE_WITH_KNOTS('',3,(#28360,#28361,#28362,#28363,#28364,
#28365,#28366,#28367,#28368,#28369,#28370,#28371,#28372,#28373,#28374,#28375,
#28376,#28377,#28378,#28379,#28380,#28381),.UNSPECIFIED.,.F.,.F.,(4,3,3,
3,3,3,3,4),(-16.4127538780512,-15.959978487208,-14.9624798317575,-13.964981176307,
-12.9674825208565,-11.969983865406,-10.9724852099555,-10.1295685708716),
 .UNSPECIFIED.);
#697=B_SPLINE_CURVE_WITH_KNOTS('',3,(#28387,#28388,#28389,#28390,#28391,
#28392,#28393,#28394,#28395,#28396,#28397,#28398,#28399),.UNSPECIFIED.,
 .F.,.F.,(4,3,3,3,4),(-3.84638326369194,-2.9924959663515,-1.994997310901,
-0.997498655450501,0.),.UNSPECIFIED.);
#698=B_SPLINE_CURVE_WITH_KNOTS('',3,(#28402,#28403,#28404,#28405,#28406,
#28407,#28408,#28409,#28410,#28411,#28412,#28413,#28414,#28415,#28416,#28417,
#28418,#28419,#28420),.UNSPECIFIED.,.F.,.F.,(4,3,3,3,3,3,4),(2.01461286527449,
2.9924959663515,3.989994621802,4.9874932772525,5.984991932703,6.9824905881535,
7.59300756235101),.UNSPECIFIED.);
#699=B_SPLINE_CURVE_WITH_KNOTS('',3,(#28426,#28427,#28428,#28429,#28430),
 .UNSPECIFIED.,.F.,.F.,(4,1,4),(128.805298797181,129.566421347416,130.563920002867),
 .UNSPECIFIED.);
#700=B_SPLINE_CURVE_WITH_KNOTS('',3,(#28433,#28434,#28435,#28436,#28437,
#28438),.UNSPECIFIED.,.F.,.F.,(4,1,1,4),(128.805298797181,129.110486389585,
130.107985045035,131.085868146112),.UNSPECIFIED.);
#701=B_SPLINE_CURVE_WITH_KNOTS('',3,(#28443,#28444,#28445,#28446,#28447,
#28448,#28449,#28450,#28451,#28452,#28453),.UNSPECIFIED.,.F.,.F.,(4,1,1,
1,1,1,1,1,4),(122.522113490002,122.583930759263,123.581429414713,124.578928070164,
125.576426725614,126.573925381065,127.571424036515,128.568922691966,128.805298797181),
 .UNSPECIFIED.);
#702=B_SPLINE_CURVE_WITH_KNOTS('',3,(#28454,#28455,#28456,#28457,#28458,
#28459,#28460,#28461,#28462,#28463),.UNSPECIFIED.,.F.,.F.,(4,1,1,1,1,1,
1,4),(122.522113490002,123.125494456882,124.122993112332,125.120491767783,
126.117990423233,127.115489078684,128.112987734134,128.805298797181),
 .UNSPECIFIED.);
#703=B_SPLINE_CURVE_WITH_KNOTS('',3,(#28468,#28469,#28470,#28471,#28472,
#28473,#28474,#28475,#28476,#28477),.UNSPECIFIED.,.F.,.F.,(4,1,1,1,1,1,
1,4),(116.238928182822,116.59893882656,117.59643748201,118.593936137461,
119.591434792911,120.588933448362,121.586432103812,122.522113490002),
 .UNSPECIFIED.);
#704=B_SPLINE_CURVE_WITH_KNOTS('',3,(#28478,#28479,#28480,#28481,#28482,
#28483,#28484,#28485,#28486,#28487),.UNSPECIFIED.,.F.,.F.,(4,1,1,1,1,1,
1,4),(116.238928182823,117.140502524179,118.138001179629,119.13549983508,
120.13299849053,121.130497145981,122.127995801431,122.522113490002),
 .UNSPECIFIED.);
#705=B_SPLINE_CURVE_WITH_KNOTS('',3,(#28492,#28493,#28494,#28495,#28496,
#28497,#28498,#28499,#28500,#28501),.UNSPECIFIED.,.F.,.F.,(4,1,1,1,1,1,
1,4),(109.955742875643,110.613946893857,111.611445549307,112.608944204758,
113.606442860208,114.603941515659,115.601440171109,116.238928182822),
 .UNSPECIFIED.);
#706=B_SPLINE_CURVE_WITH_KNOTS('',3,(#28502,#28503,#28504,#28505,#28506,
#28507,#28508,#28509,#28510,#28511,#28512),.UNSPECIFIED.,.F.,.F.,(4,1,1,
1,1,1,1,1,4),(109.955742875643,110.158011936025,111.155510591476,112.153009246926,
113.150507902377,114.148006557827,115.145505213278,116.143003868728,116.238928182823),
 .UNSPECIFIED.);
#707=B_SPLINE_CURVE_WITH_KNOTS('',3,(#28517,#28518,#28519,#28520,#28521,
#28522,#28523,#28524,#28525,#28526),.UNSPECIFIED.,.F.,.F.,(4,1,1,1,1,1,
1,4),(103.672557568463,104.628954961154,105.626453616604,106.623952272055,
107.621450927505,108.618949582956,109.616448238406,109.955742875643),
 .UNSPECIFIED.);
#708=B_SPLINE_CURVE_WITH_KNOTS('',3,(#28527,#28528,#28529,#28530,#28531,
#28532,#28533,#28534,#28535,#28536),.UNSPECIFIED.,.F.,.F.,(4,1,1,1,1,1,
1,4),(103.672557568463,104.173020003322,105.170518658773,106.168017314223,
107.165515969674,108.163014625124,109.160513280575,109.955742875643),
 .UNSPECIFIED.);
#709=B_SPLINE_CURVE_WITH_KNOTS('',3,(#28541,#28542,#28543,#28544,#28545,
#28546,#28547,#28548,#28549,#28550,#28551),.UNSPECIFIED.,.F.,.F.,(4,1,1,
1,1,1,1,1,4),(97.3893722612837,97.646464373,98.6439630284505,99.641461683901,
100.638960339352,101.636458994802,102.633957650253,103.631456305703,103.672557568463),
 .UNSPECIFIED.);
#710=B_SPLINE_CURVE_WITH_KNOTS('',3,(#28552,#28553,#28554,#28555,#28556,
#28557,#28558,#28559,#28560,#28561),.UNSPECIFIED.,.F.,.F.,(4,1,1,1,1,1,
1,4),(97.3893722612837,98.1880280706194,99.1855267260699,100.18302538152,
101.180524036971,102.178022692421,103.175521347872,103.672557568463),
 .UNSPECIFIED.);
#711=B_SPLINE_CURVE_WITH_KNOTS('',3,(#28566,#28567,#28568,#28569,#28570,
#28571,#28572,#28573,#28574,#28575),.UNSPECIFIED.,.F.,.F.,(4,1,1,1,1,1,
1,4),(91.106186954104,91.661472440297,92.6589710957475,93.656469751198,
94.6539684066485,95.651467062099,96.6489657175495,97.3893722612837),
 .UNSPECIFIED.);
#712=B_SPLINE_CURVE_WITH_KNOTS('',3,(#28576,#28577,#28578,#28579,#28580,
#28581,#28582,#28583,#28584,#28585,#28586),.UNSPECIFIED.,.F.,.F.,(4,1,1,
1,1,1,1,1,4),(91.106186954104,91.2055374824659,92.2030361379164,93.2005347933669,
94.1980334488174,95.1955321042679,96.1930307597184,97.1905294151689,97.3893722612837),
 .UNSPECIFIED.);
#713=B_SPLINE_CURVE_WITH_KNOTS('',3,(#28591,#28592,#28593,#28594,#28595,
#28596,#28597,#28598,#28599,#28600),.UNSPECIFIED.,.F.,.F.,(4,1,1,1,1,1,
1,4),(84.8230016469245,85.676480507594,86.6739791630445,87.671477818495,
88.6689764739455,89.666475129396,90.6639737848465,91.106186954104),
 .UNSPECIFIED.);
#714=B_SPLINE_CURVE_WITH_KNOTS('',3,(#28601,#28602,#28603,#28604,#28605,
#28606,#28607,#28608,#28609,#28610),.UNSPECIFIED.,.F.,.F.,(4,1,1,1,1,1,
1,4),(84.8230016469245,85.2205455497629,86.2180442052134,87.2155428606639,
88.2130415161144,89.2105401715649,90.2080388270154,91.106186954104),
 .UNSPECIFIED.);
#715=B_SPLINE_CURVE_WITH_KNOTS('',3,(#28615,#28616,#28617,#28618,#28619,
#28620,#28621,#28622,#28623,#28624,#28625),.UNSPECIFIED.,.F.,.F.,(4,1,1,
1,1,1,1,1,4),(78.5398163397448,78.6939899194405,79.691488574891,80.6889872303415,
81.686485885792,82.6839845412425,83.681483196693,84.6789818521435,84.8230016469245),
 .UNSPECIFIED.);
#716=B_SPLINE_CURVE_WITH_KNOTS('',3,(#28626,#28627,#28628,#28629,#28630,
#28631,#28632,#28633,#28634,#28635),.UNSPECIFIED.,.F.,.F.,(4,1,1,1,1,1,
1,4),(78.5398163397448,79.2355536170598,80.2330522725103,81.2305509279608,
82.2280495834113,83.2255482388618,84.2230468943123,84.8230016469245),
 .UNSPECIFIED.);
#717=B_SPLINE_CURVE_WITH_KNOTS('',3,(#28640,#28641,#28642,#28643,#28644,
#28645,#28646,#28647,#28648,#28649),.UNSPECIFIED.,.F.,.F.,(4,1,1,1,1,1,
1,4),(72.2566310325652,72.7089979867375,73.706496642188,74.7039952976385,
75.701493953089,76.6989926085395,77.69649126399,78.5398163397448),
 .UNSPECIFIED.);
#718=B_SPLINE_CURVE_WITH_KNOTS('',3,(#28650,#28651,#28652,#28653,#28654,
#28655,#28656,#28657,#28658,#28659),.UNSPECIFIED.,.F.,.F.,(4,1,1,1,1,1,
1,4),(72.2566310325652,73.2505616843569,74.2480603398074,75.2455589952579,
76.2430576507084,77.2405563061589,78.2380549616094,78.5398163397448),
 .UNSPECIFIED.);
#719=B_SPLINE_CURVE_WITH_KNOTS('',3,(#28664,#28665,#28666,#28667,#28668,
#28669,#28670,#28671,#28672,#28673),.UNSPECIFIED.,.F.,.F.,(4,1,1,1,1,1,
1,4),(65.9734457253856,66.7240060540345,67.721504709485,68.7190033649355,
69.716502020386,70.7140006758365,71.711499331287,72.2566310325652),
 .UNSPECIFIED.);
#720=B_SPLINE_CURVE_WITH_KNOTS('',3,(#28674,#28675,#28676,#28677,#28678,
#28679,#28680,#28681,#28682,#28683,#28684),.UNSPECIFIED.,.F.,.F.,(4,1,1,
1,1,1,1,1,4),(65.9734457253856,66.2680710962033,67.2655697516538,68.2630684071043,
69.2605670625549,70.2580657180054,71.2555643734559,72.2530630289064,72.2566310325652),
 .UNSPECIFIED.);
#721=B_SPLINE_CURVE_WITH_KNOTS('',3,(#28689,#28690,#28691,#28692,#28693,
#28694,#28695,#28696,#28697,#28698,#28699),.UNSPECIFIED.,.F.,.F.,(4,1,1,
1,1,1,1,1,4),(59.690260418206,59.741515465881,60.7390141213315,61.736512776782,
62.7340114322325,63.731510087683,64.7290087431335,65.726507398584,65.9734457253856),
 .UNSPECIFIED.);
#722=B_SPLINE_CURVE_WITH_KNOTS('',3,(#28700,#28701,#28702,#28703,#28704,
#28705,#28706,#28707,#28708,#28709),.UNSPECIFIED.,.F.,.F.,(4,1,1,1,1,1,
1,4),(59.690260418206,60.2830791635003,61.2805778189508,62.2780764744013,
63.2755751298518,64.2730737853023,65.2705724407528,65.9734457253856),
 .UNSPECIFIED.);
#723=B_SPLINE_CURVE_WITH_KNOTS('',3,(#28714,#28715,#28716,#28717,#28718,
#28719,#28720,#28721,#28722,#28723),.UNSPECIFIED.,.F.,.F.,(4,1,1,1,1,1,
1,4),(53.4070751110264,53.756523533178,54.7540221886285,55.751520844079,
56.7490194995295,57.74651815498,58.7440168104305,59.690260418206),
 .UNSPECIFIED.);
#724=B_SPLINE_CURVE_WITH_KNOTS('',3,(#28724,#28725,#28726,#28727,#28728,
#28729,#28730,#28731,#28732,#28733),.UNSPECIFIED.,.F.,.F.,(4,1,1,1,1,1,
1,4),(53.4070751110264,54.2980872307973,55.2955858862478,56.2930845416983,
57.2905831971488,58.2880818525993,59.2855805080498,59.690260418206),
 .UNSPECIFIED.);
#725=B_SPLINE_CURVE_WITH_KNOTS('',3,(#28738,#28739,#28740,#28741,#28742,
#28743,#28744,#28745,#28746,#28747),.UNSPECIFIED.,.F.,.F.,(4,1,1,1,1,1,
1,4),(47.1238898038468,47.771531600475,48.7690302559255,49.766528911376,
50.7640275668265,51.761526222277,52.7590248777275,53.4070751110264),
 .UNSPECIFIED.);
#726=B_SPLINE_CURVE_WITH_KNOTS('',3,(#28748,#28749,#28750,#28751,#28752,
#28753,#28754,#28755,#28756,#28757,#28758),.UNSPECIFIED.,.F.,.F.,(4,1,1,
1,1,1,1,1,4),(47.1238898038468,47.3155966426438,48.3130952980943,49.3105939535448,
50.3080926089953,51.3055912644458,52.3030899198963,53.3005885753468,53.4070751110264),
 .UNSPECIFIED.);
#727=B_SPLINE_CURVE_WITH_KNOTS('',3,(#28763,#28764,#28765,#28766,#28767,
#28768,#28769,#28770,#28771,#28772),.UNSPECIFIED.,.F.,.F.,(4,1,1,1,1,1,
1,4),(40.8407044966672,41.786539667772,42.7840383232225,43.781536978673,
44.7790356341235,45.776534289574,46.7740329450245,47.1238898038468),
 .UNSPECIFIED.);
#728=B_SPLINE_CURVE_WITH_KNOTS('',3,(#28773,#28774,#28775,#28776,#28777,
#28778,#28779,#28780,#28781,#28782),.UNSPECIFIED.,.F.,.F.,(4,1,1,1,1,1,
1,4),(40.8407044966672,41.3306047099408,42.3281033653913,43.3256020208418,
44.3231006762923,45.3205993317428,46.3180979871933,47.1238898038468),
 .UNSPECIFIED.);
#729=B_SPLINE_CURVE_WITH_KNOTS('',3,(#28787,#28788,#28789,#28790,#28791,
#28792,#28793,#28794,#28795,#28796,#28797),.UNSPECIFIED.,.F.,.F.,(4,1,1,
1,1,1,1,1,4),(34.5575191894876,34.8040490796185,35.801547735069,36.7990463905195,
37.79654504597,38.7940437014205,39.791542356871,40.7890410123215,40.8407044966672),
 .UNSPECIFIED.);
#730=B_SPLINE_CURVE_WITH_KNOTS('',3,(#28798,#28799,#28800,#28801,#28802,
#28803,#28804,#28805,#28806,#28807),.UNSPECIFIED.,.F.,.F.,(4,1,1,1,1,1,
1,4),(34.5575191894876,35.3456127772378,36.3431114326883,37.3406100881388,
38.3381087435893,39.3356073990398,40.3331060544903,40.8407044966672),
 .UNSPECIFIED.);
#731=B_SPLINE_CURVE_WITH_KNOTS('',3,(#28812,#28813,#28814,#28815,#28816,
#28817,#28818,#28819,#28820,#28821),.UNSPECIFIED.,.F.,.F.,(4,1,1,1,1,1,
1,4),(28.2743338823079,28.8190571469155,29.816555802366,30.8140544578165,
31.811553113267,32.8090517687175,33.806550424168,34.5575191894876),
 .UNSPECIFIED.);
#732=B_SPLINE_CURVE_WITH_KNOTS('',3,(#28822,#28823,#28824,#28825,#28826,
#28827,#28828,#28829,#28830,#28831,#28832),.UNSPECIFIED.,.F.,.F.,(4,1,1,
1,1,1,1,1,4),(28.2743338823079,28.3631221890843,29.3606208445348,30.3581194999853,
31.3556181554358,32.3531168108863,33.3506154663368,34.3481141217873,34.5575191894876),
 .UNSPECIFIED.);
#733=B_SPLINE_CURVE_WITH_KNOTS('',3,(#28837,#28838,#28839,#28840,#28841,
#28842,#28843,#28844,#28845,#28846),.UNSPECIFIED.,.F.,.F.,(4,1,1,1,1,1,
1,4),(21.9911485751283,22.8340652142125,23.831563869663,24.8290625251135,
25.826561180564,26.8240598360145,27.821558491465,28.2743338823079),
 .UNSPECIFIED.);
#734=B_SPLINE_CURVE_WITH_KNOTS('',3,(#28847,#28848,#28849,#28850,#28851,
#28852,#28853,#28854,#28855,#28856),.UNSPECIFIED.,.F.,.F.,(4,1,1,1,1,1,
1,4),(21.9911485751283,22.3781302563813,23.3756289118318,24.3731275672823,
25.3706262227328,26.3681248781833,27.3656235336338,28.2743338823079),
 .UNSPECIFIED.);
#735=B_SPLINE_CURVE_WITH_KNOTS('',3,(#28862,#28863,#28864,#28865,#28866),
 .UNSPECIFIED.,.F.,.F.,(4,1,4),(14.3981410127773,15.3956396682278,15.707963267949),
 .UNSPECIFIED.);
#736=B_SPLINE_CURVE_WITH_KNOTS('',3,(#28869,#28870,#28871,#28872,#28873),
 .UNSPECIFIED.,.F.,.F.,(4,1,4),(13.8761928695316,14.8540759706085,15.707963267949),
 .UNSPECIFIED.);
#737=B_SPLINE_CURVE_WITH_KNOTS('',3,(#28879,#28880,#28881,#28882,#28883,
#28884,#28885,#28886,#28887,#28888,#28889,#28890,#28891,#28892,#28893,#28894),
 .UNSPECIFIED.,.F.,.F.,(4,3,3,3,3,4),(114.407157784404,114.712345376808,
115.709844032258,116.707342687709,117.704841343159,118.702339998609),
 .UNSPECIFIED.);
#738=B_SPLINE_CURVE_WITH_KNOTS('',3,(#28902,#28903,#28904,#28905,#28906,
#28907,#28908,#28909,#28910,#28911,#28912,#28913,#28914,#28915,#28916,#28917,
#28918,#28919,#28920,#28921,#28922,#28923),.UNSPECIFIED.,.F.,.F.,(4,3,3,
3,3,3,3,4),(-116.687727133335,-115.709844032258,-114.712345376807,-113.714846721357,
-112.717348065906,-111.719849410456,-110.722350755005,-110.660533485745),
 .UNSPECIFIED.);
#739=B_SPLINE_CURVE_WITH_KNOTS('',3,(#28928,#28929,#28930,#28931,#28932,
#28933,#28934,#28935,#28936,#28937,#28938,#28939,#28940,#28941,#28942,#28943,
#28944,#28945,#28946,#28947,#28948,#28949),.UNSPECIFIED.,.F.,.F.,(4,3,3,
3,3,3,3,4),(108.123972477225,108.727353444105,109.724852099555,110.722350755006,
111.719849410456,112.717348065907,113.714846721357,114.407157784404),
 .UNSPECIFIED.);
#740=B_SPLINE_CURVE_WITH_KNOTS('',3,(#28950,#28951,#28952,#28953,#28954,
#28955,#28956,#28957,#28958,#28959,#28960,#28961,#28962,#28963,#28964,#28965,
#28966,#28967,#28968,#28969,#28970,#28971),.UNSPECIFIED.,.F.,.F.,(4,3,3,
3,3,3,3,4),(-110.660533485745,-109.724852099555,-108.727353444105,-107.729854788654,
-106.732356133204,-105.734857477753,-104.737358822303,-104.377348178566),
 .UNSPECIFIED.);
#741=B_SPLINE_CURVE_WITH_KNOTS('',3,(#28976,#28977,#28978,#28979,#28980,
#28981,#28982,#28983,#28984,#28985,#28986,#28987,#28988,#28989,#28990,#28991,
#28992,#28993,#28994,#28995,#28996,#28997),.UNSPECIFIED.,.F.,.F.,(4,3,3,
3,3,3,3,4),(101.840787170045,102.742361511402,103.739860166852,104.737358822303,
105.734857477753,106.732356133204,107.729854788654,108.123972477225),
 .UNSPECIFIED.);
#742=B_SPLINE_CURVE_WITH_KNOTS('',3,(#28998,#28999,#29000,#29001,#29002,
#29003,#29004,#29005,#29006,#29007,#29008,#29009,#29010,#29011,#29012,#29013,
#29014,#29015,#29016,#29017,#29018,#29019),.UNSPECIFIED.,.F.,.F.,(4,3,3,
3,3,3,3,4),(-104.377348178566,-103.739860166852,-102.742361511402,-101.744862855951,
-100.747364200501,-99.74986554505,-98.7523668895995,-98.0941628713861),
 .UNSPECIFIED.);
#743=B_SPLINE_CURVE_WITH_KNOTS('',3,(#29024,#29025,#29026,#29027,#29028,
#29029,#29030,#29031,#29032,#29033,#29034,#29035,#29036,#29037,#29038,#29039,
#29040,#29041,#29042,#29043,#29044,#29045,#29046,#29047,#29048),
 .UNSPECIFIED.,.F.,.F.,(4,3,3,3,3,3,3,3,4),(95.5576018628656,95.7598709232481,
96.7573695786986,97.7548682341491,98.7523668895996,99.7498655450501,100.747364200501,
101.744862855951,101.840787170045),.UNSPECIFIED.);
#744=B_SPLINE_CURVE_WITH_KNOTS('',3,(#29049,#29050,#29051,#29052,#29053,
#29054,#29055,#29056,#29057,#29058,#29059,#29060,#29061,#29062,#29063,#29064,
#29065,#29066,#29067,#29068,#29069,#29070),.UNSPECIFIED.,.F.,.F.,(4,3,3,
3,3,3,3,4),(-98.0941628713861,-97.754868234149,-96.7573695786985,-95.759870923248,
-94.7623722677975,-93.764873612347,-92.7673749568965,-91.8109775642065),
 .UNSPECIFIED.);
#745=B_SPLINE_CURVE_WITH_KNOTS('',3,(#29075,#29076,#29077,#29078,#29079,
#29080,#29081,#29082,#29083,#29084,#29085,#29086,#29087,#29088,#29089,#29090,
#29091,#29092,#29093,#29094,#29095,#29096),.UNSPECIFIED.,.F.,.F.,(4,3,3,
3,3,3,3,4),(89.274416555686,89.774878990545,90.7723776459956,91.7698763014461,
92.7673749568966,93.764873612347,94.7623722677975,95.5576018628656),
 .UNSPECIFIED.);
#746=B_SPLINE_CURVE_WITH_KNOTS('',3,(#29097,#29098,#29099,#29100,#29101,
#29102,#29103,#29104,#29105,#29106,#29107,#29108,#29109,#29110,#29111,#29112,
#29113,#29114,#29115,#29116,#29117,#29118,#29119,#29120,#29121),
 .UNSPECIFIED.,.F.,.F.,(4,3,3,3,3,3,3,3,4),(-91.8109775642065,-91.769876301446,
-90.7723776459955,-89.774878990545,-88.7773803350945,-87.779881679644,-86.7823830241935,
-85.784884368743,-85.5277922570269),.UNSPECIFIED.);
#747=B_SPLINE_CURVE_WITH_KNOTS('',3,(#29126,#29127,#29128,#29129,#29130,
#29131,#29132,#29133,#29134,#29135,#29136,#29137,#29138,#29139,#29140,#29141,
#29142,#29143,#29144,#29145,#29146,#29147),.UNSPECIFIED.,.F.,.F.,(4,3,3,
3,3,3,3,4),(82.9912312485064,83.7898870578421,84.7873857132926,85.7848843687431,
86.7823830241936,87.7798816796441,88.7773803350946,89.274416555686),
 .UNSPECIFIED.);
#748=B_SPLINE_CURVE_WITH_KNOTS('',3,(#29148,#29149,#29150,#29151,#29152,
#29153,#29154,#29155,#29156,#29157,#29158,#29159,#29160,#29161,#29162,#29163,
#29164,#29165,#29166,#29167,#29168,#29169),.UNSPECIFIED.,.F.,.F.,(4,3,3,
3,3,3,3,4),(-85.5277922570269,-84.7873857132925,-83.789887057842,-82.7923884023915,
-81.794889746941,-80.7973910914905,-79.79989243604,-79.2446069498473),
 .UNSPECIFIED.);
#749=B_SPLINE_CURVE_WITH_KNOTS('',3,(#29174,#29175,#29176,#29177,#29178,
#29179,#29180,#29181,#29182,#29183,#29184,#29185,#29186,#29187,#29188,#29189,
#29190,#29191,#29192,#29193,#29194,#29195,#29196,#29197,#29198),
 .UNSPECIFIED.,.F.,.F.,(4,3,3,3,3,3,3,3,4),(76.7080459413267,76.8073964696886,
77.8048951251391,78.8023937805896,79.7998924360401,80.7973910914905,81.7948897469411,
82.7923884023916,82.9912312485064),.UNSPECIFIED.);
#750=B_SPLINE_CURVE_WITH_KNOTS('',3,(#29199,#29200,#29201,#29202,#29203,
#29204,#29205,#29206,#29207,#29208,#29209,#29210,#29211,#29212,#29213,#29214,
#29215,#29216,#29217,#29218,#29219,#29220),.UNSPECIFIED.,.F.,.F.,(4,3,3,
3,3,3,3,4),(-79.2446069498473,-78.8023937805895,-77.804895125139,-76.8073964696885,
-75.809897814238,-74.8123991587875,-73.814900503337,-72.9614216426677),
 .UNSPECIFIED.);
#751=B_SPLINE_CURVE_WITH_KNOTS('',3,(#29225,#29226,#29227,#29228,#29229,
#29230,#29231,#29232,#29233,#29234,#29235,#29236,#29237,#29238,#29239,#29240,
#29241,#29242,#29243,#29244,#29245,#29246),.UNSPECIFIED.,.F.,.F.,(4,3,3,
3,3,3,3,4),(70.4248606341471,70.8224045369855,71.819903192436,72.8174018478866,
73.814900503337,74.8123991587875,75.8098978142381,76.7080459413267),
 .UNSPECIFIED.);
#752=B_SPLINE_CURVE_WITH_KNOTS('',3,(#29247,#29248,#29249,#29250,#29251,
#29252,#29253,#29254,#29255,#29256,#29257,#29258,#29259,#29260,#29261,#29262,
#29263,#29264,#29265,#29266,#29267,#29268,#29269,#29270,#29271),
 .UNSPECIFIED.,.F.,.F.,(4,3,3,3,3,3,3,3,4),(-72.9614216426677,-72.8174018478865,
-71.819903192436,-70.8224045369855,-69.824905881535,-68.8274072260845,-67.829908570634,
-66.8324099151835,-66.6782363354881),.UNSPECIFIED.);
#753=B_SPLINE_CURVE_WITH_KNOTS('',3,(#29276,#29277,#29278,#29279,#29280,
#29281,#29282,#29283,#29284,#29285,#29286,#29287,#29288,#29289,#29290,#29291,
#29292,#29293,#29294,#29295,#29296,#29297),.UNSPECIFIED.,.F.,.F.,(4,3,3,
3,3,3,3,4),(64.1416753269675,64.8374126042825,65.834911259733,66.8324099151835,
67.829908570634,68.8274072260845,69.824905881535,70.4248606341471),
 .UNSPECIFIED.);
#754=B_SPLINE_CURVE_WITH_KNOTS('',3,(#29298,#29299,#29300,#29301,#29302,
#29303,#29304,#29305,#29306,#29307,#29308,#29309,#29310,#29311,#29312,#29313,
#29314,#29315,#29316,#29317,#29318,#29319),.UNSPECIFIED.,.F.,.F.,(4,3,3,
3,3,3,3,4),(-66.6782363354881,-65.834911259733,-64.8374126042825,-63.839913948832,
-62.8424152933815,-61.844916637931,-60.8474179824805,-60.3950510283085),
 .UNSPECIFIED.);
#755=B_SPLINE_CURVE_WITH_KNOTS('',3,(#29324,#29325,#29326,#29327,#29328,
#29329,#29330,#29331,#29332,#29333,#29334,#29335,#29336,#29337,#29338,#29339,
#29340,#29341,#29342,#29343,#29344,#29345),.UNSPECIFIED.,.F.,.F.,(4,3,3,
3,3,3,3,4),(57.8584900197882,58.8524206715795,59.84991932703,60.8474179824806,
61.844916637931,62.8424152933815,63.839913948832,64.1416753269675),
 .UNSPECIFIED.);
#756=B_SPLINE_CURVE_WITH_KNOTS('',3,(#29346,#29347,#29348,#29349,#29350,
#29351,#29352,#29353,#29354,#29355,#29356,#29357,#29358,#29359,#29360,#29361,
#29362,#29363,#29364,#29365,#29366,#29367),.UNSPECIFIED.,.F.,.F.,(4,3,3,
3,3,3,3,4),(-60.3950510283085,-59.84991932703,-58.8524206715795,-57.854922016129,
-56.8574233606785,-55.859924705228,-54.8624260497775,-54.1118657211288),
 .UNSPECIFIED.);
#757=B_SPLINE_CURVE_WITH_KNOTS('',3,(#29372,#29373,#29374,#29375,#29376,
#29377,#29378,#29379,#29380,#29381,#29382,#29383,#29384,#29385,#29386,#29387,
#29388,#29389,#29390,#29391,#29392,#29393,#29394,#29395,#29396),
 .UNSPECIFIED.,.F.,.F.,(4,3,3,3,3,3,3,3,4),(51.5753047126086,51.869930083426,
52.8674287388765,53.864927394327,54.8624260497775,55.859924705228,56.8574233606785,
57.8549220161291,57.8584900197882),.UNSPECIFIED.);
#758=B_SPLINE_CURVE_WITH_KNOTS('',3,(#29397,#29398,#29399,#29400,#29401,
#29402,#29403,#29404,#29405,#29406,#29407,#29408,#29409,#29410,#29411,#29412,
#29413,#29414,#29415,#29416,#29417,#29418,#29419,#29420,#29421),
 .UNSPECIFIED.,.F.,.F.,(4,3,3,3,3,3,3,3,4),(-54.1118657211288,-53.864927394327,
-52.8674287388765,-51.869930083426,-50.8724314279755,-49.874932772525,-48.8774341170745,
-47.879935461624,-47.8286804139492),.UNSPECIFIED.);
#759=B_SPLINE_CURVE_WITH_KNOTS('',3,(#29426,#29427,#29428,#29429,#29430,
#29431,#29432,#29433,#29434,#29435,#29436,#29437,#29438,#29439,#29440,#29441,
#29442,#29443,#29444,#29445,#29446,#29447),.UNSPECIFIED.,.F.,.F.,(4,3,3,
3,3,3,3,4),(45.292119405429,45.884938150723,46.8824368061735,47.879935461624,
48.8774341170745,49.874932772525,50.8724314279755,51.5753047126086),
 .UNSPECIFIED.);
#760=B_SPLINE_CURVE_WITH_KNOTS('',3,(#29448,#29449,#29450,#29451,#29452,
#29453,#29454,#29455,#29456,#29457,#29458,#29459,#29460,#29461,#29462,#29463,
#29464,#29465,#29466,#29467,#29468,#29469),.UNSPECIFIED.,.F.,.F.,(4,3,3,
3,3,3,3,4),(-47.8286804139492,-46.8824368061735,-45.884938150723,-44.8874394952725,
-43.889940839822,-42.8924421843715,-41.894943528921,-41.5454951067696),
 .UNSPECIFIED.);
#761=B_SPLINE_CURVE_WITH_KNOTS('',3,(#29474,#29475,#29476,#29477,#29478,
#29479,#29480,#29481,#29482,#29483,#29484,#29485,#29486,#29487,#29488,#29489,
#29490,#29491,#29492,#29493,#29494,#29495),.UNSPECIFIED.,.F.,.F.,(4,3,3,
3,3,3,3,4),(39.0089340982494,39.89994621802,40.8974448734705,41.894943528921,
42.8924421843715,43.889940839822,44.8874394952725,45.292119405429),
 .UNSPECIFIED.);
#762=B_SPLINE_CURVE_WITH_KNOTS('',3,(#29496,#29497,#29498,#29499,#29500,
#29501,#29502,#29503,#29504,#29505,#29506,#29507,#29508,#29509,#29510,#29511,
#29512,#29513,#29514,#29515,#29516,#29517),.UNSPECIFIED.,.F.,.F.,(4,3,3,
3,3,3,3,4),(-41.5454951067696,-40.8974448734705,-39.89994621802,-38.9024475625695,
-37.904948907119,-36.9074502516685,-35.909951596218,-35.26230979959),
 .UNSPECIFIED.);
#763=B_SPLINE_CURVE_WITH_KNOTS('',3,(#29522,#29523,#29524,#29525,#29526,
#29527,#29528,#29529,#29530,#29531,#29532,#29533,#29534,#29535,#29536,#29537,
#29538,#29539,#29540,#29541,#29542,#29543,#29544,#29545,#29546),
 .UNSPECIFIED.,.F.,.F.,(4,3,3,3,3,3,3,3,4),(32.7257487910698,32.9174556298665,
33.914954285317,34.9124529407675,35.909951596218,36.9074502516685,37.904948907119,
38.9024475625695,39.0089340982494),.UNSPECIFIED.);
#764=B_SPLINE_CURVE_WITH_KNOTS('',3,(#29547,#29548,#29549,#29550,#29551,
#29552,#29553,#29554,#29555,#29556,#29557,#29558,#29559,#29560,#29561,#29562,
#29563,#29564,#29565,#29566,#29567,#29568),.UNSPECIFIED.,.F.,.F.,(4,3,3,
3,3,3,3,4),(-35.26230979959,-34.9124529407675,-33.914954285317,-32.9174556298665,
-31.919956974416,-30.9224583189655,-29.924959663515,-28.9791244924104),
 .UNSPECIFIED.);
#765=B_SPLINE_CURVE_WITH_KNOTS('',3,(#29573,#29574,#29575,#29576,#29577,
#29578,#29579,#29580,#29581,#29582,#29583,#29584,#29585,#29586,#29587,#29588,
#29589,#29590,#29591,#29592,#29593,#29594),.UNSPECIFIED.,.F.,.F.,(4,3,3,
3,3,3,3,4),(26.4425634838902,26.9324636971635,27.929962352614,28.9274610080645,
29.924959663515,30.9224583189655,31.919956974416,32.7257487910698),
 .UNSPECIFIED.);
#766=B_SPLINE_CURVE_WITH_KNOTS('',3,(#29595,#29596,#29597,#29598,#29599,
#29600,#29601,#29602,#29603,#29604,#29605,#29606,#29607,#29608,#29609,#29610,
#29611,#29612,#29613,#29614,#29615,#29616,#29617,#29618,#29619),
 .UNSPECIFIED.,.F.,.F.,(4,3,3,3,3,3,3,3,4),(-28.9791244924104,-28.9274610080645,
-27.929962352614,-26.9324636971635,-25.934965041713,-24.9374663862625,-23.939967730812,
-22.9424690753615,-22.6959391852311),.UNSPECIFIED.);
#767=B_SPLINE_CURVE_WITH_KNOTS('',3,(#29624,#29625,#29626,#29627,#29628,
#29629,#29630,#29631,#29632,#29633,#29634,#29635,#29636,#29637,#29638,#29639,
#29640,#29641,#29642,#29643,#29644,#29645),.UNSPECIFIED.,.F.,.F.,(4,3,3,
3,3,3,3,4),(20.1593781767106,20.9474717644605,21.944970419911,22.9424690753615,
23.939967730812,24.9374663862625,25.934965041713,26.4425634838902),
 .UNSPECIFIED.);
#768=B_SPLINE_CURVE_WITH_KNOTS('',3,(#29646,#29647,#29648,#29649,#29650,
#29651,#29652,#29653,#29654,#29655,#29656,#29657,#29658,#29659,#29660,#29661,
#29662,#29663,#29664,#29665,#29666,#29667),.UNSPECIFIED.,.F.,.F.,(4,3,3,
3,3,3,3,4),(-22.6959391852311,-21.944970419911,-20.9474717644605,-19.94997310901,
-18.9524744535595,-17.954975798109,-16.9574771426585,-16.4127538780515),
 .UNSPECIFIED.);
#769=B_SPLINE_CURVE_WITH_KNOTS('',3,(#29672,#29673,#29674,#29675,#29676,
#29677,#29678,#29679,#29680,#29681,#29682,#29683,#29684,#29685,#29686,#29687,
#29688,#29689,#29690,#29691,#29692,#29693,#29694,#29695,#29696),
 .UNSPECIFIED.,.F.,.F.,(4,3,3,3,3,3,3,3,4),(13.8761928695309,13.964981176307,
14.9624798317575,15.959978487208,16.9574771426585,17.954975798109,18.9524744535595,
19.94997310901,20.1593781767106),.UNSPECIFIED.);
#770=B_SPLINE_CURVE_WITH_KNOTS('',3,(#29697,#29698,#29699,#29700,#29701,
#29702,#29703,#29704,#29705,#29706,#29707,#29708,#29709,#29710,#29711,#29712,
#29713,#29714,#29715,#29716,#29717,#29718),.UNSPECIFIED.,.F.,.F.,(4,3,3,
3,3,3,3,4),(-16.4127538780515,-15.959978487208,-14.9624798317575,-13.964981176307,
-12.9674825208565,-11.969983865406,-10.9724852099555,-10.1295685708719),
 .UNSPECIFIED.);
#771=B_SPLINE_CURVE_WITH_KNOTS('',3,(#29724,#29725,#29726,#29727,#29728,
#29729,#29730,#29731,#29732,#29733,#29734,#29735,#29736),.UNSPECIFIED.,
 .F.,.F.,(4,3,3,3,4),(-3.84638326369226,-2.9924959663515,-1.994997310901,
-0.9974986554505,0.),.UNSPECIFIED.);
#772=B_SPLINE_CURVE_WITH_KNOTS('',3,(#29739,#29740,#29741,#29742,#29743,
#29744,#29745,#29746,#29747,#29748,#29749,#29750,#29751,#29752,#29753,#29754,
#29755,#29756,#29757),.UNSPECIFIED.,.F.,.F.,(4,3,3,3,3,3,4),(2.01461286527449,
2.9924959663515,3.989994621802,4.9874932772525,5.984991932703,6.9824905881535,
7.59300756235133),.UNSPECIFIED.);
#773=B_SPLINE_CURVE_WITH_KNOTS('',3,(#29763,#29764,#29765,#29766,#29767),
 .UNSPECIFIED.,.F.,.F.,(4,1,4),(128.805298797181,129.566421347416,130.563920002866),
 .UNSPECIFIED.);
#774=B_SPLINE_CURVE_WITH_KNOTS('',3,(#29770,#29771,#29772,#29773,#29774,
#29775),.UNSPECIFIED.,.F.,.F.,(4,1,1,4),(128.805298797181,129.110486389585,
130.107985045035,131.085868146112),.UNSPECIFIED.);
#775=B_SPLINE_CURVE_WITH_KNOTS('',3,(#29780,#29781,#29782,#29783,#29784,
#29785,#29786,#29787,#29788,#29789,#29790),.UNSPECIFIED.,.F.,.F.,(4,1,1,
1,1,1,1,1,4),(122.522113490002,122.583930759262,123.581429414713,124.578928070163,
125.576426725614,126.573925381064,127.571424036515,128.568922691965,128.805298797181),
 .UNSPECIFIED.);
#776=B_SPLINE_CURVE_WITH_KNOTS('',3,(#29791,#29792,#29793,#29794,#29795,
#29796,#29797,#29798,#29799,#29800),.UNSPECIFIED.,.F.,.F.,(4,1,1,1,1,1,
1,4),(122.522113490002,123.125494456882,124.122993112332,125.120491767783,
126.117990423233,127.115489078684,128.112987734134,128.805298797181),
 .UNSPECIFIED.);
#777=B_SPLINE_CURVE_WITH_KNOTS('',3,(#29805,#29806,#29807,#29808,#29809,
#29810,#29811,#29812,#29813,#29814),.UNSPECIFIED.,.F.,.F.,(4,1,1,1,1,1,
1,4),(116.238928182823,116.598938826559,117.59643748201,118.59393613746,
119.591434792911,120.588933448361,121.586432103812,122.522113490002),
 .UNSPECIFIED.);
#778=B_SPLINE_CURVE_WITH_KNOTS('',3,(#29815,#29816,#29817,#29818,#29819,
#29820,#29821,#29822,#29823,#29824),.UNSPECIFIED.,.F.,.F.,(4,1,1,1,1,1,
1,4),(116.238928182822,117.140502524179,118.138001179629,119.13549983508,
120.13299849053,121.130497145981,122.127995801431,122.522113490002),
 .UNSPECIFIED.);
#779=B_SPLINE_CURVE_WITH_KNOTS('',3,(#29829,#29830,#29831,#29832,#29833,
#29834,#29835,#29836,#29837,#29838),.UNSPECIFIED.,.F.,.F.,(4,1,1,1,1,1,
1,4),(109.955742875643,110.613946893856,111.611445549307,112.608944204757,
113.606442860208,114.603941515658,115.601440171109,116.238928182823),
 .UNSPECIFIED.);
#780=B_SPLINE_CURVE_WITH_KNOTS('',3,(#29839,#29840,#29841,#29842,#29843,
#29844,#29845,#29846,#29847,#29848,#29849),.UNSPECIFIED.,.F.,.F.,(4,1,1,
1,1,1,1,1,4),(109.955742875643,110.158011936025,111.155510591476,112.153009246926,
113.150507902377,114.148006557827,115.145505213278,116.143003868728,116.238928182822),
 .UNSPECIFIED.);
#781=B_SPLINE_CURVE_WITH_KNOTS('',3,(#29854,#29855,#29856,#29857,#29858,
#29859,#29860,#29861,#29862,#29863),.UNSPECIFIED.,.F.,.F.,(4,1,1,1,1,1,
1,4),(103.672557568463,104.628954961153,105.626453616604,106.623952272054,
107.621450927505,108.618949582955,109.616448238406,109.955742875643),
 .UNSPECIFIED.);
#782=B_SPLINE_CURVE_WITH_KNOTS('',3,(#29864,#29865,#29866,#29867,#29868,
#29869,#29870,#29871,#29872,#29873),.UNSPECIFIED.,.F.,.F.,(4,1,1,1,1,1,
1,4),(103.672557568463,104.173020003322,105.170518658773,106.168017314223,
107.165515969674,108.163014625124,109.160513280575,109.955742875643),
 .UNSPECIFIED.);
#783=B_SPLINE_CURVE_WITH_KNOTS('',3,(#29878,#29879,#29880,#29881,#29882,
#29883,#29884,#29885,#29886,#29887,#29888),.UNSPECIFIED.,.F.,.F.,(4,1,1,
1,1,1,1,1,4),(97.3893722612837,97.6464643729997,98.6439630284502,99.6414616839007,
100.638960339351,101.636458994802,102.633957650252,103.631456305703,103.672557568463),
 .UNSPECIFIED.);
#784=B_SPLINE_CURVE_WITH_KNOTS('',3,(#29889,#29890,#29891,#29892,#29893,
#29894,#29895,#29896,#29897,#29898),.UNSPECIFIED.,.F.,.F.,(4,1,1,1,1,1,
1,4),(97.3893722612837,98.1880280706191,99.1855267260696,100.18302538152,
101.180524036971,102.178022692421,103.175521347872,103.672557568463),
 .UNSPECIFIED.);
#785=B_SPLINE_CURVE_WITH_KNOTS('',3,(#29903,#29904,#29905,#29906,#29907,
#29908,#29909,#29910,#29911,#29912),.UNSPECIFIED.,.F.,.F.,(4,1,1,1,1,1,
1,4),(91.106186954104,91.6614724402967,92.6589710957472,93.6564697511977,
94.6539684066482,95.6514670620987,96.6489657175492,97.3893722612837),
 .UNSPECIFIED.);
#786=B_SPLINE_CURVE_WITH_KNOTS('',3,(#29913,#29914,#29915,#29916,#29917,
#29918,#29919,#29920,#29921,#29922,#29923),.UNSPECIFIED.,.F.,.F.,(4,1,1,
1,1,1,1,1,4),(91.106186954104,91.2055374824655,92.203036137916,93.2005347933665,
94.198033448817,95.1955321042675,96.193030759718,97.1905294151685,97.3893722612837),
 .UNSPECIFIED.);
#787=B_SPLINE_CURVE_WITH_KNOTS('',3,(#29928,#29929,#29930,#29931,#29932,
#29933,#29934,#29935,#29936,#29937),.UNSPECIFIED.,.F.,.F.,(4,1,1,1,1,1,
1,4),(84.8230016469244,85.6764805075937,86.6739791630442,87.6714778184947,
88.6689764739452,89.6664751293957,90.6639737848462,91.106186954104),
 .UNSPECIFIED.);
#788=B_SPLINE_CURVE_WITH_KNOTS('',3,(#29938,#29939,#29940,#29941,#29942,
#29943,#29944,#29945,#29946,#29947),.UNSPECIFIED.,.F.,.F.,(4,1,1,1,1,1,
1,4),(84.8230016469245,85.2205455497625,86.218044205213,87.2155428606635,
88.213041516114,89.2105401715645,90.208038827015,91.106186954104),
 .UNSPECIFIED.);
#789=B_SPLINE_CURVE_WITH_KNOTS('',3,(#29952,#29953,#29954,#29955,#29956,
#29957,#29958,#29959,#29960,#29961,#29962),.UNSPECIFIED.,.F.,.F.,(4,1,1,
1,1,1,1,1,4),(78.5398163397449,78.6939899194402,79.6914885748907,80.6889872303412,
81.6864858857917,82.6839845412422,83.6814831966927,84.6789818521432,84.8230016469244),
 .UNSPECIFIED.);
#790=B_SPLINE_CURVE_WITH_KNOTS('',3,(#29963,#29964,#29965,#29966,#29967,
#29968,#29969,#29970,#29971,#29972),.UNSPECIFIED.,.F.,.F.,(4,1,1,1,1,1,
1,4),(78.5398163397448,79.2355536170595,80.23305227251,81.2305509279605,
82.228049583411,83.2255482388615,84.223046894312,84.8230016469245),
 .UNSPECIFIED.);
#791=B_SPLINE_CURVE_WITH_KNOTS('',3,(#29977,#29978,#29979,#29980,#29981,
#29982,#29983,#29984,#29985,#29986),.UNSPECIFIED.,.F.,.F.,(4,1,1,1,1,1,
1,4),(72.2566310325652,72.7089979867372,73.7064966421877,74.7039952976382,
75.7014939530887,76.6989926085392,77.6964912639897,78.5398163397449),
 .UNSPECIFIED.);
#792=B_SPLINE_CURVE_WITH_KNOTS('',3,(#29987,#29988,#29989,#29990,#29991,
#29992,#29993,#29994,#29995,#29996),.UNSPECIFIED.,.F.,.F.,(4,1,1,1,1,1,
1,4),(72.2566310325652,73.2505616843565,74.248060339807,75.2455589952575,
76.243057650708,77.2405563061585,78.238054961609,78.5398163397448),
 .UNSPECIFIED.);
#793=B_SPLINE_CURVE_WITH_KNOTS('',3,(#30001,#30002,#30003,#30004,#30005,
#30006,#30007,#30008,#30009,#30010),.UNSPECIFIED.,.F.,.F.,(4,1,1,1,1,1,
1,4),(65.9734457253856,66.7240060540342,67.7215047094847,68.7190033649352,
69.7165020203857,70.7140006758362,71.7114993312867,72.2566310325652),
 .UNSPECIFIED.);
#794=B_SPLINE_CURVE_WITH_KNOTS('',3,(#30011,#30012,#30013,#30014,#30015,
#30016,#30017,#30018,#30019,#30020,#30021),.UNSPECIFIED.,.F.,.F.,(4,1,1,
1,1,1,1,1,4),(65.9734457253856,66.268071096203,67.2655697516535,68.263068407104,
69.2605670625545,70.258065718005,71.2555643734555,72.253063028906,72.2566310325652),
 .UNSPECIFIED.);
#795=B_SPLINE_CURVE_WITH_KNOTS('',3,(#30026,#30027,#30028,#30029,#30030,
#30031,#30032,#30033,#30034,#30035,#30036),.UNSPECIFIED.,.F.,.F.,(4,1,1,
1,1,1,1,1,4),(59.690260418206,59.7415154658807,60.7390141213312,61.7365127767817,
62.7340114322322,63.7315100876827,64.7290087431332,65.7265073985837,65.9734457253856),
 .UNSPECIFIED.);
#796=B_SPLINE_CURVE_WITH_KNOTS('',3,(#30037,#30038,#30039,#30040,#30041,
#30042,#30043,#30044,#30045,#30046),.UNSPECIFIED.,.F.,.F.,(4,1,1,1,1,1,
1,4),(59.690260418206,60.2830791635,61.2805778189505,62.278076474401,63.2755751298515,
64.273073785302,65.2705724407525,65.9734457253856),.UNSPECIFIED.);
#797=B_SPLINE_CURVE_WITH_KNOTS('',3,(#30051,#30052,#30053,#30054,#30055,
#30056,#30057,#30058,#30059,#30060),.UNSPECIFIED.,.F.,.F.,(4,1,1,1,1,1,
1,4),(53.4070751110264,53.7565235331777,54.7540221886282,55.7515208440787,
56.7490194995292,57.7465181549797,58.7440168104302,59.690260418206),
 .UNSPECIFIED.);
#798=B_SPLINE_CURVE_WITH_KNOTS('',3,(#30061,#30062,#30063,#30064,#30065,
#30066,#30067,#30068,#30069,#30070),.UNSPECIFIED.,.F.,.F.,(4,1,1,1,1,1,
1,4),(53.4070751110264,54.298087230797,55.2955858862475,56.293084541698,
57.2905831971485,58.288081852599,59.2855805080495,59.690260418206),
 .UNSPECIFIED.);
#799=B_SPLINE_CURVE_WITH_KNOTS('',3,(#30075,#30076,#30077,#30078,#30079,
#30080,#30081,#30082,#30083,#30084),.UNSPECIFIED.,.F.,.F.,(4,1,1,1,1,1,
1,4),(47.1238898038468,47.7715316004747,48.7690302559252,49.7665289113757,
50.7640275668262,51.7615262222767,52.7590248777272,53.4070751110264),
 .UNSPECIFIED.);
#800=B_SPLINE_CURVE_WITH_KNOTS('',3,(#30085,#30086,#30087,#30088,#30089,
#30090,#30091,#30092,#30093,#30094,#30095),.UNSPECIFIED.,.F.,.F.,(4,1,1,
1,1,1,1,1,4),(47.1238898038468,47.3155966426435,48.313095298094,49.3105939535445,
50.308092608995,51.3055912644455,52.303089919896,53.3005885753465,53.4070751110264),
 .UNSPECIFIED.);
#801=B_SPLINE_CURVE_WITH_KNOTS('',3,(#30100,#30101,#30102,#30103,#30104,
#30105,#30106,#30107,#30108,#30109),.UNSPECIFIED.,.F.,.F.,(4,1,1,1,1,1,
1,4),(40.8407044966672,41.7865396677717,42.7840383232222,43.7815369786727,
44.7790356341232,45.7765342895737,46.7740329450242,47.1238898038468),
 .UNSPECIFIED.);
#802=B_SPLINE_CURVE_WITH_KNOTS('',3,(#30110,#30111,#30112,#30113,#30114,
#30115,#30116,#30117,#30118,#30119),.UNSPECIFIED.,.F.,.F.,(4,1,1,1,1,1,
1,4),(40.8407044966672,41.3306047099405,42.328103365391,43.3256020208415,
44.323100676292,45.3205993317425,46.318097987193,47.1238898038468),
 .UNSPECIFIED.);
#803=B_SPLINE_CURVE_WITH_KNOTS('',3,(#30124,#30125,#30126,#30127,#30128,
#30129,#30130,#30131,#30132,#30133,#30134),.UNSPECIFIED.,.F.,.F.,(4,1,1,
1,1,1,1,1,4),(34.5575191894876,34.8040490796182,35.8015477350687,36.7990463905192,
37.7965450459697,38.7940437014202,39.7915423568707,40.7890410123212,40.8407044966672),
 .UNSPECIFIED.);
#804=B_SPLINE_CURVE_WITH_KNOTS('',3,(#30135,#30136,#30137,#30138,#30139,
#30140,#30141,#30142,#30143,#30144),.UNSPECIFIED.,.F.,.F.,(4,1,1,1,1,1,
1,4),(34.5575191894876,35.3456127772375,36.343111432688,37.3406100881385,
38.338108743589,39.3356073990395,40.33310605449,40.8407044966672),
 .UNSPECIFIED.);
#805=B_SPLINE_CURVE_WITH_KNOTS('',3,(#30149,#30150,#30151,#30152,#30153,
#30154,#30155,#30156,#30157,#30158),.UNSPECIFIED.,.F.,.F.,(4,1,1,1,1,1,
1,4),(28.2743338823079,28.8190571469152,29.8165558023657,30.8140544578162,
31.8115531132667,32.8090517687172,33.8065504241677,34.5575191894876),
 .UNSPECIFIED.);
#806=B_SPLINE_CURVE_WITH_KNOTS('',3,(#30159,#30160,#30161,#30162,#30163,
#30164,#30165,#30166,#30167,#30168,#30169),.UNSPECIFIED.,.F.,.F.,(4,1,1,
1,1,1,1,1,4),(28.2743338823079,28.363122189084,29.3606208445345,30.358119499985,
31.3556181554355,32.353116810886,33.3506154663365,34.348114121787,34.5575191894876),
 .UNSPECIFIED.);
#807=B_SPLINE_CURVE_WITH_KNOTS('',3,(#30174,#30175,#30176,#30177,#30178,
#30179,#30180,#30181,#30182,#30183),.UNSPECIFIED.,.F.,.F.,(4,1,1,1,1,1,
1,4),(21.9911485751283,22.8340652142122,23.8315638696627,24.8290625251132,
25.8265611805637,26.8240598360142,27.8215584914647,28.2743338823079),
 .UNSPECIFIED.);
#808=B_SPLINE_CURVE_WITH_KNOTS('',3,(#30184,#30185,#30186,#30187,#30188,
#30189,#30190,#30191,#30192,#30193),.UNSPECIFIED.,.F.,.F.,(4,1,1,1,1,1,
1,4),(21.9911485751283,22.378130256381,23.3756289118315,24.373127567282,
25.3706262227325,26.368124878183,27.3656235336335,28.2743338823079),
 .UNSPECIFIED.);
#809=B_SPLINE_CURVE_WITH_KNOTS('',3,(#30199,#30200,#30201,#30202,#30203),
 .UNSPECIFIED.,.F.,.F.,(4,1,4),(14.398141012777,15.3956396682275,15.707963267949),
 .UNSPECIFIED.);
#810=B_SPLINE_CURVE_WITH_KNOTS('',3,(#30206,#30207,#30208,#30209,#30210),
 .UNSPECIFIED.,.F.,.F.,(4,1,4),(13.8761928695313,14.8540759706082,15.707963267949),
 .UNSPECIFIED.);
#811=B_SPLINE_CURVE_WITH_KNOTS('',3,(#30216,#30217,#30218,#30219,#30220,
#30221,#30222,#30223,#30224,#30225,#30226,#30227,#30228,#30229,#30230,#30231),
 .UNSPECIFIED.,.F.,.F.,(4,3,3,3,3,4),(114.407157784404,114.712345376807,
115.709844032258,116.707342687708,117.704841343159,118.702339998609),
 .UNSPECIFIED.);
#812=B_SPLINE_CURVE_WITH_KNOTS('',3,(#30239,#30240,#30241,#30242,#30243,
#30244,#30245,#30246,#30247,#30248,#30249,#30250,#30251,#30252,#30253,#30254,
#30255,#30256,#30257,#30258,#30259,#30260),.UNSPECIFIED.,.F.,.F.,(4,3,3,
3,3,3,3,4),(-116.687727133335,-115.709844032258,-114.712345376808,-113.714846721357,
-112.717348065907,-111.719849410456,-110.722350755006,-110.660533485745),
 .UNSPECIFIED.);
#813=B_SPLINE_CURVE_WITH_KNOTS('',3,(#30265,#30266,#30267,#30268,#30269,
#30270,#30271,#30272,#30273,#30274,#30275,#30276,#30277,#30278,#30279,#30280,
#30281,#30282,#30283,#30284,#30285,#30286),.UNSPECIFIED.,.F.,.F.,(4,3,3,
3,3,3,3,4),(108.123972477224,108.727353444104,109.724852099555,110.722350755005,
111.719849410456,112.717348065906,113.714846721357,114.407157784404),
 .UNSPECIFIED.);
#814=B_SPLINE_CURVE_WITH_KNOTS('',3,(#30287,#30288,#30289,#30290,#30291,
#30292,#30293,#30294,#30295,#30296,#30297,#30298,#30299,#30300,#30301,#30302,
#30303,#30304,#30305,#30306,#30307,#30308),.UNSPECIFIED.,.F.,.F.,(4,3,3,
3,3,3,3,4),(-110.660533485745,-109.724852099555,-108.727353444105,-107.729854788654,
-106.732356133204,-105.734857477753,-104.737358822303,-104.377348178565),
 .UNSPECIFIED.);
#815=B_SPLINE_CURVE_WITH_KNOTS('',3,(#30313,#30314,#30315,#30316,#30317,
#30318,#30319,#30320,#30321,#30322,#30323,#30324,#30325,#30326,#30327,#30328,
#30329,#30330,#30331,#30332,#30333,#30334),.UNSPECIFIED.,.F.,.F.,(4,3,3,
3,3,3,3,4),(101.840787170045,102.742361511401,103.739860166852,104.737358822302,
105.734857477753,106.732356133203,107.729854788654,108.123972477224),
 .UNSPECIFIED.);
#816=B_SPLINE_CURVE_WITH_KNOTS('',3,(#30335,#30336,#30337,#30338,#30339,
#30340,#30341,#30342,#30343,#30344,#30345,#30346,#30347,#30348,#30349,#30350,
#30351,#30352,#30353,#30354,#30355,#30356),.UNSPECIFIED.,.F.,.F.,(4,3,3,
3,3,3,3,4),(-104.377348178565,-103.739860166852,-102.742361511402,-101.744862855951,
-100.747364200501,-99.74986554505,-98.7523668895995,-98.0941628713855),
 .UNSPECIFIED.);
#817=B_SPLINE_CURVE_WITH_KNOTS('',3,(#30361,#30362,#30363,#30364,#30365,
#30366,#30367,#30368,#30369,#30370,#30371,#30372,#30373,#30374,#30375,#30376,
#30377,#30378,#30379,#30380,#30381,#30382,#30383,#30384,#30385),
 .UNSPECIFIED.,.F.,.F.,(4,3,3,3,3,3,3,3,4),(95.5576018628649,95.7598709232479,
96.7573695786984,97.7548682341489,98.7523668895994,99.7498655450499,100.7473642005,
101.744862855951,101.840787170045),.UNSPECIFIED.);
#818=B_SPLINE_CURVE_WITH_KNOTS('',3,(#30386,#30387,#30388,#30389,#30390,
#30391,#30392,#30393,#30394,#30395,#30396,#30397,#30398,#30399,#30400,#30401,
#30402,#30403,#30404,#30405,#30406,#30407),.UNSPECIFIED.,.F.,.F.,(4,3,3,
3,3,3,3,4),(-98.0941628713855,-97.754868234149,-96.7573695786985,-95.759870923248,
-94.7623722677975,-93.764873612347,-92.7673749568965,-91.8109775642059),
 .UNSPECIFIED.);
#819=B_SPLINE_CURVE_WITH_KNOTS('',3,(#30412,#30413,#30414,#30415,#30416,
#30417,#30418,#30419,#30420,#30421,#30422,#30423,#30424,#30425,#30426,#30427,
#30428,#30429,#30430,#30431,#30432,#30433),.UNSPECIFIED.,.F.,.F.,(4,3,3,
3,3,3,3,4),(89.2744165556853,89.774878990545,90.7723776459954,91.7698763014459,
92.7673749568964,93.7648736123469,94.7623722677974,95.5576018628649),
 .UNSPECIFIED.);
#820=B_SPLINE_CURVE_WITH_KNOTS('',3,(#30434,#30435,#30436,#30437,#30438,
#30439,#30440,#30441,#30442,#30443,#30444,#30445,#30446,#30447,#30448,#30449,
#30450,#30451,#30452,#30453,#30454,#30455,#30456,#30457,#30458),
 .UNSPECIFIED.,.F.,.F.,(4,3,3,3,3,3,3,3,4),(-91.8109775642059,-91.769876301446,
-90.7723776459955,-89.774878990545,-88.7773803350945,-87.779881679644,-86.7823830241935,
-85.784884368743,-85.5277922570263),.UNSPECIFIED.);
#821=B_SPLINE_CURVE_WITH_KNOTS('',3,(#30463,#30464,#30465,#30466,#30467,
#30468,#30469,#30470,#30471,#30472,#30473,#30474,#30475,#30476,#30477,#30478,
#30479,#30480,#30481,#30482,#30483,#30484),.UNSPECIFIED.,.F.,.F.,(4,3,3,
3,3,3,3,4),(82.9912312485057,83.789887057842,84.7873857132925,85.784884368743,
86.7823830241934,87.7798816796439,88.7773803350944,89.2744165556853),
 .UNSPECIFIED.);
#822=B_SPLINE_CURVE_WITH_KNOTS('',3,(#30485,#30486,#30487,#30488,#30489,
#30490,#30491,#30492,#30493,#30494,#30495,#30496,#30497,#30498,#30499,#30500,
#30501,#30502,#30503,#30504,#30505,#30506),.UNSPECIFIED.,.F.,.F.,(4,3,3,
3,3,3,3,4),(-85.5277922570263,-84.7873857132925,-83.789887057842,-82.7923884023915,
-81.794889746941,-80.7973910914905,-79.79989243604,-79.2446069498467),
 .UNSPECIFIED.);
#823=B_SPLINE_CURVE_WITH_KNOTS('',3,(#30511,#30512,#30513,#30514,#30515,
#30516,#30517,#30518,#30519,#30520,#30521,#30522,#30523,#30524,#30525,#30526,
#30527,#30528,#30529,#30530,#30531,#30532,#30533,#30534,#30535),
 .UNSPECIFIED.,.F.,.F.,(4,3,3,3,3,3,3,3,4),(76.7080459413261,76.8073964696885,
77.8048951251389,78.8023937805895,79.79989243604,80.7973910914905,81.7948897469409,
82.7923884023915,82.9912312485057),.UNSPECIFIED.);
#824=B_SPLINE_CURVE_WITH_KNOTS('',3,(#30536,#30537,#30538,#30539,#30540,
#30541,#30542,#30543,#30544,#30545,#30546,#30547,#30548,#30549,#30550,#30551,
#30552,#30553,#30554,#30555,#30556,#30557),.UNSPECIFIED.,.F.,.F.,(4,3,3,
3,3,3,3,4),(-79.2446069498467,-78.8023937805895,-77.804895125139,-76.8073964696885,
-75.809897814238,-74.8123991587875,-73.814900503337,-72.961421642667),
 .UNSPECIFIED.);
#825=B_SPLINE_CURVE_WITH_KNOTS('',3,(#30562,#30563,#30564,#30565,#30566,
#30567,#30568,#30569,#30570,#30571,#30572,#30573,#30574,#30575,#30576,#30577,
#30578,#30579,#30580,#30581,#30582,#30583),.UNSPECIFIED.,.F.,.F.,(4,3,3,
3,3,3,3,4),(70.4248606341465,70.8224045369854,71.8199031924359,72.8174018478865,
73.8149005033369,74.8123991587874,75.809897814238,76.7080459413261),
 .UNSPECIFIED.);
#826=B_SPLINE_CURVE_WITH_KNOTS('',3,(#30584,#30585,#30586,#30587,#30588,
#30589,#30590,#30591,#30592,#30593,#30594,#30595,#30596,#30597,#30598,#30599,
#30600,#30601,#30602,#30603,#30604,#30605,#30606,#30607,#30608),
 .UNSPECIFIED.,.F.,.F.,(4,3,3,3,3,3,3,3,4),(-72.961421642667,-72.8174018478865,
-71.819903192436,-70.8224045369855,-69.824905881535,-68.8274072260845,-67.829908570634,
-66.8324099151835,-66.6782363354874),.UNSPECIFIED.);
#827=B_SPLINE_CURVE_WITH_KNOTS('',3,(#30613,#30614,#30615,#30616,#30617,
#30618,#30619,#30620,#30621,#30622,#30623,#30624,#30625,#30626,#30627,#30628,
#30629,#30630,#30631,#30632,#30633,#30634),.UNSPECIFIED.,.F.,.F.,(4,3,3,
3,3,3,3,4),(64.1416753269669,64.8374126042824,65.8349112597329,66.8324099151835,
67.8299085706339,68.8274072260845,69.824905881535,70.4248606341465),
 .UNSPECIFIED.);
#828=B_SPLINE_CURVE_WITH_KNOTS('',3,(#30635,#30636,#30637,#30638,#30639,
#30640,#30641,#30642,#30643,#30644,#30645,#30646,#30647,#30648,#30649,#30650,
#30651,#30652,#30653,#30654,#30655,#30656),.UNSPECIFIED.,.F.,.F.,(4,3,3,
3,3,3,3,4),(-66.6782363354874,-65.834911259733,-64.8374126042825,-63.839913948832,
-62.8424152933815,-61.844916637931,-60.8474179824805,-60.3950510283078),
 .UNSPECIFIED.);
#829=B_SPLINE_CURVE_WITH_KNOTS('',3,(#30661,#30662,#30663,#30664,#30665,
#30666,#30667,#30668,#30669,#30670,#30671,#30672,#30673,#30674,#30675,#30676,
#30677,#30678,#30679,#30680,#30681,#30682),.UNSPECIFIED.,.F.,.F.,(4,3,3,
3,3,3,3,4),(57.8584900197873,58.8524206715795,59.84991932703,60.8474179824805,
61.844916637931,62.8424152933815,63.839913948832,64.1416753269669),
 .UNSPECIFIED.);
#830=B_SPLINE_CURVE_WITH_KNOTS('',3,(#30683,#30684,#30685,#30686,#30687,
#30688,#30689,#30690,#30691,#30692,#30693,#30694,#30695,#30696,#30697,#30698,
#30699,#30700,#30701,#30702,#30703,#30704),.UNSPECIFIED.,.F.,.F.,(4,3,3,
3,3,3,3,4),(-60.3950510283078,-59.84991932703,-58.8524206715795,-57.854922016129,
-56.8574233606785,-55.859924705228,-54.8624260497775,-54.1118657211282),
 .UNSPECIFIED.);
#831=B_SPLINE_CURVE_WITH_KNOTS('',3,(#30709,#30710,#30711,#30712,#30713,
#30714,#30715,#30716,#30717,#30718,#30719,#30720,#30721,#30722,#30723,#30724,
#30725,#30726,#30727,#30728,#30729,#30730,#30731,#30732,#30733),
 .UNSPECIFIED.,.F.,.F.,(4,3,3,3,3,3,3,3,4),(51.575304712608,51.869930083426,
52.8674287388765,53.8649273943269,54.8624260497775,55.859924705228,56.8574233606785,
57.854922016129,57.8584900197873),.UNSPECIFIED.);
#832=B_SPLINE_CURVE_WITH_KNOTS('',3,(#30734,#30735,#30736,#30737,#30738,
#30739,#30740,#30741,#30742,#30743,#30744,#30745,#30746,#30747,#30748,#30749,
#30750,#30751,#30752,#30753,#30754,#30755,#30756,#30757,#30758),
 .UNSPECIFIED.,.F.,.F.,(4,3,3,3,3,3,3,3,4),(-54.1118657211282,-53.864927394327,
-52.8674287388765,-51.869930083426,-50.8724314279755,-49.874932772525,-48.8774341170745,
-47.879935461624,-47.8286804139486),.UNSPECIFIED.);
#833=B_SPLINE_CURVE_WITH_KNOTS('',3,(#30763,#30764,#30765,#30766,#30767,
#30768,#30769,#30770,#30771,#30772,#30773,#30774,#30775,#30776,#30777,#30778,
#30779,#30780,#30781,#30782,#30783,#30784),.UNSPECIFIED.,.F.,.F.,(4,3,3,
3,3,3,3,4),(45.2921194054284,45.884938150723,46.8824368061735,47.879935461624,
48.8774341170745,49.874932772525,50.8724314279755,51.575304712608),
 .UNSPECIFIED.);
#834=B_SPLINE_CURVE_WITH_KNOTS('',3,(#30785,#30786,#30787,#30788,#30789,
#30790,#30791,#30792,#30793,#30794,#30795,#30796,#30797,#30798,#30799,#30800,
#30801,#30802,#30803,#30804,#30805,#30806),.UNSPECIFIED.,.F.,.F.,(4,3,3,
3,3,3,3,4),(-47.8286804139486,-46.8824368061735,-45.884938150723,-44.8874394952725,
-43.889940839822,-42.8924421843715,-41.894943528921,-41.545495106769),
 .UNSPECIFIED.);
#835=B_SPLINE_CURVE_WITH_KNOTS('',3,(#30811,#30812,#30813,#30814,#30815,
#30816,#30817,#30818,#30819,#30820,#30821,#30822,#30823,#30824,#30825,#30826,
#30827,#30828,#30829,#30830,#30831,#30832),.UNSPECIFIED.,.F.,.F.,(4,3,3,
3,3,3,3,4),(39.0089340982488,39.89994621802,40.8974448734705,41.894943528921,
42.8924421843715,43.889940839822,44.8874394952725,45.2921194054284),
 .UNSPECIFIED.);
#836=B_SPLINE_CURVE_WITH_KNOTS('',3,(#30833,#30834,#30835,#30836,#30837,
#30838,#30839,#30840,#30841,#30842,#30843,#30844,#30845,#30846,#30847,#30848,
#30849,#30850,#30851,#30852,#30853,#30854),.UNSPECIFIED.,.F.,.F.,(4,3,3,
3,3,3,3,4),(-41.545495106769,-40.8974448734705,-39.89994621802,-38.9024475625695,
-37.904948907119,-36.9074502516685,-35.909951596218,-35.2623097995894),
 .UNSPECIFIED.);
#837=B_SPLINE_CURVE_WITH_KNOTS('',3,(#30859,#30860,#30861,#30862,#30863,
#30864,#30865,#30866,#30867,#30868,#30869,#30870,#30871,#30872,#30873,#30874,
#30875,#30876,#30877,#30878,#30879,#30880,#30881,#30882,#30883),
 .UNSPECIFIED.,.F.,.F.,(4,3,3,3,3,3,3,3,4),(32.7257487910691,32.9174556298665,
33.914954285317,34.9124529407675,35.909951596218,36.9074502516685,37.904948907119,
38.9024475625695,39.0089340982488),.UNSPECIFIED.);
#838=B_SPLINE_CURVE_WITH_KNOTS('',3,(#30884,#30885,#30886,#30887,#30888,
#30889,#30890,#30891,#30892,#30893,#30894,#30895,#30896,#30897,#30898,#30899,
#30900,#30901,#30902,#30903,#30904,#30905),.UNSPECIFIED.,.F.,.F.,(4,3,3,
3,3,3,3,4),(-35.2623097995894,-34.9124529407675,-33.914954285317,-32.9174556298665,
-31.919956974416,-30.9224583189655,-29.924959663515,-28.9791244924098),
 .UNSPECIFIED.);
#839=B_SPLINE_CURVE_WITH_KNOTS('',3,(#30910,#30911,#30912,#30913,#30914,
#30915,#30916,#30917,#30918,#30919,#30920,#30921,#30922,#30923,#30924,#30925,
#30926,#30927,#30928,#30929,#30930,#30931),.UNSPECIFIED.,.F.,.F.,(4,3,3,
3,3,3,3,4),(26.4425634838895,26.9324636971635,27.929962352614,28.9274610080645,
29.924959663515,30.9224583189655,31.919956974416,32.7257487910691),
 .UNSPECIFIED.);
#840=B_SPLINE_CURVE_WITH_KNOTS('',3,(#30932,#30933,#30934,#30935,#30936,
#30937,#30938,#30939,#30940,#30941,#30942,#30943,#30944,#30945,#30946,#30947,
#30948,#30949,#30950,#30951,#30952,#30953,#30954,#30955,#30956),
 .UNSPECIFIED.,.F.,.F.,(4,3,3,3,3,3,3,3,4),(-28.9791244924098,-28.9274610080645,
-27.929962352614,-26.9324636971635,-25.934965041713,-24.9374663862625,-23.939967730812,
-22.9424690753615,-22.6959391852305),.UNSPECIFIED.);
#841=B_SPLINE_CURVE_WITH_KNOTS('',3,(#30961,#30962,#30963,#30964,#30965,
#30966,#30967,#30968,#30969,#30970,#30971,#30972,#30973,#30974,#30975,#30976,
#30977,#30978,#30979,#30980,#30981,#30982),.UNSPECIFIED.,.F.,.F.,(4,3,3,
3,3,3,3,4),(20.1593781767099,20.9474717644605,21.944970419911,22.9424690753615,
23.939967730812,24.9374663862625,25.934965041713,26.4425634838895),
 .UNSPECIFIED.);
#842=B_SPLINE_CURVE_WITH_KNOTS('',3,(#30983,#30984,#30985,#30986,#30987,
#30988,#30989,#30990,#30991,#30992,#30993,#30994,#30995,#30996,#30997,#30998,
#30999,#31000,#31001,#31002,#31003,#31004),.UNSPECIFIED.,.F.,.F.,(4,3,3,
3,3,3,3,4),(-22.6959391852305,-21.944970419911,-20.9474717644605,-19.94997310901,
-18.9524744535595,-17.954975798109,-16.9574771426585,-16.4127538780508),
 .UNSPECIFIED.);
#843=B_SPLINE_CURVE_WITH_KNOTS('',3,(#31009,#31010,#31011,#31012,#31013,
#31014,#31015,#31016,#31017,#31018,#31019,#31020,#31021,#31022,#31023,#31024,
#31025,#31026,#31027,#31028,#31029,#31030,#31031,#31032,#31033),
 .UNSPECIFIED.,.F.,.F.,(4,3,3,3,3,3,3,3,4),(13.8761928695303,13.964981176307,
14.9624798317575,15.959978487208,16.9574771426585,17.954975798109,18.9524744535595,
19.94997310901,20.1593781767099),.UNSPECIFIED.);
#844=B_SPLINE_CURVE_WITH_KNOTS('',3,(#31034,#31035,#31036,#31037,#31038,
#31039,#31040,#31041,#31042,#31043,#31044,#31045,#31046,#31047,#31048,#31049,
#31050,#31051,#31052,#31053,#31054,#31055),.UNSPECIFIED.,.F.,.F.,(4,3,3,
3,3,3,3,4),(-16.4127538780508,-15.959978487208,-14.9624798317575,-13.964981176307,
-12.9674825208565,-11.969983865406,-10.9724852099555,-10.1295685708712),
 .UNSPECIFIED.);
#845=B_SPLINE_CURVE_WITH_KNOTS('',3,(#31061,#31062,#31063,#31064,#31065,
#31066,#31067,#31068,#31069,#31070,#31071,#31072,#31073),.UNSPECIFIED.,
 .F.,.F.,(4,3,3,3,4),(-3.84638326369162,-2.9924959663515,-1.994997310901,
-0.9974986554505,0.),.UNSPECIFIED.);
#846=B_SPLINE_CURVE_WITH_KNOTS('',3,(#31076,#31077,#31078,#31079,#31080,
#31081,#31082,#31083,#31084,#31085,#31086,#31087,#31088,#31089,#31090,#31091,
#31092,#31093,#31094),.UNSPECIFIED.,.F.,.F.,(4,3,3,3,3,3,4),(2.01461286527449,
2.9924959663515,3.989994621802,4.9874932772525,5.984991932703,6.9824905881535,
7.59300756235069),.UNSPECIFIED.);
#847=B_SPLINE_CURVE_WITH_KNOTS('',3,(#31100,#31101,#31102,#31103,#31104),
 .UNSPECIFIED.,.F.,.F.,(4,1,4),(128.805298797181,129.566421347416,130.563920002867),
 .UNSPECIFIED.);
#848=B_SPLINE_CURVE_WITH_KNOTS('',3,(#31107,#31108,#31109,#31110,#31111,
#31112),.UNSPECIFIED.,.F.,.F.,(4,1,1,4),(128.805298797181,129.110486389585,
130.107985045036,131.085868146113),.UNSPECIFIED.);
#849=B_SPLINE_CURVE_WITH_KNOTS('',3,(#31117,#31118,#31119,#31120,#31121,
#31122,#31123,#31124,#31125,#31126,#31127),.UNSPECIFIED.,.F.,.F.,(4,1,1,
1,1,1,1,1,4),(122.522113490002,122.583930759263,123.581429414713,124.578928070164,
125.576426725614,126.573925381065,127.571424036515,128.568922691966,128.805298797181),
 .UNSPECIFIED.);
#850=B_SPLINE_CURVE_WITH_KNOTS('',3,(#31128,#31129,#31130,#31131,#31132,
#31133,#31134,#31135,#31136,#31137),.UNSPECIFIED.,.F.,.F.,(4,1,1,1,1,1,
1,4),(122.522113490002,123.125494456882,124.122993112333,125.120491767783,
126.117990423234,127.115489078684,128.112987734135,128.805298797181),
 .UNSPECIFIED.);
#851=B_SPLINE_CURVE_WITH_KNOTS('',3,(#31142,#31143,#31144,#31145,#31146,
#31147,#31148,#31149,#31150,#31151),.UNSPECIFIED.,.F.,.F.,(4,1,1,1,1,1,
1,4),(116.238928182822,116.59893882656,117.59643748201,118.593936137461,
119.591434792911,120.588933448362,121.586432103812,122.522113490002),
 .UNSPECIFIED.);
#852=B_SPLINE_CURVE_WITH_KNOTS('',3,(#31152,#31153,#31154,#31155,#31156,
#31157,#31158,#31159,#31160,#31161),.UNSPECIFIED.,.F.,.F.,(4,1,1,1,1,1,
1,4),(116.238928182822,117.140502524179,118.13800117963,119.13549983508,
120.132998490531,121.130497145981,122.127995801432,122.522113490002),
 .UNSPECIFIED.);
#853=B_SPLINE_CURVE_WITH_KNOTS('',3,(#31166,#31167,#31168,#31169,#31170,
#31171,#31172,#31173,#31174,#31175),.UNSPECIFIED.,.F.,.F.,(4,1,1,1,1,1,
1,4),(109.955742875643,110.613946893857,111.611445549307,112.608944204758,
113.606442860208,114.603941515659,115.601440171109,116.238928182822),
 .UNSPECIFIED.);
#854=B_SPLINE_CURVE_WITH_KNOTS('',3,(#31176,#31177,#31178,#31179,#31180,
#31181,#31182,#31183,#31184,#31185,#31186),.UNSPECIFIED.,.F.,.F.,(4,1,1,
1,1,1,1,1,4),(109.955742875643,110.158011936026,111.155510591476,112.153009246927,
113.150507902377,114.148006557828,115.145505213278,116.143003868729,116.238928182822),
 .UNSPECIFIED.);
#855=B_SPLINE_CURVE_WITH_KNOTS('',3,(#31191,#31192,#31193,#31194,#31195,
#31196,#31197,#31198,#31199,#31200),.UNSPECIFIED.,.F.,.F.,(4,1,1,1,1,1,
1,4),(103.672557568463,104.628954961154,105.626453616604,106.623952272055,
107.621450927505,108.618949582956,109.616448238406,109.955742875643),
 .UNSPECIFIED.);
#856=B_SPLINE_CURVE_WITH_KNOTS('',3,(#31201,#31202,#31203,#31204,#31205,
#31206,#31207,#31208,#31209,#31210),.UNSPECIFIED.,.F.,.F.,(4,1,1,1,1,1,
1,4),(103.672557568463,104.173020003323,105.170518658773,106.168017314224,
107.165515969674,108.163014625125,109.160513280575,109.955742875643),
 .UNSPECIFIED.);
#857=B_SPLINE_CURVE_WITH_KNOTS('',3,(#31215,#31216,#31217,#31218,#31219,
#31220,#31221,#31222,#31223,#31224,#31225),.UNSPECIFIED.,.F.,.F.,(4,1,1,
1,1,1,1,1,4),(97.3893722612837,97.6464643730003,98.6439630284508,99.6414616839013,
100.638960339352,101.636458994802,102.633957650253,103.631456305703,103.672557568463),
 .UNSPECIFIED.);
#858=B_SPLINE_CURVE_WITH_KNOTS('',3,(#31226,#31227,#31228,#31229,#31230,
#31231,#31232,#31233,#31234,#31235),.UNSPECIFIED.,.F.,.F.,(4,1,1,1,1,1,
1,4),(97.3893722612837,98.1880280706196,99.1855267260701,100.183025381521,
101.180524036971,102.178022692422,103.175521347872,103.672557568463),
 .UNSPECIFIED.);
#859=B_SPLINE_CURVE_WITH_KNOTS('',3,(#31240,#31241,#31242,#31243,#31244,
#31245,#31246,#31247,#31248,#31249),.UNSPECIFIED.,.F.,.F.,(4,1,1,1,1,1,
1,4),(91.106186954104,91.6614724402973,92.6589710957478,93.6564697511983,
94.6539684066488,95.6514670620993,96.6489657175498,97.3893722612837),
 .UNSPECIFIED.);
#860=B_SPLINE_CURVE_WITH_KNOTS('',3,(#31250,#31251,#31252,#31253,#31254,
#31255,#31256,#31257,#31258,#31259,#31260),.UNSPECIFIED.,.F.,.F.,(4,1,1,
1,1,1,1,1,4),(91.106186954104,91.2055374824661,92.2030361379166,93.2005347933671,
94.1980334488176,95.1955321042681,96.1930307597186,97.1905294151691,97.3893722612837),
 .UNSPECIFIED.);
#861=B_SPLINE_CURVE_WITH_KNOTS('',3,(#31265,#31266,#31267,#31268,#31269,
#31270,#31271,#31272,#31273,#31274),.UNSPECIFIED.,.F.,.F.,(4,1,1,1,1,1,
1,4),(84.8230016469245,85.6764805075943,86.6739791630448,87.6714778184953,
88.6689764739458,89.6664751293963,90.6639737848468,91.106186954104),
 .UNSPECIFIED.);
#862=B_SPLINE_CURVE_WITH_KNOTS('',3,(#31275,#31276,#31277,#31278,#31279,
#31280,#31281,#31282,#31283,#31284),.UNSPECIFIED.,.F.,.F.,(4,1,1,1,1,1,
1,4),(84.8230016469245,85.2205455497631,86.2180442052136,87.2155428606641,
88.2130415161146,89.2105401715651,90.2080388270156,91.106186954104),
 .UNSPECIFIED.);
#863=B_SPLINE_CURVE_WITH_KNOTS('',3,(#31289,#31290,#31291,#31292,#31293,
#31294,#31295,#31296,#31297,#31298,#31299),.UNSPECIFIED.,.F.,.F.,(4,1,1,
1,1,1,1,1,4),(78.5398163397448,78.6939899194408,79.6914885748913,80.6889872303418,
81.6864858857923,82.6839845412428,83.6814831966933,84.6789818521438,84.8230016469245),
 .UNSPECIFIED.);
#864=B_SPLINE_CURVE_WITH_KNOTS('',3,(#31300,#31301,#31302,#31303,#31304,
#31305,#31306,#31307,#31308,#31309),.UNSPECIFIED.,.F.,.F.,(4,1,1,1,1,1,
1,4),(78.5398163397448,79.2355536170601,80.2330522725106,81.2305509279611,
82.2280495834116,83.2255482388621,84.2230468943126,84.8230016469245),
 .UNSPECIFIED.);
#865=B_SPLINE_CURVE_WITH_KNOTS('',3,(#31314,#31315,#31316,#31317,#31318,
#31319,#31320,#31321,#31322,#31323),.UNSPECIFIED.,.F.,.F.,(4,1,1,1,1,1,
1,4),(72.2566310325652,72.7089979867378,73.7064966421883,74.7039952976388,
75.7014939530893,76.6989926085398,77.6964912639903,78.5398163397448),
 .UNSPECIFIED.);
#866=B_SPLINE_CURVE_WITH_KNOTS('',3,(#31324,#31325,#31326,#31327,#31328,
#31329,#31330,#31331,#31332,#31333),.UNSPECIFIED.,.F.,.F.,(4,1,1,1,1,1,
1,4),(72.2566310325652,73.2505616843571,74.2480603398076,75.2455589952581,
76.2430576507086,77.2405563061591,78.2380549616096,78.5398163397448),
 .UNSPECIFIED.);
#867=B_SPLINE_CURVE_WITH_KNOTS('',3,(#31338,#31339,#31340,#31341,#31342,
#31343,#31344,#31345,#31346,#31347),.UNSPECIFIED.,.F.,.F.,(4,1,1,1,1,1,
1,4),(65.9734457253856,66.7240060540348,67.7215047094853,68.7190033649358,
69.7165020203863,70.7140006758368,71.7114993312873,72.2566310325652),
 .UNSPECIFIED.);
#868=B_SPLINE_CURVE_WITH_KNOTS('',3,(#31348,#31349,#31350,#31351,#31352,
#31353,#31354,#31355,#31356,#31357,#31358),.UNSPECIFIED.,.F.,.F.,(4,1,1,
1,1,1,1,1,4),(65.9734457253856,66.2680710962036,67.2655697516541,68.2630684071046,
69.2605670625551,70.2580657180056,71.2555643734561,72.2530630289066,72.2566310325652),
 .UNSPECIFIED.);
#869=B_SPLINE_CURVE_WITH_KNOTS('',3,(#31363,#31364,#31365,#31366,#31367,
#31368,#31369,#31370,#31371,#31372,#31373),.UNSPECIFIED.,.F.,.F.,(4,1,1,
1,1,1,1,1,4),(59.690260418206,59.7415154658813,60.7390141213318,61.7365127767823,
62.7340114322328,63.7315100876833,64.7290087431338,65.7265073985843,65.9734457253856),
 .UNSPECIFIED.);
#870=B_SPLINE_CURVE_WITH_KNOTS('',3,(#31374,#31375,#31376,#31377,#31378,
#31379,#31380,#31381,#31382,#31383),.UNSPECIFIED.,.F.,.F.,(4,1,1,1,1,1,
1,4),(59.690260418206,60.2830791635006,61.2805778189511,62.2780764744016,
63.2755751298521,64.2730737853026,65.2705724407531,65.9734457253856),
 .UNSPECIFIED.);
#871=B_SPLINE_CURVE_WITH_KNOTS('',3,(#31388,#31389,#31390,#31391,#31392,
#31393,#31394,#31395,#31396,#31397),.UNSPECIFIED.,.F.,.F.,(4,1,1,1,1,1,
1,4),(53.4070751110264,53.7565235331783,54.7540221886288,55.7515208440793,
56.7490194995298,57.7465181549803,58.7440168104308,59.690260418206),
 .UNSPECIFIED.);
#872=B_SPLINE_CURVE_WITH_KNOTS('',3,(#31398,#31399,#31400,#31401,#31402,
#31403,#31404,#31405,#31406,#31407),.UNSPECIFIED.,.F.,.F.,(4,1,1,1,1,1,
1,4),(53.4070751110264,54.2980872307976,55.2955858862481,56.2930845416986,
57.2905831971491,58.2880818525996,59.2855805080501,59.690260418206),
 .UNSPECIFIED.);
#873=B_SPLINE_CURVE_WITH_KNOTS('',3,(#31412,#31413,#31414,#31415,#31416,
#31417,#31418,#31419,#31420,#31421),.UNSPECIFIED.,.F.,.F.,(4,1,1,1,1,1,
1,4),(47.1238898038468,47.7715316004753,48.7690302559258,49.7665289113763,
50.7640275668268,51.7615262222773,52.7590248777278,53.4070751110264),
 .UNSPECIFIED.);
#874=B_SPLINE_CURVE_WITH_KNOTS('',3,(#31422,#31423,#31424,#31425,#31426,
#31427,#31428,#31429,#31430,#31431,#31432),.UNSPECIFIED.,.F.,.F.,(4,1,1,
1,1,1,1,1,4),(47.1238898038468,47.3155966426441,48.3130952980946,49.3105939535451,
50.3080926089956,51.3055912644461,52.3030899198966,53.3005885753471,53.4070751110264),
 .UNSPECIFIED.);
#875=B_SPLINE_CURVE_WITH_KNOTS('',3,(#31437,#31438,#31439,#31440,#31441,
#31442,#31443,#31444,#31445,#31446),.UNSPECIFIED.,.F.,.F.,(4,1,1,1,1,1,
1,4),(40.8407044966672,41.7865396677723,42.7840383232228,43.7815369786733,
44.7790356341238,45.7765342895743,46.7740329450248,47.1238898038468),
 .UNSPECIFIED.);
#876=B_SPLINE_CURVE_WITH_KNOTS('',3,(#31447,#31448,#31449,#31450,#31451,
#31452,#31453,#31454,#31455,#31456),.UNSPECIFIED.,.F.,.F.,(4,1,1,1,1,1,
1,4),(40.8407044966672,41.3306047099411,42.3281033653916,43.3256020208421,
44.3231006762926,45.3205993317431,46.3180979871936,47.1238898038468),
 .UNSPECIFIED.);
#877=B_SPLINE_CURVE_WITH_KNOTS('',3,(#31461,#31462,#31463,#31464,#31465,
#31466,#31467,#31468,#31469,#31470,#31471),.UNSPECIFIED.,.F.,.F.,(4,1,1,
1,1,1,1,1,4),(34.5575191894876,34.8040490796188,35.8015477350693,36.7990463905198,
37.7965450459703,38.7940437014208,39.7915423568713,40.7890410123218,40.8407044966672),
 .UNSPECIFIED.);
#878=B_SPLINE_CURVE_WITH_KNOTS('',3,(#31472,#31473,#31474,#31475,#31476,
#31477,#31478,#31479,#31480,#31481),.UNSPECIFIED.,.F.,.F.,(4,1,1,1,1,1,
1,4),(34.5575191894876,35.3456127772381,36.3431114326886,37.3406100881391,
38.3381087435896,39.3356073990401,40.3331060544906,40.8407044966672),
 .UNSPECIFIED.);
#879=B_SPLINE_CURVE_WITH_KNOTS('',3,(#31486,#31487,#31488,#31489,#31490,
#31491,#31492,#31493,#31494,#31495),.UNSPECIFIED.,.F.,.F.,(4,1,1,1,1,1,
1,4),(28.2743338823079,28.8190571469158,29.8165558023663,30.8140544578168,
31.8115531132673,32.8090517687178,33.8065504241683,34.5575191894876),
 .UNSPECIFIED.);
#880=B_SPLINE_CURVE_WITH_KNOTS('',3,(#31496,#31497,#31498,#31499,#31500,
#31501,#31502,#31503,#31504,#31505,#31506),.UNSPECIFIED.,.F.,.F.,(4,1,1,
1,1,1,1,1,4),(28.2743338823079,28.3631221890846,29.3606208445351,30.3581194999856,
31.3556181554361,32.3531168108866,33.3506154663371,34.3481141217876,34.5575191894876),
 .UNSPECIFIED.);
#881=B_SPLINE_CURVE_WITH_KNOTS('',3,(#31511,#31512,#31513,#31514,#31515,
#31516,#31517,#31518,#31519,#31520),.UNSPECIFIED.,.F.,.F.,(4,1,1,1,1,1,
1,4),(21.9911485751283,22.8340652142128,23.8315638696633,24.8290625251138,
25.8265611805643,26.8240598360148,27.8215584914653,28.2743338823079),
 .UNSPECIFIED.);
#882=B_SPLINE_CURVE_WITH_KNOTS('',3,(#31521,#31522,#31523,#31524,#31525,
#31526,#31527,#31528,#31529,#31530),.UNSPECIFIED.,.F.,.F.,(4,1,1,1,1,1,
1,4),(21.9911485751283,22.3781302563816,23.3756289118321,24.3731275672826,
25.3706262227331,26.3681248781836,27.3656235336341,28.2743338823079),
 .UNSPECIFIED.);
#883=B_SPLINE_CURVE_WITH_KNOTS('',3,(#31536,#31537,#31538,#31539,#31540),
 .UNSPECIFIED.,.F.,.F.,(4,1,4),(14.3981410127776,15.3956396682281,15.707963267949),
 .UNSPECIFIED.);
#884=B_SPLINE_CURVE_WITH_KNOTS('',3,(#31543,#31544,#31545,#31546,#31547),
 .UNSPECIFIED.,.F.,.F.,(4,1,4),(13.8761928695319,14.8540759706088,15.7079632679487),
 .UNSPECIFIED.);
#885=B_SPLINE_CURVE_WITH_KNOTS('',3,(#31549,#31550,#31551,#31552,#31553,
#31554,#31555,#31556,#31557,#31558,#31559,#31560,#31561,#31562,#31563,#31564,
#31565,#31566,#31567,#31568,#31569,#31570,#31571,#31572,#31573,#31574,#31575,
#31576,#31577,#31578,#31579,#31580,#31581,#31582,#31583,#31584,#31585,#31586,
#31587,#31588,#31589,#31590,#31591,#31592,#31593,#31594,#31595,#31596,#31597,
#31598,#31599,#31600,#31601,#31602,#31603,#31604,#31605,#31606,#31607,#31608,
#31609,#31610,#31611,#31612,#31613,#31614,#31615,#31616,#31617,#31618,#31619,
#31620,#31621,#31622,#31623,#31624,#31625,#31626,#31627,#31628,#31629,#31630,
#31631,#31632,#31633,#31634,#31635,#31636),.UNSPECIFIED.,.F.,.F.,(4,3,3,
3,3,3,3,3,3,3,3,3,3,3,3,3,3,3,3,3,3,3,3,3,3,3,3,3,3,4),(-0.378621596831491,
-0.359799974259491,-0.347867720488378,-0.339795904888389,-0.335415766246889,
-0.315546491055276,-0.301208576176833,-0.297330142863398,-0.293235364838415,
-0.272834900814394,-0.252137033433983,-0.23931356808242,-0.228820743229234,
-0.224509894764592,-0.203205274087435,-0.200843172027728,-0.180354289318363,
-0.158315828378964,-0.154363755179046,-0.150814789240723,-0.129430304994364,
-0.107595617692396,-0.0856289754902388,-0.080208065969872,-0.0759455790412052,
-0.0533977706849842,-0.0308256528945546,-0.00876661790841547,-0.00404660180317386,
0.),.UNSPECIFIED.);
#886=B_SPLINE_CURVE_WITH_KNOTS('',3,(#31637,#31638,#31639,#31640,#31641,
#31642,#31643,#31644,#31645,#31646,#31647,#31648,#31649,#31650,#31651,#31652,
#31653,#31654,#31655,#31656,#31657,#31658,#31659,#31660,#31661,#31662,#31663,
#31664,#31665,#31666,#31667,#31668,#31669,#31670,#31671,#31672,#31673,#31674,
#31675,#31676,#31677,#31678,#31679,#31680,#31681,#31682,#31683,#31684,#31685,
#31686,#31687,#31688,#31689,#31690,#31691,#31692,#31693,#31694,#31695,#31696,
#31697,#31698,#31699,#31700,#31701,#31702,#31703,#31704,#31705,#31706,#31707,
#31708,#31709,#31710,#31711,#31712,#31713,#31714,#31715,#31716,#31717,#31718,
#31719,#31720,#31721),.UNSPECIFIED.,.F.,.F.,(4,3,3,3,3,3,3,3,3,3,3,3,3,
3,3,3,3,3,3,3,3,3,3,3,3,3,3,3,4),(-0.37694081721165,-0.35463588075101,-0.332914954557582,
-0.328066888666082,-0.305818294401826,-0.290199566502046,-0.284267361548342,
-0.278599939690394,-0.256916538505875,-0.235698318877041,-0.214945663233777,
-0.208192982084683,-0.204402876940358,-0.183826063192256,-0.180868471203588,
-0.159885877939655,-0.140312002594425,-0.136050822944271,-0.13260723132917,
-0.112148152518366,-0.0917831465515227,-0.0718536005353655,-0.0676631141183089,
-0.0636717608241292,-0.0441132632842336,-0.02492609063918,-0.0063612278911709,
-0.00329487517781129,0.),.UNSPECIFIED.);
#887=B_SPLINE_CURVE_WITH_KNOTS('',3,(#31723,#31724,#31725,#31726,#31727,
#31728,#31729,#31730,#31731,#31732,#31733),.UNSPECIFIED.,.F.,.F.,(4,1,1,
1,1,1,1,1,4),(15.7079632679487,15.8515746260593,16.8490732815098,17.8465719369603,
18.8440705924108,19.8415692478613,20.8390679033118,21.8365665587623,21.9911485751283),
 .UNSPECIFIED.);
#888=B_SPLINE_CURVE_WITH_KNOTS('',3,(#31734,#31735,#31736,#31737,#31738,
#31739,#31740,#31741,#31742,#31743),.UNSPECIFIED.,.F.,.F.,(4,1,1,1,1,1,
1,4),(15.707963267949,16.3931383236786,17.3906369791291,18.3881356345796,
19.3856342900301,20.3831329454806,21.3806316009311,21.9911485751283),
 .UNSPECIFIED.);
#889=B_SPLINE_CURVE_WITH_KNOTS('',3,(#32232,#32233,#32234,#32235,#32236,
#32237,#32238,#32239,#32240,#32241,#32242,#32243,#32244,#32245,#32246,#32247,
#32248,#32249,#32250,#32251,#32252,#32253,#32254,#32255,#32256,#32257,#32258,
#32259,#32260,#32261,#32262,#32263,#32264,#32265,#32266,#32267,#32268,#32269,
#32270,#32271,#32272,#32273,#32274,#32275,#32276,#32277,#32278,#32279,#32280,
#32281,#32282,#32283,#32284,#32285,#32286,#32287,#32288,#32289,#32290,#32291,
#32292,#32293,#32294,#32295,#32296,#32297,#32298,#32299,#32300,#32301,#32302,
#32303,#32304,#32305,#32306,#32307,#32308,#32309,#32310,#32311,#32312,#32313),
 .UNSPECIFIED.,.F.,.F.,(4,3,3,3,3,3,3,3,3,3,3,3,3,3,3,3,3,3,3,3,3,3,3,3,
3,3,3,4),(0.,0.018594885873403,0.0384194798631932,0.0557659996042597,0.0644652503371223,
0.0684490524568481,0.0885013376974244,0.108910426790898,0.125980729541105,
0.133839897547683,0.137280413419243,0.158355507126299,0.177191637791725,
0.1977206197196,0.205647900544446,0.209124298098342,0.23013147760292,0.25162452459456,
0.268078695962123,0.278325048323282,0.284043739612251,0.306312804123555,
0.322962328214973,0.328177032612165,0.333185055167668,0.355706471451577,
0.372910900489228,0.37694081721157),.UNSPECIFIED.);
#890=B_SPLINE_CURVE_WITH_KNOTS('',3,(#32314,#32315,#32316,#32317,#32318,
#32319,#32320,#32321,#32322,#32323,#32324,#32325,#32326,#32327,#32328,#32329,
#32330,#32331,#32332,#32333,#32334,#32335,#32336,#32337,#32338),
 .UNSPECIFIED.,.F.,.F.,(4,3,3,3,3,3,3,3,4),(-10.1295685708712,-9.974986554505,
-8.9774878990545,-7.979989243604,-6.9824905881535,-5.984991932703,-4.9874932772525,
-3.989994621802,-3.84638326369162),.UNSPECIFIED.);
#891=B_SPLINE_CURVE_WITH_KNOTS('',3,(#32827,#32828,#32829,#32830,#32831,
#32832,#32833,#32834,#32835,#32836,#32837,#32838,#32839,#32840,#32841,#32842,
#32843,#32844,#32845,#32846,#32847,#32848),.UNSPECIFIED.,.F.,.F.,(4,3,3,
3,3,3,3,4),(7.59300756235069,7.979989243604,8.97748789905449,9.97498655450499,
10.9724852099555,11.969983865406,12.9674825208565,13.8761928695303),
 .UNSPECIFIED.);
#892=B_SPLINE_CURVE_WITH_KNOTS('',3,(#32849,#32850,#32851,#32852,#32853,
#32854,#32855,#32856,#32857,#32858,#32859,#32860,#32861,#32862,#32863,#32864,
#32865,#32866,#32867,#32868,#32869,#32870,#32871,#32872,#32873,#32874,#32875,
#32876,#32877,#32878,#32879,#32880,#32881,#32882,#32883,#32884,#32885,#32886,
#32887,#32888,#32889,#32890,#32891,#32892,#32893,#32894,#32895,#32896,#32897,
#32898,#32899,#32900,#32901,#32902,#32903,#32904,#32905,#32906,#32907,#32908,
#32909,#32910,#32911,#32912,#32913,#32914,#32915,#32916,#32917,#32918,#32919,
#32920,#32921,#32922,#32923,#32924,#32925,#32926,#32927,#32928,#32929,#32930,
#32931,#32932,#32933),.UNSPECIFIED.,.F.,.F.,(4,3,3,3,3,3,3,3,3,3,3,3,3,
3,3,3,3,3,3,3,3,3,3,3,3,3,3,3,4),(0.,0.0219639704547416,0.0445412096053718,
0.0636172943766679,0.0720964150895219,0.0767535446244105,0.0810482748727846,
0.102994889675057,0.124771807731429,0.142866327742507,0.150422049143916,
0.153915429401351,0.157566138461075,0.17833757213313,0.19714988777574,0.219420483792499,
0.224320878182838,0.22940319248336,0.250068207912569,0.270729023241509,
0.285676322508746,0.29689251627475,0.300623397883779,0.320396471336199,
0.334299980346825,0.338766705971823,0.357793075396352,0.375314655909808,
0.378621596831459),.UNSPECIFIED.);
#893=B_SPLINE_CURVE_WITH_KNOTS('',3,(#32936,#32937,#32938,#32939,#32940,
#32941,#32942,#32943,#32944,#32945,#32946,#32947,#32948,#32949,#32950,#32951,
#32952,#32953,#32954,#32955,#32956,#32957,#32958,#32959,#32960,#32961,#32962,
#32963,#32964,#32965,#32966,#32967,#32968,#32969,#32970,#32971,#32972,#32973,
#32974,#32975,#32976,#32977,#32978,#32979,#32980,#32981,#32982,#32983,#32984,
#32985,#32986,#32987,#32988,#32989,#32990,#32991,#32992,#32993,#32994,#32995,
#32996,#32997,#32998,#32999,#33000,#33001,#33002,#33003,#33004,#33005,#33006,
#33007,#33008,#33009,#33010,#33011,#33012,#33013,#33014,#33015,#33016,#33017,
#33018,#33019,#33020,#33021,#33022,#33023),.UNSPECIFIED.,.F.,.F.,(4,3,3,
3,3,3,3,3,3,3,3,3,3,3,3,3,3,3,3,3,3,3,3,3,3,3,3,3,3,4),(-0.378621596831415,
-0.359799982681486,-0.347867741892736,-0.339796092108079,-0.335415835589243,
-0.315546567792779,-0.301208643322146,-0.297330292477441,-0.293235380625517,
-0.272834922399814,-0.2521370543926,-0.23931358380138,-0.228820766465177,
-0.224509902039135,-0.203205281153447,-0.20084317202772,-0.18035428381319,
-0.158315823561941,-0.154363723715015,-0.150814783989309,-0.129430295261392,
-0.107595605944727,-0.0856289636990593,-0.0802080454028315,-0.0759455719174419,
-0.0533977626018103,-0.0308256449926057,-0.00876660921494158,-0.00404660180319711,
0.),.UNSPECIFIED.);
#894=B_SPLINE_CURVE_WITH_KNOTS('',3,(#33024,#33025,#33026,#33027,#33028,
#33029,#33030,#33031,#33032,#33033,#33034,#33035,#33036,#33037,#33038,#33039,
#33040,#33041,#33042,#33043,#33044,#33045,#33046,#33047,#33048,#33049,#33050,
#33051,#33052,#33053,#33054,#33055,#33056,#33057,#33058,#33059,#33060,#33061,
#33062,#33063,#33064,#33065,#33066,#33067,#33068,#33069,#33070,#33071,#33072,
#33073,#33074,#33075,#33076,#33077,#33078,#33079,#33080,#33081,#33082,#33083,
#33084,#33085,#33086,#33087,#33088,#33089,#33090,#33091,#33092,#33093,#33094,
#33095,#33096,#33097,#33098,#33099,#33100,#33101,#33102,#33103,#33104,#33105,
#33106,#33107,#33108),.UNSPECIFIED.,.F.,.F.,(4,3,3,3,3,3,3,3,3,3,3,3,3,
3,3,3,3,3,3,3,3,3,3,3,3,3,3,3,4),(-0.376940817211667,-0.35463587601936,
-0.332914950417388,-0.328066883946824,-0.305818289667664,-0.290199562359655,
-0.284267352350603,-0.278599940314396,-0.256916539828167,-0.235698322125015,
-0.214945667731477,-0.208192979048904,-0.20440287735044,-0.1838260654653,
-0.180868471203587,-0.159885877932906,-0.140312002588519,-0.136050825693189,
-0.132607233423575,-0.112148154257823,-0.0917831486981529,-0.0718536049354341,
-0.0676631265382839,-0.0636717646905323,-0.0441132683370721,-0.0249260984199674,
-0.00636124025136225,-0.00329487517780647,0.),.UNSPECIFIED.);
#895=B_SPLINE_CURVE_WITH_KNOTS('',3,(#33110,#33111,#33112,#33113,#33114,
#33115,#33116,#33117,#33118,#33119,#33120),.UNSPECIFIED.,.F.,.F.,(4,1,1,
1,1,1,1,1,4),(15.707963267949,15.8515746260587,16.8490732815092,17.8465719369597,
18.8440705924102,19.8415692478607,20.8390679033112,21.8365665587617,21.9911485751283),
 .UNSPECIFIED.);
#896=B_SPLINE_CURVE_WITH_KNOTS('',3,(#33121,#33122,#33123,#33124,#33125,
#33126,#33127,#33128,#33129,#33130),.UNSPECIFIED.,.F.,.F.,(4,1,1,1,1,1,
1,4),(15.707963267949,16.393138323678,17.3906369791285,18.388135634579,
19.3856342900295,20.38313294548,21.3806316009305,21.9911485751283),
 .UNSPECIFIED.);
#897=B_SPLINE_CURVE_WITH_KNOTS('',3,(#33619,#33620,#33621,#33622,#33623,
#33624,#33625,#33626,#33627,#33628,#33629,#33630,#33631,#33632,#33633,#33634,
#33635,#33636,#33637,#33638,#33639,#33640,#33641,#33642,#33643,#33644,#33645,
#33646,#33647,#33648,#33649,#33650,#33651,#33652,#33653,#33654,#33655,#33656,
#33657,#33658,#33659,#33660,#33661,#33662,#33663,#33664,#33665,#33666,#33667,
#33668,#33669,#33670,#33671,#33672,#33673,#33674,#33675,#33676,#33677,#33678,
#33679,#33680,#33681,#33682,#33683,#33684,#33685,#33686,#33687,#33688,#33689,
#33690,#33691,#33692,#33693,#33694,#33695,#33696,#33697,#33698,#33699,#33700),
 .UNSPECIFIED.,.F.,.F.,(4,3,3,3,3,3,3,3,3,3,3,3,3,3,3,3,3,3,3,3,3,3,3,3,
3,3,3,4),(0.,0.0185948935798831,0.0384194866063638,0.0557660055045345,0.0644652605573106,
0.0684490550799758,0.0885013458730424,0.108910437440259,0.125980737528127,
0.133839910140703,0.137280419791478,0.158355512918852,0.177191637791729,
0.197720615992758,0.205647898698541,0.20912429682451,0.230131471962516,
0.251624516628207,0.268078697930462,0.278325052897778,0.284043738565929,
0.306312802790669,0.322962327215306,0.328177030451769,0.333185054058664,
0.355706470426897,0.372910900489216,0.376940817211557),.UNSPECIFIED.);
#898=B_SPLINE_CURVE_WITH_KNOTS('',3,(#33701,#33702,#33703,#33704,#33705,
#33706,#33707,#33708,#33709,#33710,#33711,#33712,#33713,#33714,#33715,#33716,
#33717,#33718,#33719,#33720,#33721,#33722,#33723,#33724,#33725),
 .UNSPECIFIED.,.F.,.F.,(4,3,3,3,3,3,3,3,4),(-10.1295685708719,-9.97498655450499,
-8.97748789905449,-7.979989243604,-6.9824905881535,-5.984991932703,-4.9874932772525,
-3.989994621802,-3.84638326369226),.UNSPECIFIED.);
#899=B_SPLINE_CURVE_WITH_KNOTS('',3,(#34214,#34215,#34216,#34217,#34218,
#34219,#34220,#34221,#34222,#34223,#34224,#34225,#34226,#34227,#34228,#34229,
#34230,#34231,#34232,#34233,#34234,#34235),.UNSPECIFIED.,.F.,.F.,(4,3,3,
3,3,3,3,4),(7.59300756235133,7.979989243604,8.97748789905451,9.97498655450501,
10.9724852099555,11.969983865406,12.9674825208565,13.8761928695309),
 .UNSPECIFIED.);
#900=B_SPLINE_CURVE_WITH_KNOTS('',3,(#34236,#34237,#34238,#34239,#34240,
#34241,#34242,#34243,#34244,#34245,#34246,#34247,#34248,#34249,#34250,#34251,
#34252,#34253,#34254,#34255,#34256,#34257,#34258,#34259,#34260,#34261,#34262,
#34263,#34264,#34265,#34266,#34267,#34268,#34269,#34270,#34271,#34272,#34273,
#34274,#34275,#34276,#34277,#34278,#34279,#34280,#34281,#34282,#34283,#34284,
#34285,#34286,#34287,#34288,#34289,#34290,#34291,#34292,#34293,#34294,#34295,
#34296,#34297,#34298,#34299,#34300,#34301,#34302,#34303,#34304,#34305,#34306,
#34307,#34308,#34309,#34310,#34311,#34312,#34313,#34314,#34315,#34316,#34317,
#34318,#34319,#34320),.UNSPECIFIED.,.F.,.F.,(4,3,3,3,3,3,3,3,3,3,3,3,3,
3,3,3,3,3,3,3,3,3,3,3,3,3,3,3,4),(0.,0.0219639631218642,0.0445412014823461,
0.0636172872690209,0.0720964129740222,0.0767535401253322,0.0810482736599176,
0.1029948885196,0.124771808689427,0.142866328461006,0.150422048595144,0.153915426485005,
0.157566137611273,0.17833757339743,0.197149887775744,0.219420483792504,
0.224320878636298,0.229403192489738,0.250068207587221,0.270729023024861,
0.285676328241119,0.296892526281026,0.300623400781932,0.320396476514032,
0.334299989050446,0.338766713939552,0.357793087087158,0.375314655909825,
0.378621596831476),.UNSPECIFIED.);
#901=B_SPLINE_CURVE_WITH_KNOTS('',3,(#34323,#34324,#34325,#34326,#34327,
#34328,#34329,#34330,#34331,#34332,#34333,#34334,#34335,#34336,#34337,#34338,
#34339,#34340,#34341,#34342,#34343,#34344,#34345,#34346,#34347,#34348,#34349,
#34350,#34351,#34352,#34353,#34354,#34355,#34356,#34357,#34358,#34359,#34360,
#34361,#34362,#34363,#34364,#34365,#34366,#34367,#34368,#34369,#34370,#34371,
#34372,#34373,#34374,#34375,#34376,#34377,#34378,#34379,#34380,#34381,#34382,
#34383,#34384,#34385,#34386,#34387,#34388,#34389,#34390,#34391,#34392,#34393,
#34394,#34395,#34396,#34397,#34398,#34399,#34400,#34401,#34402,#34403,#34404,
#34405,#34406,#34407,#34408,#34409,#34410),.UNSPECIFIED.,.F.,.F.,(4,3,3,
3,3,3,3,3,3,3,3,3,3,3,3,3,3,3,3,3,3,3,3,3,3,3,3,3,3,4),(-0.378621596831342,
-0.359799978647325,-0.347867731642752,-0.339796002462411,-0.335415802350538,
-0.315546531014861,-0.301208611141465,-0.297330220816646,-0.293235373064883,
-0.272834912064565,-0.252137044356719,-0.239313576274462,-0.228820755338192,
-0.224509898510171,-0.203205277724662,-0.200843172027689,-0.180354286447876,
-0.158315825867291,-0.154363738841701,-0.1508147865132,-0.129430299930584,
-0.107595611579441,-0.0856289693581657,-0.0802080552723695,-0.0759455753061188,
-0.0533977664431355,-0.0308256487487178,-0.00876661335280336,-0.00404660180319768,
0.),.UNSPECIFIED.);
#902=B_SPLINE_CURVE_WITH_KNOTS('',3,(#34411,#34412,#34413,#34414,#34415,
#34416,#34417,#34418,#34419,#34420,#34421,#34422,#34423,#34424,#34425,#34426,
#34427,#34428,#34429,#34430,#34431,#34432,#34433,#34434,#34435,#34436,#34437,
#34438,#34439,#34440,#34441,#34442,#34443,#34444,#34445,#34446,#34447,#34448,
#34449,#34450,#34451,#34452,#34453,#34454,#34455,#34456,#34457,#34458,#34459,
#34460,#34461,#34462,#34463,#34464,#34465,#34466,#34467,#34468,#34469,#34470,
#34471,#34472,#34473,#34474,#34475,#34476,#34477,#34478,#34479,#34480,#34481,
#34482,#34483,#34484,#34485,#34486,#34487,#34488,#34489,#34490,#34491,#34492,
#34493,#34494,#34495),.UNSPECIFIED.,.F.,.F.,(4,3,3,3,3,3,3,3,3,3,3,3,3,
3,3,3,3,3,3,3,3,3,3,3,3,3,3,3,4),(-0.376940817211729,-0.354635873302002,
-0.332914948039702,-0.328066881211475,-0.305818286928304,-0.290199559962716,
-0.284267347028432,-0.278599940670464,-0.256916540583258,-0.235698323984283,
-0.21494567030162,-0.208192977306597,-0.204402877464087,-0.183826066657456,
-0.180868471203602,-0.159885877922097,-0.140312002579062,-0.13605082724227,
-0.132607234529552,-0.112148155157824,-0.0917831498359287,-0.0718536073792482,
-0.0676631334737326,-0.0636717668358761,-0.0441132711599333,-0.024926102814774,
-0.00636124727006412,-0.00329487517781668,0.),.UNSPECIFIED.);
#903=B_SPLINE_CURVE_WITH_KNOTS('',3,(#34497,#34498,#34499,#34500,#34501,
#34502,#34503,#34504,#34505,#34506,#34507),.UNSPECIFIED.,.F.,.F.,(4,1,1,
1,1,1,1,1,4),(15.707963267949,15.851574626059,16.8490732815095,17.84657193696,
18.8440705924105,19.841569247861,20.8390679033115,21.836566558762,21.9911485751283),
 .UNSPECIFIED.);
#904=B_SPLINE_CURVE_WITH_KNOTS('',3,(#34508,#34509,#34510,#34511,#34512,
#34513,#34514,#34515,#34516,#34517),.UNSPECIFIED.,.F.,.F.,(4,1,1,1,1,1,
1,4),(15.707963267949,16.3931383236783,17.3906369791288,18.3881356345793,
19.3856342900298,20.3831329454803,21.3806316009308,21.9911485751283),
 .UNSPECIFIED.);
#905=B_SPLINE_CURVE_WITH_KNOTS('',3,(#35006,#35007,#35008,#35009,#35010,
#35011,#35012,#35013,#35014,#35015,#35016,#35017,#35018,#35019,#35020,#35021,
#35022,#35023,#35024,#35025,#35026,#35027,#35028,#35029,#35030,#35031,#35032,
#35033,#35034,#35035,#35036,#35037,#35038,#35039,#35040,#35041,#35042,#35043,
#35044,#35045,#35046,#35047,#35048,#35049,#35050,#35051,#35052,#35053,#35054,
#35055,#35056,#35057,#35058,#35059,#35060,#35061,#35062,#35063,#35064,#35065,
#35066,#35067,#35068,#35069,#35070,#35071,#35072,#35073,#35074,#35075,#35076,
#35077,#35078,#35079,#35080,#35081,#35082,#35083,#35084,#35085,#35086,#35087),
 .UNSPECIFIED.,.F.,.F.,(4,3,3,3,3,3,3,3,3,3,3,3,3,3,3,3,3,3,3,3,3,3,3,3,
3,3,3,4),(0.,0.0185948979987812,0.0384194904729007,0.0557660088877552,0.0644652664176503,
0.0684490565818861,0.0885013505592445,0.108910443544607,0.12598074210639,
0.133839917359234,0.137280423449418,0.158355516244424,0.177191637791737,
0.197720613855199,0.205647897639485,0.209124296087971,0.230131468721749,
0.251624512053417,0.268078699062201,0.278325055529064,0.284043737962168,
0.306312802022573,0.322962326639242,0.328177029191476,0.333185053418253,
0.355706469834782,0.372910900489249,0.376940817211591),.UNSPECIFIED.);
#906=B_SPLINE_CURVE_WITH_KNOTS('',3,(#35088,#35089,#35090,#35091,#35092,
#35093,#35094,#35095,#35096,#35097,#35098,#35099,#35100,#35101,#35102,#35103,
#35104,#35105,#35106,#35107,#35108,#35109,#35110,#35111,#35112),
 .UNSPECIFIED.,.F.,.F.,(4,3,3,3,3,3,3,3,4),(-10.1295685708716,-9.974986554505,
-8.9774878990545,-7.979989243604,-6.9824905881535,-5.984991932703,-4.9874932772525,
-3.989994621802,-3.84638326369194),.UNSPECIFIED.);
#907=B_SPLINE_CURVE_WITH_KNOTS('',3,(#35601,#35602,#35603,#35604,#35605,
#35606,#35607,#35608,#35609,#35610,#35611,#35612,#35613,#35614,#35615,#35616,
#35617,#35618,#35619,#35620,#35621,#35622),.UNSPECIFIED.,.F.,.F.,(4,3,3,
3,3,3,3,4),(7.59300756235101,7.979989243604,8.97748789905451,9.974986554505,
10.9724852099555,11.969983865406,12.9674825208565,13.8761928695306),
 .UNSPECIFIED.);
#908=B_SPLINE_CURVE_WITH_KNOTS('',3,(#35623,#35624,#35625,#35626,#35627,
#35628,#35629,#35630,#35631,#35632,#35633,#35634,#35635,#35636,#35637,#35638,
#35639,#35640,#35641,#35642,#35643,#35644,#35645,#35646,#35647,#35648,#35649,
#35650,#35651,#35652,#35653,#35654,#35655,#35656,#35657,#35658,#35659,#35660,
#35661,#35662,#35663,#35664,#35665,#35666,#35667,#35668,#35669,#35670,#35671,
#35672,#35673,#35674,#35675,#35676,#35677,#35678,#35679,#35680,#35681,#35682,
#35683,#35684,#35685,#35686,#35687,#35688,#35689,#35690,#35691,#35692,#35693,
#35694,#35695,#35696,#35697,#35698,#35699,#35700,#35701,#35702,#35703,#35704,
#35705,#35706,#35707),.UNSPECIFIED.,.F.,.F.,(4,3,3,3,3,3,3,3,3,3,3,3,3,
3,3,3,3,3,3,3,3,3,3,3,3,3,3,3,4),(0.,0.0219639666312835,0.0445412053698155,
0.063617290670558,0.0720964139865945,0.0767535422787978,0.0810482742366969,
0.102994889069381,0.124771808227842,0.142866328114821,0.150422048856047,
0.153915427873857,0.157566138016919,0.178337572791375,0.197149887775755,
0.219420483792515,0.224320878419338,0.229403192482163,0.250068207738402,
0.270729023124161,0.285676325486174,0.29689252147315,0.300623399390804,
0.320396474032259,0.334299984879898,0.338766710117096,0.357793081483418,
0.375314655909829,0.378621596831479),.UNSPECIFIED.);
#909=B_SPLINE_CURVE_WITH_KNOTS('',3,(#35710,#35711,#35712,#35713,#35714,
#35715,#35716,#35717,#35718,#35719,#35720,#35721,#35722,#35723,#35724,#35725,
#35726,#35727,#35728,#35729,#35730,#35731,#35732,#35733,#35734,#35735,#35736,
#35737,#35738,#35739,#35740,#35741,#35742,#35743,#35744,#35745,#35746,#35747,
#35748,#35749,#35750,#35751,#35752,#35753,#35754,#35755,#35756,#35757,#35758,
#35759,#35760,#35761,#35762,#35763,#35764,#35765,#35766,#35767,#35768,#35769,
#35770,#35771,#35772,#35773,#35774,#35775,#35776,#35777,#35778,#35779,#35780,
#35781,#35782,#35783,#35784,#35785,#35786,#35787,#35788,#35789,#35790,#35791,
#35792,#35793,#35794,#35795,#35796,#35797),.UNSPECIFIED.,.F.,.F.,(4,3,3,
3,3,3,3,3,3,3,3,3,3,3,3,3,3,3,3,3,3,3,3,3,3,3,3,3,3,4),(-0.378621596831322,
-0.359799969507972,-0.347867708396688,-0.33979579913089,-0.335415727239428,
-0.315546447878259,-0.301208538396937,-0.297330058742659,-0.29323535595745,
-0.272834888678764,-0.252137021650703,-0.239313559244948,-0.228820730165096,
-0.224509890616438,-0.203205270049206,-0.200843172027682,-0.180354292423732,
-0.158315831096164,-0.154363773062407,-0.150814792225547,-0.129430310507984,
-0.107595624341076,-0.0856289821639265,-0.0802080776082638,-0.0759455830362766,
-0.0533977752247224,-0.0308256573292537,-0.00876662278122885,-0.00404660180318586,
0.),.UNSPECIFIED.);
#910=B_SPLINE_CURVE_WITH_KNOTS('',3,(#35798,#35799,#35800,#35801,#35802,
#35803,#35804,#35805,#35806,#35807,#35808,#35809,#35810,#35811,#35812,#35813,
#35814,#35815,#35816,#35817,#35818,#35819,#35820,#35821,#35822,#35823,#35824,
#35825,#35826,#35827,#35828,#35829,#35830,#35831,#35832,#35833,#35834,#35835,
#35836,#35837,#35838,#35839,#35840,#35841,#35842,#35843,#35844,#35845,#35846,
#35847,#35848,#35849,#35850,#35851,#35852,#35853,#35854,#35855,#35856,#35857,
#35858,#35859,#35860,#35861,#35862,#35863,#35864,#35865,#35866,#35867,#35868,
#35869,#35870,#35871,#35872,#35873,#35874,#35875,#35876,#35877,#35878,#35879,
#35880,#35881,#35882),.UNSPECIFIED.,.F.,.F.,(4,3,3,3,3,3,3,3,3,3,3,3,3,
3,3,3,3,3,3,3,3,3,3,3,3,3,3,3,4),(-0.376940817211723,-0.354635878503461,
-0.332914952590979,-0.328066886478521,-0.305818292205571,-0.290199564580325,
-0.284267357272115,-0.278599940003547,-0.256916539151692,-0.235698320438349,
-0.21494566539322,-0.208192980636845,-0.20440287701073,-0.183826064152281,
-0.180868471203602,-0.159885877939701,-0.140312002594464,-0.136050824265609,
-0.132607232292872,-0.112148153313923,-0.091783147541673,-0.0718536026117019,
-0.0676631199850014,-0.0636717626539058,-0.044113265676923,-0.024926094327708,
-0.00636123375821928,-0.00329487517780647,0.),.UNSPECIFIED.);
#911=B_SPLINE_CURVE_WITH_KNOTS('',3,(#35884,#35885,#35886,#35887,#35888,
#35889,#35890,#35891,#35892,#35893,#35894),.UNSPECIFIED.,.F.,.F.,(4,1,1,
1,1,1,1,1,4),(15.707963267949,15.851574626059,16.8490732815095,17.84657193696,
18.8440705924105,19.841569247861,20.8390679033115,21.836566558762,21.9911485751283),
 .UNSPECIFIED.);
#912=B_SPLINE_CURVE_WITH_KNOTS('',3,(#35895,#35896,#35897,#35898,#35899,
#35900,#35901,#35902,#35903,#35904),.UNSPECIFIED.,.F.,.F.,(4,1,1,1,1,1,
1,4),(15.707963267949,16.3931383236783,17.3906369791288,18.3881356345793,
19.3856342900298,20.3831329454803,21.3806316009308,21.9911485751283),
 .UNSPECIFIED.);
#913=B_SPLINE_CURVE_WITH_KNOTS('',3,(#36393,#36394,#36395,#36396,#36397,
#36398,#36399,#36400,#36401,#36402,#36403,#36404,#36405,#36406,#36407,#36408,
#36409,#36410,#36411,#36412,#36413,#36414,#36415,#36416,#36417,#36418,#36419,
#36420,#36421,#36422,#36423,#36424,#36425,#36426,#36427,#36428,#36429,#36430,
#36431,#36432,#36433,#36434,#36435,#36436,#36437,#36438,#36439,#36440,#36441,
#36442,#36443,#36444,#36445,#36446,#36447,#36448,#36449,#36450,#36451,#36452,
#36453,#36454,#36455,#36456,#36457,#36458,#36459,#36460,#36461,#36462,#36463,
#36464,#36465,#36466,#36467,#36468,#36469,#36470,#36471,#36472,#36473,#36474),
 .UNSPECIFIED.,.F.,.F.,(4,3,3,3,3,3,3,3,3,3,3,3,3,3,3,3,3,3,3,3,3,3,3,3,
3,3,3,4),(0.,0.0185948895377003,0.0384194830694538,0.0557660024097381,0.0644652551966428,
0.0684490537106689,0.0885013415914402,0.108910431860699,0.125980733343456,
0.133839903542633,0.13728041645897,0.158355509890479,0.177191637791728,
0.197720617947217,0.205647899666576,0.209124297504269,0.230131474933047,
0.25162452081887,0.268078696891712,0.278325050479978,0.284043739119617,
0.306312803494651,0.322962327743294,0.328177031572274,0.333185054637632,
0.355706470961523,0.372910900489225,0.376940817211566),.UNSPECIFIED.);
#914=B_SPLINE_CURVE_WITH_KNOTS('',3,(#36475,#36476,#36477,#36478,#36479,
#36480,#36481,#36482,#36483,#36484,#36485,#36486,#36487,#36488,#36489,#36490,
#36491,#36492,#36493,#36494,#36495,#36496,#36497,#36498,#36499),
 .UNSPECIFIED.,.F.,.F.,(4,3,3,3,3,3,3,3,4),(-10.1295685708716,-9.974986554505,
-8.9774878990545,-7.979989243604,-6.9824905881535,-5.984991932703,-4.9874932772525,
-3.989994621802,-3.84638326369194),.UNSPECIFIED.);
#915=B_SPLINE_CURVE_WITH_KNOTS('',3,(#36988,#36989,#36990,#36991,#36992,
#36993,#36994,#36995,#36996,#36997,#36998,#36999,#37000,#37001,#37002,#37003,
#37004,#37005,#37006,#37007,#37008,#37009),.UNSPECIFIED.,.F.,.F.,(4,3,3,
3,3,3,3,4),(7.59300756235101,7.979989243604,8.97748789905451,9.974986554505,
10.9724852099555,11.969983865406,12.9674825208565,13.8761928695306),
 .UNSPECIFIED.);
#916=B_SPLINE_CURVE_WITH_KNOTS('',3,(#37010,#37011,#37012,#37013,#37014,
#37015,#37016,#37017,#37018,#37019,#37020,#37021,#37022,#37023,#37024,#37025,
#37026,#37027,#37028,#37029,#37030,#37031,#37032,#37033,#37034,#37035,#37036,
#37037,#37038,#37039,#37040,#37041,#37042,#37043,#37044,#37045,#37046,#37047,
#37048,#37049,#37050,#37051,#37052,#37053,#37054,#37055,#37056,#37057,#37058,
#37059,#37060,#37061,#37062,#37063,#37064,#37065,#37066,#37067,#37068,#37069,
#37070,#37071,#37072,#37073,#37074,#37075,#37076,#37077,#37078,#37079,#37080,
#37081,#37082,#37083,#37084,#37085,#37086,#37087,#37088,#37089,#37090,#37091,
#37092,#37093,#37094),.UNSPECIFIED.,.F.,.F.,(4,3,3,3,3,3,3,3,3,3,3,3,3,
3,3,3,3,3,3,3,3,3,3,3,3,3,3,3,4),(0.,0.0219639745899241,0.0445412141859538,
0.0636172983846773,0.0720964162823181,0.0767535471614663,0.0810482755548609,
0.10299489032468,0.124771807189166,0.14286632733581,0.150422049452129,0.153915431031089,
0.157566138937898,0.178337571417637,0.197149887775741,0.219420483792501,
0.224320877927013,0.229403192462999,0.25006820807906,0.270729023346635,
0.285676319229185,0.296892510554946,0.300623396232423,0.320396468398677,
0.33429997541392,0.338766701437846,0.357793068763078,0.375314655909822,
0.378621596831473),.UNSPECIFIED.);
#917=B_SPLINE_CURVE_WITH_KNOTS('',3,(#37101,#37102,#37103,#37104,#37105,
#37106,#37107,#37108,#37109,#37110,#37111,#37112,#37113,#37114,#37115,#37116,
#37117,#37118,#37119,#37120,#37121,#37122,#37123,#37124,#37125,#37126,#37127,
#37128,#37129,#37130,#37131,#37132,#37133,#37134,#37135,#37136,#37137,#37138,
#37139,#37140,#37141,#37142,#37143,#37144,#37145,#37146,#37147,#37148,#37149,
#37150,#37151,#37152,#37153,#37154,#37155,#37156,#37157,#37158,#37159,#37160,
#37161,#37162,#37163,#37164,#37165,#37166,#37167,#37168,#37169,#37170,#37171,
#37172,#37173,#37174,#37175,#37176,#37177,#37178,#37179,#37180,#37181,#37182,
#37183,#37184,#37185,#37186,#37187,#37188),.UNSPECIFIED.,.F.,.F.,(4,3,3,
3,3,3,3,3,3,3,3,3,3,3,3,3,3,3,3,3,3,3,3,3,3,3,3,3,3,4),(-0.378621596831422,
-0.359796720372466,-0.347859447299365,-0.339722632399601,-0.335384312800265,
-0.315512099822729,-0.301178483848345,-0.297262500366189,-0.293227435760253,
-0.272824713995647,-0.252127134942234,-0.23930614421359,-0.228809794789834,
-0.224506446570609,-0.203201941946953,-0.200843172027657,-0.18035647359203,
-0.15831773961842,-0.154376205977353,-0.150816849886109,-0.129434137392224,
-0.107600238535838,-0.0856336136104227,-0.0802161718332497,-0.0759483538506766,
-0.0534009168486348,-0.0308287327199469,-0.00877004870084194,-0.00404660180315077,
0.),.UNSPECIFIED.);
#918=B_SPLINE_CURVE_WITH_KNOTS('',3,(#37189,#37190,#37191,#37192,#37193,
#37194,#37195,#37196,#37197,#37198,#37199,#37200,#37201,#37202,#37203,#37204,
#37205,#37206,#37207,#37208,#37209,#37210,#37211,#37212,#37213,#37214,#37215,
#37216,#37217,#37218,#37219,#37220,#37221,#37222,#37223,#37224,#37225,#37226,
#37227,#37228,#37229,#37230,#37231,#37232,#37233,#37234,#37235,#37236,#37237,
#37238,#37239,#37240,#37241,#37242,#37243,#37244,#37245,#37246,#37247,#37248,
#37249,#37250,#37251,#37252,#37253,#37254,#37255,#37256,#37257,#37258,#37259,
#37260,#37261,#37262,#37263,#37264,#37265,#37266,#37267,#37268,#37269,#37270,
#37271,#37272,#37273),.UNSPECIFIED.,.F.,.F.,(4,3,3,3,3,3,3,3,3,3,3,3,3,
3,3,3,3,3,3,3,3,3,3,3,3,3,3,3,4),(-0.376940817211671,-0.35463378592243,
-0.332913121582575,-0.328064780620112,-0.305816203186943,-0.290197736689024,
-0.284263301474814,-0.278600204901399,-0.25691713780292,-0.235699797645294,
-0.214947714870497,-0.208191635443227,-0.204403035574647,-0.183827074928476,
-0.180868471203591,-0.159885881087144,-0.140312005348477,-0.136052161826863,
-0.132608232099475,-0.112149009613445,-0.0917842308919543,-0.0718557743436045,
-0.0660574195493053,-0.0628401741813833,-0.0432952248143112,-0.0232950499960591,
-0.0047591197577418,-0.00329487517780703,0.),.UNSPECIFIED.);
#919=B_SPLINE_CURVE_WITH_KNOTS('',3,(#37275,#37276,#37277,#37278,#37279,
#37280,#37281,#37282,#37283,#37284,#37285),.UNSPECIFIED.,.F.,.F.,(4,1,1,
1,1,1,1,1,4),(15.7079632679488,15.8515746260587,16.8490732815092,17.8465719369597,
18.8440705924102,19.8415692478607,20.8390679033112,21.8365665587617,21.9911485751284),
 .UNSPECIFIED.);
#920=B_SPLINE_CURVE_WITH_KNOTS('',3,(#37286,#37287,#37288,#37289,#37290,
#37291,#37292,#37293,#37294,#37295),.UNSPECIFIED.,.F.,.F.,(4,1,1,1,1,1,
1,4),(15.7079632679489,16.3931383236779,17.3906369791284,18.3881356345789,
19.3856342900294,20.3831329454799,21.3806316009304,21.9911485751284),
 .UNSPECIFIED.);
#921=B_SPLINE_CURVE_WITH_KNOTS('',3,(#37784,#37785,#37786,#37787,#37788,
#37789,#37790,#37791,#37792,#37793,#37794,#37795,#37796,#37797,#37798,#37799,
#37800,#37801,#37802,#37803,#37804,#37805,#37806,#37807,#37808,#37809,#37810,
#37811,#37812,#37813,#37814,#37815,#37816,#37817,#37818,#37819,#37820,#37821,
#37822,#37823,#37824,#37825,#37826,#37827,#37828,#37829,#37830,#37831,#37832,
#37833,#37834,#37835,#37836,#37837,#37838,#37839,#37840,#37841,#37842,#37843,
#37844,#37845,#37846,#37847,#37848,#37849,#37850,#37851,#37852,#37853,#37854,
#37855,#37856,#37857,#37858,#37859,#37860,#37861,#37862,#37863,#37864,#37865),
 .UNSPECIFIED.,.F.,.F.,(4,3,3,3,3,3,3,3,3,3,3,3,3,3,3,3,3,3,3,3,3,3,3,3,
3,3,3,4),(0.,0.0185983140321727,0.0384224795021175,0.0557686242883193,0.0644697932614127,
0.0684502210277478,0.0885049607621097,0.108915120509374,0.125984249829963,
0.13384544115498,0.137283243835269,0.158358039582652,0.177191637791731,
0.197718921929196,0.205647026423371,0.209123684847396,0.230128871311592,
0.25162086484219,0.268079555535016,0.278327028951233,0.284043271874226,
0.306312209751215,0.32296188243573,0.32817603610564,0.333184545813206,0.35570598540302,
0.372910900489273,0.376940817211655),.UNSPECIFIED.);
#922=B_SPLINE_CURVE_WITH_KNOTS('',3,(#37866,#37867,#37868,#37869,#37870,
#37871,#37872,#37873,#37874,#37875,#37876,#37877,#37878,#37879,#37880,#37881,
#37882,#37883,#37884,#37885,#37886,#37887,#37888,#37889,#37890),
 .UNSPECIFIED.,.F.,.F.,(4,3,3,3,3,3,3,3,4),(-10.1295685708718,-9.97498655450501,
-8.97748789905451,-7.97998924360401,-6.98249058815351,-5.98499193270301,
-4.98749327725251,-3.98999462180201,-3.84638326369218),.UNSPECIFIED.);
#923=B_SPLINE_CURVE_WITH_KNOTS('',3,(#38379,#38380,#38381,#38382,#38383,
#38384,#38385,#38386,#38387,#38388,#38389,#38390,#38391,#38392,#38393,#38394,
#38395,#38396,#38397,#38398,#38399,#38400),.UNSPECIFIED.,.F.,.F.,(4,3,3,
3,3,3,3,4),(7.59300756235149,7.97998924360401,8.97748789905451,9.97498655450502,
10.9724852099555,11.969983865406,12.9674825208565,13.8761928695311),
 .UNSPECIFIED.);
#924=B_SPLINE_CURVE_WITH_KNOTS('',3,(#38401,#38402,#38403,#38404,#38405,
#38406,#38407,#38408,#38409,#38410,#38411,#38412,#38413,#38414,#38415,#38416,
#38417,#38418,#38419,#38420,#38421,#38422,#38423,#38424,#38425,#38426,#38427,
#38428,#38429,#38430,#38431,#38432,#38433,#38434,#38435,#38436,#38437,#38438,
#38439,#38440,#38441,#38442,#38443,#38444,#38445,#38446,#38447,#38448,#38449,
#38450,#38451,#38452,#38453,#38454,#38455,#38456,#38457,#38458,#38459,#38460,
#38461,#38462,#38463,#38464,#38465,#38466,#38467,#38468,#38469,#38470,#38471,
#38472,#38473,#38474,#38475,#38476,#38477,#38478,#38479,#38480,#38481,#38482,
#38483,#38484,#38485),.UNSPECIFIED.,.F.,.F.,(4,3,3,3,3,3,3,3,3,3,3,3,3,
3,3,3,3,3,3,3,3,3,3,3,3,3,3,3,4),(0.,0.0219667982761558,0.0445443217220367,
0.0636200174787497,0.0720972266024481,0.0767552653548233,0.0810487382353878,
0.102995309296695,0.124771387449721,0.142866012531226,0.150422220722031,
0.153916412782485,0.157566438108027,0.178337033896873,0.197149887775741,
0.219420483792492,0.224320671605659,0.229403188154647,0.250068321092155,
0.270729057144868,0.285673893016582,0.296888246100129,0.300622182306411,
0.32039429496601,0.334296359328725,0.33876343006628,0.357788259279217,0.375314655909755,
0.378621596831423),.UNSPECIFIED.);
#925=B_SPLINE_CURVE_WITH_KNOTS('',3,(#38488,#38489,#38490,#38491,#38492,
#38493,#38494,#38495,#38496,#38497,#38498,#38499,#38500,#38501,#38502,#38503,
#38504,#38505,#38506,#38507,#38508,#38509,#38510,#38511,#38512,#38513,#38514,
#38515,#38516,#38517,#38518,#38519,#38520,#38521,#38522,#38523,#38524,#38525,
#38526,#38527,#38528,#38529,#38530,#38531,#38532,#38533,#38534,#38535,#38536,
#38537,#38538,#38539,#38540,#38541,#38542,#38543,#38544,#38545,#38546,#38547,
#38548,#38549,#38550,#38551,#38552,#38553,#38554,#38555,#38556,#38557,#38558,
#38559,#38560,#38561,#38562,#38563,#38564,#38565,#38566,#38567,#38568,#38569,
#38570,#38571,#38572,#38573,#38574,#38575),.UNSPECIFIED.,.F.,.F.,(4,3,3,
3,3,3,3,3,3,3,3,3,3,3,3,3,3,3,3,3,3,3,3,3,3,3,3,3,3,4),(-0.378621596831422,
-0.359796715870711,-0.347859435880365,-0.339722530007006,-0.335384262776704,
-0.315512045618215,-0.301178436419395,-0.29726239278539,-0.29322742189176,
-0.272824696964274,-0.252127118373726,-0.239306131787209,-0.228809776489813,
-0.224506440767185,-0.20320193635774,-0.200843172027657,-0.180356476691574,
-0.158317742330522,-0.154376223555756,-0.150816852768337,-0.129434142783147,
-0.107600245031064,-0.0856336201278072,-0.080216183244537,-0.0759483577713782,
-0.0534009212866121,-0.0308287370694683,-0.00877005360278791,-0.00404660180315077,
0.),.UNSPECIFIED.);
#926=B_SPLINE_CURVE_WITH_KNOTS('',3,(#38576,#38577,#38578,#38579,#38580,
#38581,#38582,#38583,#38584,#38585,#38586,#38587,#38588,#38589,#38590,#38591,
#38592,#38593,#38594,#38595,#38596,#38597,#38598,#38599,#38600,#38601,#38602,
#38603,#38604,#38605,#38606,#38607,#38608,#38609,#38610,#38611,#38612,#38613,
#38614,#38615,#38616,#38617,#38618,#38619,#38620,#38621,#38622,#38623,#38624,
#38625,#38626,#38627,#38628,#38629,#38630,#38631,#38632,#38633,#38634,#38635,
#38636,#38637,#38638,#38639,#38640,#38641,#38642,#38643,#38644,#38645,#38646,
#38647,#38648,#38649,#38650,#38651,#38652,#38653,#38654,#38655,#38656,#38657,
#38658,#38659,#38660),.UNSPECIFIED.,.F.,.F.,(4,3,3,3,3,3,3,3,3,3,3,3,3,
3,3,3,3,3,3,3,3,3,3,3,3,3,3,3,4),(-0.376940817211671,-0.354633785210935,
-0.332913120960017,-0.328064779829376,-0.305816202409768,-0.290197736008996,
-0.284263299980245,-0.278600205016827,-0.256917138043544,-0.235699798192756,
-0.214947715616542,-0.208191634969854,-0.20440303563573,-0.183827075288029,
-0.180868471203591,-0.159885881090851,-0.14031200535172,-0.136052162326922,
-0.132608232466673,-0.112149009937429,-0.0917842313090905,-0.071855775169603,
-0.0660574218689477,-0.0628401747625342,-0.0432952256330311,-0.0232950504054191,
-0.00475912097892364,-0.00329487517780703,0.),.UNSPECIFIED.);
#927=B_SPLINE_CURVE_WITH_KNOTS('',3,(#38662,#38663,#38664,#38665,#38666,
#38667,#38668,#38669,#38670,#38671,#38672),.UNSPECIFIED.,.F.,.F.,(4,1,1,
1,1,1,1,1,4),(15.7079632679488,15.8515746260587,16.8490732815092,17.8465719369597,
18.8440705924102,19.8415692478607,20.8390679033112,21.8365665587617,21.9911485751284),
 .UNSPECIFIED.);
#928=B_SPLINE_CURVE_WITH_KNOTS('',3,(#38673,#38674,#38675,#38676,#38677,
#38678,#38679,#38680,#38681,#38682),.UNSPECIFIED.,.F.,.F.,(4,1,1,1,1,1,
1,4),(15.7079632679489,16.3931383236779,17.3906369791284,18.3881356345789,
19.3856342900294,20.3831329454799,21.3806316009304,21.9911485751284),
 .UNSPECIFIED.);
#929=B_SPLINE_CURVE_WITH_KNOTS('',3,(#39171,#39172,#39173,#39174,#39175,
#39176,#39177,#39178,#39179,#39180,#39181,#39182,#39183,#39184,#39185,#39186,
#39187,#39188,#39189,#39190,#39191,#39192,#39193,#39194,#39195,#39196,#39197,
#39198,#39199,#39200,#39201,#39202,#39203,#39204,#39205,#39206,#39207,#39208,
#39209,#39210,#39211,#39212,#39213,#39214,#39215,#39216,#39217,#39218,#39219,
#39220,#39221,#39222,#39223,#39224,#39225,#39226,#39227,#39228,#39229,#39230,
#39231,#39232,#39233,#39234,#39235,#39236,#39237,#39238,#39239,#39240,#39241,
#39242,#39243,#39244,#39245,#39246,#39247,#39248,#39249,#39250,#39251,#39252),
 .UNSPECIFIED.,.F.,.F.,(4,3,3,3,3,3,3,3,3,3,3,3,3,3,3,3,3,3,3,3,3,3,3,3,
3,3,3,4),(0.,0.018598315202886,0.0384224805264917,0.0557686251846467,0.0644697948116091,
0.0684502214259709,0.0885049619928401,0.108915122095826,0.125984251019803,
0.133845443026534,0.137283244809287,0.158358040441789,0.177191637791731,
0.197718921336747,0.205647026107811,0.209123684625284,0.230128870392712,
0.251620863557925,0.268079555819901,0.278327029600694,0.284043271715027,
0.306312209549515,0.322961882284454,0.328176035756772,0.33318454563508,
0.355705985227969,0.372910900489273,0.376940817211655),.UNSPECIFIED.);
#930=B_SPLINE_CURVE_WITH_KNOTS('',3,(#39253,#39254,#39255,#39256,#39257,
#39258,#39259,#39260,#39261,#39262,#39263,#39264,#39265,#39266,#39267,#39268,
#39269,#39270,#39271,#39272,#39273,#39274,#39275,#39276,#39277),
 .UNSPECIFIED.,.F.,.F.,(4,3,3,3,3,3,3,3,4),(-10.1295685708718,-9.97498655450501,
-8.97748789905451,-7.97998924360401,-6.98249058815351,-5.98499193270301,
-4.98749327725251,-3.98999462180201,-3.84638326369218),.UNSPECIFIED.);
#931=B_SPLINE_CURVE_WITH_KNOTS('',3,(#39766,#39767,#39768,#39769,#39770,
#39771,#39772,#39773,#39774,#39775,#39776,#39777,#39778,#39779,#39780,#39781,
#39782,#39783,#39784,#39785,#39786,#39787),.UNSPECIFIED.,.F.,.F.,(4,3,3,
3,3,3,3,4),(7.59300756235149,7.97998924360401,8.97748789905451,9.97498655450502,
10.9724852099555,11.969983865406,12.9674825208565,13.8761928695311),
 .UNSPECIFIED.);
#932=B_SPLINE_CURVE_WITH_KNOTS('',3,(#39788,#39789,#39790,#39791,#39792,
#39793,#39794,#39795,#39796,#39797,#39798,#39799,#39800,#39801,#39802,#39803,
#39804,#39805,#39806,#39807,#39808,#39809,#39810,#39811,#39812,#39813,#39814,
#39815,#39816,#39817,#39818,#39819,#39820,#39821,#39822,#39823,#39824,#39825,
#39826,#39827,#39828,#39829,#39830,#39831,#39832,#39833,#39834,#39835,#39836,
#39837,#39838,#39839,#39840,#39841,#39842,#39843,#39844,#39845,#39846,#39847,
#39848,#39849,#39850,#39851,#39852,#39853,#39854,#39855,#39856,#39857,#39858,
#39859,#39860,#39861,#39862,#39863,#39864,#39865,#39866,#39867,#39868,#39869,
#39870,#39871,#39872),.UNSPECIFIED.,.F.,.F.,(4,3,3,3,3,3,3,3,3,3,3,3,3,
3,3,3,3,3,3,3,3,3,3,3,3,3,3,3,4),(0.,0.0219668021829663,0.0445443259943986,
0.0636200212170664,0.072097227717834,0.0767552677136324,0.0810487388755533,
0.102995309847675,0.124771386807676,0.142866012049692,0.150422220909751,
0.153916413967334,0.157566438486861,0.178337033089236,0.197149887775741,
0.219420483792492,0.224320671278011,0.229403188144959,0.250068321231503,
0.27072905712376,0.285673889363844,0.296888239638748,0.300622180494816,
0.320394291714806,0.33429635396776,0.33876342528417,0.357788252225625,0.375314655909755,
0.378621596831423),.UNSPECIFIED.);
#933=B_SPLINE_CURVE_WITH_KNOTS('',3,(#39875,#39876,#39877,#39878,#39879,
#39880,#39881,#39882,#39883,#39884,#39885,#39886,#39887,#39888,#39889,#39890,
#39891,#39892,#39893,#39894,#39895,#39896,#39897,#39898,#39899,#39900,#39901,
#39902,#39903,#39904,#39905,#39906,#39907,#39908,#39909,#39910,#39911,#39912,
#39913,#39914,#39915,#39916,#39917,#39918,#39919,#39920,#39921,#39922,#39923,
#39924,#39925,#39926,#39927,#39928,#39929,#39930,#39931,#39932,#39933,#39934,
#39935,#39936,#39937,#39938,#39939,#39940,#39941,#39942,#39943,#39944,#39945,
#39946,#39947,#39948,#39949,#39950,#39951,#39952,#39953,#39954,#39955,#39956,
#39957,#39958,#39959,#39960,#39961,#39962),.UNSPECIFIED.,.F.,.F.,(4,3,3,
3,3,3,3,3,3,3,3,3,3,3,3,3,3,3,3,3,3,3,3,3,3,3,3,3,3,4),(-0.378621596831447,
-0.359796710872288,-0.347859423166103,-0.33972241597309,-0.335384206951527,
-0.315511985148213,-0.301178383508145,-0.297262272762722,-0.293227406416186,
-0.272824677970899,-0.252127099894785,-0.239306117928005,-0.228809756083023,
-0.224506434279775,-0.20320193009925,-0.200843172027666,-0.180356480134043,
-0.158317745342681,-0.154376243245955,-0.15081685599556,-0.129434148792156,
-0.107600252262854,-0.0856336273826065,-0.0802161959430344,-0.0759483620831669,
-0.0534009261697563,-0.0308287418563685,-0.00877005900130109,-0.00404660180315016,
0.),.UNSPECIFIED.);
#934=B_SPLINE_CURVE_WITH_KNOTS('',3,(#39963,#39964,#39965,#39966,#39967,
#39968,#39969,#39970,#39971,#39972,#39973,#39974,#39975,#39976,#39977,#39978,
#39979,#39980,#39981,#39982,#39983,#39984,#39985,#39986,#39987,#39988,#39989,
#39990,#39991,#39992,#39993,#39994,#39995,#39996,#39997,#39998,#39999,#40000,
#40001,#40002,#40003,#40004,#40005,#40006,#40007,#40008,#40009,#40010,#40011,
#40012,#40013,#40014,#40015,#40016,#40017,#40018,#40019,#40020,#40021,#40022,
#40023,#40024,#40025,#40026,#40027,#40028,#40029,#40030,#40031,#40032,#40033,
#40034,#40035,#40036,#40037,#40038,#40039,#40040,#40041,#40042,#40043,#40044,
#40045,#40046,#40047),.UNSPECIFIED.,.F.,.F.,(4,3,3,3,3,3,3,3,3,3,3,3,3,
3,3,3,3,3,3,3,3,3,3,3,3,3,3,3,4),(-0.376940817211671,-0.354633792851345,
-0.332913127645376,-0.328064787566693,-0.305816210006314,-0.290197742655974,
-0.284263314719502,-0.278600204072656,-0.256917135797309,-0.235699792648004,
-0.214947707908054,-0.208191639892869,-0.204403035028373,-0.183827071480399,
-0.180868471203591,-0.159885881051101,-0.140312005316939,-0.136052156980596,
-0.132608228475344,-0.112149006418658,-0.0917842267934174,-0.0718557663450377,
-0.0660573970583436,-0.0628401685443772,-0.0432952168894413,-0.0232950460336242,
-0.00475910796593208,-0.00329487517780703,0.),.UNSPECIFIED.);
#935=B_SPLINE_CURVE_WITH_KNOTS('',3,(#40049,#40050,#40051,#40052,#40053,
#40054,#40055,#40056,#40057,#40058,#40059),.UNSPECIFIED.,.F.,.F.,(4,1,1,
1,1,1,1,1,4),(15.7079632679488,15.8515746260587,16.8490732815092,17.8465719369597,
18.8440705924102,19.8415692478607,20.8390679033112,21.8365665587617,21.9911485751284),
 .UNSPECIFIED.);
#936=B_SPLINE_CURVE_WITH_KNOTS('',3,(#40060,#40061,#40062,#40063,#40064,
#40065,#40066,#40067,#40068,#40069),.UNSPECIFIED.,.F.,.F.,(4,1,1,1,1,1,
1,4),(15.7079632679489,16.3931383236779,17.3906369791284,18.3881356345789,
19.3856342900294,20.3831329454799,21.3806316009304,21.9911485751284),
 .UNSPECIFIED.);
#937=B_SPLINE_CURVE_WITH_KNOTS('',3,(#40558,#40559,#40560,#40561,#40562,
#40563,#40564,#40565,#40566,#40567,#40568,#40569,#40570,#40571,#40572,#40573,
#40574,#40575,#40576,#40577,#40578,#40579,#40580,#40581,#40582,#40583,#40584,
#40585,#40586,#40587,#40588,#40589,#40590,#40591,#40592,#40593,#40594,#40595,
#40596,#40597,#40598,#40599,#40600,#40601,#40602,#40603,#40604,#40605,#40606,
#40607,#40608,#40609,#40610,#40611,#40612,#40613,#40614,#40615,#40616,#40617,
#40618,#40619,#40620,#40621,#40622,#40623,#40624,#40625,#40626,#40627,#40628,
#40629,#40630,#40631,#40632,#40633,#40634,#40635,#40636,#40637,#40638,#40639),
 .UNSPECIFIED.,.F.,.F.,(4,3,3,3,3,3,3,3,3,3,3,3,3,3,3,3,3,3,3,3,3,3,3,3,
3,3,3,4),(0.,0.0185983026316204,0.0384224695266343,0.0557686155597714,0.0644697781641698,
0.0684502171318133,0.088504948753686,0.10891510503595,0.125984238224895,
0.133845422901441,0.137283234431239,0.158358031297179,0.177191637791731,
0.197718927698151,0.205647029496634,0.209123687024891,0.230128880274258,
0.251620877362912,0.268079552746722,0.278327022586856,0.284043273416826,
0.306312211709011,0.322961883904076,0.328176039524306,0.333184547554318,
0.355705987113168,0.372910900489273,0.376940817211655),.UNSPECIFIED.);
#938=B_SPLINE_CURVE_WITH_KNOTS('',3,(#40640,#40641,#40642,#40643,#40644,
#40645,#40646,#40647,#40648,#40649,#40650,#40651,#40652,#40653,#40654,#40655,
#40656,#40657,#40658,#40659,#40660,#40661,#40662,#40663,#40664),
 .UNSPECIFIED.,.F.,.F.,(4,3,3,3,3,3,3,3,4),(-10.1295685708718,-9.97498655450501,
-8.97748789905451,-7.97998924360401,-6.98249058815351,-5.98499193270301,
-4.98749327725251,-3.98999462180201,-3.84638326369218),.UNSPECIFIED.);
#939=B_SPLINE_CURVE_WITH_KNOTS('',3,(#41153,#41154,#41155,#41156,#41157,
#41158,#41159,#41160,#41161,#41162,#41163,#41164,#41165,#41166,#41167,#41168,
#41169,#41170,#41171,#41172,#41173,#41174),.UNSPECIFIED.,.F.,.F.,(4,3,3,
3,3,3,3,4),(7.59300756235149,7.97998924360401,8.97748789905451,9.97498655450501,
10.9724852099555,11.969983865406,12.9674825208565,13.8761928695311),
 .UNSPECIFIED.);
#940=B_SPLINE_CURVE_WITH_KNOTS('',3,(#41175,#41176,#41177,#41178,#41179,
#41180,#41181,#41182,#41183,#41184,#41185,#41186,#41187,#41188,#41189,#41190,
#41191,#41192,#41193,#41194,#41195,#41196,#41197,#41198,#41199,#41200,#41201,
#41202,#41203,#41204,#41205,#41206,#41207,#41208,#41209,#41210,#41211,#41212,
#41213,#41214,#41215,#41216,#41217,#41218,#41219,#41220,#41221,#41222,#41223,
#41224,#41225,#41226,#41227,#41228,#41229,#41230,#41231,#41232,#41233,#41234,
#41235,#41236,#41237,#41238,#41239,#41240,#41241,#41242,#41243,#41244,#41245,
#41246,#41247,#41248,#41249,#41250,#41251,#41252,#41253,#41254,#41255,#41256,
#41257,#41258,#41259),.UNSPECIFIED.,.F.,.F.,(4,3,3,3,3,3,3,3,3,3,3,3,3,
3,3,3,3,3,3,3,3,3,3,3,3,3,3,3,4),(0.,0.0219668065215099,0.044544330738594,
0.063620025368238,0.0720972289566785,0.0767552703331067,0.0810487395771697,
0.102995310450109,0.124771386085693,0.142866011508206,0.150422221112997,
0.153916415282172,0.157566438907463,0.178337032192192,0.197149887775746,
0.219420483792496,0.224320670914036,0.229403188139166,0.250068321391114,
0.270729057104618,0.28567388531636,0.29688823247747,0.300622178485964,0.320394288107146,
0.334296348018114,0.338763419960212,0.357788244378528,0.375314655909751,
0.378621596831419),.UNSPECIFIED.);
#941=B_SPLINE_CURVE_WITH_KNOTS('',3,(#41262,#41263,#41264,#41265,#41266,
#41267,#41268,#41269,#41270,#41271,#41272,#41273,#41274,#41275,#41276,#41277,
#41278,#41279,#41280,#41281,#41282,#41283,#41284,#41285,#41286,#41287,#41288,
#41289,#41290,#41291,#41292,#41293,#41294,#41295,#41296,#41297,#41298,#41299,
#41300,#41301,#41302,#41303,#41304,#41305,#41306,#41307,#41308,#41309,#41310,
#41311,#41312,#41313,#41314,#41315,#41316,#41317,#41318,#41319,#41320,#41321,
#41322,#41323,#41324,#41325,#41326,#41327,#41328,#41329,#41330,#41331,#41332,
#41333,#41334,#41335,#41336,#41337,#41338,#41339,#41340,#41341,#41342,#41343,
#41344,#41345,#41346,#41347,#41348,#41349),.UNSPECIFIED.,.F.,.F.,(4,3,3,
3,3,3,3,3,3,3,3,3,3,3,3,3,3,3,3,3,3,3,3,3,3,3,3,3,3,4),(-0.378621596831452,
-0.359796705378914,-0.347859409196764,-0.339722290714836,-0.335384145609123,
-0.315511918694978,-0.301178325361564,-0.297262140747381,-0.293227389389929,
-0.272824657081609,-0.252127079571064,-0.239306102685213,-0.228809733635619,
-0.224506427219249,-0.203201923301277,-0.200843172027663,-0.180356483920826,
-0.158317748656117,-0.15437626458939,-0.150816859497235,-0.129434155353511,
-0.107600260175084,-0.0856336353261905,-0.0802162098561028,-0.0759483668387633,
-0.0534009315506567,-0.0308287471341723,-0.00877006494761552,-0.00404660180315015,
0.),.UNSPECIFIED.);
#942=B_SPLINE_CURVE_WITH_KNOTS('',3,(#41350,#41351,#41352,#41353,#41354,
#41355,#41356,#41357,#41358,#41359,#41360,#41361,#41362,#41363,#41364,#41365,
#41366,#41367,#41368,#41369,#41370,#41371,#41372,#41373,#41374,#41375,#41376,
#41377,#41378,#41379,#41380,#41381,#41382,#41383,#41384,#41385,#41386,#41387,
#41388,#41389,#41390,#41391,#41392,#41393,#41394,#41395,#41396,#41397,#41398,
#41399,#41400,#41401,#41402,#41403,#41404,#41405,#41406,#41407,#41408,#41409,
#41410,#41411,#41412,#41413,#41414,#41415,#41416,#41417,#41418,#41419,#41420,
#41421,#41422,#41423,#41424,#41425,#41426,#41427,#41428,#41429,#41430,#41431,
#41432,#41433,#41434),.UNSPECIFIED.,.F.,.F.,(4,3,3,3,3,3,3,3,3,3,3,3,3,
3,3,3,3,3,3,3,3,3,3,3,3,3,3,3,4),(-0.37694081721169,-0.354633789541522,
-0.332913124749281,-0.328064784261468,-0.305816206760707,-0.290197739816068,
-0.284263308414124,-0.278600204509387,-0.256917136791431,-0.235699795068636,
-0.21494771125805,-0.208191637754358,-0.20440303529233,-0.183827073127399,
-0.180868471203594,-0.159885881066344,-0.140312005330277,-0.136052159286264,
-0.132608230235817,-0.112149007974764,-0.0917842287792549,-0.0718557701882082,
-0.0660574078525838,-0.0628401712479354,-0.0432952206848533,-0.0232950479313323,
-0.004759113596582,-0.00329487517781129,0.),.UNSPECIFIED.);
#943=B_SPLINE_CURVE_WITH_KNOTS('',3,(#41436,#41437,#41438,#41439,#41440,
#41441,#41442,#41443,#41444,#41445,#41446),.UNSPECIFIED.,.F.,.F.,(4,1,1,
1,1,1,1,1,4),(15.7079632679489,15.8515746260587,16.8490732815092,17.8465719369597,
18.8440705924102,19.8415692478607,20.8390679033112,21.8365665587617,21.9911485751284),
 .UNSPECIFIED.);
#944=B_SPLINE_CURVE_WITH_KNOTS('',3,(#41447,#41448,#41449,#41450,#41451,
#41452,#41453,#41454,#41455,#41456),.UNSPECIFIED.,.F.,.F.,(4,1,1,1,1,1,
1,4),(15.7079632679489,16.3931383236779,17.3906369791284,18.3881356345789,
19.3856342900294,20.3831329454799,21.3806316009304,21.9911485751284),
 .UNSPECIFIED.);
#945=B_SPLINE_CURVE_WITH_KNOTS('',3,(#41945,#41946,#41947,#41948,#41949,
#41950,#41951,#41952,#41953,#41954,#41955,#41956,#41957,#41958,#41959,#41960,
#41961,#41962,#41963,#41964,#41965,#41966,#41967,#41968,#41969,#41970,#41971,
#41972,#41973,#41974,#41975,#41976,#41977,#41978,#41979,#41980,#41981,#41982,
#41983,#41984,#41985,#41986,#41987,#41988,#41989,#41990,#41991,#41992,#41993,
#41994,#41995,#41996,#41997,#41998,#41999,#42000,#42001,#42002,#42003,#42004,
#42005,#42006,#42007,#42008,#42009,#42010,#42011,#42012,#42013,#42014,#42015,
#42016,#42017,#42018,#42019,#42020,#42021,#42022,#42023,#42024,#42025,#42026),
 .UNSPECIFIED.,.F.,.F.,(4,3,3,3,3,3,3,3,3,3,3,3,3,3,3,3,3,3,3,3,3,3,3,3,
3,3,3,4),(0.,0.0185983080711966,0.0384224742862614,0.0557686197244432,0.064469785367515,
0.0684502189902693,0.0885049544828708,0.108915112418223,0.125984243761596,
0.133845431610119,0.137283238917139,0.158358035249346,0.177191637791715,
0.197718924945687,0.205647028030362,0.20912368598177,0.230128875993472,
0.251620871384311,0.268079554079538,0.278327025631043,0.284043272680096,
0.306312210774225,0.32296188320297,0.328176037890519,0.333184546722924,
0.355705986296573,0.372910900489207,0.37694081721159),.UNSPECIFIED.);
#946=B_SPLINE_CURVE_WITH_KNOTS('',3,(#42027,#42028,#42029,#42030,#42031,
#42032,#42033,#42034,#42035,#42036,#42037,#42038,#42039,#42040,#42041,#42042,
#42043,#42044,#42045,#42046,#42047,#42048,#42049,#42050,#42051),
 .UNSPECIFIED.,.F.,.F.,(4,3,3,3,3,3,3,3,4),(-10.1295685708718,-9.97498655450501,
-8.97748789905451,-7.97998924360401,-6.98249058815351,-5.98499193270301,
-4.98749327725251,-3.98999462180201,-3.84638326369218),.UNSPECIFIED.);
#947=B_SPLINE_CURVE_WITH_KNOTS('',3,(#42540,#42541,#42542,#42543,#42544,
#42545,#42546,#42547,#42548,#42549,#42550,#42551,#42552,#42553,#42554,#42555,
#42556,#42557,#42558,#42559,#42560,#42561),.UNSPECIFIED.,.F.,.F.,(4,3,3,
3,3,3,3,4),(7.59300756235149,7.97998924360401,8.97748789905451,9.97498655450502,
10.9724852099555,11.969983865406,12.9674825208565,13.8761928695311),
 .UNSPECIFIED.);
#948=B_SPLINE_CURVE_WITH_KNOTS('',3,(#42562,#42563,#42564,#42565,#42566,
#42567,#42568,#42569,#42570,#42571,#42572,#42573,#42574,#42575,#42576,#42577,
#42578,#42579,#42580,#42581,#42582,#42583,#42584,#42585,#42586,#42587,#42588,
#42589,#42590,#42591,#42592,#42593,#42594,#42595,#42596,#42597,#42598,#42599,
#42600,#42601,#42602,#42603,#42604,#42605,#42606,#42607,#42608,#42609,#42610,
#42611,#42612,#42613,#42614,#42615,#42616,#42617,#42618,#42619,#42620,#42621,
#42622,#42623,#42624,#42625,#42626,#42627,#42628,#42629,#42630,#42631,#42632,
#42633,#42634,#42635,#42636,#42637,#42638,#42639,#42640,#42641,#42642,#42643,
#42644,#42645,#42646),.UNSPECIFIED.,.F.,.F.,(4,3,3,3,3,3,3,3,3,3,3,3,3,
3,3,3,3,3,3,3,3,3,3,3,3,3,3,3,4),(0.,0.0219668112926134,0.0445443359559021,
0.0636200299333845,0.0720972303188465,0.0767552732140828,0.0810487403619284,
0.102995311125728,0.124771385304016,0.142866010921953,0.150422221343388,
0.15391641673982,0.157566439371711,0.178337031207171,0.197149887775761,
0.219420483792519,0.224320670513702,0.229403188138886,0.250068321572831,
0.270729057089704,0.285673880884443,0.296888224632328,0.300622176283363,
0.320394284144993,0.334296341483546,0.338763414131696,0.357788235774701,
0.37531465590982,0.37862159683149),.UNSPECIFIED.);
#949=B_SPLINE_CURVE_WITH_KNOTS('',3,(#42678,#42679,#42680,#42681,#42682,
#42683,#42684,#42685,#42686,#42687,#42688,#42689,#42690,#42691,#42692,#42693,
#42694),.UNSPECIFIED.,.F.,.F.,(4,1,1,1,1,1,1,1,1,1,1,1,1,1,4),(15.7079632679489,
15.7742466509132,16.264560774171,16.7548748974288,17.2451890206866,17.7355031439444,
18.2258172672022,18.71613139046,19.2064455137178,19.6967596369755,20.1870737602333,
20.6773878834911,21.1677020067489,21.6580161300067,21.9911485751285),
 .UNSPECIFIED.);
#950=B_SPLINE_CURVE_WITH_KNOTS('',3,(#42695,#42696,#42697,#42698,#42699,
#42700,#42701,#42702,#42703,#42704,#42705,#42706,#42707,#42708,#42709,#42710,
#42711),.UNSPECIFIED.,.F.,.F.,(4,1,1,1,1,1,1,1,1,1,1,1,1,1,4),(15.7079632679489,
15.8693424967452,16.359656620003,16.8499707432608,17.3402848665186,17.8305989897764,
18.3209131130342,18.811227236292,19.3015413595498,19.7918554828076,20.2821696060654,
20.7724837293232,21.2627978525809,21.7531119758387,21.9911485751285),
 .UNSPECIFIED.);
#951=B_SPLINE_CURVE_WITH_KNOTS('',3,(#43092,#43093,#43094,#43095,#43096,
#43097,#43098,#43099,#43100,#43101,#43102,#43103,#43104,#43105,#43106,#43107,
#43108,#43109,#43110,#43111,#43112,#43113,#43114,#43115,#43116,#43117,#43118,
#43119,#43120,#43121,#43122,#43123,#43124,#43125,#43126,#43127,#43128,#43129,
#43130,#43131,#43132,#43133,#43134,#43135,#43136,#43137,#43138,#43139,#43140,
#43141,#43142,#43143,#43144,#43145,#43146,#43147,#43148,#43149,#43150,#43151,
#43152,#43153,#43154,#43155,#43156,#43157,#43158,#43159,#43160,#43161,#43162,
#43163,#43164,#43165,#43166,#43167,#43168,#43169,#43170,#43171,#43172,#43173,
#43174,#43175,#43176,#43177,#43178,#43179,#43180,#43181,#43182,#43183,#43184,
#43185,#43186,#43187,#43188,#43189,#43190,#43191,#43192,#43193,#43194,#43195,
#43196,#43197,#43198,#43199,#43200,#43201,#43202,#43203,#43204,#43205,#43206),
 .UNSPECIFIED.,.F.,.F.,(4,3,3,3,3,3,3,3,3,3,3,3,3,3,3,3,3,3,3,3,3,3,3,3,
3,3,3,3,3,3,3,3,3,3,3,3,3,3,4),(0.,0.0505708571042727,0.101542673109873,
0.152182389706113,0.202219346658589,0.225638835489441,0.233898271119954,
0.240735485265272,0.290357617639612,0.295897301981998,0.345686264875582,
0.395413843633949,0.441706626966609,0.453063312881571,0.461070828559911,
0.467176391962776,0.515730570603939,0.563915442824477,0.580584976964589,
0.629137535103161,0.657230420337627,0.674238537119372,0.682110594253873,
0.688083279696401,0.735480735434175,0.782731786350779,0.829225244483419,
0.853880616978884,0.886547113898524,0.894686952978892,0.901806441759792,
0.948290089624541,0.990020715302407,1.01021978261714,1.02166124456445,1.02855221389401,
1.0738110712865,1.11521259233601,1.14791015664657),.UNSPECIFIED.);
#952=B_SPLINE_CURVE_WITH_KNOTS('',3,(#43207,#43208,#43209,#43210,#43211,
#43212,#43213,#43214,#43215,#43216,#43217,#43218,#43219,#43220,#43221,#43222,
#43223,#43224,#43225,#43226,#43227,#43228,#43229,#43230,#43231,#43232,#43233,
#43234,#43235,#43236,#43237,#43238,#43239,#43240,#43241,#43242,#43243,#43244,
#43245,#43246,#43247,#43248,#43249,#43250,#43251,#43252,#43253,#43254,#43255,
#43256,#43257,#43258,#43259,#43260,#43261,#43262,#43263,#43264,#43265,#43266,
#43267,#43268,#43269,#43270,#43271,#43272,#43273,#43274,#43275,#43276,#43277,
#43278,#43279,#43280,#43281,#43282,#43283,#43284,#43285,#43286,#43287,#43288,
#43289,#43290,#43291,#43292,#43293,#43294,#43295,#43296,#43297,#43298,#43299,
#43300,#43301,#43302,#43303,#43304,#43305,#43306,#43307,#43308,#43309,#43310,
#43311,#43312,#43313,#43314,#43315,#43316,#43317,#43318,#43319,#43320,#43321),
 .UNSPECIFIED.,.F.,.F.,(4,3,3,3,3,3,3,3,3,3,3,3,3,3,3,3,3,3,3,3,3,3,3,3,
3,3,3,3,3,3,3,3,3,3,3,3,3,3,4),(0.,0.0442982788118636,0.0893818690181126,
0.135122693119257,0.180798269742455,0.192189224643416,0.201490490453158,
0.207330447631488,0.254018913968702,0.259381740752703,0.305561249420596,
0.352304439716772,0.396784766685594,0.407417643265349,0.413596814657803,
0.419491730417116,0.467135890742667,0.515289047534096,0.53022574759206,
0.578093773825496,0.607379019530261,0.623354033228688,0.630969399843706,
0.637303510397527,0.686063011063978,0.735282487221379,0.784567458473146,
0.812375739463615,0.848989885401632,0.855830972691235,0.862937690127921,
0.912534157810533,0.960722845099838,0.982643323209691,0.993796749973554,
1.00410992606059,1.05516230274151,1.10528890696775,1.14369947197754),
 .UNSPECIFIED.);
#953=B_SPLINE_CURVE_WITH_KNOTS('',3,(#43322,#43323,#43324,#43325,#43326,
#43327,#43328,#43329,#43330,#43331,#43332,#43333,#43334,#43335,#43336,#43337,
#43338,#43339,#43340,#43341,#43342,#43343,#43344,#43345,#43346,#43347,#43348,
#43349,#43350,#43351,#43352,#43353,#43354,#43355,#43356,#43357,#43358,#43359,
#43360,#43361,#43362,#43363,#43364),.UNSPECIFIED.,.F.,.F.,(4,3,3,3,3,3,
3,3,3,3,3,3,3,3,4),(-10.1394149102777,-9.80628246515584,-9.31596834189804,
-8.82565421864025,-8.33534009538246,-7.84502597212467,-7.35471184886688,
-6.86439772560908,-6.37408360235129,-5.8837694790935,-5.39345535583571,
-4.90314123257792,-4.41282710932013,-3.92251298606233,-3.85622960309808),
 .UNSPECIFIED.);
#954=B_SPLINE_CURVE_WITH_KNOTS('',3,(#43745,#43746,#43747,#43748,#43749,
#43750,#43751,#43752,#43753,#43754,#43755,#43756,#43757,#43758,#43759,#43760,
#43761,#43762,#43763,#43764,#43765,#43766,#43767,#43768,#43769,#43770,#43771,
#43772,#43773,#43774,#43775,#43776,#43777,#43778,#43779,#43780,#43781,#43782,
#43783,#43784,#43785,#43786,#43787,#43788,#43789,#43790,#43791,#43792,#43793,
#43794,#43795,#43796,#43797,#43798,#43799,#43800,#43801,#43802,#43803,#43804,
#43805,#43806,#43807,#43808,#43809,#43810,#43811,#43812,#43813,#43814,#43815,
#43816,#43817,#43818,#43819,#43820,#43821,#43822,#43823,#43824,#43825,#43826,
#43827,#43828,#43829,#43830,#43831,#43832,#43833,#43834,#43835,#43836,#43837,
#43838,#43839,#43840,#43841,#43842,#43843,#43844,#43845,#43846,#43847,#43848,
#43849,#43850,#43851,#43852,#43853,#43854,#43855,#43856,#43857,#43858,#43859),
 .UNSPECIFIED.,.F.,.F.,(4,3,3,3,3,3,3,3,3,3,3,3,3,3,3,3,3,3,3,3,3,3,3,3,
3,3,3,3,3,3,3,3,3,3,3,3,3,3,4),(0.,0.04429834024652,0.089381979475409,0.135122817034445,
0.18079838316134,0.192189399543316,0.20149081189225,0.207330624426604,0.254019121588896,
0.259381740752706,0.305561208101797,0.352304372648012,0.396784716384027,
0.407417348322894,0.41359569479113,0.419491539259941,0.467135664198151,
0.515288809852319,0.530225747592073,0.578093783520646,0.607379028013523,
0.623354030000456,0.63096936113017,0.637303502944702,0.686063016433146,
0.735282499868879,0.784567472007001,0.812375739463663,0.848989885401685,
0.85583097269828,0.862937690097506,0.912534156610552,0.960722844199872,
0.982643321680792,0.993796738994502,1.00410992500793,1.0551623020005,1.10528890696783,
1.14369947197762),.UNSPECIFIED.);
#955=B_SPLINE_CURVE_WITH_KNOTS('',3,(#43860,#43861,#43862,#43863,#43864,
#43865,#43866,#43867,#43868,#43869,#43870,#43871,#43872,#43873,#43874,#43875,
#43876,#43877,#43878,#43879,#43880,#43881,#43882,#43883,#43884,#43885,#43886,
#43887,#43888,#43889,#43890,#43891,#43892,#43893,#43894,#43895,#43896,#43897,
#43898,#43899,#43900,#43901,#43902),.UNSPECIFIED.,.F.,.F.,(4,3,3,3,3,3,
3,3,3,3,3,3,3,3,4),(7.59274844815668,7.84502597212467,8.33534009538246,
8.82565421864025,9.31596834189804,9.80628246515583,10.2965965884136,10.7869107116714,
11.2772248349292,11.767538958187,12.2578530814448,12.7481672047026,13.2384813279604,
13.7287954512182,13.8759337553363),.UNSPECIFIED.);
#956=B_SPLINE_CURVE_WITH_KNOTS('',3,(#43903,#43904,#43905,#43906,#43907,
#43908,#43909,#43910,#43911,#43912,#43913,#43914,#43915,#43916,#43917,#43918,
#43919,#43920,#43921,#43922,#43923,#43924,#43925,#43926,#43927,#43928,#43929,
#43930,#43931,#43932,#43933,#43934,#43935,#43936,#43937,#43938,#43939,#43940,
#43941,#43942,#43943,#43944,#43945,#43946,#43947,#43948,#43949,#43950,#43951,
#43952,#43953,#43954,#43955,#43956,#43957,#43958,#43959,#43960,#43961,#43962,
#43963,#43964,#43965,#43966,#43967,#43968,#43969,#43970,#43971,#43972,#43973,
#43974,#43975,#43976,#43977,#43978,#43979,#43980,#43981,#43982,#43983,#43984,
#43985,#43986,#43987,#43988,#43989,#43990,#43991,#43992,#43993,#43994,#43995,
#43996,#43997,#43998,#43999,#44000,#44001,#44002,#44003,#44004,#44005,#44006,
#44007,#44008,#44009,#44010,#44011,#44012,#44013,#44014,#44015,#44016,#44017),
 .UNSPECIFIED.,.F.,.F.,(4,3,3,3,3,3,3,3,3,3,3,3,3,3,3,3,3,3,3,3,3,3,3,3,
3,3,3,3,3,3,3,3,3,3,3,3,3,3,4),(0.,0.05057089589372,0.101542722275973,0.152182412916207,
0.202219333720841,0.225638825786133,0.233898233275305,0.24073547777789,
0.290357594353021,0.295897301982008,0.345686254294586,0.395413835081348,
0.44170662055217,0.453063297205788,0.461070756512692,0.467176281050606,
0.515730458090084,0.56391533759721,0.580584976964637,0.629137535716166,
0.657230420874013,0.674238539358194,0.682110620359464,0.688083286117201,
0.735480742780762,0.782731794499091,0.829225256981287,0.85388061697894,
0.886547113898585,0.894686952580864,0.901806441637606,0.948290090133573,
0.990020715684203,1.0102197832758,1.02166123242085,1.02855218820189,1.07381104284631,
1.11521259233609,1.14791015664666),.UNSPECIFIED.);
#1557=SHAPE_REPRESENTATION_RELATIONSHIP('SRR','None',#63996,#1575);
#1575=ADVANCED_BREP_SHAPE_REPRESENTATION('',(#1611),#63881);
#1593=STYLED_ITEM('',(#64095),#1611);
#1611=MANIFOLD_SOLID_BREP('Body1',#15479);
#1644=FACE_BOUND('',#3901,.T.);
#1645=FACE_BOUND('',#3902,.T.);
#1646=FACE_BOUND('',#3903,.T.);
#1647=FACE_BOUND('',#3904,.T.);
#1648=FACE_BOUND('',#3905,.T.);
#1649=FACE_BOUND('',#3910,.T.);
#1650=FACE_BOUND('',#3916,.T.);
#1651=FACE_BOUND('',#3918,.T.);
#1652=FACE_BOUND('',#3920,.T.);
#1653=FACE_BOUND('',#3924,.T.);
#1654=FACE_BOUND('',#3926,.T.);
#1655=FACE_BOUND('',#3931,.T.);
#1656=FACE_BOUND('',#3933,.T.);
#1657=FACE_BOUND('',#3934,.T.);
#1658=FACE_BOUND('',#3935,.T.);
#1659=FACE_BOUND('',#3936,.T.);
#1660=FACE_BOUND('',#3937,.T.);
#1726=CYLINDRICAL_SURFACE('',#15753,5.13675);
#1727=CYLINDRICAL_SURFACE('',#15755,5.13675);
#1728=CYLINDRICAL_SURFACE('',#15757,5.13675);
#1729=CYLINDRICAL_SURFACE('',#15758,5.13675);
#1730=CYLINDRICAL_SURFACE('',#15759,5.13675);
#1731=CYLINDRICAL_SURFACE('',#15760,5.13675);
#1732=CYLINDRICAL_SURFACE('',#15761,5.13675);
#1733=CYLINDRICAL_SURFACE('',#15763,6.11325000000001);
#1734=CYLINDRICAL_SURFACE('',#15765,6.11325000000001);
#1735=CYLINDRICAL_SURFACE('',#15766,6.11325000000001);
#1736=CYLINDRICAL_SURFACE('',#15767,6.11325000000001);
#1737=CYLINDRICAL_SURFACE('',#15768,6.11325000000001);
#1738=CYLINDRICAL_SURFACE('',#15769,6.11325000000001);
#1739=CYLINDRICAL_SURFACE('',#15770,6.11325000000001);
#1740=CYLINDRICAL_SURFACE('',#15772,1.666);
#1741=CYLINDRICAL_SURFACE('',#15776,1.666);
#1742=CYLINDRICAL_SURFACE('',#15777,1.666);
#1743=CYLINDRICAL_SURFACE('',#15778,1.666);
#1744=CYLINDRICAL_SURFACE('',#15779,1.666);
#1745=CYLINDRICAL_SURFACE('',#15780,1.666);
#1746=CYLINDRICAL_SURFACE('',#15781,1.666);
#1747=CYLINDRICAL_SURFACE('',#15782,1.666);
#1748=CYLINDRICAL_SURFACE('',#15783,1.666);
#1749=CYLINDRICAL_SURFACE('',#15784,1.666);
#1750=CYLINDRICAL_SURFACE('',#15785,1.666);
#1751=CYLINDRICAL_SURFACE('',#15786,1.666);
#1752=CYLINDRICAL_SURFACE('',#15787,1.666);
#1753=CYLINDRICAL_SURFACE('',#15788,1.666);
#1754=CYLINDRICAL_SURFACE('',#15789,1.666);
#1755=CYLINDRICAL_SURFACE('',#15790,1.666);
#1756=CYLINDRICAL_SURFACE('',#15791,1.666);
#1757=CYLINDRICAL_SURFACE('',#15792,1.666);
#1758=CYLINDRICAL_SURFACE('',#15794,2.05475);
#1759=CYLINDRICAL_SURFACE('',#15796,2.05475);
#1760=CYLINDRICAL_SURFACE('',#15797,2.05475);
#1761=CYLINDRICAL_SURFACE('',#15798,2.05475);
#1762=CYLINDRICAL_SURFACE('',#15799,2.05475);
#1763=CYLINDRICAL_SURFACE('',#15800,2.05475);
#1764=CYLINDRICAL_SURFACE('',#15801,2.05475);
#1765=CYLINDRICAL_SURFACE('',#15802,2.05475);
#1766=CYLINDRICAL_SURFACE('',#15803,2.05475);
#1767=CYLINDRICAL_SURFACE('',#15804,2.05475);
#1768=CYLINDRICAL_SURFACE('',#15805,2.05475);
#1769=CYLINDRICAL_SURFACE('',#15806,2.05475);
#1770=CYLINDRICAL_SURFACE('',#15807,2.05475);
#1771=CYLINDRICAL_SURFACE('',#15808,2.05475);
#1772=CYLINDRICAL_SURFACE('',#15809,2.05475);
#1773=CYLINDRICAL_SURFACE('',#15810,2.05475);
#1774=CYLINDRICAL_SURFACE('',#15811,2.05475);
#1775=CYLINDRICAL_SURFACE('',#15812,2.05475);
#1776=CYLINDRICAL_SURFACE('',#15813,2.05475);
#1777=CYLINDRICAL_SURFACE('',#15815,1.666);
#1778=CYLINDRICAL_SURFACE('',#15819,1.666);
#1779=CYLINDRICAL_SURFACE('',#15820,1.666);
#1780=CYLINDRICAL_SURFACE('',#15821,1.666);
#1781=CYLINDRICAL_SURFACE('',#15822,1.666);
#1782=CYLINDRICAL_SURFACE('',#15823,1.666);
#1783=CYLINDRICAL_SURFACE('',#15824,1.666);
#1784=CYLINDRICAL_SURFACE('',#15825,1.666);
#1785=CYLINDRICAL_SURFACE('',#15826,1.666);
#1786=CYLINDRICAL_SURFACE('',#15827,1.666);
#1787=CYLINDRICAL_SURFACE('',#15828,1.666);
#1788=CYLINDRICAL_SURFACE('',#15829,1.666);
#1789=CYLINDRICAL_SURFACE('',#15830,1.666);
#1790=CYLINDRICAL_SURFACE('',#15831,1.666);
#1791=CYLINDRICAL_SURFACE('',#15832,1.666);
#1792=CYLINDRICAL_SURFACE('',#15833,1.666);
#1793=CYLINDRICAL_SURFACE('',#15834,1.666);
#1794=CYLINDRICAL_SURFACE('',#15835,1.666);
#1795=CYLINDRICAL_SURFACE('',#15837,2.05475);
#1796=CYLINDRICAL_SURFACE('',#15839,2.05475);
#1797=CYLINDRICAL_SURFACE('',#15840,2.05475);
#1798=CYLINDRICAL_SURFACE('',#15841,2.05475);
#1799=CYLINDRICAL_SURFACE('',#15842,2.05475);
#1800=CYLINDRICAL_SURFACE('',#15843,2.05475);
#1801=CYLINDRICAL_SURFACE('',#15844,2.05475);
#1802=CYLINDRICAL_SURFACE('',#15845,2.05475);
#1803=CYLINDRICAL_SURFACE('',#15846,2.05475);
#1804=CYLINDRICAL_SURFACE('',#15847,2.05475);
#1805=CYLINDRICAL_SURFACE('',#15848,2.05475);
#1806=CYLINDRICAL_SURFACE('',#15849,2.05475);
#1807=CYLINDRICAL_SURFACE('',#15850,2.05475);
#1808=CYLINDRICAL_SURFACE('',#15851,2.05475);
#1809=CYLINDRICAL_SURFACE('',#15852,2.05475);
#1810=CYLINDRICAL_SURFACE('',#15853,2.05475);
#1811=CYLINDRICAL_SURFACE('',#15854,2.05475);
#1812=CYLINDRICAL_SURFACE('',#15855,2.05475);
#1813=CYLINDRICAL_SURFACE('',#15856,2.05475);
#1814=CYLINDRICAL_SURFACE('',#15858,1.666);
#1815=CYLINDRICAL_SURFACE('',#15862,1.666);
#1816=CYLINDRICAL_SURFACE('',#15863,1.666);
#1817=CYLINDRICAL_SURFACE('',#15864,1.666);
#1818=CYLINDRICAL_SURFACE('',#15865,1.666);
#1819=CYLINDRICAL_SURFACE('',#15866,1.666);
#1820=CYLINDRICAL_SURFACE('',#15867,1.666);
#1821=CYLINDRICAL_SURFACE('',#15868,1.666);
#1822=CYLINDRICAL_SURFACE('',#15869,1.666);
#1823=CYLINDRICAL_SURFACE('',#15870,1.666);
#1824=CYLINDRICAL_SURFACE('',#15871,1.666);
#1825=CYLINDRICAL_SURFACE('',#15872,1.666);
#1826=CYLINDRICAL_SURFACE('',#15873,1.666);
#1827=CYLINDRICAL_SURFACE('',#15874,1.666);
#1828=CYLINDRICAL_SURFACE('',#15875,1.666);
#1829=CYLINDRICAL_SURFACE('',#15876,1.666);
#1830=CYLINDRICAL_SURFACE('',#15877,1.666);
#1831=CYLINDRICAL_SURFACE('',#15878,1.666);
#1832=CYLINDRICAL_SURFACE('',#15880,2.05475);
#1833=CYLINDRICAL_SURFACE('',#15882,2.05475);
#1834=CYLINDRICAL_SURFACE('',#15883,2.05475);
#1835=CYLINDRICAL_SURFACE('',#15884,2.05475);
#1836=CYLINDRICAL_SURFACE('',#15885,2.05475);
#1837=CYLINDRICAL_SURFACE('',#15886,2.05475);
#1838=CYLINDRICAL_SURFACE('',#15887,2.05475);
#1839=CYLINDRICAL_SURFACE('',#15888,2.05475);
#1840=CYLINDRICAL_SURFACE('',#15889,2.05475);
#1841=CYLINDRICAL_SURFACE('',#15890,2.05475);
#1842=CYLINDRICAL_SURFACE('',#15891,2.05475);
#1843=CYLINDRICAL_SURFACE('',#15892,2.05475);
#1844=CYLINDRICAL_SURFACE('',#15893,2.05475);
#1845=CYLINDRICAL_SURFACE('',#15894,2.05475);
#1846=CYLINDRICAL_SURFACE('',#15895,2.05475);
#1847=CYLINDRICAL_SURFACE('',#15896,2.05475);
#1848=CYLINDRICAL_SURFACE('',#15897,2.05475);
#1849=CYLINDRICAL_SURFACE('',#15898,2.05475);
#1850=CYLINDRICAL_SURFACE('',#15899,2.05475);
#1851=CYLINDRICAL_SURFACE('',#15901,1.666);
#1852=CYLINDRICAL_SURFACE('',#15905,1.666);
#1853=CYLINDRICAL_SURFACE('',#15906,1.666);
#1854=CYLINDRICAL_SURFACE('',#15907,1.666);
#1855=CYLINDRICAL_SURFACE('',#15908,1.666);
#1856=CYLINDRICAL_SURFACE('',#15909,1.666);
#1857=CYLINDRICAL_SURFACE('',#15910,1.666);
#1858=CYLINDRICAL_SURFACE('',#15911,1.666);
#1859=CYLINDRICAL_SURFACE('',#15912,1.666);
#1860=CYLINDRICAL_SURFACE('',#15913,1.666);
#1861=CYLINDRICAL_SURFACE('',#15914,1.666);
#1862=CYLINDRICAL_SURFACE('',#15915,1.666);
#1863=CYLINDRICAL_SURFACE('',#15916,1.666);
#1864=CYLINDRICAL_SURFACE('',#15917,1.666);
#1865=CYLINDRICAL_SURFACE('',#15918,1.666);
#1866=CYLINDRICAL_SURFACE('',#15919,1.666);
#1867=CYLINDRICAL_SURFACE('',#15920,1.666);
#1868=CYLINDRICAL_SURFACE('',#15921,1.666);
#1869=CYLINDRICAL_SURFACE('',#15923,2.05475);
#1870=CYLINDRICAL_SURFACE('',#15925,2.05475);
#1871=CYLINDRICAL_SURFACE('',#15926,2.05475);
#1872=CYLINDRICAL_SURFACE('',#15927,2.05475);
#1873=CYLINDRICAL_SURFACE('',#15928,2.05475);
#1874=CYLINDRICAL_SURFACE('',#15929,2.05475);
#1875=CYLINDRICAL_SURFACE('',#15930,2.05475);
#1876=CYLINDRICAL_SURFACE('',#15931,2.05475);
#1877=CYLINDRICAL_SURFACE('',#15932,2.05475);
#1878=CYLINDRICAL_SURFACE('',#15933,2.05475);
#1879=CYLINDRICAL_SURFACE('',#15934,2.05475);
#1880=CYLINDRICAL_SURFACE('',#15935,2.05475);
#1881=CYLINDRICAL_SURFACE('',#15936,2.05475);
#1882=CYLINDRICAL_SURFACE('',#15937,2.05475);
#1883=CYLINDRICAL_SURFACE('',#15938,2.05475);
#1884=CYLINDRICAL_SURFACE('',#15939,2.05475);
#1885=CYLINDRICAL_SURFACE('',#15940,2.05475);
#1886=CYLINDRICAL_SURFACE('',#15941,2.05475);
#1887=CYLINDRICAL_SURFACE('',#15942,2.05475);
#1888=CYLINDRICAL_SURFACE('',#15944,1.666);
#1889=CYLINDRICAL_SURFACE('',#15948,1.666);
#1890=CYLINDRICAL_SURFACE('',#15949,1.666);
#1891=CYLINDRICAL_SURFACE('',#15950,1.666);
#1892=CYLINDRICAL_SURFACE('',#15951,1.666);
#1893=CYLINDRICAL_SURFACE('',#15952,1.666);
#1894=CYLINDRICAL_SURFACE('',#15953,1.666);
#1895=CYLINDRICAL_SURFACE('',#15954,1.666);
#1896=CYLINDRICAL_SURFACE('',#15955,1.666);
#1897=CYLINDRICAL_SURFACE('',#15956,1.666);
#1898=CYLINDRICAL_SURFACE('',#15957,1.666);
#1899=CYLINDRICAL_SURFACE('',#15958,1.666);
#1900=CYLINDRICAL_SURFACE('',#15959,1.666);
#1901=CYLINDRICAL_SURFACE('',#15960,1.666);
#1902=CYLINDRICAL_SURFACE('',#15961,1.666);
#1903=CYLINDRICAL_SURFACE('',#15962,1.666);
#1904=CYLINDRICAL_SURFACE('',#15963,1.666);
#1905=CYLINDRICAL_SURFACE('',#15964,1.666);
#1906=CYLINDRICAL_SURFACE('',#15966,2.05475);
#1907=CYLINDRICAL_SURFACE('',#15968,2.05475);
#1908=CYLINDRICAL_SURFACE('',#15969,2.05475);
#1909=CYLINDRICAL_SURFACE('',#15970,2.05475);
#1910=CYLINDRICAL_SURFACE('',#15971,2.05475);
#1911=CYLINDRICAL_SURFACE('',#15972,2.05475);
#1912=CYLINDRICAL_SURFACE('',#15973,2.05475);
#1913=CYLINDRICAL_SURFACE('',#15974,2.05475);
#1914=CYLINDRICAL_SURFACE('',#15975,2.05475);
#1915=CYLINDRICAL_SURFACE('',#15976,2.05475);
#1916=CYLINDRICAL_SURFACE('',#15977,2.05475);
#1917=CYLINDRICAL_SURFACE('',#15978,2.05475);
#1918=CYLINDRICAL_SURFACE('',#15979,2.05475);
#1919=CYLINDRICAL_SURFACE('',#15980,2.05475);
#1920=CYLINDRICAL_SURFACE('',#15981,2.05475);
#1921=CYLINDRICAL_SURFACE('',#15982,2.05475);
#1922=CYLINDRICAL_SURFACE('',#15983,2.05475);
#1923=CYLINDRICAL_SURFACE('',#15984,2.05475);
#1924=CYLINDRICAL_SURFACE('',#15985,2.05475);
#1925=CYLINDRICAL_SURFACE('',#15987,1.666);
#1926=CYLINDRICAL_SURFACE('',#15991,1.666);
#1927=CYLINDRICAL_SURFACE('',#15992,1.666);
#1928=CYLINDRICAL_SURFACE('',#15993,1.666);
#1929=CYLINDRICAL_SURFACE('',#15994,1.666);
#1930=CYLINDRICAL_SURFACE('',#15995,1.666);
#1931=CYLINDRICAL_SURFACE('',#15996,1.666);
#1932=CYLINDRICAL_SURFACE('',#15997,1.666);
#1933=CYLINDRICAL_SURFACE('',#15998,1.666);
#1934=CYLINDRICAL_SURFACE('',#15999,1.666);
#1935=CYLINDRICAL_SURFACE('',#16000,1.666);
#1936=CYLINDRICAL_SURFACE('',#16001,1.666);
#1937=CYLINDRICAL_SURFACE('',#16002,1.666);
#1938=CYLINDRICAL_SURFACE('',#16003,1.666);
#1939=CYLINDRICAL_SURFACE('',#16004,1.666);
#1940=CYLINDRICAL_SURFACE('',#16005,1.666);
#1941=CYLINDRICAL_SURFACE('',#16006,1.666);
#1942=CYLINDRICAL_SURFACE('',#16007,1.666);
#1943=CYLINDRICAL_SURFACE('',#16009,2.05475000000001);
#1944=CYLINDRICAL_SURFACE('',#16011,2.05475000000001);
#1945=CYLINDRICAL_SURFACE('',#16012,2.05475000000001);
#1946=CYLINDRICAL_SURFACE('',#16013,2.05475000000001);
#1947=CYLINDRICAL_SURFACE('',#16014,2.05475000000001);
#1948=CYLINDRICAL_SURFACE('',#16015,2.05475000000001);
#1949=CYLINDRICAL_SURFACE('',#16016,2.05475000000001);
#1950=CYLINDRICAL_SURFACE('',#16017,2.05475000000001);
#1951=CYLINDRICAL_SURFACE('',#16018,2.05475000000001);
#1952=CYLINDRICAL_SURFACE('',#16019,2.05475000000001);
#1953=CYLINDRICAL_SURFACE('',#16020,2.05475000000001);
#1954=CYLINDRICAL_SURFACE('',#16021,2.05475000000001);
#1955=CYLINDRICAL_SURFACE('',#16022,2.05475000000001);
#1956=CYLINDRICAL_SURFACE('',#16023,2.05475000000001);
#1957=CYLINDRICAL_SURFACE('',#16024,2.05475000000001);
#1958=CYLINDRICAL_SURFACE('',#16025,2.05475000000001);
#1959=CYLINDRICAL_SURFACE('',#16026,2.05475000000001);
#1960=CYLINDRICAL_SURFACE('',#16027,2.05475000000001);
#1961=CYLINDRICAL_SURFACE('',#16028,2.05475000000001);
#1962=CYLINDRICAL_SURFACE('',#16030,1.666);
#1963=CYLINDRICAL_SURFACE('',#16034,1.666);
#1964=CYLINDRICAL_SURFACE('',#16035,1.666);
#1965=CYLINDRICAL_SURFACE('',#16036,1.666);
#1966=CYLINDRICAL_SURFACE('',#16037,1.666);
#1967=CYLINDRICAL_SURFACE('',#16038,1.666);
#1968=CYLINDRICAL_SURFACE('',#16039,1.666);
#1969=CYLINDRICAL_SURFACE('',#16040,1.666);
#1970=CYLINDRICAL_SURFACE('',#16041,1.666);
#1971=CYLINDRICAL_SURFACE('',#16042,1.666);
#1972=CYLINDRICAL_SURFACE('',#16043,1.666);
#1973=CYLINDRICAL_SURFACE('',#16044,1.666);
#1974=CYLINDRICAL_SURFACE('',#16045,1.666);
#1975=CYLINDRICAL_SURFACE('',#16046,1.666);
#1976=CYLINDRICAL_SURFACE('',#16047,1.666);
#1977=CYLINDRICAL_SURFACE('',#16048,1.666);
#1978=CYLINDRICAL_SURFACE('',#16049,1.666);
#1979=CYLINDRICAL_SURFACE('',#16050,1.666);
#1980=CYLINDRICAL_SURFACE('',#16052,2.05475);
#1981=CYLINDRICAL_SURFACE('',#16054,2.05475);
#1982=CYLINDRICAL_SURFACE('',#16055,2.05475);
#1983=CYLINDRICAL_SURFACE('',#16056,2.05475);
#1984=CYLINDRICAL_SURFACE('',#16057,2.05475);
#1985=CYLINDRICAL_SURFACE('',#16058,2.05475);
#1986=CYLINDRICAL_SURFACE('',#16059,2.05475);
#1987=CYLINDRICAL_SURFACE('',#16060,2.05475);
#1988=CYLINDRICAL_SURFACE('',#16061,2.05475);
#1989=CYLINDRICAL_SURFACE('',#16062,2.05475);
#1990=CYLINDRICAL_SURFACE('',#16063,2.05475);
#1991=CYLINDRICAL_SURFACE('',#16064,2.05475);
#1992=CYLINDRICAL_SURFACE('',#16065,2.05475);
#1993=CYLINDRICAL_SURFACE('',#16066,2.05475);
#1994=CYLINDRICAL_SURFACE('',#16067,2.05475);
#1995=CYLINDRICAL_SURFACE('',#16068,2.05475);
#1996=CYLINDRICAL_SURFACE('',#16069,2.05475);
#1997=CYLINDRICAL_SURFACE('',#16070,2.05475);
#1998=CYLINDRICAL_SURFACE('',#16071,2.05475);
#1999=CYLINDRICAL_SURFACE('',#16073,1.666);
#2000=CYLINDRICAL_SURFACE('',#16077,1.666);
#2001=CYLINDRICAL_SURFACE('',#16078,1.666);
#2002=CYLINDRICAL_SURFACE('',#16079,1.666);
#2003=CYLINDRICAL_SURFACE('',#16080,1.666);
#2004=CYLINDRICAL_SURFACE('',#16081,1.666);
#2005=CYLINDRICAL_SURFACE('',#16082,1.666);
#2006=CYLINDRICAL_SURFACE('',#16083,1.666);
#2007=CYLINDRICAL_SURFACE('',#16084,1.666);
#2008=CYLINDRICAL_SURFACE('',#16085,1.666);
#2009=CYLINDRICAL_SURFACE('',#16086,1.666);
#2010=CYLINDRICAL_SURFACE('',#16087,1.666);
#2011=CYLINDRICAL_SURFACE('',#16088,1.666);
#2012=CYLINDRICAL_SURFACE('',#16089,1.666);
#2013=CYLINDRICAL_SURFACE('',#16090,1.666);
#2014=CYLINDRICAL_SURFACE('',#16091,1.666);
#2015=CYLINDRICAL_SURFACE('',#16092,1.666);
#2016=CYLINDRICAL_SURFACE('',#16093,1.666);
#2017=CYLINDRICAL_SURFACE('',#16095,2.05475000000001);
#2018=CYLINDRICAL_SURFACE('',#16097,2.05475000000001);
#2019=CYLINDRICAL_SURFACE('',#16098,2.05475000000001);
#2020=CYLINDRICAL_SURFACE('',#16099,2.05475000000001);
#2021=CYLINDRICAL_SURFACE('',#16100,2.05475000000001);
#2022=CYLINDRICAL_SURFACE('',#16101,2.05475000000001);
#2023=CYLINDRICAL_SURFACE('',#16102,2.05475000000001);
#2024=CYLINDRICAL_SURFACE('',#16103,2.05475000000001);
#2025=CYLINDRICAL_SURFACE('',#16104,2.05475000000001);
#2026=CYLINDRICAL_SURFACE('',#16105,2.05475000000001);
#2027=CYLINDRICAL_SURFACE('',#16106,2.05475000000001);
#2028=CYLINDRICAL_SURFACE('',#16107,2.05475000000001);
#2029=CYLINDRICAL_SURFACE('',#16108,2.05475000000001);
#2030=CYLINDRICAL_SURFACE('',#16109,2.05475000000001);
#2031=CYLINDRICAL_SURFACE('',#16110,2.05475000000001);
#2032=CYLINDRICAL_SURFACE('',#16111,2.05475000000001);
#2033=CYLINDRICAL_SURFACE('',#16112,2.05475000000001);
#2034=CYLINDRICAL_SURFACE('',#16113,2.05475000000001);
#2035=CYLINDRICAL_SURFACE('',#16114,2.05475000000001);
#2036=CYLINDRICAL_SURFACE('',#16117,2.05475000000001);
#2037=CYLINDRICAL_SURFACE('',#16118,1.666);
#2038=CYLINDRICAL_SURFACE('',#16120,2.05475);
#2039=CYLINDRICAL_SURFACE('',#16121,1.666);
#2040=CYLINDRICAL_SURFACE('',#16123,2.05475000000001);
#2041=CYLINDRICAL_SURFACE('',#16124,1.666);
#2042=CYLINDRICAL_SURFACE('',#16126,2.05475);
#2043=CYLINDRICAL_SURFACE('',#16127,1.666);
#2044=CYLINDRICAL_SURFACE('',#16133,2.05475);
#2045=CYLINDRICAL_SURFACE('',#16134,1.666);
#2046=CYLINDRICAL_SURFACE('',#16136,2.05475);
#2047=CYLINDRICAL_SURFACE('',#16137,1.666);
#2048=CYLINDRICAL_SURFACE('',#16139,2.05475);
#2049=CYLINDRICAL_SURFACE('',#16140,1.666);
#2050=CYLINDRICAL_SURFACE('',#16142,2.05475);
#2051=CYLINDRICAL_SURFACE('',#16143,1.666);
#2052=CYLINDRICAL_SURFACE('',#16154,6.11325000000001);
#2053=CYLINDRICAL_SURFACE('',#16157,5.13675);
#2054=CYLINDRICAL_SURFACE('',#16169,35.);
#2055=CYLINDRICAL_SURFACE('',#16170,40.);
#2056=CYLINDRICAL_SURFACE('',#16177,35.);
#2057=CYLINDRICAL_SURFACE('',#16178,40.);
#2058=CYLINDRICAL_SURFACE('',#16179,40.);
#2059=CYLINDRICAL_SURFACE('',#16181,50.);
#2410=CIRCLE('',#15754,5.13675);
#2411=CIRCLE('',#15756,5.13675);
#2412=CIRCLE('',#15762,5.13675);
#2413=CIRCLE('',#15764,6.11325000000001);
#2414=CIRCLE('',#15771,6.11325000000001);
#2415=CIRCLE('',#15773,1.666);
#2416=CIRCLE('',#15774,1.666);
#2417=CIRCLE('',#15775,1.666);
#2418=CIRCLE('',#15793,1.666);
#2419=CIRCLE('',#15795,2.05475);
#2420=CIRCLE('',#15814,2.05475);
#2421=CIRCLE('',#15816,1.666);
#2422=CIRCLE('',#15817,1.666);
#2423=CIRCLE('',#15818,1.666);
#2424=CIRCLE('',#15836,1.666);
#2425=CIRCLE('',#15838,2.05475);
#2426=CIRCLE('',#15857,2.05475);
#2427=CIRCLE('',#15859,1.666);
#2428=CIRCLE('',#15860,1.666);
#2429=CIRCLE('',#15861,1.666);
#2430=CIRCLE('',#15879,1.666);
#2431=CIRCLE('',#15881,2.05475);
#2432=CIRCLE('',#15900,2.05475);
#2433=CIRCLE('',#15902,1.666);
#2434=CIRCLE('',#15903,1.666);
#2435=CIRCLE('',#15904,1.666);
#2436=CIRCLE('',#15922,1.666);
#2437=CIRCLE('',#15924,2.05475);
#2438=CIRCLE('',#15943,2.05475);
#2439=CIRCLE('',#15945,1.666);
#2440=CIRCLE('',#15946,1.666);
#2441=CIRCLE('',#15947,1.666);
#2442=CIRCLE('',#15965,1.666);
#2443=CIRCLE('',#15967,2.05475);
#2444=CIRCLE('',#15986,2.05475);
#2445=CIRCLE('',#15988,1.666);
#2446=CIRCLE('',#15989,1.666);
#2447=CIRCLE('',#15990,1.666);
#2448=CIRCLE('',#16008,1.666);
#2449=CIRCLE('',#16010,2.05475000000001);
#2450=CIRCLE('',#16029,2.05475000000001);
#2451=CIRCLE('',#16031,1.666);
#2452=CIRCLE('',#16032,1.666);
#2453=CIRCLE('',#16033,1.666);
#2454=CIRCLE('',#16051,1.666);
#2455=CIRCLE('',#16053,2.05475);
#2456=CIRCLE('',#16072,2.05475);
#2457=CIRCLE('',#16074,1.666);
#2458=CIRCLE('',#16075,1.666);
#2459=CIRCLE('',#16076,1.666);
#2460=CIRCLE('',#16094,1.666);
#2461=CIRCLE('',#16096,2.05475000000001);
#2462=CIRCLE('',#16115,2.05475000000001);
#2463=CIRCLE('',#16152,50.);
#2464=CIRCLE('',#16153,40.);
#2465=CIRCLE('',#16156,50.);
#2466=CIRCLE('',#16162,50.);
#2467=CIRCLE('',#16164,40.);
#2468=CIRCLE('',#16165,35.);
#2469=CIRCLE('',#16167,40.);
#2470=CIRCLE('',#16168,35.);
#2471=CIRCLE('',#16171,40.);
#2472=CIRCLE('',#16173,35.);
#2473=CIRCLE('',#16175,40.);
#2474=CIRCLE('',#16176,35.);
#2475=CIRCLE('',#16180,40.);
#2476=CIRCLE('',#16182,50.);
#2685=FACE_OUTER_BOUND('',#3539,.T.);
#2686=FACE_OUTER_BOUND('',#3540,.T.);
#2687=FACE_OUTER_BOUND('',#3541,.T.);
#2688=FACE_OUTER_BOUND('',#3542,.T.);
#2689=FACE_OUTER_BOUND('',#3543,.T.);
#2690=FACE_OUTER_BOUND('',#3544,.T.);
#2691=FACE_OUTER_BOUND('',#3545,.T.);
#2692=FACE_OUTER_BOUND('',#3546,.T.);
#2693=FACE_OUTER_BOUND('',#3547,.T.);
#2694=FACE_OUTER_BOUND('',#3548,.T.);
#2695=FACE_OUTER_BOUND('',#3549,.T.);
#2696=FACE_OUTER_BOUND('',#3550,.T.);
#2697=FACE_OUTER_BOUND('',#3551,.T.);
#2698=FACE_OUTER_BOUND('',#3552,.T.);
#2699=FACE_OUTER_BOUND('',#3553,.T.);
#2700=FACE_OUTER_BOUND('',#3554,.T.);
#2701=FACE_OUTER_BOUND('',#3555,.T.);
#2702=FACE_OUTER_BOUND('',#3556,.T.);
#2703=FACE_OUTER_BOUND('',#3557,.T.);
#2704=FACE_OUTER_BOUND('',#3558,.T.);
#2705=FACE_OUTER_BOUND('',#3559,.T.);
#2706=FACE_OUTER_BOUND('',#3560,.T.);
#2707=FACE_OUTER_BOUND('',#3561,.T.);
#2708=FACE_OUTER_BOUND('',#3562,.T.);
#2709=FACE_OUTER_BOUND('',#3563,.T.);
#2710=FACE_OUTER_BOUND('',#3564,.T.);
#2711=FACE_OUTER_BOUND('',#3565,.T.);
#2712=FACE_OUTER_BOUND('',#3566,.T.);
#2713=FACE_OUTER_BOUND('',#3567,.T.);
#2714=FACE_OUTER_BOUND('',#3568,.T.);
#2715=FACE_OUTER_BOUND('',#3569,.T.);
#2716=FACE_OUTER_BOUND('',#3570,.T.);
#2717=FACE_OUTER_BOUND('',#3571,.T.);
#2718=FACE_OUTER_BOUND('',#3572,.T.);
#2719=FACE_OUTER_BOUND('',#3573,.T.);
#2720=FACE_OUTER_BOUND('',#3574,.T.);
#2721=FACE_OUTER_BOUND('',#3575,.T.);
#2722=FACE_OUTER_BOUND('',#3576,.T.);
#2723=FACE_OUTER_BOUND('',#3577,.T.);
#2724=FACE_OUTER_BOUND('',#3578,.T.);
#2725=FACE_OUTER_BOUND('',#3579,.T.);
#2726=FACE_OUTER_BOUND('',#3580,.T.);
#2727=FACE_OUTER_BOUND('',#3581,.T.);
#2728=FACE_OUTER_BOUND('',#3582,.T.);
#2729=FACE_OUTER_BOUND('',#3583,.T.);
#2730=FACE_OUTER_BOUND('',#3584,.T.);
#2731=FACE_OUTER_BOUND('',#3585,.T.);
#2732=FACE_OUTER_BOUND('',#3586,.T.);
#2733=FACE_OUTER_BOUND('',#3587,.T.);
#2734=FACE_OUTER_BOUND('',#3588,.T.);
#2735=FACE_OUTER_BOUND('',#3589,.T.);
#2736=FACE_OUTER_BOUND('',#3590,.T.);
#2737=FACE_OUTER_BOUND('',#3591,.T.);
#2738=FACE_OUTER_BOUND('',#3592,.T.);
#2739=FACE_OUTER_BOUND('',#3593,.T.);
#2740=FACE_OUTER_BOUND('',#3594,.T.);
#2741=FACE_OUTER_BOUND('',#3595,.T.);
#2742=FACE_OUTER_BOUND('',#3596,.T.);
#2743=FACE_OUTER_BOUND('',#3597,.T.);
#2744=FACE_OUTER_BOUND('',#3598,.T.);
#2745=FACE_OUTER_BOUND('',#3599,.T.);
#2746=FACE_OUTER_BOUND('',#3600,.T.);
#2747=FACE_OUTER_BOUND('',#3601,.T.);
#2748=FACE_OUTER_BOUND('',#3602,.T.);
#2749=FACE_OUTER_BOUND('',#3603,.T.);
#2750=FACE_OUTER_BOUND('',#3604,.T.);
#2751=FACE_OUTER_BOUND('',#3605,.T.);
#2752=FACE_OUTER_BOUND('',#3606,.T.);
#2753=FACE_OUTER_BOUND('',#3607,.T.);
#2754=FACE_OUTER_BOUND('',#3608,.T.);
#2755=FACE_OUTER_BOUND('',#3609,.T.);
#2756=FACE_OUTER_BOUND('',#3610,.T.);
#2757=FACE_OUTER_BOUND('',#3611,.T.);
#2758=FACE_OUTER_BOUND('',#3612,.T.);
#2759=FACE_OUTER_BOUND('',#3613,.T.);
#2760=FACE_OUTER_BOUND('',#3614,.T.);
#2761=FACE_OUTER_BOUND('',#3615,.T.);
#2762=FACE_OUTER_BOUND('',#3616,.T.);
#2763=FACE_OUTER_BOUND('',#3617,.T.);
#2764=FACE_OUTER_BOUND('',#3618,.T.);
#2765=FACE_OUTER_BOUND('',#3619,.T.);
#2766=FACE_OUTER_BOUND('',#3620,.T.);
#2767=FACE_OUTER_BOUND('',#3621,.T.);
#2768=FACE_OUTER_BOUND('',#3622,.T.);
#2769=FACE_OUTER_BOUND('',#3623,.T.);
#2770=FACE_OUTER_BOUND('',#3624,.T.);
#2771=FACE_OUTER_BOUND('',#3625,.T.);
#2772=FACE_OUTER_BOUND('',#3626,.T.);
#2773=FACE_OUTER_BOUND('',#3627,.T.);
#2774=FACE_OUTER_BOUND('',#3628,.T.);
#2775=FACE_OUTER_BOUND('',#3629,.T.);
#2776=FACE_OUTER_BOUND('',#3630,.T.);
#2777=FACE_OUTER_BOUND('',#3631,.T.);
#2778=FACE_OUTER_BOUND('',#3632,.T.);
#2779=FACE_OUTER_BOUND('',#3633,.T.);
#2780=FACE_OUTER_BOUND('',#3634,.T.);
#2781=FACE_OUTER_BOUND('',#3635,.T.);
#2782=FACE_OUTER_BOUND('',#3636,.T.);
#2783=FACE_OUTER_BOUND('',#3637,.T.);
#2784=FACE_OUTER_BOUND('',#3638,.T.);
#2785=FACE_OUTER_BOUND('',#3639,.T.);
#2786=FACE_OUTER_BOUND('',#3640,.T.);
#2787=FACE_OUTER_BOUND('',#3641,.T.);
#2788=FACE_OUTER_BOUND('',#3642,.T.);
#2789=FACE_OUTER_BOUND('',#3643,.T.);
#2790=FACE_OUTER_BOUND('',#3644,.T.);
#2791=FACE_OUTER_BOUND('',#3645,.T.);
#2792=FACE_OUTER_BOUND('',#3646,.T.);
#2793=FACE_OUTER_BOUND('',#3647,.T.);
#2794=FACE_OUTER_BOUND('',#3648,.T.);
#2795=FACE_OUTER_BOUND('',#3649,.T.);
#2796=FACE_OUTER_BOUND('',#3650,.T.);
#2797=FACE_OUTER_BOUND('',#3651,.T.);
#2798=FACE_OUTER_BOUND('',#3652,.T.);
#2799=FACE_OUTER_BOUND('',#3653,.T.);
#2800=FACE_OUTER_BOUND('',#3654,.T.);
#2801=FACE_OUTER_BOUND('',#3655,.T.);
#2802=FACE_OUTER_BOUND('',#3656,.T.);
#2803=FACE_OUTER_BOUND('',#3657,.T.);
#2804=FACE_OUTER_BOUND('',#3658,.T.);
#2805=FACE_OUTER_BOUND('',#3659,.T.);
#2806=FACE_OUTER_BOUND('',#3660,.T.);
#2807=FACE_OUTER_BOUND('',#3661,.T.);
#2808=FACE_OUTER_BOUND('',#3662,.T.);
#2809=FACE_OUTER_BOUND('',#3663,.T.);
#2810=FACE_OUTER_BOUND('',#3664,.T.);
#2811=FACE_OUTER_BOUND('',#3665,.T.);
#2812=FACE_OUTER_BOUND('',#3666,.T.);
#2813=FACE_OUTER_BOUND('',#3667,.T.);
#2814=FACE_OUTER_BOUND('',#3668,.T.);
#2815=FACE_OUTER_BOUND('',#3669,.T.);
#2816=FACE_OUTER_BOUND('',#3670,.T.);
#2817=FACE_OUTER_BOUND('',#3671,.T.);
#2818=FACE_OUTER_BOUND('',#3672,.T.);
#2819=FACE_OUTER_BOUND('',#3673,.T.);
#2820=FACE_OUTER_BOUND('',#3674,.T.);
#2821=FACE_OUTER_BOUND('',#3675,.T.);
#2822=FACE_OUTER_BOUND('',#3676,.T.);
#2823=FACE_OUTER_BOUND('',#3677,.T.);
#2824=FACE_OUTER_BOUND('',#3678,.T.);
#2825=FACE_OUTER_BOUND('',#3679,.T.);
#2826=FACE_OUTER_BOUND('',#3680,.T.);
#2827=FACE_OUTER_BOUND('',#3681,.T.);
#2828=FACE_OUTER_BOUND('',#3682,.T.);
#2829=FACE_OUTER_BOUND('',#3683,.T.);
#2830=FACE_OUTER_BOUND('',#3684,.T.);
#2831=FACE_OUTER_BOUND('',#3685,.T.);
#2832=FACE_OUTER_BOUND('',#3686,.T.);
#2833=FACE_OUTER_BOUND('',#3687,.T.);
#2834=FACE_OUTER_BOUND('',#3688,.T.);
#2835=FACE_OUTER_BOUND('',#3689,.T.);
#2836=FACE_OUTER_BOUND('',#3690,.T.);
#2837=FACE_OUTER_BOUND('',#3691,.T.);
#2838=FACE_OUTER_BOUND('',#3692,.T.);
#2839=FACE_OUTER_BOUND('',#3693,.T.);
#2840=FACE_OUTER_BOUND('',#3694,.T.);
#2841=FACE_OUTER_BOUND('',#3695,.T.);
#2842=FACE_OUTER_BOUND('',#3696,.T.);
#2843=FACE_OUTER_BOUND('',#3697,.T.);
#2844=FACE_OUTER_BOUND('',#3698,.T.);
#2845=FACE_OUTER_BOUND('',#3699,.T.);
#2846=FACE_OUTER_BOUND('',#3700,.T.);
#2847=FACE_OUTER_BOUND('',#3701,.T.);
#2848=FACE_OUTER_BOUND('',#3702,.T.);
#2849=FACE_OUTER_BOUND('',#3703,.T.);
#2850=FACE_OUTER_BOUND('',#3704,.T.);
#2851=FACE_OUTER_BOUND('',#3705,.T.);
#2852=FACE_OUTER_BOUND('',#3706,.T.);
#2853=FACE_OUTER_BOUND('',#3707,.T.);
#2854=FACE_OUTER_BOUND('',#3708,.T.);
#2855=FACE_OUTER_BOUND('',#3709,.T.);
#2856=FACE_OUTER_BOUND('',#3710,.T.);
#2857=FACE_OUTER_BOUND('',#3711,.T.);
#2858=FACE_OUTER_BOUND('',#3712,.T.);
#2859=FACE_OUTER_BOUND('',#3713,.T.);
#2860=FACE_OUTER_BOUND('',#3714,.T.);
#2861=FACE_OUTER_BOUND('',#3715,.T.);
#2862=FACE_OUTER_BOUND('',#3716,.T.);
#2863=FACE_OUTER_BOUND('',#3717,.T.);
#2864=FACE_OUTER_BOUND('',#3718,.T.);
#2865=FACE_OUTER_BOUND('',#3719,.T.);
#2866=FACE_OUTER_BOUND('',#3720,.T.);
#2867=FACE_OUTER_BOUND('',#3721,.T.);
#2868=FACE_OUTER_BOUND('',#3722,.T.);
#2869=FACE_OUTER_BOUND('',#3723,.T.);
#2870=FACE_OUTER_BOUND('',#3724,.T.);
#2871=FACE_OUTER_BOUND('',#3725,.T.);
#2872=FACE_OUTER_BOUND('',#3726,.T.);
#2873=FACE_OUTER_BOUND('',#3727,.T.);
#2874=FACE_OUTER_BOUND('',#3728,.T.);
#2875=FACE_OUTER_BOUND('',#3729,.T.);
#2876=FACE_OUTER_BOUND('',#3730,.T.);
#2877=FACE_OUTER_BOUND('',#3731,.T.);
#2878=FACE_OUTER_BOUND('',#3732,.T.);
#2879=FACE_OUTER_BOUND('',#3733,.T.);
#2880=FACE_OUTER_BOUND('',#3734,.T.);
#2881=FACE_OUTER_BOUND('',#3735,.T.);
#2882=FACE_OUTER_BOUND('',#3736,.T.);
#2883=FACE_OUTER_BOUND('',#3737,.T.);
#2884=FACE_OUTER_BOUND('',#3738,.T.);
#2885=FACE_OUTER_BOUND('',#3739,.T.);
#2886=FACE_OUTER_BOUND('',#3740,.T.);
#2887=FACE_OUTER_BOUND('',#3741,.T.);
#2888=FACE_OUTER_BOUND('',#3742,.T.);
#2889=FACE_OUTER_BOUND('',#3743,.T.);
#2890=FACE_OUTER_BOUND('',#3744,.T.);
#2891=FACE_OUTER_BOUND('',#3745,.T.);
#2892=FACE_OUTER_BOUND('',#3746,.T.);
#2893=FACE_OUTER_BOUND('',#3747,.T.);
#2894=FACE_OUTER_BOUND('',#3748,.T.);
#2895=FACE_OUTER_BOUND('',#3749,.T.);
#2896=FACE_OUTER_BOUND('',#3750,.T.);
#2897=FACE_OUTER_BOUND('',#3751,.T.);
#2898=FACE_OUTER_BOUND('',#3752,.T.);
#2899=FACE_OUTER_BOUND('',#3753,.T.);
#2900=FACE_OUTER_BOUND('',#3754,.T.);
#2901=FACE_OUTER_BOUND('',#3755,.T.);
#2902=FACE_OUTER_BOUND('',#3756,.T.);
#2903=FACE_OUTER_BOUND('',#3757,.T.);
#2904=FACE_OUTER_BOUND('',#3758,.T.);
#2905=FACE_OUTER_BOUND('',#3759,.T.);
#2906=FACE_OUTER_BOUND('',#3760,.T.);
#2907=FACE_OUTER_BOUND('',#3761,.T.);
#2908=FACE_OUTER_BOUND('',#3762,.T.);
#2909=FACE_OUTER_BOUND('',#3763,.T.);
#2910=FACE_OUTER_BOUND('',#3764,.T.);
#2911=FACE_OUTER_BOUND('',#3765,.T.);
#2912=FACE_OUTER_BOUND('',#3766,.T.);
#2913=FACE_OUTER_BOUND('',#3767,.T.);
#2914=FACE_OUTER_BOUND('',#3768,.T.);
#2915=FACE_OUTER_BOUND('',#3769,.T.);
#2916=FACE_OUTER_BOUND('',#3770,.T.);
#2917=FACE_OUTER_BOUND('',#3771,.T.);
#2918=FACE_OUTER_BOUND('',#3772,.T.);
#2919=FACE_OUTER_BOUND('',#3773,.T.);
#2920=FACE_OUTER_BOUND('',#3774,.T.);
#2921=FACE_OUTER_BOUND('',#3775,.T.);
#2922=FACE_OUTER_BOUND('',#3776,.T.);
#2923=FACE_OUTER_BOUND('',#3777,.T.);
#2924=FACE_OUTER_BOUND('',#3778,.T.);
#2925=FACE_OUTER_BOUND('',#3779,.T.);
#2926=FACE_OUTER_BOUND('',#3780,.T.);
#2927=FACE_OUTER_BOUND('',#3781,.T.);
#2928=FACE_OUTER_BOUND('',#3782,.T.);
#2929=FACE_OUTER_BOUND('',#3783,.T.);
#2930=FACE_OUTER_BOUND('',#3784,.T.);
#2931=FACE_OUTER_BOUND('',#3785,.T.);
#2932=FACE_OUTER_BOUND('',#3786,.T.);
#2933=FACE_OUTER_BOUND('',#3787,.T.);
#2934=FACE_OUTER_BOUND('',#3788,.T.);
#2935=FACE_OUTER_BOUND('',#3789,.T.);
#2936=FACE_OUTER_BOUND('',#3790,.T.);
#2937=FACE_OUTER_BOUND('',#3791,.T.);
#2938=FACE_OUTER_BOUND('',#3792,.T.);
#2939=FACE_OUTER_BOUND('',#3793,.T.);
#2940=FACE_OUTER_BOUND('',#3794,.T.);
#2941=FACE_OUTER_BOUND('',#3795,.T.);
#2942=FACE_OUTER_BOUND('',#3796,.T.);
#2943=FACE_OUTER_BOUND('',#3797,.T.);
#2944=FACE_OUTER_BOUND('',#3798,.T.);
#2945=FACE_OUTER_BOUND('',#3799,.T.);
#2946=FACE_OUTER_BOUND('',#3800,.T.);
#2947=FACE_OUTER_BOUND('',#3801,.T.);
#2948=FACE_OUTER_BOUND('',#3802,.T.);
#2949=FACE_OUTER_BOUND('',#3803,.T.);
#2950=FACE_OUTER_BOUND('',#3804,.T.);
#2951=FACE_OUTER_BOUND('',#3805,.T.);
#2952=FACE_OUTER_BOUND('',#3806,.T.);
#2953=FACE_OUTER_BOUND('',#3807,.T.);
#2954=FACE_OUTER_BOUND('',#3808,.T.);
#2955=FACE_OUTER_BOUND('',#3809,.T.);
#2956=FACE_OUTER_BOUND('',#3810,.T.);
#2957=FACE_OUTER_BOUND('',#3811,.T.);
#2958=FACE_OUTER_BOUND('',#3812,.T.);
#2959=FACE_OUTER_BOUND('',#3813,.T.);
#2960=FACE_OUTER_BOUND('',#3814,.T.);
#2961=FACE_OUTER_BOUND('',#3815,.T.);
#2962=FACE_OUTER_BOUND('',#3816,.T.);
#2963=FACE_OUTER_BOUND('',#3817,.T.);
#2964=FACE_OUTER_BOUND('',#3818,.T.);
#2965=FACE_OUTER_BOUND('',#3819,.T.);
#2966=FACE_OUTER_BOUND('',#3820,.T.);
#2967=FACE_OUTER_BOUND('',#3821,.T.);
#2968=FACE_OUTER_BOUND('',#3822,.T.);
#2969=FACE_OUTER_BOUND('',#3823,.T.);
#2970=FACE_OUTER_BOUND('',#3824,.T.);
#2971=FACE_OUTER_BOUND('',#3825,.T.);
#2972=FACE_OUTER_BOUND('',#3826,.T.);
#2973=FACE_OUTER_BOUND('',#3827,.T.);
#2974=FACE_OUTER_BOUND('',#3828,.T.);
#2975=FACE_OUTER_BOUND('',#3829,.T.);
#2976=FACE_OUTER_BOUND('',#3830,.T.);
#2977=FACE_OUTER_BOUND('',#3831,.T.);
#2978=FACE_OUTER_BOUND('',#3832,.T.);
#2979=FACE_OUTER_BOUND('',#3833,.T.);
#2980=FACE_OUTER_BOUND('',#3834,.T.);
#2981=FACE_OUTER_BOUND('',#3835,.T.);
#2982=FACE_OUTER_BOUND('',#3836,.T.);
#2983=FACE_OUTER_BOUND('',#3837,.T.);
#2984=FACE_OUTER_BOUND('',#3838,.T.);
#2985=FACE_OUTER_BOUND('',#3839,.T.);
#2986=FACE_OUTER_BOUND('',#3840,.T.);
#2987=FACE_OUTER_BOUND('',#3841,.T.);
#2988=FACE_OUTER_BOUND('',#3842,.T.);
#2989=FACE_OUTER_BOUND('',#3843,.T.);
#2990=FACE_OUTER_BOUND('',#3844,.T.);
#2991=FACE_OUTER_BOUND('',#3845,.T.);
#2992=FACE_OUTER_BOUND('',#3846,.T.);
#2993=FACE_OUTER_BOUND('',#3847,.T.);
#2994=FACE_OUTER_BOUND('',#3848,.T.);
#2995=FACE_OUTER_BOUND('',#3849,.T.);
#2996=FACE_OUTER_BOUND('',#3850,.T.);
#2997=FACE_OUTER_BOUND('',#3851,.T.);
#2998=FACE_OUTER_BOUND('',#3852,.T.);
#2999=FACE_OUTER_BOUND('',#3853,.T.);
#3000=FACE_OUTER_BOUND('',#3854,.T.);
#3001=FACE_OUTER_BOUND('',#3855,.T.);
#3002=FACE_OUTER_BOUND('',#3856,.T.);
#3003=FACE_OUTER_BOUND('',#3857,.T.);
#3004=FACE_OUTER_BOUND('',#3858,.T.);
#3005=FACE_OUTER_BOUND('',#3859,.T.);
#3006=FACE_OUTER_BOUND('',#3860,.T.);
#3007=FACE_OUTER_BOUND('',#3861,.T.);
#3008=FACE_OUTER_BOUND('',#3862,.T.);
#3009=FACE_OUTER_BOUND('',#3863,.T.);
#3010=FACE_OUTER_BOUND('',#3864,.T.);
#3011=FACE_OUTER_BOUND('',#3865,.T.);
#3012=FACE_OUTER_BOUND('',#3866,.T.);
#3013=FACE_OUTER_BOUND('',#3867,.T.);
#3014=FACE_OUTER_BOUND('',#3868,.T.);
#3015=FACE_OUTER_BOUND('',#3869,.T.);
#3016=FACE_OUTER_BOUND('',#3870,.T.);
#3017=FACE_OUTER_BOUND('',#3871,.T.);
#3018=FACE_OUTER_BOUND('',#3872,.T.);
#3019=FACE_OUTER_BOUND('',#3873,.T.);
#3020=FACE_OUTER_BOUND('',#3874,.T.);
#3021=FACE_OUTER_BOUND('',#3875,.T.);
#3022=FACE_OUTER_BOUND('',#3876,.T.);
#3023=FACE_OUTER_BOUND('',#3877,.T.);
#3024=FACE_OUTER_BOUND('',#3878,.T.);
#3025=FACE_OUTER_BOUND('',#3879,.T.);
#3026=FACE_OUTER_BOUND('',#3880,.T.);
#3027=FACE_OUTER_BOUND('',#3881,.T.);
#3028=FACE_OUTER_BOUND('',#3882,.T.);
#3029=FACE_OUTER_BOUND('',#3883,.T.);
#3030=FACE_OUTER_BOUND('',#3884,.T.);
#3031=FACE_OUTER_BOUND('',#3885,.T.);
#3032=FACE_OUTER_BOUND('',#3886,.T.);
#3033=FACE_OUTER_BOUND('',#3887,.T.);
#3034=FACE_OUTER_BOUND('',#3888,.T.);
#3035=FACE_OUTER_BOUND('',#3889,.T.);
#3036=FACE_OUTER_BOUND('',#3890,.T.);
#3037=FACE_OUTER_BOUND('',#3891,.T.);
#3038=FACE_OUTER_BOUND('',#3892,.T.);
#3039=FACE_OUTER_BOUND('',#3893,.T.);
#3040=FACE_OUTER_BOUND('',#3894,.T.);
#3041=FACE_OUTER_BOUND('',#3895,.T.);
#3042=FACE_OUTER_BOUND('',#3896,.T.);
#3043=FACE_OUTER_BOUND('',#3897,.T.);
#3044=FACE_OUTER_BOUND('',#3898,.T.);
#3045=FACE_OUTER_BOUND('',#3899,.T.);
#3046=FACE_OUTER_BOUND('',#3900,.T.);
#3047=FACE_OUTER_BOUND('',#3906,.T.);
#3048=FACE_OUTER_BOUND('',#3907,.T.);
#3049=FACE_OUTER_BOUND('',#3908,.T.);
#3050=FACE_OUTER_BOUND('',#3909,.T.);
#3051=FACE_OUTER_BOUND('',#3911,.T.);
#3052=FACE_OUTER_BOUND('',#3912,.T.);
#3053=FACE_OUTER_BOUND('',#3913,.T.);
#3054=FACE_OUTER_BOUND('',#3914,.T.);
#3055=FACE_OUTER_BOUND('',#3915,.T.);
#3056=FACE_OUTER_BOUND('',#3917,.T.);
#3057=FACE_OUTER_BOUND('',#3919,.T.);
#3058=FACE_OUTER_BOUND('',#3921,.T.);
#3059=FACE_OUTER_BOUND('',#3922,.T.);
#3060=FACE_OUTER_BOUND('',#3923,.T.);
#3061=FACE_OUTER_BOUND('',#3925,.T.);
#3062=FACE_OUTER_BOUND('',#3927,.T.);
#3063=FACE_OUTER_BOUND('',#3928,.T.);
#3064=FACE_OUTER_BOUND('',#3929,.T.);
#3065=FACE_OUTER_BOUND('',#3930,.T.);
#3066=FACE_OUTER_BOUND('',#3932,.T.);
#3539=EDGE_LOOP('',(#9970,#9971,#9972));
#3540=EDGE_LOOP('',(#9973,#9974,#9975,#9976,#9977));
#3541=EDGE_LOOP('',(#9978,#9979,#9980,#9981));
#3542=EDGE_LOOP('',(#9982,#9983,#9984,#9985));
#3543=EDGE_LOOP('',(#9986,#9987,#9988,#9989));
#3544=EDGE_LOOP('',(#9990,#9991,#9992,#9993));
#3545=EDGE_LOOP('',(#9994,#9995,#9996,#9997));
#3546=EDGE_LOOP('',(#9998,#9999,#10000,#10001));
#3547=EDGE_LOOP('',(#10002,#10003,#10004,#10005));
#3548=EDGE_LOOP('',(#10006,#10007,#10008,#10009));
#3549=EDGE_LOOP('',(#10010,#10011,#10012,#10013));
#3550=EDGE_LOOP('',(#10014,#10015,#10016,#10017));
#3551=EDGE_LOOP('',(#10018,#10019,#10020,#10021));
#3552=EDGE_LOOP('',(#10022,#10023,#10024,#10025));
#3553=EDGE_LOOP('',(#10026,#10027,#10028,#10029,#10030,#10031,#10032,#10033));
#3554=EDGE_LOOP('',(#10034,#10035,#10036,#10037));
#3555=EDGE_LOOP('',(#10038,#10039,#10040,#10041));
#3556=EDGE_LOOP('',(#10042,#10043,#10044,#10045));
#3557=EDGE_LOOP('',(#10046,#10047,#10048,#10049));
#3558=EDGE_LOOP('',(#10050,#10051,#10052,#10053));
#3559=EDGE_LOOP('',(#10054,#10055,#10056,#10057));
#3560=EDGE_LOOP('',(#10058,#10059,#10060,#10061));
#3561=EDGE_LOOP('',(#10062,#10063,#10064,#10065));
#3562=EDGE_LOOP('',(#10066,#10067,#10068,#10069));
#3563=EDGE_LOOP('',(#10070,#10071,#10072,#10073));
#3564=EDGE_LOOP('',(#10074,#10075,#10076,#10077));
#3565=EDGE_LOOP('',(#10078,#10079,#10080,#10081));
#3566=EDGE_LOOP('',(#10082,#10083,#10084,#10085));
#3567=EDGE_LOOP('',(#10086,#10087,#10088,#10089));
#3568=EDGE_LOOP('',(#10090,#10091,#10092,#10093));
#3569=EDGE_LOOP('',(#10094,#10095,#10096,#10097));
#3570=EDGE_LOOP('',(#10098,#10099,#10100,#10101));
#3571=EDGE_LOOP('',(#10102,#10103,#10104,#10105));
#3572=EDGE_LOOP('',(#10106,#10107,#10108,#10109));
#3573=EDGE_LOOP('',(#10110,#10111,#10112,#10113));
#3574=EDGE_LOOP('',(#10114,#10115,#10116,#10117));
#3575=EDGE_LOOP('',(#10118,#10119,#10120,#10121));
#3576=EDGE_LOOP('',(#10122,#10123,#10124,#10125));
#3577=EDGE_LOOP('',(#10126,#10127,#10128,#10129));
#3578=EDGE_LOOP('',(#10130,#10131,#10132,#10133));
#3579=EDGE_LOOP('',(#10134,#10135,#10136,#10137));
#3580=EDGE_LOOP('',(#10138,#10139,#10140,#10141));
#3581=EDGE_LOOP('',(#10142,#10143,#10144,#10145));
#3582=EDGE_LOOP('',(#10146,#10147,#10148,#10149));
#3583=EDGE_LOOP('',(#10150,#10151,#10152,#10153));
#3584=EDGE_LOOP('',(#10154,#10155,#10156,#10157));
#3585=EDGE_LOOP('',(#10158,#10159,#10160,#10161));
#3586=EDGE_LOOP('',(#10162,#10163,#10164,#10165));
#3587=EDGE_LOOP('',(#10166,#10167,#10168,#10169));
#3588=EDGE_LOOP('',(#10170,#10171,#10172,#10173));
#3589=EDGE_LOOP('',(#10174,#10175,#10176,#10177));
#3590=EDGE_LOOP('',(#10178,#10179,#10180,#10181,#10182,#10183,#10184,#10185));
#3591=EDGE_LOOP('',(#10186,#10187,#10188,#10189));
#3592=EDGE_LOOP('',(#10190,#10191,#10192,#10193));
#3593=EDGE_LOOP('',(#10194,#10195,#10196,#10197));
#3594=EDGE_LOOP('',(#10198,#10199,#10200,#10201));
#3595=EDGE_LOOP('',(#10202,#10203,#10204,#10205));
#3596=EDGE_LOOP('',(#10206,#10207,#10208,#10209));
#3597=EDGE_LOOP('',(#10210,#10211,#10212,#10213));
#3598=EDGE_LOOP('',(#10214,#10215,#10216,#10217));
#3599=EDGE_LOOP('',(#10218,#10219,#10220,#10221));
#3600=EDGE_LOOP('',(#10222,#10223,#10224,#10225));
#3601=EDGE_LOOP('',(#10226,#10227,#10228,#10229));
#3602=EDGE_LOOP('',(#10230,#10231,#10232,#10233));
#3603=EDGE_LOOP('',(#10234,#10235,#10236,#10237));
#3604=EDGE_LOOP('',(#10238,#10239,#10240,#10241));
#3605=EDGE_LOOP('',(#10242,#10243,#10244,#10245));
#3606=EDGE_LOOP('',(#10246,#10247,#10248,#10249));
#3607=EDGE_LOOP('',(#10250,#10251,#10252,#10253));
#3608=EDGE_LOOP('',(#10254,#10255,#10256,#10257));
#3609=EDGE_LOOP('',(#10258,#10259,#10260,#10261));
#3610=EDGE_LOOP('',(#10262,#10263,#10264,#10265));
#3611=EDGE_LOOP('',(#10266,#10267,#10268,#10269));
#3612=EDGE_LOOP('',(#10270,#10271,#10272,#10273));
#3613=EDGE_LOOP('',(#10274,#10275,#10276,#10277));
#3614=EDGE_LOOP('',(#10278,#10279,#10280,#10281));
#3615=EDGE_LOOP('',(#10282,#10283,#10284,#10285));
#3616=EDGE_LOOP('',(#10286,#10287,#10288,#10289));
#3617=EDGE_LOOP('',(#10290,#10291,#10292,#10293));
#3618=EDGE_LOOP('',(#10294,#10295,#10296,#10297));
#3619=EDGE_LOOP('',(#10298,#10299,#10300,#10301));
#3620=EDGE_LOOP('',(#10302,#10303,#10304,#10305));
#3621=EDGE_LOOP('',(#10306,#10307,#10308,#10309));
#3622=EDGE_LOOP('',(#10310,#10311,#10312,#10313));
#3623=EDGE_LOOP('',(#10314,#10315,#10316,#10317));
#3624=EDGE_LOOP('',(#10318,#10319,#10320,#10321));
#3625=EDGE_LOOP('',(#10322,#10323,#10324,#10325));
#3626=EDGE_LOOP('',(#10326,#10327,#10328,#10329));
#3627=EDGE_LOOP('',(#10330,#10331,#10332,#10333,#10334,#10335,#10336,#10337));
#3628=EDGE_LOOP('',(#10338,#10339,#10340,#10341));
#3629=EDGE_LOOP('',(#10342,#10343,#10344,#10345));
#3630=EDGE_LOOP('',(#10346,#10347,#10348,#10349));
#3631=EDGE_LOOP('',(#10350,#10351,#10352,#10353));
#3632=EDGE_LOOP('',(#10354,#10355,#10356,#10357));
#3633=EDGE_LOOP('',(#10358,#10359,#10360,#10361));
#3634=EDGE_LOOP('',(#10362,#10363,#10364,#10365));
#3635=EDGE_LOOP('',(#10366,#10367,#10368,#10369));
#3636=EDGE_LOOP('',(#10370,#10371,#10372,#10373));
#3637=EDGE_LOOP('',(#10374,#10375,#10376,#10377));
#3638=EDGE_LOOP('',(#10378,#10379,#10380,#10381));
#3639=EDGE_LOOP('',(#10382,#10383,#10384,#10385));
#3640=EDGE_LOOP('',(#10386,#10387,#10388,#10389));
#3641=EDGE_LOOP('',(#10390,#10391,#10392,#10393));
#3642=EDGE_LOOP('',(#10394,#10395,#10396,#10397));
#3643=EDGE_LOOP('',(#10398,#10399,#10400,#10401));
#3644=EDGE_LOOP('',(#10402,#10403,#10404,#10405));
#3645=EDGE_LOOP('',(#10406,#10407,#10408,#10409));
#3646=EDGE_LOOP('',(#10410,#10411,#10412,#10413));
#3647=EDGE_LOOP('',(#10414,#10415,#10416,#10417));
#3648=EDGE_LOOP('',(#10418,#10419,#10420,#10421));
#3649=EDGE_LOOP('',(#10422,#10423,#10424,#10425));
#3650=EDGE_LOOP('',(#10426,#10427,#10428,#10429));
#3651=EDGE_LOOP('',(#10430,#10431,#10432,#10433));
#3652=EDGE_LOOP('',(#10434,#10435,#10436,#10437));
#3653=EDGE_LOOP('',(#10438,#10439,#10440,#10441));
#3654=EDGE_LOOP('',(#10442,#10443,#10444,#10445));
#3655=EDGE_LOOP('',(#10446,#10447,#10448,#10449));
#3656=EDGE_LOOP('',(#10450,#10451,#10452,#10453));
#3657=EDGE_LOOP('',(#10454,#10455,#10456,#10457));
#3658=EDGE_LOOP('',(#10458,#10459,#10460,#10461));
#3659=EDGE_LOOP('',(#10462,#10463,#10464,#10465));
#3660=EDGE_LOOP('',(#10466,#10467,#10468,#10469));
#3661=EDGE_LOOP('',(#10470,#10471,#10472,#10473));
#3662=EDGE_LOOP('',(#10474,#10475,#10476,#10477));
#3663=EDGE_LOOP('',(#10478,#10479,#10480,#10481));
#3664=EDGE_LOOP('',(#10482,#10483,#10484,#10485,#10486,#10487,#10488,#10489));
#3665=EDGE_LOOP('',(#10490,#10491,#10492,#10493));
#3666=EDGE_LOOP('',(#10494,#10495,#10496,#10497));
#3667=EDGE_LOOP('',(#10498,#10499,#10500,#10501));
#3668=EDGE_LOOP('',(#10502,#10503,#10504,#10505));
#3669=EDGE_LOOP('',(#10506,#10507,#10508,#10509));
#3670=EDGE_LOOP('',(#10510,#10511,#10512,#10513));
#3671=EDGE_LOOP('',(#10514,#10515,#10516,#10517));
#3672=EDGE_LOOP('',(#10518,#10519,#10520,#10521));
#3673=EDGE_LOOP('',(#10522,#10523,#10524,#10525));
#3674=EDGE_LOOP('',(#10526,#10527,#10528,#10529));
#3675=EDGE_LOOP('',(#10530,#10531,#10532,#10533));
#3676=EDGE_LOOP('',(#10534,#10535,#10536,#10537));
#3677=EDGE_LOOP('',(#10538,#10539,#10540,#10541));
#3678=EDGE_LOOP('',(#10542,#10543,#10544,#10545));
#3679=EDGE_LOOP('',(#10546,#10547,#10548,#10549));
#3680=EDGE_LOOP('',(#10550,#10551,#10552,#10553));
#3681=EDGE_LOOP('',(#10554,#10555,#10556,#10557));
#3682=EDGE_LOOP('',(#10558,#10559,#10560,#10561));
#3683=EDGE_LOOP('',(#10562,#10563,#10564,#10565));
#3684=EDGE_LOOP('',(#10566,#10567,#10568,#10569));
#3685=EDGE_LOOP('',(#10570,#10571,#10572,#10573));
#3686=EDGE_LOOP('',(#10574,#10575,#10576,#10577));
#3687=EDGE_LOOP('',(#10578,#10579,#10580,#10581));
#3688=EDGE_LOOP('',(#10582,#10583,#10584,#10585));
#3689=EDGE_LOOP('',(#10586,#10587,#10588,#10589));
#3690=EDGE_LOOP('',(#10590,#10591,#10592,#10593));
#3691=EDGE_LOOP('',(#10594,#10595,#10596,#10597));
#3692=EDGE_LOOP('',(#10598,#10599,#10600,#10601));
#3693=EDGE_LOOP('',(#10602,#10603,#10604,#10605));
#3694=EDGE_LOOP('',(#10606,#10607,#10608,#10609));
#3695=EDGE_LOOP('',(#10610,#10611,#10612,#10613));
#3696=EDGE_LOOP('',(#10614,#10615,#10616,#10617));
#3697=EDGE_LOOP('',(#10618,#10619,#10620,#10621));
#3698=EDGE_LOOP('',(#10622,#10623,#10624,#10625));
#3699=EDGE_LOOP('',(#10626,#10627,#10628,#10629));
#3700=EDGE_LOOP('',(#10630,#10631,#10632,#10633));
#3701=EDGE_LOOP('',(#10634,#10635,#10636,#10637,#10638,#10639,#10640,#10641));
#3702=EDGE_LOOP('',(#10642,#10643,#10644,#10645));
#3703=EDGE_LOOP('',(#10646,#10647,#10648,#10649));
#3704=EDGE_LOOP('',(#10650,#10651,#10652,#10653));
#3705=EDGE_LOOP('',(#10654,#10655,#10656,#10657));
#3706=EDGE_LOOP('',(#10658,#10659,#10660,#10661));
#3707=EDGE_LOOP('',(#10662,#10663,#10664,#10665));
#3708=EDGE_LOOP('',(#10666,#10667,#10668,#10669));
#3709=EDGE_LOOP('',(#10670,#10671,#10672,#10673));
#3710=EDGE_LOOP('',(#10674,#10675,#10676,#10677));
#3711=EDGE_LOOP('',(#10678,#10679,#10680,#10681));
#3712=EDGE_LOOP('',(#10682,#10683,#10684,#10685));
#3713=EDGE_LOOP('',(#10686,#10687,#10688,#10689));
#3714=EDGE_LOOP('',(#10690,#10691,#10692,#10693));
#3715=EDGE_LOOP('',(#10694,#10695,#10696,#10697));
#3716=EDGE_LOOP('',(#10698,#10699,#10700,#10701));
#3717=EDGE_LOOP('',(#10702,#10703,#10704,#10705));
#3718=EDGE_LOOP('',(#10706,#10707,#10708,#10709));
#3719=EDGE_LOOP('',(#10710,#10711,#10712,#10713));
#3720=EDGE_LOOP('',(#10714,#10715,#10716,#10717));
#3721=EDGE_LOOP('',(#10718,#10719,#10720,#10721));
#3722=EDGE_LOOP('',(#10722,#10723,#10724,#10725));
#3723=EDGE_LOOP('',(#10726,#10727,#10728,#10729));
#3724=EDGE_LOOP('',(#10730,#10731,#10732,#10733));
#3725=EDGE_LOOP('',(#10734,#10735,#10736,#10737));
#3726=EDGE_LOOP('',(#10738,#10739,#10740,#10741));
#3727=EDGE_LOOP('',(#10742,#10743,#10744,#10745));
#3728=EDGE_LOOP('',(#10746,#10747,#10748,#10749));
#3729=EDGE_LOOP('',(#10750,#10751,#10752,#10753));
#3730=EDGE_LOOP('',(#10754,#10755,#10756,#10757));
#3731=EDGE_LOOP('',(#10758,#10759,#10760,#10761));
#3732=EDGE_LOOP('',(#10762,#10763,#10764,#10765));
#3733=EDGE_LOOP('',(#10766,#10767,#10768,#10769));
#3734=EDGE_LOOP('',(#10770,#10771,#10772,#10773));
#3735=EDGE_LOOP('',(#10774,#10775,#10776,#10777));
#3736=EDGE_LOOP('',(#10778,#10779,#10780,#10781));
#3737=EDGE_LOOP('',(#10782,#10783,#10784,#10785));
#3738=EDGE_LOOP('',(#10786,#10787,#10788,#10789,#10790,#10791,#10792,#10793));
#3739=EDGE_LOOP('',(#10794,#10795,#10796,#10797));
#3740=EDGE_LOOP('',(#10798,#10799,#10800,#10801));
#3741=EDGE_LOOP('',(#10802,#10803,#10804,#10805));
#3742=EDGE_LOOP('',(#10806,#10807,#10808,#10809));
#3743=EDGE_LOOP('',(#10810,#10811,#10812,#10813));
#3744=EDGE_LOOP('',(#10814,#10815,#10816,#10817));
#3745=EDGE_LOOP('',(#10818,#10819,#10820,#10821));
#3746=EDGE_LOOP('',(#10822,#10823,#10824,#10825));
#3747=EDGE_LOOP('',(#10826,#10827,#10828,#10829));
#3748=EDGE_LOOP('',(#10830,#10831,#10832,#10833));
#3749=EDGE_LOOP('',(#10834,#10835,#10836,#10837));
#3750=EDGE_LOOP('',(#10838,#10839,#10840,#10841));
#3751=EDGE_LOOP('',(#10842,#10843,#10844,#10845));
#3752=EDGE_LOOP('',(#10846,#10847,#10848,#10849));
#3753=EDGE_LOOP('',(#10850,#10851,#10852,#10853));
#3754=EDGE_LOOP('',(#10854,#10855,#10856,#10857));
#3755=EDGE_LOOP('',(#10858,#10859,#10860,#10861));
#3756=EDGE_LOOP('',(#10862,#10863,#10864,#10865));
#3757=EDGE_LOOP('',(#10866,#10867,#10868,#10869));
#3758=EDGE_LOOP('',(#10870,#10871,#10872,#10873));
#3759=EDGE_LOOP('',(#10874,#10875,#10876,#10877));
#3760=EDGE_LOOP('',(#10878,#10879,#10880,#10881));
#3761=EDGE_LOOP('',(#10882,#10883,#10884,#10885));
#3762=EDGE_LOOP('',(#10886,#10887,#10888,#10889));
#3763=EDGE_LOOP('',(#10890,#10891,#10892,#10893));
#3764=EDGE_LOOP('',(#10894,#10895,#10896,#10897));
#3765=EDGE_LOOP('',(#10898,#10899,#10900,#10901));
#3766=EDGE_LOOP('',(#10902,#10903,#10904,#10905));
#3767=EDGE_LOOP('',(#10906,#10907,#10908,#10909));
#3768=EDGE_LOOP('',(#10910,#10911,#10912,#10913));
#3769=EDGE_LOOP('',(#10914,#10915,#10916,#10917));
#3770=EDGE_LOOP('',(#10918,#10919,#10920,#10921));
#3771=EDGE_LOOP('',(#10922,#10923,#10924,#10925));
#3772=EDGE_LOOP('',(#10926,#10927,#10928,#10929));
#3773=EDGE_LOOP('',(#10930,#10931,#10932,#10933));
#3774=EDGE_LOOP('',(#10934,#10935,#10936,#10937));
#3775=EDGE_LOOP('',(#10938,#10939,#10940,#10941,#10942,#10943,#10944,#10945));
#3776=EDGE_LOOP('',(#10946,#10947,#10948,#10949));
#3777=EDGE_LOOP('',(#10950,#10951,#10952,#10953));
#3778=EDGE_LOOP('',(#10954,#10955,#10956,#10957));
#3779=EDGE_LOOP('',(#10958,#10959,#10960,#10961));
#3780=EDGE_LOOP('',(#10962,#10963,#10964,#10965));
#3781=EDGE_LOOP('',(#10966,#10967,#10968,#10969));
#3782=EDGE_LOOP('',(#10970,#10971,#10972,#10973));
#3783=EDGE_LOOP('',(#10974,#10975,#10976,#10977));
#3784=EDGE_LOOP('',(#10978,#10979,#10980,#10981));
#3785=EDGE_LOOP('',(#10982,#10983,#10984,#10985));
#3786=EDGE_LOOP('',(#10986,#10987,#10988,#10989));
#3787=EDGE_LOOP('',(#10990,#10991,#10992,#10993));
#3788=EDGE_LOOP('',(#10994,#10995,#10996,#10997));
#3789=EDGE_LOOP('',(#10998,#10999,#11000,#11001));
#3790=EDGE_LOOP('',(#11002,#11003,#11004,#11005));
#3791=EDGE_LOOP('',(#11006,#11007,#11008,#11009));
#3792=EDGE_LOOP('',(#11010,#11011,#11012,#11013));
#3793=EDGE_LOOP('',(#11014,#11015,#11016,#11017));
#3794=EDGE_LOOP('',(#11018,#11019,#11020,#11021));
#3795=EDGE_LOOP('',(#11022,#11023,#11024,#11025));
#3796=EDGE_LOOP('',(#11026,#11027,#11028,#11029));
#3797=EDGE_LOOP('',(#11030,#11031,#11032,#11033));
#3798=EDGE_LOOP('',(#11034,#11035,#11036,#11037));
#3799=EDGE_LOOP('',(#11038,#11039,#11040,#11041));
#3800=EDGE_LOOP('',(#11042,#11043,#11044,#11045));
#3801=EDGE_LOOP('',(#11046,#11047,#11048,#11049));
#3802=EDGE_LOOP('',(#11050,#11051,#11052,#11053));
#3803=EDGE_LOOP('',(#11054,#11055,#11056,#11057));
#3804=EDGE_LOOP('',(#11058,#11059,#11060,#11061));
#3805=EDGE_LOOP('',(#11062,#11063,#11064,#11065));
#3806=EDGE_LOOP('',(#11066,#11067,#11068,#11069));
#3807=EDGE_LOOP('',(#11070,#11071,#11072,#11073));
#3808=EDGE_LOOP('',(#11074,#11075,#11076,#11077));
#3809=EDGE_LOOP('',(#11078,#11079,#11080,#11081));
#3810=EDGE_LOOP('',(#11082,#11083,#11084,#11085));
#3811=EDGE_LOOP('',(#11086,#11087,#11088,#11089));
#3812=EDGE_LOOP('',(#11090,#11091,#11092,#11093,#11094,#11095,#11096,#11097));
#3813=EDGE_LOOP('',(#11098,#11099,#11100,#11101));
#3814=EDGE_LOOP('',(#11102,#11103,#11104,#11105));
#3815=EDGE_LOOP('',(#11106,#11107,#11108,#11109));
#3816=EDGE_LOOP('',(#11110,#11111,#11112,#11113));
#3817=EDGE_LOOP('',(#11114,#11115,#11116,#11117));
#3818=EDGE_LOOP('',(#11118,#11119,#11120,#11121));
#3819=EDGE_LOOP('',(#11122,#11123,#11124,#11125));
#3820=EDGE_LOOP('',(#11126,#11127,#11128,#11129));
#3821=EDGE_LOOP('',(#11130,#11131,#11132,#11133));
#3822=EDGE_LOOP('',(#11134,#11135,#11136,#11137));
#3823=EDGE_LOOP('',(#11138,#11139,#11140,#11141));
#3824=EDGE_LOOP('',(#11142,#11143,#11144,#11145));
#3825=EDGE_LOOP('',(#11146,#11147,#11148,#11149));
#3826=EDGE_LOOP('',(#11150,#11151,#11152,#11153));
#3827=EDGE_LOOP('',(#11154,#11155,#11156,#11157));
#3828=EDGE_LOOP('',(#11158,#11159,#11160,#11161));
#3829=EDGE_LOOP('',(#11162,#11163,#11164,#11165));
#3830=EDGE_LOOP('',(#11166,#11167,#11168,#11169));
#3831=EDGE_LOOP('',(#11170,#11171,#11172,#11173));
#3832=EDGE_LOOP('',(#11174,#11175,#11176,#11177));
#3833=EDGE_LOOP('',(#11178,#11179,#11180,#11181));
#3834=EDGE_LOOP('',(#11182,#11183,#11184,#11185));
#3835=EDGE_LOOP('',(#11186,#11187,#11188,#11189));
#3836=EDGE_LOOP('',(#11190,#11191,#11192,#11193));
#3837=EDGE_LOOP('',(#11194,#11195,#11196,#11197));
#3838=EDGE_LOOP('',(#11198,#11199,#11200,#11201));
#3839=EDGE_LOOP('',(#11202,#11203,#11204,#11205));
#3840=EDGE_LOOP('',(#11206,#11207,#11208,#11209));
#3841=EDGE_LOOP('',(#11210,#11211,#11212,#11213));
#3842=EDGE_LOOP('',(#11214,#11215,#11216,#11217));
#3843=EDGE_LOOP('',(#11218,#11219,#11220,#11221));
#3844=EDGE_LOOP('',(#11222,#11223,#11224,#11225));
#3845=EDGE_LOOP('',(#11226,#11227,#11228,#11229));
#3846=EDGE_LOOP('',(#11230,#11231,#11232,#11233));
#3847=EDGE_LOOP('',(#11234,#11235,#11236,#11237));
#3848=EDGE_LOOP('',(#11238,#11239,#11240,#11241));
#3849=EDGE_LOOP('',(#11242,#11243,#11244,#11245,#11246));
#3850=EDGE_LOOP('',(#11247,#11248,#11249,#11250));
#3851=EDGE_LOOP('',(#11251,#11252,#11253,#11254,#11255,#11256,#11257,#11258,
#11259,#11260,#11261,#11262,#11263,#11264,#11265,#11266,#11267,#11268,#11269,
#11270,#11271,#11272,#11273,#11274,#11275,#11276,#11277,#11278,#11279,#11280,
#11281,#11282,#11283,#11284,#11285,#11286,#11287,#11288,#11289,#11290,#11291));
#3852=EDGE_LOOP('',(#11292,#11293,#11294,#11295,#11296,#11297,#11298,#11299,
#11300,#11301,#11302,#11303,#11304,#11305,#11306,#11307,#11308,#11309,#11310,
#11311,#11312,#11313,#11314,#11315,#11316,#11317,#11318,#11319,#11320,#11321,
#11322,#11323,#11324,#11325,#11326,#11327,#11328,#11329,#11330,#11331,#11332));
#3853=EDGE_LOOP('',(#11333,#11334,#11335,#11336));
#3854=EDGE_LOOP('',(#11337,#11338,#11339,#11340,#11341));
#3855=EDGE_LOOP('',(#11342,#11343,#11344,#11345));
#3856=EDGE_LOOP('',(#11346,#11347,#11348,#11349,#11350,#11351,#11352,#11353,
#11354,#11355,#11356,#11357,#11358,#11359,#11360,#11361,#11362,#11363,#11364,
#11365,#11366,#11367,#11368,#11369,#11370,#11371,#11372,#11373,#11374,#11375,
#11376,#11377,#11378,#11379,#11380,#11381,#11382,#11383,#11384,#11385,#11386));
#3857=EDGE_LOOP('',(#11387,#11388,#11389,#11390,#11391,#11392,#11393,#11394,
#11395,#11396,#11397,#11398,#11399,#11400,#11401,#11402,#11403,#11404,#11405,
#11406,#11407,#11408,#11409,#11410,#11411,#11412,#11413,#11414,#11415,#11416,
#11417,#11418,#11419,#11420,#11421,#11422,#11423,#11424,#11425,#11426,#11427));
#3858=EDGE_LOOP('',(#11428,#11429,#11430,#11431));
#3859=EDGE_LOOP('',(#11432,#11433,#11434,#11435,#11436));
#3860=EDGE_LOOP('',(#11437,#11438,#11439,#11440));
#3861=EDGE_LOOP('',(#11441,#11442,#11443,#11444,#11445,#11446,#11447,#11448,
#11449,#11450,#11451,#11452,#11453,#11454,#11455,#11456,#11457,#11458,#11459,
#11460,#11461,#11462,#11463,#11464,#11465,#11466,#11467,#11468,#11469,#11470,
#11471,#11472,#11473,#11474,#11475,#11476,#11477,#11478,#11479,#11480,#11481));
#3862=EDGE_LOOP('',(#11482,#11483,#11484,#11485,#11486,#11487,#11488,#11489,
#11490,#11491,#11492,#11493,#11494,#11495,#11496,#11497,#11498,#11499,#11500,
#11501,#11502,#11503,#11504,#11505,#11506,#11507,#11508,#11509,#11510,#11511,
#11512,#11513,#11514,#11515,#11516,#11517,#11518,#11519,#11520,#11521,#11522));
#3863=EDGE_LOOP('',(#11523,#11524,#11525,#11526));
#3864=EDGE_LOOP('',(#11527,#11528,#11529,#11530,#11531));
#3865=EDGE_LOOP('',(#11532,#11533,#11534,#11535));
#3866=EDGE_LOOP('',(#11536,#11537,#11538,#11539,#11540,#11541,#11542,#11543,
#11544,#11545,#11546,#11547,#11548,#11549,#11550,#11551,#11552,#11553,#11554,
#11555,#11556,#11557,#11558,#11559,#11560,#11561,#11562,#11563,#11564,#11565,
#11566,#11567,#11568,#11569,#11570,#11571,#11572,#11573,#11574,#11575,#11576));
#3867=EDGE_LOOP('',(#11577,#11578,#11579,#11580,#11581,#11582,#11583,#11584,
#11585,#11586,#11587,#11588,#11589,#11590,#11591,#11592,#11593,#11594,#11595,
#11596,#11597,#11598,#11599,#11600,#11601,#11602,#11603,#11604,#11605,#11606,
#11607,#11608,#11609,#11610,#11611,#11612,#11613,#11614,#11615,#11616,#11617));
#3868=EDGE_LOOP('',(#11618,#11619,#11620,#11621));
#3869=EDGE_LOOP('',(#11622));
#3870=EDGE_LOOP('',(#11623));
#3871=EDGE_LOOP('',(#11624));
#3872=EDGE_LOOP('',(#11625));
#3873=EDGE_LOOP('',(#11626,#11627,#11628,#11629,#11630));
#3874=EDGE_LOOP('',(#11631,#11632,#11633,#11634));
#3875=EDGE_LOOP('',(#11635,#11636,#11637,#11638,#11639,#11640,#11641,#11642,
#11643,#11644,#11645,#11646,#11647,#11648,#11649,#11650,#11651,#11652,#11653,
#11654,#11655,#11656,#11657,#11658,#11659,#11660,#11661,#11662,#11663,#11664,
#11665,#11666,#11667,#11668,#11669,#11670,#11671,#11672,#11673,#11674,#11675));
#3876=EDGE_LOOP('',(#11676,#11677,#11678,#11679,#11680,#11681,#11682,#11683,
#11684,#11685,#11686,#11687,#11688,#11689,#11690,#11691,#11692,#11693,#11694,
#11695,#11696,#11697,#11698,#11699,#11700,#11701,#11702,#11703,#11704,#11705,
#11706,#11707,#11708,#11709,#11710,#11711,#11712,#11713,#11714,#11715,#11716));
#3877=EDGE_LOOP('',(#11717,#11718,#11719,#11720));
#3878=EDGE_LOOP('',(#11721,#11722,#11723,#11724,#11725));
#3879=EDGE_LOOP('',(#11726,#11727,#11728,#11729));
#3880=EDGE_LOOP('',(#11730,#11731,#11732,#11733,#11734,#11735,#11736,#11737,
#11738,#11739,#11740,#11741,#11742,#11743,#11744,#11745,#11746,#11747,#11748,
#11749,#11750,#11751,#11752,#11753,#11754,#11755,#11756,#11757,#11758,#11759,
#11760,#11761,#11762,#11763,#11764,#11765,#11766,#11767,#11768,#11769,#11770));
#3881=EDGE_LOOP('',(#11771,#11772,#11773,#11774,#11775,#11776,#11777,#11778,
#11779,#11780,#11781,#11782,#11783,#11784,#11785,#11786,#11787,#11788,#11789,
#11790,#11791,#11792,#11793,#11794,#11795,#11796,#11797,#11798,#11799,#11800,
#11801,#11802,#11803,#11804,#11805,#11806,#11807,#11808,#11809,#11810,#11811));
#3882=EDGE_LOOP('',(#11812,#11813,#11814,#11815));
#3883=EDGE_LOOP('',(#11816,#11817,#11818,#11819,#11820));
#3884=EDGE_LOOP('',(#11821,#11822,#11823,#11824));
#3885=EDGE_LOOP('',(#11825,#11826,#11827,#11828,#11829,#11830,#11831,#11832,
#11833,#11834,#11835,#11836,#11837,#11838,#11839,#11840,#11841,#11842,#11843,
#11844,#11845,#11846,#11847,#11848,#11849,#11850,#11851,#11852,#11853,#11854,
#11855,#11856,#11857,#11858,#11859,#11860,#11861,#11862,#11863,#11864,#11865));
#3886=EDGE_LOOP('',(#11866,#11867,#11868,#11869,#11870,#11871,#11872,#11873,
#11874,#11875,#11876,#11877,#11878,#11879,#11880,#11881,#11882,#11883,#11884,
#11885,#11886,#11887,#11888,#11889,#11890,#11891,#11892,#11893,#11894,#11895,
#11896,#11897,#11898,#11899,#11900,#11901,#11902,#11903,#11904,#11905,#11906));
#3887=EDGE_LOOP('',(#11907,#11908,#11909,#11910));
#3888=EDGE_LOOP('',(#11911,#11912,#11913,#11914,#11915));
#3889=EDGE_LOOP('',(#11916,#11917,#11918,#11919));
#3890=EDGE_LOOP('',(#11920,#11921,#11922,#11923,#11924,#11925,#11926,#11927,
#11928,#11929,#11930,#11931,#11932,#11933,#11934,#11935,#11936,#11937,#11938,
#11939,#11940,#11941,#11942,#11943,#11944,#11945,#11946,#11947,#11948,#11949,
#11950,#11951,#11952,#11953,#11954,#11955,#11956,#11957,#11958,#11959,#11960));
#3891=EDGE_LOOP('',(#11961,#11962,#11963,#11964,#11965,#11966,#11967,#11968,
#11969,#11970,#11971,#11972,#11973,#11974,#11975,#11976,#11977,#11978,#11979,
#11980,#11981,#11982,#11983,#11984,#11985,#11986,#11987,#11988,#11989,#11990,
#11991,#11992,#11993,#11994,#11995,#11996,#11997,#11998,#11999,#12000,#12001));
#3892=EDGE_LOOP('',(#12002,#12003,#12004,#12005));
#3893=EDGE_LOOP('',(#12006));
#3894=EDGE_LOOP('',(#12007));
#3895=EDGE_LOOP('',(#12008));
#3896=EDGE_LOOP('',(#12009));
#3897=EDGE_LOOP('',(#12010,#12011,#12012,#12013));
#3898=EDGE_LOOP('',(#12014,#12015,#12016,#12017));
#3899=EDGE_LOOP('',(#12018,#12019,#12020,#12021));
#3900=EDGE_LOOP('',(#12022,#12023,#12024,#12025));
#3901=EDGE_LOOP('',(#12026,#12027,#12028,#12029));
#3902=EDGE_LOOP('',(#12030,#12031,#12032,#12033));
#3903=EDGE_LOOP('',(#12034,#12035,#12036,#12037));
#3904=EDGE_LOOP('',(#12038,#12039,#12040,#12041));
#3905=EDGE_LOOP('',(#12042));
#3906=EDGE_LOOP('',(#12043,#12044,#12045,#12046));
#3907=EDGE_LOOP('',(#12047,#12048,#12049,#12050,#12051,#12052,#12053,#12054,
#12055,#12056,#12057,#12058,#12059,#12060,#12061,#12062,#12063,#12064));
#3908=EDGE_LOOP('',(#12065,#12066,#12067,#12068,#12069,#12070,#12071,#12072,
#12073,#12074,#12075,#12076,#12077,#12078,#12079,#12080,#12081));
#3909=EDGE_LOOP('',(#12082,#12083,#12084,#12085));
#3910=EDGE_LOOP('',(#12086,#12087,#12088,#12089));
#3911=EDGE_LOOP('',(#12090,#12091,#12092,#12093));
#3912=EDGE_LOOP('',(#12094,#12095,#12096,#12097));
#3913=EDGE_LOOP('',(#12098,#12099,#12100,#12101));
#3914=EDGE_LOOP('',(#12102,#12103,#12104,#12105));
#3915=EDGE_LOOP('',(#12106,#12107,#12108,#12109));
#3916=EDGE_LOOP('',(#12110,#12111,#12112,#12113,#12114));
#3917=EDGE_LOOP('',(#12115));
#3918=EDGE_LOOP('',(#12116));
#3919=EDGE_LOOP('',(#12117));
#3920=EDGE_LOOP('',(#12118));
#3921=EDGE_LOOP('',(#12119,#12120,#12121,#12122));
#3922=EDGE_LOOP('',(#12123,#12124,#12125,#12126));
#3923=EDGE_LOOP('',(#12127));
#3924=EDGE_LOOP('',(#12128));
#3925=EDGE_LOOP('',(#12129));
#3926=EDGE_LOOP('',(#12130));
#3927=EDGE_LOOP('',(#12131,#12132,#12133,#12134));
#3928=EDGE_LOOP('',(#12135,#12136,#12137,#12138));
#3929=EDGE_LOOP('',(#12139,#12140,#12141,#12142));
#3930=EDGE_LOOP('',(#12143,#12144,#12145,#12146));
#3931=EDGE_LOOP('',(#12147,#12148,#12149,#12150));
#3932=EDGE_LOOP('',(#12151,#12152,#12153,#12154));
#3933=EDGE_LOOP('',(#12155,#12156,#12157,#12158));
#3934=EDGE_LOOP('',(#12159,#12160,#12161,#12162));
#3935=EDGE_LOOP('',(#12163,#12164,#12165,#12166));
#3936=EDGE_LOOP('',(#12167,#12168,#12169,#12170));
#3937=EDGE_LOOP('',(#12171));
#4456=LINE('',#20086,#5219);
#4457=LINE('',#20105,#5220);
#4458=LINE('',#20194,#5221);
#4459=LINE('',#20281,#5222);
#4460=LINE('',#20371,#5223);
#4461=LINE('',#20458,#5224);
#4462=LINE('',#20548,#5225);
#4463=LINE('',#20617,#5226);
#4464=LINE('',#20647,#5227);
#4465=LINE('',#20685,#5228);
#4466=LINE('',#20722,#5229);
#4467=LINE('',#20759,#5230);
#4468=LINE('',#20797,#5231);
#4469=LINE('',#20835,#5232);
#4470=LINE('',#20855,#5233);
#4471=LINE('',#20876,#5234);
#4472=LINE('',#20905,#5235);
#4473=LINE('',#20953,#5236);
#4474=LINE('',#21001,#5237);
#4475=LINE('',#21052,#5238);
#4476=LINE('',#21103,#5239);
#4477=LINE('',#21151,#5240);
#4478=LINE('',#21202,#5241);
#4479=LINE('',#21253,#5242);
#4480=LINE('',#21301,#5243);
#4481=LINE('',#21349,#5244);
#4482=LINE('',#21403,#5245);
#4483=LINE('',#21451,#5246);
#4484=LINE('',#21499,#5247);
#4485=LINE('',#21550,#5248);
#4486=LINE('',#21601,#5249);
#4487=LINE('',#21649,#5250);
#4488=LINE('',#21700,#5251);
#4489=LINE('',#21739,#5252);
#4490=LINE('',#21757,#5253);
#4491=LINE('',#21782,#5254);
#4492=LINE('',#21806,#5255);
#4493=LINE('',#21831,#5256);
#4494=LINE('',#21855,#5257);
#4495=LINE('',#21880,#5258);
#4496=LINE('',#21905,#5259);
#4497=LINE('',#21929,#5260);
#4498=LINE('',#21954,#5261);
#4499=LINE('',#21978,#5262);
#4500=LINE('',#22003,#5263);
#4501=LINE('',#22028,#5264);
#4502=LINE('',#22052,#5265);
#4503=LINE('',#22077,#5266);
#4504=LINE('',#22101,#5267);
#4505=LINE('',#22126,#5268);
#4506=LINE('',#22151,#5269);
#4507=LINE('',#22175,#5270);
#4508=LINE('',#22192,#5271);
#4509=LINE('',#22213,#5272);
#4510=LINE('',#22242,#5273);
#4511=LINE('',#22290,#5274);
#4512=LINE('',#22338,#5275);
#4513=LINE('',#22389,#5276);
#4514=LINE('',#22440,#5277);
#4515=LINE('',#22488,#5278);
#4516=LINE('',#22539,#5279);
#4517=LINE('',#22590,#5280);
#4518=LINE('',#22638,#5281);
#4519=LINE('',#22686,#5282);
#4520=LINE('',#22740,#5283);
#4521=LINE('',#22788,#5284);
#4522=LINE('',#22836,#5285);
#4523=LINE('',#22887,#5286);
#4524=LINE('',#22938,#5287);
#4525=LINE('',#22986,#5288);
#4526=LINE('',#23037,#5289);
#4527=LINE('',#23076,#5290);
#4528=LINE('',#23094,#5291);
#4529=LINE('',#23119,#5292);
#4530=LINE('',#23143,#5293);
#4531=LINE('',#23168,#5294);
#4532=LINE('',#23192,#5295);
#4533=LINE('',#23217,#5296);
#4534=LINE('',#23242,#5297);
#4535=LINE('',#23266,#5298);
#4536=LINE('',#23291,#5299);
#4537=LINE('',#23315,#5300);
#4538=LINE('',#23340,#5301);
#4539=LINE('',#23365,#5302);
#4540=LINE('',#23389,#5303);
#4541=LINE('',#23414,#5304);
#4542=LINE('',#23438,#5305);
#4543=LINE('',#23463,#5306);
#4544=LINE('',#23488,#5307);
#4545=LINE('',#23512,#5308);
#4546=LINE('',#23529,#5309);
#4547=LINE('',#23550,#5310);
#4548=LINE('',#23579,#5311);
#4549=LINE('',#23627,#5312);
#4550=LINE('',#23675,#5313);
#4551=LINE('',#23726,#5314);
#4552=LINE('',#23777,#5315);
#4553=LINE('',#23825,#5316);
#4554=LINE('',#23876,#5317);
#4555=LINE('',#23927,#5318);
#4556=LINE('',#23975,#5319);
#4557=LINE('',#24023,#5320);
#4558=LINE('',#24077,#5321);
#4559=LINE('',#24125,#5322);
#4560=LINE('',#24173,#5323);
#4561=LINE('',#24224,#5324);
#4562=LINE('',#24275,#5325);
#4563=LINE('',#24323,#5326);
#4564=LINE('',#24374,#5327);
#4565=LINE('',#24413,#5328);
#4566=LINE('',#24431,#5329);
#4567=LINE('',#24456,#5330);
#4568=LINE('',#24480,#5331);
#4569=LINE('',#24505,#5332);
#4570=LINE('',#24529,#5333);
#4571=LINE('',#24554,#5334);
#4572=LINE('',#24579,#5335);
#4573=LINE('',#24603,#5336);
#4574=LINE('',#24628,#5337);
#4575=LINE('',#24652,#5338);
#4576=LINE('',#24677,#5339);
#4577=LINE('',#24702,#5340);
#4578=LINE('',#24726,#5341);
#4579=LINE('',#24751,#5342);
#4580=LINE('',#24775,#5343);
#4581=LINE('',#24800,#5344);
#4582=LINE('',#24825,#5345);
#4583=LINE('',#24849,#5346);
#4584=LINE('',#24866,#5347);
#4585=LINE('',#24887,#5348);
#4586=LINE('',#24916,#5349);
#4587=LINE('',#24964,#5350);
#4588=LINE('',#25012,#5351);
#4589=LINE('',#25063,#5352);
#4590=LINE('',#25114,#5353);
#4591=LINE('',#25162,#5354);
#4592=LINE('',#25213,#5355);
#4593=LINE('',#25264,#5356);
#4594=LINE('',#25312,#5357);
#4595=LINE('',#25360,#5358);
#4596=LINE('',#25414,#5359);
#4597=LINE('',#25462,#5360);
#4598=LINE('',#25510,#5361);
#4599=LINE('',#25561,#5362);
#4600=LINE('',#25612,#5363);
#4601=LINE('',#25660,#5364);
#4602=LINE('',#25711,#5365);
#4603=LINE('',#25750,#5366);
#4604=LINE('',#25768,#5367);
#4605=LINE('',#25793,#5368);
#4606=LINE('',#25817,#5369);
#4607=LINE('',#25842,#5370);
#4608=LINE('',#25866,#5371);
#4609=LINE('',#25891,#5372);
#4610=LINE('',#25916,#5373);
#4611=LINE('',#25940,#5374);
#4612=LINE('',#25965,#5375);
#4613=LINE('',#25989,#5376);
#4614=LINE('',#26014,#5377);
#4615=LINE('',#26039,#5378);
#4616=LINE('',#26063,#5379);
#4617=LINE('',#26088,#5380);
#4618=LINE('',#26112,#5381);
#4619=LINE('',#26137,#5382);
#4620=LINE('',#26162,#5383);
#4621=LINE('',#26186,#5384);
#4622=LINE('',#26203,#5385);
#4623=LINE('',#26224,#5386);
#4624=LINE('',#26253,#5387);
#4625=LINE('',#26301,#5388);
#4626=LINE('',#26349,#5389);
#4627=LINE('',#26400,#5390);
#4628=LINE('',#26451,#5391);
#4629=LINE('',#26499,#5392);
#4630=LINE('',#26550,#5393);
#4631=LINE('',#26601,#5394);
#4632=LINE('',#26649,#5395);
#4633=LINE('',#26697,#5396);
#4634=LINE('',#26751,#5397);
#4635=LINE('',#26799,#5398);
#4636=LINE('',#26847,#5399);
#4637=LINE('',#26898,#5400);
#4638=LINE('',#26949,#5401);
#4639=LINE('',#26997,#5402);
#4640=LINE('',#27048,#5403);
#4641=LINE('',#27087,#5404);
#4642=LINE('',#27105,#5405);
#4643=LINE('',#27130,#5406);
#4644=LINE('',#27154,#5407);
#4645=LINE('',#27179,#5408);
#4646=LINE('',#27203,#5409);
#4647=LINE('',#27228,#5410);
#4648=LINE('',#27253,#5411);
#4649=LINE('',#27277,#5412);
#4650=LINE('',#27302,#5413);
#4651=LINE('',#27326,#5414);
#4652=LINE('',#27351,#5415);
#4653=LINE('',#27376,#5416);
#4654=LINE('',#27400,#5417);
#4655=LINE('',#27425,#5418);
#4656=LINE('',#27449,#5419);
#4657=LINE('',#27474,#5420);
#4658=LINE('',#27499,#5421);
#4659=LINE('',#27523,#5422);
#4660=LINE('',#27540,#5423);
#4661=LINE('',#27561,#5424);
#4662=LINE('',#27590,#5425);
#4663=LINE('',#27638,#5426);
#4664=LINE('',#27686,#5427);
#4665=LINE('',#27737,#5428);
#4666=LINE('',#27788,#5429);
#4667=LINE('',#27836,#5430);
#4668=LINE('',#27887,#5431);
#4669=LINE('',#27938,#5432);
#4670=LINE('',#27986,#5433);
#4671=LINE('',#28034,#5434);
#4672=LINE('',#28088,#5435);
#4673=LINE('',#28136,#5436);
#4674=LINE('',#28184,#5437);
#4675=LINE('',#28235,#5438);
#4676=LINE('',#28286,#5439);
#4677=LINE('',#28334,#5440);
#4678=LINE('',#28385,#5441);
#4679=LINE('',#28424,#5442);
#4680=LINE('',#28442,#5443);
#4681=LINE('',#28467,#5444);
#4682=LINE('',#28491,#5445);
#4683=LINE('',#28516,#5446);
#4684=LINE('',#28540,#5447);
#4685=LINE('',#28565,#5448);
#4686=LINE('',#28590,#5449);
#4687=LINE('',#28614,#5450);
#4688=LINE('',#28639,#5451);
#4689=LINE('',#28663,#5452);
#4690=LINE('',#28688,#5453);
#4691=LINE('',#28713,#5454);
#4692=LINE('',#28737,#5455);
#4693=LINE('',#28762,#5456);
#4694=LINE('',#28786,#5457);
#4695=LINE('',#28811,#5458);
#4696=LINE('',#28836,#5459);
#4697=LINE('',#28860,#5460);
#4698=LINE('',#28877,#5461);
#4699=LINE('',#28898,#5462);
#4700=LINE('',#28927,#5463);
#4701=LINE('',#28975,#5464);
#4702=LINE('',#29023,#5465);
#4703=LINE('',#29074,#5466);
#4704=LINE('',#29125,#5467);
#4705=LINE('',#29173,#5468);
#4706=LINE('',#29224,#5469);
#4707=LINE('',#29275,#5470);
#4708=LINE('',#29323,#5471);
#4709=LINE('',#29371,#5472);
#4710=LINE('',#29425,#5473);
#4711=LINE('',#29473,#5474);
#4712=LINE('',#29521,#5475);
#4713=LINE('',#29572,#5476);
#4714=LINE('',#29623,#5477);
#4715=LINE('',#29671,#5478);
#4716=LINE('',#29722,#5479);
#4717=LINE('',#29761,#5480);
#4718=LINE('',#29779,#5481);
#4719=LINE('',#29804,#5482);
#4720=LINE('',#29828,#5483);
#4721=LINE('',#29853,#5484);
#4722=LINE('',#29877,#5485);
#4723=LINE('',#29902,#5486);
#4724=LINE('',#29927,#5487);
#4725=LINE('',#29951,#5488);
#4726=LINE('',#29976,#5489);
#4727=LINE('',#30000,#5490);
#4728=LINE('',#30025,#5491);
#4729=LINE('',#30050,#5492);
#4730=LINE('',#30074,#5493);
#4731=LINE('',#30099,#5494);
#4732=LINE('',#30123,#5495);
#4733=LINE('',#30148,#5496);
#4734=LINE('',#30173,#5497);
#4735=LINE('',#30197,#5498);
#4736=LINE('',#30214,#5499);
#4737=LINE('',#30235,#5500);
#4738=LINE('',#30264,#5501);
#4739=LINE('',#30312,#5502);
#4740=LINE('',#30360,#5503);
#4741=LINE('',#30411,#5504);
#4742=LINE('',#30462,#5505);
#4743=LINE('',#30510,#5506);
#4744=LINE('',#30561,#5507);
#4745=LINE('',#30612,#5508);
#4746=LINE('',#30660,#5509);
#4747=LINE('',#30708,#5510);
#4748=LINE('',#30762,#5511);
#4749=LINE('',#30810,#5512);
#4750=LINE('',#30858,#5513);
#4751=LINE('',#30909,#5514);
#4752=LINE('',#30960,#5515);
#4753=LINE('',#31008,#5516);
#4754=LINE('',#31059,#5517);
#4755=LINE('',#31098,#5518);
#4756=LINE('',#31116,#5519);
#4757=LINE('',#31141,#5520);
#4758=LINE('',#31165,#5521);
#4759=LINE('',#31190,#5522);
#4760=LINE('',#31214,#5523);
#4761=LINE('',#31239,#5524);
#4762=LINE('',#31264,#5525);
#4763=LINE('',#31288,#5526);
#4764=LINE('',#31313,#5527);
#4765=LINE('',#31337,#5528);
#4766=LINE('',#31362,#5529);
#4767=LINE('',#31387,#5530);
#4768=LINE('',#31411,#5531);
#4769=LINE('',#31436,#5532);
#4770=LINE('',#31460,#5533);
#4771=LINE('',#31485,#5534);
#4772=LINE('',#31510,#5535);
#4773=LINE('',#31534,#5536);
#4774=LINE('',#42655,#5537);
#4775=LINE('',#42657,#5538);
#4776=LINE('',#42659,#5539);
#4777=LINE('',#42660,#5540);
#4778=LINE('',#42663,#5541);
#4779=LINE('',#42665,#5542);
#4780=LINE('',#42666,#5543);
#4781=LINE('',#42670,#5544);
#4782=LINE('',#42671,#5545);
#4783=LINE('',#42672,#5546);
#4784=LINE('',#44023,#5547);
#4785=LINE('',#44025,#5548);
#4786=LINE('',#44026,#5549);
#4787=LINE('',#44030,#5550);
#4788=LINE('',#44032,#5551);
#4789=LINE('',#44033,#5552);
#4790=LINE('',#44036,#5553);
#4791=LINE('',#44038,#5554);
#4792=LINE('',#44039,#5555);
#4793=LINE('',#44041,#5556);
#4794=LINE('',#44055,#5557);
#4795=LINE('',#44058,#5558);
#4796=LINE('',#44069,#5559);
#4797=LINE('',#44071,#5560);
#4798=LINE('',#44075,#5561);
#5219=VECTOR('',#17010,6.);
#5220=VECTOR('',#17015,6.);
#5221=VECTOR('',#17020,6.);
#5222=VECTOR('',#17023,6.);
#5223=VECTOR('',#17026,6.);
#5224=VECTOR('',#17029,6.);
#5225=VECTOR('',#17032,6.);
#5226=VECTOR('',#17037,6.11325000000001);
#5227=VECTOR('',#17042,6.11325000000001);
#5228=VECTOR('',#17045,6.11325000000001);
#5229=VECTOR('',#17048,6.11325000000001);
#5230=VECTOR('',#17051,6.11325000000001);
#5231=VECTOR('',#17054,6.11325000000001);
#5232=VECTOR('',#17057,6.11325000000001);
#5233=VECTOR('',#17062,2.);
#5234=VECTOR('',#17065,2.);
#5235=VECTOR('',#17072,2.);
#5236=VECTOR('',#17075,2.);
#5237=VECTOR('',#17078,2.);
#5238=VECTOR('',#17081,2.);
#5239=VECTOR('',#17084,2.);
#5240=VECTOR('',#17087,2.);
#5241=VECTOR('',#17090,2.);
#5242=VECTOR('',#17093,2.);
#5243=VECTOR('',#17096,2.);
#5244=VECTOR('',#17099,2.);
#5245=VECTOR('',#17102,2.);
#5246=VECTOR('',#17105,2.);
#5247=VECTOR('',#17108,2.);
#5248=VECTOR('',#17111,2.);
#5249=VECTOR('',#17114,2.);
#5250=VECTOR('',#17117,2.);
#5251=VECTOR('',#17120,2.);
#5252=VECTOR('',#17125,2.05475);
#5253=VECTOR('',#17130,2.05475);
#5254=VECTOR('',#17133,2.05475);
#5255=VECTOR('',#17136,2.05475);
#5256=VECTOR('',#17139,2.05475);
#5257=VECTOR('',#17142,2.05475);
#5258=VECTOR('',#17145,2.05475);
#5259=VECTOR('',#17148,2.05475);
#5260=VECTOR('',#17151,2.05475);
#5261=VECTOR('',#17154,2.05475);
#5262=VECTOR('',#17157,2.05475);
#5263=VECTOR('',#17160,2.05475);
#5264=VECTOR('',#17163,2.05475);
#5265=VECTOR('',#17166,2.05475);
#5266=VECTOR('',#17169,2.05475);
#5267=VECTOR('',#17172,2.05475);
#5268=VECTOR('',#17175,2.05475);
#5269=VECTOR('',#17178,2.05475);
#5270=VECTOR('',#17181,2.05475);
#5271=VECTOR('',#17186,2.);
#5272=VECTOR('',#17189,2.);
#5273=VECTOR('',#17196,2.);
#5274=VECTOR('',#17199,2.);
#5275=VECTOR('',#17202,2.);
#5276=VECTOR('',#17205,2.);
#5277=VECTOR('',#17208,2.);
#5278=VECTOR('',#17211,2.);
#5279=VECTOR('',#17214,2.);
#5280=VECTOR('',#17217,2.);
#5281=VECTOR('',#17220,2.);
#5282=VECTOR('',#17223,2.);
#5283=VECTOR('',#17226,2.);
#5284=VECTOR('',#17229,2.);
#5285=VECTOR('',#17232,2.);
#5286=VECTOR('',#17235,2.);
#5287=VECTOR('',#17238,2.);
#5288=VECTOR('',#17241,2.);
#5289=VECTOR('',#17244,2.);
#5290=VECTOR('',#17249,2.05475);
#5291=VECTOR('',#17254,2.05475);
#5292=VECTOR('',#17257,2.05475);
#5293=VECTOR('',#17260,2.05475);
#5294=VECTOR('',#17263,2.05475);
#5295=VECTOR('',#17266,2.05475);
#5296=VECTOR('',#17269,2.05475);
#5297=VECTOR('',#17272,2.05475);
#5298=VECTOR('',#17275,2.05475);
#5299=VECTOR('',#17278,2.05475);
#5300=VECTOR('',#17281,2.05475);
#5301=VECTOR('',#17284,2.05475);
#5302=VECTOR('',#17287,2.05475);
#5303=VECTOR('',#17290,2.05475);
#5304=VECTOR('',#17293,2.05475);
#5305=VECTOR('',#17296,2.05475);
#5306=VECTOR('',#17299,2.05475);
#5307=VECTOR('',#17302,2.05475);
#5308=VECTOR('',#17305,2.05475);
#5309=VECTOR('',#17310,2.);
#5310=VECTOR('',#17313,2.);
#5311=VECTOR('',#17320,2.);
#5312=VECTOR('',#17323,2.);
#5313=VECTOR('',#17326,2.);
#5314=VECTOR('',#17329,2.);
#5315=VECTOR('',#17332,2.);
#5316=VECTOR('',#17335,2.);
#5317=VECTOR('',#17338,2.);
#5318=VECTOR('',#17341,2.);
#5319=VECTOR('',#17344,2.);
#5320=VECTOR('',#17347,2.);
#5321=VECTOR('',#17350,2.);
#5322=VECTOR('',#17353,2.);
#5323=VECTOR('',#17356,2.);
#5324=VECTOR('',#17359,2.);
#5325=VECTOR('',#17362,2.);
#5326=VECTOR('',#17365,2.);
#5327=VECTOR('',#17368,2.);
#5328=VECTOR('',#17373,2.05475);
#5329=VECTOR('',#17378,2.05475);
#5330=VECTOR('',#17381,2.05475);
#5331=VECTOR('',#17384,2.05475);
#5332=VECTOR('',#17387,2.05475);
#5333=VECTOR('',#17390,2.05475);
#5334=VECTOR('',#17393,2.05475);
#5335=VECTOR('',#17396,2.05475);
#5336=VECTOR('',#17399,2.05475);
#5337=VECTOR('',#17402,2.05475);
#5338=VECTOR('',#17405,2.05475);
#5339=VECTOR('',#17408,2.05475);
#5340=VECTOR('',#17411,2.05475);
#5341=VECTOR('',#17414,2.05475);
#5342=VECTOR('',#17417,2.05475);
#5343=VECTOR('',#17420,2.05475);
#5344=VECTOR('',#17423,2.05475);
#5345=VECTOR('',#17426,2.05475);
#5346=VECTOR('',#17429,2.05475);
#5347=VECTOR('',#17434,2.);
#5348=VECTOR('',#17437,2.);
#5349=VECTOR('',#17444,2.);
#5350=VECTOR('',#17447,2.);
#5351=VECTOR('',#17450,2.);
#5352=VECTOR('',#17453,2.);
#5353=VECTOR('',#17456,2.);
#5354=VECTOR('',#17459,2.);
#5355=VECTOR('',#17462,2.);
#5356=VECTOR('',#17465,2.);
#5357=VECTOR('',#17468,2.);
#5358=VECTOR('',#17471,2.);
#5359=VECTOR('',#17474,2.);
#5360=VECTOR('',#17477,2.);
#5361=VECTOR('',#17480,2.);
#5362=VECTOR('',#17483,2.);
#5363=VECTOR('',#17486,2.);
#5364=VECTOR('',#17489,2.);
#5365=VECTOR('',#17492,2.);
#5366=VECTOR('',#17497,2.05475);
#5367=VECTOR('',#17502,2.05475);
#5368=VECTOR('',#17505,2.05475);
#5369=VECTOR('',#17508,2.05475);
#5370=VECTOR('',#17511,2.05475);
#5371=VECTOR('',#17514,2.05475);
#5372=VECTOR('',#17517,2.05475);
#5373=VECTOR('',#17520,2.05475);
#5374=VECTOR('',#17523,2.05475);
#5375=VECTOR('',#17526,2.05475);
#5376=VECTOR('',#17529,2.05475);
#5377=VECTOR('',#17532,2.05475);
#5378=VECTOR('',#17535,2.05475);
#5379=VECTOR('',#17538,2.05475);
#5380=VECTOR('',#17541,2.05475);
#5381=VECTOR('',#17544,2.05475);
#5382=VECTOR('',#17547,2.05475);
#5383=VECTOR('',#17550,2.05475);
#5384=VECTOR('',#17553,2.05475);
#5385=VECTOR('',#17558,2.);
#5386=VECTOR('',#17561,2.);
#5387=VECTOR('',#17568,2.);
#5388=VECTOR('',#17571,2.);
#5389=VECTOR('',#17574,2.);
#5390=VECTOR('',#17577,2.);
#5391=VECTOR('',#17580,2.);
#5392=VECTOR('',#17583,2.);
#5393=VECTOR('',#17586,2.);
#5394=VECTOR('',#17589,2.);
#5395=VECTOR('',#17592,2.);
#5396=VECTOR('',#17595,2.);
#5397=VECTOR('',#17598,2.);
#5398=VECTOR('',#17601,2.);
#5399=VECTOR('',#17604,2.);
#5400=VECTOR('',#17607,2.);
#5401=VECTOR('',#17610,2.);
#5402=VECTOR('',#17613,2.);
#5403=VECTOR('',#17616,2.);
#5404=VECTOR('',#17621,2.05475);
#5405=VECTOR('',#17626,2.05475);
#5406=VECTOR('',#17629,2.05475);
#5407=VECTOR('',#17632,2.05475);
#5408=VECTOR('',#17635,2.05475);
#5409=VECTOR('',#17638,2.05475);
#5410=VECTOR('',#17641,2.05475);
#5411=VECTOR('',#17644,2.05475);
#5412=VECTOR('',#17647,2.05475);
#5413=VECTOR('',#17650,2.05475);
#5414=VECTOR('',#17653,2.05475);
#5415=VECTOR('',#17656,2.05475);
#5416=VECTOR('',#17659,2.05475);
#5417=VECTOR('',#17662,2.05475);
#5418=VECTOR('',#17665,2.05475);
#5419=VECTOR('',#17668,2.05475);
#5420=VECTOR('',#17671,2.05475);
#5421=VECTOR('',#17674,2.05475);
#5422=VECTOR('',#17677,2.05475);
#5423=VECTOR('',#17682,2.);
#5424=VECTOR('',#17685,2.);
#5425=VECTOR('',#17692,2.);
#5426=VECTOR('',#17695,2.);
#5427=VECTOR('',#17698,2.);
#5428=VECTOR('',#17701,2.);
#5429=VECTOR('',#17704,2.);
#5430=VECTOR('',#17707,2.);
#5431=VECTOR('',#17710,2.);
#5432=VECTOR('',#17713,2.);
#5433=VECTOR('',#17716,2.);
#5434=VECTOR('',#17719,2.);
#5435=VECTOR('',#17722,2.);
#5436=VECTOR('',#17725,2.);
#5437=VECTOR('',#17728,2.);
#5438=VECTOR('',#17731,2.);
#5439=VECTOR('',#17734,2.);
#5440=VECTOR('',#17737,2.);
#5441=VECTOR('',#17740,2.);
#5442=VECTOR('',#17745,2.05475000000001);
#5443=VECTOR('',#17750,2.05475000000001);
#5444=VECTOR('',#17753,2.05475000000001);
#5445=VECTOR('',#17756,2.05475000000001);
#5446=VECTOR('',#17759,2.05475000000001);
#5447=VECTOR('',#17762,2.05475000000001);
#5448=VECTOR('',#17765,2.05475000000001);
#5449=VECTOR('',#17768,2.05475000000001);
#5450=VECTOR('',#17771,2.05475000000001);
#5451=VECTOR('',#17774,2.05475000000001);
#5452=VECTOR('',#17777,2.05475000000001);
#5453=VECTOR('',#17780,2.05475000000001);
#5454=VECTOR('',#17783,2.05475000000001);
#5455=VECTOR('',#17786,2.05475000000001);
#5456=VECTOR('',#17789,2.05475000000001);
#5457=VECTOR('',#17792,2.05475000000001);
#5458=VECTOR('',#17795,2.05475000000001);
#5459=VECTOR('',#17798,2.05475000000001);
#5460=VECTOR('',#17801,2.05475000000001);
#5461=VECTOR('',#17806,2.);
#5462=VECTOR('',#17809,2.);
#5463=VECTOR('',#17816,2.);
#5464=VECTOR('',#17819,2.);
#5465=VECTOR('',#17822,2.);
#5466=VECTOR('',#17825,2.);
#5467=VECTOR('',#17828,2.);
#5468=VECTOR('',#17831,2.);
#5469=VECTOR('',#17834,2.);
#5470=VECTOR('',#17837,2.);
#5471=VECTOR('',#17840,2.);
#5472=VECTOR('',#17843,2.);
#5473=VECTOR('',#17846,2.);
#5474=VECTOR('',#17849,2.);
#5475=VECTOR('',#17852,2.);
#5476=VECTOR('',#17855,2.);
#5477=VECTOR('',#17858,2.);
#5478=VECTOR('',#17861,2.);
#5479=VECTOR('',#17864,2.);
#5480=VECTOR('',#17869,2.05475);
#5481=VECTOR('',#17874,2.05475);
#5482=VECTOR('',#17877,2.05475);
#5483=VECTOR('',#17880,2.05475);
#5484=VECTOR('',#17883,2.05475);
#5485=VECTOR('',#17886,2.05475);
#5486=VECTOR('',#17889,2.05475);
#5487=VECTOR('',#17892,2.05475);
#5488=VECTOR('',#17895,2.05475);
#5489=VECTOR('',#17898,2.05475);
#5490=VECTOR('',#17901,2.05475);
#5491=VECTOR('',#17904,2.05475);
#5492=VECTOR('',#17907,2.05475);
#5493=VECTOR('',#17910,2.05475);
#5494=VECTOR('',#17913,2.05475);
#5495=VECTOR('',#17916,2.05475);
#5496=VECTOR('',#17919,2.05475);
#5497=VECTOR('',#17922,2.05475);
#5498=VECTOR('',#17925,2.05475);
#5499=VECTOR('',#17930,2.);
#5500=VECTOR('',#17933,2.);
#5501=VECTOR('',#17940,2.);
#5502=VECTOR('',#17943,2.);
#5503=VECTOR('',#17946,2.);
#5504=VECTOR('',#17949,2.);
#5505=VECTOR('',#17952,2.);
#5506=VECTOR('',#17955,2.);
#5507=VECTOR('',#17958,2.);
#5508=VECTOR('',#17961,2.);
#5509=VECTOR('',#17964,2.);
#5510=VECTOR('',#17967,2.);
#5511=VECTOR('',#17970,2.);
#5512=VECTOR('',#17973,2.);
#5513=VECTOR('',#17976,2.);
#5514=VECTOR('',#17979,2.);
#5515=VECTOR('',#17982,2.);
#5516=VECTOR('',#17985,2.);
#5517=VECTOR('',#17988,2.);
#5518=VECTOR('',#17993,2.05475000000001);
#5519=VECTOR('',#17998,2.05475000000001);
#5520=VECTOR('',#18001,2.05475000000001);
#5521=VECTOR('',#18004,2.05475000000001);
#5522=VECTOR('',#18007,2.05475000000001);
#5523=VECTOR('',#18010,2.05475000000001);
#5524=VECTOR('',#18013,2.05475000000001);
#5525=VECTOR('',#18016,2.05475000000001);
#5526=VECTOR('',#18019,2.05475000000001);
#5527=VECTOR('',#18022,2.05475000000001);
#5528=VECTOR('',#18025,2.05475000000001);
#5529=VECTOR('',#18028,2.05475000000001);
#5530=VECTOR('',#18031,2.05475000000001);
#5531=VECTOR('',#18034,2.05475000000001);
#5532=VECTOR('',#18037,2.05475000000001);
#5533=VECTOR('',#18040,2.05475000000001);
#5534=VECTOR('',#18043,2.05475000000001);
#5535=VECTOR('',#18046,2.05475000000001);
#5536=VECTOR('',#18049,2.05475000000001);
#5537=VECTOR('',#18118,10.);
#5538=VECTOR('',#18119,10.);
#5539=VECTOR('',#18120,10.);
#5540=VECTOR('',#18121,10.);
#5541=VECTOR('',#18124,10.);
#5542=VECTOR('',#18125,10.);
#5543=VECTOR('',#18126,10.);
#5544=VECTOR('',#18129,10.);
#5545=VECTOR('',#18130,10.);
#5546=VECTOR('',#18131,10.);
#5547=VECTOR('',#18144,10.);
#5548=VECTOR('',#18145,10.);
#5549=VECTOR('',#18146,10.);
#5550=VECTOR('',#18151,10.);
#5551=VECTOR('',#18152,10.);
#5552=VECTOR('',#18153,10.);
#5553=VECTOR('',#18156,10.);
#5554=VECTOR('',#18157,10.);
#5555=VECTOR('',#18158,10.);
#5556=VECTOR('',#18161,10.);
#5557=VECTOR('',#18180,35.);
#5558=VECTOR('',#18183,40.);
#5559=VECTOR('',#18198,35.);
#5560=VECTOR('',#18201,40.);
#5561=VECTOR('',#18206,40.);
#5991=VERTEX_POINT('',#20084);
#5992=VERTEX_POINT('',#20085);
#5993=VERTEX_POINT('',#20087);
#5994=VERTEX_POINT('',#20103);
#5995=VERTEX_POINT('',#20104);
#5996=VERTEX_POINT('',#20106);
#5997=VERTEX_POINT('',#20192);
#5998=VERTEX_POINT('',#20193);
#5999=VERTEX_POINT('',#20279);
#6000=VERTEX_POINT('',#20280);
#6001=VERTEX_POINT('',#20369);
#6002=VERTEX_POINT('',#20370);
#6003=VERTEX_POINT('',#20456);
#6004=VERTEX_POINT('',#20457);
#6005=VERTEX_POINT('',#20546);
#6006=VERTEX_POINT('',#20547);
#6007=VERTEX_POINT('',#20549);
#6008=VERTEX_POINT('',#20575);
#6009=VERTEX_POINT('',#20615);
#6010=VERTEX_POINT('',#20616);
#6011=VERTEX_POINT('',#20618);
#6012=VERTEX_POINT('',#20630);
#6013=VERTEX_POINT('',#20645);
#6014=VERTEX_POINT('',#20646);
#6015=VERTEX_POINT('',#20683);
#6016=VERTEX_POINT('',#20684);
#6017=VERTEX_POINT('',#20720);
#6018=VERTEX_POINT('',#20721);
#6019=VERTEX_POINT('',#20757);
#6020=VERTEX_POINT('',#20758);
#6021=VERTEX_POINT('',#20795);
#6022=VERTEX_POINT('',#20796);
#6023=VERTEX_POINT('',#20833);
#6024=VERTEX_POINT('',#20834);
#6025=VERTEX_POINT('',#20836);
#6026=VERTEX_POINT('',#20843);
#6027=VERTEX_POINT('',#20853);
#6028=VERTEX_POINT('',#20854);
#6029=VERTEX_POINT('',#20856);
#6030=VERTEX_POINT('',#20873);
#6031=VERTEX_POINT('',#20875);
#6032=VERTEX_POINT('',#20878);
#6033=VERTEX_POINT('',#20903);
#6034=VERTEX_POINT('',#20904);
#6035=VERTEX_POINT('',#20951);
#6036=VERTEX_POINT('',#20952);
#6037=VERTEX_POINT('',#20999);
#6038=VERTEX_POINT('',#21000);
#6039=VERTEX_POINT('',#21050);
#6040=VERTEX_POINT('',#21051);
#6041=VERTEX_POINT('',#21101);
#6042=VERTEX_POINT('',#21102);
#6043=VERTEX_POINT('',#21149);
#6044=VERTEX_POINT('',#21150);
#6045=VERTEX_POINT('',#21200);
#6046=VERTEX_POINT('',#21201);
#6047=VERTEX_POINT('',#21251);
#6048=VERTEX_POINT('',#21252);
#6049=VERTEX_POINT('',#21299);
#6050=VERTEX_POINT('',#21300);
#6051=VERTEX_POINT('',#21347);
#6052=VERTEX_POINT('',#21348);
#6053=VERTEX_POINT('',#21401);
#6054=VERTEX_POINT('',#21402);
#6055=VERTEX_POINT('',#21449);
#6056=VERTEX_POINT('',#21450);
#6057=VERTEX_POINT('',#21497);
#6058=VERTEX_POINT('',#21498);
#6059=VERTEX_POINT('',#21548);
#6060=VERTEX_POINT('',#21549);
#6061=VERTEX_POINT('',#21599);
#6062=VERTEX_POINT('',#21600);
#6063=VERTEX_POINT('',#21647);
#6064=VERTEX_POINT('',#21648);
#6065=VERTEX_POINT('',#21698);
#6066=VERTEX_POINT('',#21699);
#6067=VERTEX_POINT('',#21701);
#6068=VERTEX_POINT('',#21715);
#6069=VERTEX_POINT('',#21737);
#6070=VERTEX_POINT('',#21738);
#6071=VERTEX_POINT('',#21740);
#6072=VERTEX_POINT('',#21746);
#6073=VERTEX_POINT('',#21755);
#6074=VERTEX_POINT('',#21756);
#6075=VERTEX_POINT('',#21780);
#6076=VERTEX_POINT('',#21781);
#6077=VERTEX_POINT('',#21804);
#6078=VERTEX_POINT('',#21805);
#6079=VERTEX_POINT('',#21829);
#6080=VERTEX_POINT('',#21830);
#6081=VERTEX_POINT('',#21853);
#6082=VERTEX_POINT('',#21854);
#6083=VERTEX_POINT('',#21878);
#6084=VERTEX_POINT('',#21879);
#6085=VERTEX_POINT('',#21903);
#6086=VERTEX_POINT('',#21904);
#6087=VERTEX_POINT('',#21927);
#6088=VERTEX_POINT('',#21928);
#6089=VERTEX_POINT('',#21952);
#6090=VERTEX_POINT('',#21953);
#6091=VERTEX_POINT('',#21976);
#6092=VERTEX_POINT('',#21977);
#6093=VERTEX_POINT('',#22001);
#6094=VERTEX_POINT('',#22002);
#6095=VERTEX_POINT('',#22026);
#6096=VERTEX_POINT('',#22027);
#6097=VERTEX_POINT('',#22050);
#6098=VERTEX_POINT('',#22051);
#6099=VERTEX_POINT('',#22075);
#6100=VERTEX_POINT('',#22076);
#6101=VERTEX_POINT('',#22099);
#6102=VERTEX_POINT('',#22100);
#6103=VERTEX_POINT('',#22124);
#6104=VERTEX_POINT('',#22125);
#6105=VERTEX_POINT('',#22149);
#6106=VERTEX_POINT('',#22150);
#6107=VERTEX_POINT('',#22173);
#6108=VERTEX_POINT('',#22174);
#6109=VERTEX_POINT('',#22176);
#6110=VERTEX_POINT('',#22182);
#6111=VERTEX_POINT('',#22190);
#6112=VERTEX_POINT('',#22191);
#6113=VERTEX_POINT('',#22193);
#6114=VERTEX_POINT('',#22210);
#6115=VERTEX_POINT('',#22212);
#6116=VERTEX_POINT('',#22215);
#6117=VERTEX_POINT('',#22240);
#6118=VERTEX_POINT('',#22241);
#6119=VERTEX_POINT('',#22288);
#6120=VERTEX_POINT('',#22289);
#6121=VERTEX_POINT('',#22336);
#6122=VERTEX_POINT('',#22337);
#6123=VERTEX_POINT('',#22387);
#6124=VERTEX_POINT('',#22388);
#6125=VERTEX_POINT('',#22438);
#6126=VERTEX_POINT('',#22439);
#6127=VERTEX_POINT('',#22486);
#6128=VERTEX_POINT('',#22487);
#6129=VERTEX_POINT('',#22537);
#6130=VERTEX_POINT('',#22538);
#6131=VERTEX_POINT('',#22588);
#6132=VERTEX_POINT('',#22589);
#6133=VERTEX_POINT('',#22636);
#6134=VERTEX_POINT('',#22637);
#6135=VERTEX_POINT('',#22684);
#6136=VERTEX_POINT('',#22685);
#6137=VERTEX_POINT('',#22738);
#6138=VERTEX_POINT('',#22739);
#6139=VERTEX_POINT('',#22786);
#6140=VERTEX_POINT('',#22787);
#6141=VERTEX_POINT('',#22834);
#6142=VERTEX_POINT('',#22835);
#6143=VERTEX_POINT('',#22885);
#6144=VERTEX_POINT('',#22886);
#6145=VERTEX_POINT('',#22936);
#6146=VERTEX_POINT('',#22937);
#6147=VERTEX_POINT('',#22984);
#6148=VERTEX_POINT('',#22985);
#6149=VERTEX_POINT('',#23035);
#6150=VERTEX_POINT('',#23036);
#6151=VERTEX_POINT('',#23038);
#6152=VERTEX_POINT('',#23052);
#6153=VERTEX_POINT('',#23074);
#6154=VERTEX_POINT('',#23075);
#6155=VERTEX_POINT('',#23077);
#6156=VERTEX_POINT('',#23083);
#6157=VERTEX_POINT('',#23092);
#6158=VERTEX_POINT('',#23093);
#6159=VERTEX_POINT('',#23117);
#6160=VERTEX_POINT('',#23118);
#6161=VERTEX_POINT('',#23141);
#6162=VERTEX_POINT('',#23142);
#6163=VERTEX_POINT('',#23166);
#6164=VERTEX_POINT('',#23167);
#6165=VERTEX_POINT('',#23190);
#6166=VERTEX_POINT('',#23191);
#6167=VERTEX_POINT('',#23215);
#6168=VERTEX_POINT('',#23216);
#6169=VERTEX_POINT('',#23240);
#6170=VERTEX_POINT('',#23241);
#6171=VERTEX_POINT('',#23264);
#6172=VERTEX_POINT('',#23265);
#6173=VERTEX_POINT('',#23289);
#6174=VERTEX_POINT('',#23290);
#6175=VERTEX_POINT('',#23313);
#6176=VERTEX_POINT('',#23314);
#6177=VERTEX_POINT('',#23338);
#6178=VERTEX_POINT('',#23339);
#6179=VERTEX_POINT('',#23363);
#6180=VERTEX_POINT('',#23364);
#6181=VERTEX_POINT('',#23387);
#6182=VERTEX_POINT('',#23388);
#6183=VERTEX_POINT('',#23412);
#6184=VERTEX_POINT('',#23413);
#6185=VERTEX_POINT('',#23436);
#6186=VERTEX_POINT('',#23437);
#6187=VERTEX_POINT('',#23461);
#6188=VERTEX_POINT('',#23462);
#6189=VERTEX_POINT('',#23486);
#6190=VERTEX_POINT('',#23487);
#6191=VERTEX_POINT('',#23510);
#6192=VERTEX_POINT('',#23511);
#6193=VERTEX_POINT('',#23513);
#6194=VERTEX_POINT('',#23519);
#6195=VERTEX_POINT('',#23527);
#6196=VERTEX_POINT('',#23528);
#6197=VERTEX_POINT('',#23530);
#6198=VERTEX_POINT('',#23547);
#6199=VERTEX_POINT('',#23549);
#6200=VERTEX_POINT('',#23552);
#6201=VERTEX_POINT('',#23577);
#6202=VERTEX_POINT('',#23578);
#6203=VERTEX_POINT('',#23625);
#6204=VERTEX_POINT('',#23626);
#6205=VERTEX_POINT('',#23673);
#6206=VERTEX_POINT('',#23674);
#6207=VERTEX_POINT('',#23724);
#6208=VERTEX_POINT('',#23725);
#6209=VERTEX_POINT('',#23775);
#6210=VERTEX_POINT('',#23776);
#6211=VERTEX_POINT('',#23823);
#6212=VERTEX_POINT('',#23824);
#6213=VERTEX_POINT('',#23874);
#6214=VERTEX_POINT('',#23875);
#6215=VERTEX_POINT('',#23925);
#6216=VERTEX_POINT('',#23926);
#6217=VERTEX_POINT('',#23973);
#6218=VERTEX_POINT('',#23974);
#6219=VERTEX_POINT('',#24021);
#6220=VERTEX_POINT('',#24022);
#6221=VERTEX_POINT('',#24075);
#6222=VERTEX_POINT('',#24076);
#6223=VERTEX_POINT('',#24123);
#6224=VERTEX_POINT('',#24124);
#6225=VERTEX_POINT('',#24171);
#6226=VERTEX_POINT('',#24172);
#6227=VERTEX_POINT('',#24222);
#6228=VERTEX_POINT('',#24223);
#6229=VERTEX_POINT('',#24273);
#6230=VERTEX_POINT('',#24274);
#6231=VERTEX_POINT('',#24321);
#6232=VERTEX_POINT('',#24322);
#6233=VERTEX_POINT('',#24372);
#6234=VERTEX_POINT('',#24373);
#6235=VERTEX_POINT('',#24375);
#6236=VERTEX_POINT('',#24389);
#6237=VERTEX_POINT('',#24411);
#6238=VERTEX_POINT('',#24412);
#6239=VERTEX_POINT('',#24414);
#6240=VERTEX_POINT('',#24420);
#6241=VERTEX_POINT('',#24429);
#6242=VERTEX_POINT('',#24430);
#6243=VERTEX_POINT('',#24454);
#6244=VERTEX_POINT('',#24455);
#6245=VERTEX_POINT('',#24478);
#6246=VERTEX_POINT('',#24479);
#6247=VERTEX_POINT('',#24503);
#6248=VERTEX_POINT('',#24504);
#6249=VERTEX_POINT('',#24527);
#6250=VERTEX_POINT('',#24528);
#6251=VERTEX_POINT('',#24552);
#6252=VERTEX_POINT('',#24553);
#6253=VERTEX_POINT('',#24577);
#6254=VERTEX_POINT('',#24578);
#6255=VERTEX_POINT('',#24601);
#6256=VERTEX_POINT('',#24602);
#6257=VERTEX_POINT('',#24626);
#6258=VERTEX_POINT('',#24627);
#6259=VERTEX_POINT('',#24650);
#6260=VERTEX_POINT('',#24651);
#6261=VERTEX_POINT('',#24675);
#6262=VERTEX_POINT('',#24676);
#6263=VERTEX_POINT('',#24700);
#6264=VERTEX_POINT('',#24701);
#6265=VERTEX_POINT('',#24724);
#6266=VERTEX_POINT('',#24725);
#6267=VERTEX_POINT('',#24749);
#6268=VERTEX_POINT('',#24750);
#6269=VERTEX_POINT('',#24773);
#6270=VERTEX_POINT('',#24774);
#6271=VERTEX_POINT('',#24798);
#6272=VERTEX_POINT('',#24799);
#6273=VERTEX_POINT('',#24823);
#6274=VERTEX_POINT('',#24824);
#6275=VERTEX_POINT('',#24847);
#6276=VERTEX_POINT('',#24848);
#6277=VERTEX_POINT('',#24850);
#6278=VERTEX_POINT('',#24856);
#6279=VERTEX_POINT('',#24864);
#6280=VERTEX_POINT('',#24865);
#6281=VERTEX_POINT('',#24867);
#6282=VERTEX_POINT('',#24884);
#6283=VERTEX_POINT('',#24886);
#6284=VERTEX_POINT('',#24889);
#6285=VERTEX_POINT('',#24914);
#6286=VERTEX_POINT('',#24915);
#6287=VERTEX_POINT('',#24962);
#6288=VERTEX_POINT('',#24963);
#6289=VERTEX_POINT('',#25010);
#6290=VERTEX_POINT('',#25011);
#6291=VERTEX_POINT('',#25061);
#6292=VERTEX_POINT('',#25062);
#6293=VERTEX_POINT('',#25112);
#6294=VERTEX_POINT('',#25113);
#6295=VERTEX_POINT('',#25160);
#6296=VERTEX_POINT('',#25161);
#6297=VERTEX_POINT('',#25211);
#6298=VERTEX_POINT('',#25212);
#6299=VERTEX_POINT('',#25262);
#6300=VERTEX_POINT('',#25263);
#6301=VERTEX_POINT('',#25310);
#6302=VERTEX_POINT('',#25311);
#6303=VERTEX_POINT('',#25358);
#6304=VERTEX_POINT('',#25359);
#6305=VERTEX_POINT('',#25412);
#6306=VERTEX_POINT('',#25413);
#6307=VERTEX_POINT('',#25460);
#6308=VERTEX_POINT('',#25461);
#6309=VERTEX_POINT('',#25508);
#6310=VERTEX_POINT('',#25509);
#6311=VERTEX_POINT('',#25559);
#6312=VERTEX_POINT('',#25560);
#6313=VERTEX_POINT('',#25610);
#6314=VERTEX_POINT('',#25611);
#6315=VERTEX_POINT('',#25658);
#6316=VERTEX_POINT('',#25659);
#6317=VERTEX_POINT('',#25709);
#6318=VERTEX_POINT('',#25710);
#6319=VERTEX_POINT('',#25712);
#6320=VERTEX_POINT('',#25726);
#6321=VERTEX_POINT('',#25748);
#6322=VERTEX_POINT('',#25749);
#6323=VERTEX_POINT('',#25751);
#6324=VERTEX_POINT('',#25757);
#6325=VERTEX_POINT('',#25766);
#6326=VERTEX_POINT('',#25767);
#6327=VERTEX_POINT('',#25791);
#6328=VERTEX_POINT('',#25792);
#6329=VERTEX_POINT('',#25815);
#6330=VERTEX_POINT('',#25816);
#6331=VERTEX_POINT('',#25840);
#6332=VERTEX_POINT('',#25841);
#6333=VERTEX_POINT('',#25864);
#6334=VERTEX_POINT('',#25865);
#6335=VERTEX_POINT('',#25889);
#6336=VERTEX_POINT('',#25890);
#6337=VERTEX_POINT('',#25914);
#6338=VERTEX_POINT('',#25915);
#6339=VERTEX_POINT('',#25938);
#6340=VERTEX_POINT('',#25939);
#6341=VERTEX_POINT('',#25963);
#6342=VERTEX_POINT('',#25964);
#6343=VERTEX_POINT('',#25987);
#6344=VERTEX_POINT('',#25988);
#6345=VERTEX_POINT('',#26012);
#6346=VERTEX_POINT('',#26013);
#6347=VERTEX_POINT('',#26037);
#6348=VERTEX_POINT('',#26038);
#6349=VERTEX_POINT('',#26061);
#6350=VERTEX_POINT('',#26062);
#6351=VERTEX_POINT('',#26086);
#6352=VERTEX_POINT('',#26087);
#6353=VERTEX_POINT('',#26110);
#6354=VERTEX_POINT('',#26111);
#6355=VERTEX_POINT('',#26135);
#6356=VERTEX_POINT('',#26136);
#6357=VERTEX_POINT('',#26160);
#6358=VERTEX_POINT('',#26161);
#6359=VERTEX_POINT('',#26184);
#6360=VERTEX_POINT('',#26185);
#6361=VERTEX_POINT('',#26187);
#6362=VERTEX_POINT('',#26193);
#6363=VERTEX_POINT('',#26201);
#6364=VERTEX_POINT('',#26202);
#6365=VERTEX_POINT('',#26204);
#6366=VERTEX_POINT('',#26221);
#6367=VERTEX_POINT('',#26223);
#6368=VERTEX_POINT('',#26226);
#6369=VERTEX_POINT('',#26251);
#6370=VERTEX_POINT('',#26252);
#6371=VERTEX_POINT('',#26299);
#6372=VERTEX_POINT('',#26300);
#6373=VERTEX_POINT('',#26347);
#6374=VERTEX_POINT('',#26348);
#6375=VERTEX_POINT('',#26398);
#6376=VERTEX_POINT('',#26399);
#6377=VERTEX_POINT('',#26449);
#6378=VERTEX_POINT('',#26450);
#6379=VERTEX_POINT('',#26497);
#6380=VERTEX_POINT('',#26498);
#6381=VERTEX_POINT('',#26548);
#6382=VERTEX_POINT('',#26549);
#6383=VERTEX_POINT('',#26599);
#6384=VERTEX_POINT('',#26600);
#6385=VERTEX_POINT('',#26647);
#6386=VERTEX_POINT('',#26648);
#6387=VERTEX_POINT('',#26695);
#6388=VERTEX_POINT('',#26696);
#6389=VERTEX_POINT('',#26749);
#6390=VERTEX_POINT('',#26750);
#6391=VERTEX_POINT('',#26797);
#6392=VERTEX_POINT('',#26798);
#6393=VERTEX_POINT('',#26845);
#6394=VERTEX_POINT('',#26846);
#6395=VERTEX_POINT('',#26896);
#6396=VERTEX_POINT('',#26897);
#6397=VERTEX_POINT('',#26947);
#6398=VERTEX_POINT('',#26948);
#6399=VERTEX_POINT('',#26995);
#6400=VERTEX_POINT('',#26996);
#6401=VERTEX_POINT('',#27046);
#6402=VERTEX_POINT('',#27047);
#6403=VERTEX_POINT('',#27049);
#6404=VERTEX_POINT('',#27063);
#6405=VERTEX_POINT('',#27085);
#6406=VERTEX_POINT('',#27086);
#6407=VERTEX_POINT('',#27088);
#6408=VERTEX_POINT('',#27094);
#6409=VERTEX_POINT('',#27103);
#6410=VERTEX_POINT('',#27104);
#6411=VERTEX_POINT('',#27128);
#6412=VERTEX_POINT('',#27129);
#6413=VERTEX_POINT('',#27152);
#6414=VERTEX_POINT('',#27153);
#6415=VERTEX_POINT('',#27177);
#6416=VERTEX_POINT('',#27178);
#6417=VERTEX_POINT('',#27201);
#6418=VERTEX_POINT('',#27202);
#6419=VERTEX_POINT('',#27226);
#6420=VERTEX_POINT('',#27227);
#6421=VERTEX_POINT('',#27251);
#6422=VERTEX_POINT('',#27252);
#6423=VERTEX_POINT('',#27275);
#6424=VERTEX_POINT('',#27276);
#6425=VERTEX_POINT('',#27300);
#6426=VERTEX_POINT('',#27301);
#6427=VERTEX_POINT('',#27324);
#6428=VERTEX_POINT('',#27325);
#6429=VERTEX_POINT('',#27349);
#6430=VERTEX_POINT('',#27350);
#6431=VERTEX_POINT('',#27374);
#6432=VERTEX_POINT('',#27375);
#6433=VERTEX_POINT('',#27398);
#6434=VERTEX_POINT('',#27399);
#6435=VERTEX_POINT('',#27423);
#6436=VERTEX_POINT('',#27424);
#6437=VERTEX_POINT('',#27447);
#6438=VERTEX_POINT('',#27448);
#6439=VERTEX_POINT('',#27472);
#6440=VERTEX_POINT('',#27473);
#6441=VERTEX_POINT('',#27497);
#6442=VERTEX_POINT('',#27498);
#6443=VERTEX_POINT('',#27521);
#6444=VERTEX_POINT('',#27522);
#6445=VERTEX_POINT('',#27524);
#6446=VERTEX_POINT('',#27530);
#6447=VERTEX_POINT('',#27538);
#6448=VERTEX_POINT('',#27539);
#6449=VERTEX_POINT('',#27541);
#6450=VERTEX_POINT('',#27558);
#6451=VERTEX_POINT('',#27560);
#6452=VERTEX_POINT('',#27563);
#6453=VERTEX_POINT('',#27588);
#6454=VERTEX_POINT('',#27589);
#6455=VERTEX_POINT('',#27636);
#6456=VERTEX_POINT('',#27637);
#6457=VERTEX_POINT('',#27684);
#6458=VERTEX_POINT('',#27685);
#6459=VERTEX_POINT('',#27735);
#6460=VERTEX_POINT('',#27736);
#6461=VERTEX_POINT('',#27786);
#6462=VERTEX_POINT('',#27787);
#6463=VERTEX_POINT('',#27834);
#6464=VERTEX_POINT('',#27835);
#6465=VERTEX_POINT('',#27885);
#6466=VERTEX_POINT('',#27886);
#6467=VERTEX_POINT('',#27936);
#6468=VERTEX_POINT('',#27937);
#6469=VERTEX_POINT('',#27984);
#6470=VERTEX_POINT('',#27985);
#6471=VERTEX_POINT('',#28032);
#6472=VERTEX_POINT('',#28033);
#6473=VERTEX_POINT('',#28086);
#6474=VERTEX_POINT('',#28087);
#6475=VERTEX_POINT('',#28134);
#6476=VERTEX_POINT('',#28135);
#6477=VERTEX_POINT('',#28182);
#6478=VERTEX_POINT('',#28183);
#6479=VERTEX_POINT('',#28233);
#6480=VERTEX_POINT('',#28234);
#6481=VERTEX_POINT('',#28284);
#6482=VERTEX_POINT('',#28285);
#6483=VERTEX_POINT('',#28332);
#6484=VERTEX_POINT('',#28333);
#6485=VERTEX_POINT('',#28383);
#6486=VERTEX_POINT('',#28384);
#6487=VERTEX_POINT('',#28386);
#6488=VERTEX_POINT('',#28400);
#6489=VERTEX_POINT('',#28422);
#6490=VERTEX_POINT('',#28423);
#6491=VERTEX_POINT('',#28425);
#6492=VERTEX_POINT('',#28431);
#6493=VERTEX_POINT('',#28440);
#6494=VERTEX_POINT('',#28441);
#6495=VERTEX_POINT('',#28465);
#6496=VERTEX_POINT('',#28466);
#6497=VERTEX_POINT('',#28489);
#6498=VERTEX_POINT('',#28490);
#6499=VERTEX_POINT('',#28514);
#6500=VERTEX_POINT('',#28515);
#6501=VERTEX_POINT('',#28538);
#6502=VERTEX_POINT('',#28539);
#6503=VERTEX_POINT('',#28563);
#6504=VERTEX_POINT('',#28564);
#6505=VERTEX_POINT('',#28588);
#6506=VERTEX_POINT('',#28589);
#6507=VERTEX_POINT('',#28612);
#6508=VERTEX_POINT('',#28613);
#6509=VERTEX_POINT('',#28637);
#6510=VERTEX_POINT('',#28638);
#6511=VERTEX_POINT('',#28661);
#6512=VERTEX_POINT('',#28662);
#6513=VERTEX_POINT('',#28686);
#6514=VERTEX_POINT('',#28687);
#6515=VERTEX_POINT('',#28711);
#6516=VERTEX_POINT('',#28712);
#6517=VERTEX_POINT('',#28735);
#6518=VERTEX_POINT('',#28736);
#6519=VERTEX_POINT('',#28760);
#6520=VERTEX_POINT('',#28761);
#6521=VERTEX_POINT('',#28784);
#6522=VERTEX_POINT('',#28785);
#6523=VERTEX_POINT('',#28809);
#6524=VERTEX_POINT('',#28810);
#6525=VERTEX_POINT('',#28834);
#6526=VERTEX_POINT('',#28835);
#6527=VERTEX_POINT('',#28858);
#6528=VERTEX_POINT('',#28859);
#6529=VERTEX_POINT('',#28861);
#6530=VERTEX_POINT('',#28867);
#6531=VERTEX_POINT('',#28875);
#6532=VERTEX_POINT('',#28876);
#6533=VERTEX_POINT('',#28878);
#6534=VERTEX_POINT('',#28895);
#6535=VERTEX_POINT('',#28897);
#6536=VERTEX_POINT('',#28900);
#6537=VERTEX_POINT('',#28925);
#6538=VERTEX_POINT('',#28926);
#6539=VERTEX_POINT('',#28973);
#6540=VERTEX_POINT('',#28974);
#6541=VERTEX_POINT('',#29021);
#6542=VERTEX_POINT('',#29022);
#6543=VERTEX_POINT('',#29072);
#6544=VERTEX_POINT('',#29073);
#6545=VERTEX_POINT('',#29123);
#6546=VERTEX_POINT('',#29124);
#6547=VERTEX_POINT('',#29171);
#6548=VERTEX_POINT('',#29172);
#6549=VERTEX_POINT('',#29222);
#6550=VERTEX_POINT('',#29223);
#6551=VERTEX_POINT('',#29273);
#6552=VERTEX_POINT('',#29274);
#6553=VERTEX_POINT('',#29321);
#6554=VERTEX_POINT('',#29322);
#6555=VERTEX_POINT('',#29369);
#6556=VERTEX_POINT('',#29370);
#6557=VERTEX_POINT('',#29423);
#6558=VERTEX_POINT('',#29424);
#6559=VERTEX_POINT('',#29471);
#6560=VERTEX_POINT('',#29472);
#6561=VERTEX_POINT('',#29519);
#6562=VERTEX_POINT('',#29520);
#6563=VERTEX_POINT('',#29570);
#6564=VERTEX_POINT('',#29571);
#6565=VERTEX_POINT('',#29621);
#6566=VERTEX_POINT('',#29622);
#6567=VERTEX_POINT('',#29669);
#6568=VERTEX_POINT('',#29670);
#6569=VERTEX_POINT('',#29720);
#6570=VERTEX_POINT('',#29721);
#6571=VERTEX_POINT('',#29723);
#6572=VERTEX_POINT('',#29737);
#6573=VERTEX_POINT('',#29759);
#6574=VERTEX_POINT('',#29760);
#6575=VERTEX_POINT('',#29762);
#6576=VERTEX_POINT('',#29768);
#6577=VERTEX_POINT('',#29777);
#6578=VERTEX_POINT('',#29778);
#6579=VERTEX_POINT('',#29802);
#6580=VERTEX_POINT('',#29803);
#6581=VERTEX_POINT('',#29826);
#6582=VERTEX_POINT('',#29827);
#6583=VERTEX_POINT('',#29851);
#6584=VERTEX_POINT('',#29852);
#6585=VERTEX_POINT('',#29875);
#6586=VERTEX_POINT('',#29876);
#6587=VERTEX_POINT('',#29900);
#6588=VERTEX_POINT('',#29901);
#6589=VERTEX_POINT('',#29925);
#6590=VERTEX_POINT('',#29926);
#6591=VERTEX_POINT('',#29949);
#6592=VERTEX_POINT('',#29950);
#6593=VERTEX_POINT('',#29974);
#6594=VERTEX_POINT('',#29975);
#6595=VERTEX_POINT('',#29998);
#6596=VERTEX_POINT('',#29999);
#6597=VERTEX_POINT('',#30023);
#6598=VERTEX_POINT('',#30024);
#6599=VERTEX_POINT('',#30048);
#6600=VERTEX_POINT('',#30049);
#6601=VERTEX_POINT('',#30072);
#6602=VERTEX_POINT('',#30073);
#6603=VERTEX_POINT('',#30097);
#6604=VERTEX_POINT('',#30098);
#6605=VERTEX_POINT('',#30121);
#6606=VERTEX_POINT('',#30122);
#6607=VERTEX_POINT('',#30146);
#6608=VERTEX_POINT('',#30147);
#6609=VERTEX_POINT('',#30171);
#6610=VERTEX_POINT('',#30172);
#6611=VERTEX_POINT('',#30195);
#6612=VERTEX_POINT('',#30196);
#6613=VERTEX_POINT('',#30198);
#6614=VERTEX_POINT('',#30204);
#6615=VERTEX_POINT('',#30212);
#6616=VERTEX_POINT('',#30213);
#6617=VERTEX_POINT('',#30215);
#6618=VERTEX_POINT('',#30232);
#6619=VERTEX_POINT('',#30234);
#6620=VERTEX_POINT('',#30237);
#6621=VERTEX_POINT('',#30262);
#6622=VERTEX_POINT('',#30263);
#6623=VERTEX_POINT('',#30310);
#6624=VERTEX_POINT('',#30311);
#6625=VERTEX_POINT('',#30358);
#6626=VERTEX_POINT('',#30359);
#6627=VERTEX_POINT('',#30409);
#6628=VERTEX_POINT('',#30410);
#6629=VERTEX_POINT('',#30460);
#6630=VERTEX_POINT('',#30461);
#6631=VERTEX_POINT('',#30508);
#6632=VERTEX_POINT('',#30509);
#6633=VERTEX_POINT('',#30559);
#6634=VERTEX_POINT('',#30560);
#6635=VERTEX_POINT('',#30610);
#6636=VERTEX_POINT('',#30611);
#6637=VERTEX_POINT('',#30658);
#6638=VERTEX_POINT('',#30659);
#6639=VERTEX_POINT('',#30706);
#6640=VERTEX_POINT('',#30707);
#6641=VERTEX_POINT('',#30760);
#6642=VERTEX_POINT('',#30761);
#6643=VERTEX_POINT('',#30808);
#6644=VERTEX_POINT('',#30809);
#6645=VERTEX_POINT('',#30856);
#6646=VERTEX_POINT('',#30857);
#6647=VERTEX_POINT('',#30907);
#6648=VERTEX_POINT('',#30908);
#6649=VERTEX_POINT('',#30958);
#6650=VERTEX_POINT('',#30959);
#6651=VERTEX_POINT('',#31006);
#6652=VERTEX_POINT('',#31007);
#6653=VERTEX_POINT('',#31057);
#6654=VERTEX_POINT('',#31058);
#6655=VERTEX_POINT('',#31060);
#6656=VERTEX_POINT('',#31074);
#6657=VERTEX_POINT('',#31096);
#6658=VERTEX_POINT('',#31097);
#6659=VERTEX_POINT('',#31099);
#6660=VERTEX_POINT('',#31105);
#6661=VERTEX_POINT('',#31114);
#6662=VERTEX_POINT('',#31115);
#6663=VERTEX_POINT('',#31139);
#6664=VERTEX_POINT('',#31140);
#6665=VERTEX_POINT('',#31163);
#6666=VERTEX_POINT('',#31164);
#6667=VERTEX_POINT('',#31188);
#6668=VERTEX_POINT('',#31189);
#6669=VERTEX_POINT('',#31212);
#6670=VERTEX_POINT('',#31213);
#6671=VERTEX_POINT('',#31237);
#6672=VERTEX_POINT('',#31238);
#6673=VERTEX_POINT('',#31262);
#6674=VERTEX_POINT('',#31263);
#6675=VERTEX_POINT('',#31286);
#6676=VERTEX_POINT('',#31287);
#6677=VERTEX_POINT('',#31311);
#6678=VERTEX_POINT('',#31312);
#6679=VERTEX_POINT('',#31335);
#6680=VERTEX_POINT('',#31336);
#6681=VERTEX_POINT('',#31360);
#6682=VERTEX_POINT('',#31361);
#6683=VERTEX_POINT('',#31385);
#6684=VERTEX_POINT('',#31386);
#6685=VERTEX_POINT('',#31409);
#6686=VERTEX_POINT('',#31410);
#6687=VERTEX_POINT('',#31434);
#6688=VERTEX_POINT('',#31435);
#6689=VERTEX_POINT('',#31458);
#6690=VERTEX_POINT('',#31459);
#6691=VERTEX_POINT('',#31483);
#6692=VERTEX_POINT('',#31484);
#6693=VERTEX_POINT('',#31508);
#6694=VERTEX_POINT('',#31509);
#6695=VERTEX_POINT('',#31532);
#6696=VERTEX_POINT('',#31533);
#6697=VERTEX_POINT('',#31535);
#6698=VERTEX_POINT('',#31541);
#6699=VERTEX_POINT('',#42653);
#6700=VERTEX_POINT('',#42654);
#6701=VERTEX_POINT('',#42656);
#6702=VERTEX_POINT('',#42658);
#6703=VERTEX_POINT('',#42662);
#6704=VERTEX_POINT('',#42664);
#6705=VERTEX_POINT('',#42668);
#6706=VERTEX_POINT('',#42669);
#6707=VERTEX_POINT('',#42675);
#6708=VERTEX_POINT('',#44019);
#6709=VERTEX_POINT('',#44020);
#6710=VERTEX_POINT('',#44022);
#6711=VERTEX_POINT('',#44024);
#6712=VERTEX_POINT('',#44029);
#6713=VERTEX_POINT('',#44031);
#6714=VERTEX_POINT('',#44035);
#6715=VERTEX_POINT('',#44037);
#6716=VERTEX_POINT('',#44045);
#6717=VERTEX_POINT('',#44047);
#6718=VERTEX_POINT('',#44050);
#6719=VERTEX_POINT('',#44052);
#6720=VERTEX_POINT('',#44057);
#6721=VERTEX_POINT('',#44061);
#6722=VERTEX_POINT('',#44064);
#6723=VERTEX_POINT('',#44066);
#6724=VERTEX_POINT('',#44073);
#7574=EDGE_CURVE('',#5991,#5992,#4456,.T.);
#7575=EDGE_CURVE('',#5993,#5992,#2410,.F.);
#7576=EDGE_CURVE('',#5993,#5991,#266,.T.);
#7577=EDGE_CURVE('',#5994,#5995,#4457,.T.);
#7578=EDGE_CURVE('',#5995,#5996,#267,.T.);
#7579=EDGE_CURVE('',#5992,#5996,#2411,.F.);
#7580=EDGE_CURVE('',#5991,#5994,#268,.T.);
#7581=EDGE_CURVE('',#5997,#5998,#4458,.T.);
#7582=EDGE_CURVE('',#5998,#5995,#269,.T.);
#7583=EDGE_CURVE('',#5994,#5997,#270,.T.);
#7584=EDGE_CURVE('',#5999,#6000,#4459,.T.);
#7585=EDGE_CURVE('',#6000,#5998,#271,.T.);
#7586=EDGE_CURVE('',#5997,#5999,#272,.T.);
#7587=EDGE_CURVE('',#6001,#6002,#4460,.T.);
#7588=EDGE_CURVE('',#6002,#6000,#273,.T.);
#7589=EDGE_CURVE('',#5999,#6001,#274,.T.);
#7590=EDGE_CURVE('',#6003,#6004,#4461,.T.);
#7591=EDGE_CURVE('',#6004,#6002,#275,.T.);
#7592=EDGE_CURVE('',#6001,#6003,#276,.T.);
#7593=EDGE_CURVE('',#6005,#6006,#4462,.T.);
#7594=EDGE_CURVE('',#6005,#6007,#277,.T.);
#7595=EDGE_CURVE('',#6008,#6007,#2412,.T.);
#7596=EDGE_CURVE('',#6008,#6006,#278,.T.);
#7597=EDGE_CURVE('',#6009,#6010,#4463,.T.);
#7598=EDGE_CURVE('',#6010,#6011,#279,.T.);
#7599=EDGE_CURVE('',#6012,#6011,#2413,.T.);
#7600=EDGE_CURVE('',#6009,#6012,#280,.T.);
#7601=EDGE_CURVE('',#6013,#6014,#4464,.T.);
#7602=EDGE_CURVE('',#6014,#6010,#281,.T.);
#7603=EDGE_CURVE('',#6013,#6009,#282,.T.);
#7604=EDGE_CURVE('',#6015,#6016,#4465,.T.);
#7605=EDGE_CURVE('',#6016,#6014,#283,.T.);
#7606=EDGE_CURVE('',#6015,#6013,#284,.T.);
#7607=EDGE_CURVE('',#6017,#6018,#4466,.T.);
#7608=EDGE_CURVE('',#6018,#6016,#285,.T.);
#7609=EDGE_CURVE('',#6017,#6015,#286,.T.);
#7610=EDGE_CURVE('',#6019,#6020,#4467,.T.);
#7611=EDGE_CURVE('',#6020,#6018,#287,.T.);
#7612=EDGE_CURVE('',#6019,#6017,#288,.T.);
#7613=EDGE_CURVE('',#6021,#6022,#4468,.T.);
#7614=EDGE_CURVE('',#6022,#6020,#289,.T.);
#7615=EDGE_CURVE('',#6021,#6019,#290,.T.);
#7616=EDGE_CURVE('',#6023,#6024,#4469,.T.);
#7617=EDGE_CURVE('',#6025,#6023,#291,.T.);
#7618=EDGE_CURVE('',#6026,#6025,#2414,.T.);
#7619=EDGE_CURVE('',#6026,#6024,#292,.T.);
#7620=EDGE_CURVE('',#6027,#6028,#4470,.T.);
#7621=EDGE_CURVE('',#6028,#6029,#293,.T.);
#7622=EDGE_CURVE('',#6029,#6030,#2415,.T.);
#7623=EDGE_CURVE('',#6030,#6031,#4471,.T.);
#7624=EDGE_CURVE('',#6031,#6031,#2416,.F.);
#7625=EDGE_CURVE('',#6030,#6032,#2417,.T.);
#7626=EDGE_CURVE('',#6032,#6027,#294,.T.);
#7627=EDGE_CURVE('',#6033,#6034,#4472,.T.);
#7628=EDGE_CURVE('',#6034,#6028,#295,.T.);
#7629=EDGE_CURVE('',#6027,#6033,#296,.T.);
#7630=EDGE_CURVE('',#6035,#6036,#4473,.T.);
#7631=EDGE_CURVE('',#6036,#6034,#297,.T.);
#7632=EDGE_CURVE('',#6033,#6035,#298,.T.);
#7633=EDGE_CURVE('',#6037,#6038,#4474,.T.);
#7634=EDGE_CURVE('',#6038,#6036,#299,.T.);
#7635=EDGE_CURVE('',#6035,#6037,#300,.T.);
#7636=EDGE_CURVE('',#6039,#6040,#4475,.T.);
#7637=EDGE_CURVE('',#6040,#6038,#301,.T.);
#7638=EDGE_CURVE('',#6037,#6039,#302,.T.);
#7639=EDGE_CURVE('',#6041,#6042,#4476,.T.);
#7640=EDGE_CURVE('',#6042,#6040,#303,.T.);
#7641=EDGE_CURVE('',#6039,#6041,#304,.T.);
#7642=EDGE_CURVE('',#6043,#6044,#4477,.T.);
#7643=EDGE_CURVE('',#6044,#6042,#305,.T.);
#7644=EDGE_CURVE('',#6041,#6043,#306,.T.);
#7645=EDGE_CURVE('',#6045,#6046,#4478,.T.);
#7646=EDGE_CURVE('',#6046,#6044,#307,.T.);
#7647=EDGE_CURVE('',#6043,#6045,#308,.T.);
#7648=EDGE_CURVE('',#6047,#6048,#4479,.T.);
#7649=EDGE_CURVE('',#6048,#6046,#309,.T.);
#7650=EDGE_CURVE('',#6045,#6047,#310,.T.);
#7651=EDGE_CURVE('',#6049,#6050,#4480,.T.);
#7652=EDGE_CURVE('',#6050,#6048,#311,.T.);
#7653=EDGE_CURVE('',#6047,#6049,#312,.T.);
#7654=EDGE_CURVE('',#6051,#6052,#4481,.T.);
#7655=EDGE_CURVE('',#6052,#6050,#313,.T.);
#7656=EDGE_CURVE('',#6049,#6051,#314,.T.);
#7657=EDGE_CURVE('',#6053,#6054,#4482,.T.);
#7658=EDGE_CURVE('',#6054,#6052,#315,.T.);
#7659=EDGE_CURVE('',#6051,#6053,#316,.T.);
#7660=EDGE_CURVE('',#6055,#6056,#4483,.T.);
#7661=EDGE_CURVE('',#6056,#6054,#317,.T.);
#7662=EDGE_CURVE('',#6053,#6055,#318,.T.);
#7663=EDGE_CURVE('',#6057,#6058,#4484,.T.);
#7664=EDGE_CURVE('',#6058,#6056,#319,.T.);
#7665=EDGE_CURVE('',#6055,#6057,#320,.T.);
#7666=EDGE_CURVE('',#6059,#6060,#4485,.T.);
#7667=EDGE_CURVE('',#6060,#6058,#321,.T.);
#7668=EDGE_CURVE('',#6057,#6059,#322,.T.);
#7669=EDGE_CURVE('',#6061,#6062,#4486,.T.);
#7670=EDGE_CURVE('',#6062,#6060,#323,.T.);
#7671=EDGE_CURVE('',#6059,#6061,#324,.T.);
#7672=EDGE_CURVE('',#6063,#6064,#4487,.T.);
#7673=EDGE_CURVE('',#6064,#6062,#325,.T.);
#7674=EDGE_CURVE('',#6061,#6063,#326,.T.);
#7675=EDGE_CURVE('',#6065,#6066,#4488,.T.);
#7676=EDGE_CURVE('',#6065,#6067,#327,.T.);
#7677=EDGE_CURVE('',#6068,#6067,#2418,.F.);
#7678=EDGE_CURVE('',#6068,#6066,#328,.T.);
#7679=EDGE_CURVE('',#6069,#6070,#4489,.T.);
#7680=EDGE_CURVE('',#6070,#6071,#329,.T.);
#7681=EDGE_CURVE('',#6072,#6071,#2419,.T.);
#7682=EDGE_CURVE('',#6069,#6072,#330,.T.);
#7683=EDGE_CURVE('',#6073,#6074,#4490,.T.);
#7684=EDGE_CURVE('',#6074,#6070,#331,.T.);
#7685=EDGE_CURVE('',#6073,#6069,#332,.T.);
#7686=EDGE_CURVE('',#6075,#6076,#4491,.T.);
#7687=EDGE_CURVE('',#6076,#6074,#333,.T.);
#7688=EDGE_CURVE('',#6075,#6073,#334,.T.);
#7689=EDGE_CURVE('',#6077,#6078,#4492,.T.);
#7690=EDGE_CURVE('',#6078,#6076,#335,.T.);
#7691=EDGE_CURVE('',#6077,#6075,#336,.T.);
#7692=EDGE_CURVE('',#6079,#6080,#4493,.T.);
#7693=EDGE_CURVE('',#6080,#6078,#337,.T.);
#7694=EDGE_CURVE('',#6079,#6077,#338,.T.);
#7695=EDGE_CURVE('',#6081,#6082,#4494,.T.);
#7696=EDGE_CURVE('',#6082,#6080,#339,.T.);
#7697=EDGE_CURVE('',#6081,#6079,#340,.T.);
#7698=EDGE_CURVE('',#6083,#6084,#4495,.T.);
#7699=EDGE_CURVE('',#6084,#6082,#341,.T.);
#7700=EDGE_CURVE('',#6083,#6081,#342,.T.);
#7701=EDGE_CURVE('',#6085,#6086,#4496,.T.);
#7702=EDGE_CURVE('',#6086,#6084,#343,.T.);
#7703=EDGE_CURVE('',#6085,#6083,#344,.T.);
#7704=EDGE_CURVE('',#6087,#6088,#4497,.T.);
#7705=EDGE_CURVE('',#6088,#6086,#345,.T.);
#7706=EDGE_CURVE('',#6087,#6085,#346,.T.);
#7707=EDGE_CURVE('',#6089,#6090,#4498,.T.);
#7708=EDGE_CURVE('',#6090,#6088,#347,.T.);
#7709=EDGE_CURVE('',#6089,#6087,#348,.T.);
#7710=EDGE_CURVE('',#6091,#6092,#4499,.T.);
#7711=EDGE_CURVE('',#6092,#6090,#349,.T.);
#7712=EDGE_CURVE('',#6091,#6089,#350,.T.);
#7713=EDGE_CURVE('',#6093,#6094,#4500,.T.);
#7714=EDGE_CURVE('',#6094,#6092,#351,.T.);
#7715=EDGE_CURVE('',#6093,#6091,#352,.T.);
#7716=EDGE_CURVE('',#6095,#6096,#4501,.T.);
#7717=EDGE_CURVE('',#6096,#6094,#353,.T.);
#7718=EDGE_CURVE('',#6095,#6093,#354,.T.);
#7719=EDGE_CURVE('',#6097,#6098,#4502,.T.);
#7720=EDGE_CURVE('',#6098,#6096,#355,.T.);
#7721=EDGE_CURVE('',#6097,#6095,#356,.T.);
#7722=EDGE_CURVE('',#6099,#6100,#4503,.T.);
#7723=EDGE_CURVE('',#6100,#6098,#357,.T.);
#7724=EDGE_CURVE('',#6099,#6097,#358,.T.);
#7725=EDGE_CURVE('',#6101,#6102,#4504,.T.);
#7726=EDGE_CURVE('',#6102,#6100,#359,.T.);
#7727=EDGE_CURVE('',#6101,#6099,#360,.T.);
#7728=EDGE_CURVE('',#6103,#6104,#4505,.T.);
#7729=EDGE_CURVE('',#6104,#6102,#361,.T.);
#7730=EDGE_CURVE('',#6103,#6101,#362,.T.);
#7731=EDGE_CURVE('',#6105,#6106,#4506,.T.);
#7732=EDGE_CURVE('',#6106,#6104,#363,.T.);
#7733=EDGE_CURVE('',#6105,#6103,#364,.T.);
#7734=EDGE_CURVE('',#6107,#6108,#4507,.T.);
#7735=EDGE_CURVE('',#6109,#6107,#365,.T.);
#7736=EDGE_CURVE('',#6110,#6109,#2420,.T.);
#7737=EDGE_CURVE('',#6110,#6108,#366,.T.);
#7738=EDGE_CURVE('',#6111,#6112,#4508,.T.);
#7739=EDGE_CURVE('',#6112,#6113,#367,.T.);
#7740=EDGE_CURVE('',#6113,#6114,#2421,.T.);
#7741=EDGE_CURVE('',#6114,#6115,#4509,.T.);
#7742=EDGE_CURVE('',#6115,#6115,#2422,.F.);
#7743=EDGE_CURVE('',#6114,#6116,#2423,.T.);
#7744=EDGE_CURVE('',#6116,#6111,#368,.T.);
#7745=EDGE_CURVE('',#6117,#6118,#4510,.T.);
#7746=EDGE_CURVE('',#6118,#6112,#369,.T.);
#7747=EDGE_CURVE('',#6111,#6117,#370,.T.);
#7748=EDGE_CURVE('',#6119,#6120,#4511,.T.);
#7749=EDGE_CURVE('',#6120,#6118,#371,.T.);
#7750=EDGE_CURVE('',#6117,#6119,#372,.T.);
#7751=EDGE_CURVE('',#6121,#6122,#4512,.T.);
#7752=EDGE_CURVE('',#6122,#6120,#373,.T.);
#7753=EDGE_CURVE('',#6119,#6121,#374,.T.);
#7754=EDGE_CURVE('',#6123,#6124,#4513,.T.);
#7755=EDGE_CURVE('',#6124,#6122,#375,.T.);
#7756=EDGE_CURVE('',#6121,#6123,#376,.T.);
#7757=EDGE_CURVE('',#6125,#6126,#4514,.T.);
#7758=EDGE_CURVE('',#6126,#6124,#377,.T.);
#7759=EDGE_CURVE('',#6123,#6125,#378,.T.);
#7760=EDGE_CURVE('',#6127,#6128,#4515,.T.);
#7761=EDGE_CURVE('',#6128,#6126,#379,.T.);
#7762=EDGE_CURVE('',#6125,#6127,#380,.T.);
#7763=EDGE_CURVE('',#6129,#6130,#4516,.T.);
#7764=EDGE_CURVE('',#6130,#6128,#381,.T.);
#7765=EDGE_CURVE('',#6127,#6129,#382,.T.);
#7766=EDGE_CURVE('',#6131,#6132,#4517,.T.);
#7767=EDGE_CURVE('',#6132,#6130,#383,.T.);
#7768=EDGE_CURVE('',#6129,#6131,#384,.T.);
#7769=EDGE_CURVE('',#6133,#6134,#4518,.T.);
#7770=EDGE_CURVE('',#6134,#6132,#385,.T.);
#7771=EDGE_CURVE('',#6131,#6133,#386,.T.);
#7772=EDGE_CURVE('',#6135,#6136,#4519,.T.);
#7773=EDGE_CURVE('',#6136,#6134,#387,.T.);
#7774=EDGE_CURVE('',#6133,#6135,#388,.T.);
#7775=EDGE_CURVE('',#6137,#6138,#4520,.T.);
#7776=EDGE_CURVE('',#6138,#6136,#389,.T.);
#7777=EDGE_CURVE('',#6135,#6137,#390,.T.);
#7778=EDGE_CURVE('',#6139,#6140,#4521,.T.);
#7779=EDGE_CURVE('',#6140,#6138,#391,.T.);
#7780=EDGE_CURVE('',#6137,#6139,#392,.T.);
#7781=EDGE_CURVE('',#6141,#6142,#4522,.T.);
#7782=EDGE_CURVE('',#6142,#6140,#393,.T.);
#7783=EDGE_CURVE('',#6139,#6141,#394,.T.);
#7784=EDGE_CURVE('',#6143,#6144,#4523,.T.);
#7785=EDGE_CURVE('',#6144,#6142,#395,.T.);
#7786=EDGE_CURVE('',#6141,#6143,#396,.T.);
#7787=EDGE_CURVE('',#6145,#6146,#4524,.T.);
#7788=EDGE_CURVE('',#6146,#6144,#397,.T.);
#7789=EDGE_CURVE('',#6143,#6145,#398,.T.);
#7790=EDGE_CURVE('',#6147,#6148,#4525,.T.);
#7791=EDGE_CURVE('',#6148,#6146,#399,.T.);
#7792=EDGE_CURVE('',#6145,#6147,#400,.T.);
#7793=EDGE_CURVE('',#6149,#6150,#4526,.T.);
#7794=EDGE_CURVE('',#6149,#6151,#401,.T.);
#7795=EDGE_CURVE('',#6152,#6151,#2424,.F.);
#7796=EDGE_CURVE('',#6152,#6150,#402,.T.);
#7797=EDGE_CURVE('',#6153,#6154,#4527,.T.);
#7798=EDGE_CURVE('',#6154,#6155,#403,.T.);
#7799=EDGE_CURVE('',#6156,#6155,#2425,.T.);
#7800=EDGE_CURVE('',#6153,#6156,#404,.T.);
#7801=EDGE_CURVE('',#6157,#6158,#4528,.T.);
#7802=EDGE_CURVE('',#6158,#6154,#405,.T.);
#7803=EDGE_CURVE('',#6157,#6153,#406,.T.);
#7804=EDGE_CURVE('',#6159,#6160,#4529,.T.);
#7805=EDGE_CURVE('',#6160,#6158,#407,.T.);
#7806=EDGE_CURVE('',#6159,#6157,#408,.T.);
#7807=EDGE_CURVE('',#6161,#6162,#4530,.T.);
#7808=EDGE_CURVE('',#6162,#6160,#409,.T.);
#7809=EDGE_CURVE('',#6161,#6159,#410,.T.);
#7810=EDGE_CURVE('',#6163,#6164,#4531,.T.);
#7811=EDGE_CURVE('',#6164,#6162,#411,.T.);
#7812=EDGE_CURVE('',#6163,#6161,#412,.T.);
#7813=EDGE_CURVE('',#6165,#6166,#4532,.T.);
#7814=EDGE_CURVE('',#6166,#6164,#413,.T.);
#7815=EDGE_CURVE('',#6165,#6163,#414,.T.);
#7816=EDGE_CURVE('',#6167,#6168,#4533,.T.);
#7817=EDGE_CURVE('',#6168,#6166,#415,.T.);
#7818=EDGE_CURVE('',#6167,#6165,#416,.T.);
#7819=EDGE_CURVE('',#6169,#6170,#4534,.T.);
#7820=EDGE_CURVE('',#6170,#6168,#417,.T.);
#7821=EDGE_CURVE('',#6169,#6167,#418,.T.);
#7822=EDGE_CURVE('',#6171,#6172,#4535,.T.);
#7823=EDGE_CURVE('',#6172,#6170,#419,.T.);
#7824=EDGE_CURVE('',#6171,#6169,#420,.T.);
#7825=EDGE_CURVE('',#6173,#6174,#4536,.T.);
#7826=EDGE_CURVE('',#6174,#6172,#421,.T.);
#7827=EDGE_CURVE('',#6173,#6171,#422,.T.);
#7828=EDGE_CURVE('',#6175,#6176,#4537,.T.);
#7829=EDGE_CURVE('',#6176,#6174,#423,.T.);
#7830=EDGE_CURVE('',#6175,#6173,#424,.T.);
#7831=EDGE_CURVE('',#6177,#6178,#4538,.T.);
#7832=EDGE_CURVE('',#6178,#6176,#425,.T.);
#7833=EDGE_CURVE('',#6177,#6175,#426,.T.);
#7834=EDGE_CURVE('',#6179,#6180,#4539,.T.);
#7835=EDGE_CURVE('',#6180,#6178,#427,.T.);
#7836=EDGE_CURVE('',#6179,#6177,#428,.T.);
#7837=EDGE_CURVE('',#6181,#6182,#4540,.T.);
#7838=EDGE_CURVE('',#6182,#6180,#429,.T.);
#7839=EDGE_CURVE('',#6181,#6179,#430,.T.);
#7840=EDGE_CURVE('',#6183,#6184,#4541,.T.);
#7841=EDGE_CURVE('',#6184,#6182,#431,.T.);
#7842=EDGE_CURVE('',#6183,#6181,#432,.T.);
#7843=EDGE_CURVE('',#6185,#6186,#4542,.T.);
#7844=EDGE_CURVE('',#6186,#6184,#433,.T.);
#7845=EDGE_CURVE('',#6185,#6183,#434,.T.);
#7846=EDGE_CURVE('',#6187,#6188,#4543,.T.);
#7847=EDGE_CURVE('',#6188,#6186,#435,.T.);
#7848=EDGE_CURVE('',#6187,#6185,#436,.T.);
#7849=EDGE_CURVE('',#6189,#6190,#4544,.T.);
#7850=EDGE_CURVE('',#6190,#6188,#437,.T.);
#7851=EDGE_CURVE('',#6189,#6187,#438,.T.);
#7852=EDGE_CURVE('',#6191,#6192,#4545,.T.);
#7853=EDGE_CURVE('',#6193,#6191,#439,.T.);
#7854=EDGE_CURVE('',#6194,#6193,#2426,.T.);
#7855=EDGE_CURVE('',#6194,#6192,#440,.T.);
#7856=EDGE_CURVE('',#6195,#6196,#4546,.T.);
#7857=EDGE_CURVE('',#6196,#6197,#441,.T.);
#7858=EDGE_CURVE('',#6197,#6198,#2427,.T.);
#7859=EDGE_CURVE('',#6198,#6199,#4547,.T.);
#7860=EDGE_CURVE('',#6199,#6199,#2428,.F.);
#7861=EDGE_CURVE('',#6198,#6200,#2429,.T.);
#7862=EDGE_CURVE('',#6200,#6195,#442,.T.);
#7863=EDGE_CURVE('',#6201,#6202,#4548,.T.);
#7864=EDGE_CURVE('',#6202,#6196,#443,.T.);
#7865=EDGE_CURVE('',#6195,#6201,#444,.T.);
#7866=EDGE_CURVE('',#6203,#6204,#4549,.T.);
#7867=EDGE_CURVE('',#6204,#6202,#445,.T.);
#7868=EDGE_CURVE('',#6201,#6203,#446,.T.);
#7869=EDGE_CURVE('',#6205,#6206,#4550,.T.);
#7870=EDGE_CURVE('',#6206,#6204,#447,.T.);
#7871=EDGE_CURVE('',#6203,#6205,#448,.T.);
#7872=EDGE_CURVE('',#6207,#6208,#4551,.T.);
#7873=EDGE_CURVE('',#6208,#6206,#449,.T.);
#7874=EDGE_CURVE('',#6205,#6207,#450,.T.);
#7875=EDGE_CURVE('',#6209,#6210,#4552,.T.);
#7876=EDGE_CURVE('',#6210,#6208,#451,.T.);
#7877=EDGE_CURVE('',#6207,#6209,#452,.T.);
#7878=EDGE_CURVE('',#6211,#6212,#4553,.T.);
#7879=EDGE_CURVE('',#6212,#6210,#453,.T.);
#7880=EDGE_CURVE('',#6209,#6211,#454,.T.);
#7881=EDGE_CURVE('',#6213,#6214,#4554,.T.);
#7882=EDGE_CURVE('',#6214,#6212,#455,.T.);
#7883=EDGE_CURVE('',#6211,#6213,#456,.T.);
#7884=EDGE_CURVE('',#6215,#6216,#4555,.T.);
#7885=EDGE_CURVE('',#6216,#6214,#457,.T.);
#7886=EDGE_CURVE('',#6213,#6215,#458,.T.);
#7887=EDGE_CURVE('',#6217,#6218,#4556,.T.);
#7888=EDGE_CURVE('',#6218,#6216,#459,.T.);
#7889=EDGE_CURVE('',#6215,#6217,#460,.T.);
#7890=EDGE_CURVE('',#6219,#6220,#4557,.T.);
#7891=EDGE_CURVE('',#6220,#6218,#461,.T.);
#7892=EDGE_CURVE('',#6217,#6219,#462,.T.);
#7893=EDGE_CURVE('',#6221,#6222,#4558,.T.);
#7894=EDGE_CURVE('',#6222,#6220,#463,.T.);
#7895=EDGE_CURVE('',#6219,#6221,#464,.T.);
#7896=EDGE_CURVE('',#6223,#6224,#4559,.T.);
#7897=EDGE_CURVE('',#6224,#6222,#465,.T.);
#7898=EDGE_CURVE('',#6221,#6223,#466,.T.);
#7899=EDGE_CURVE('',#6225,#6226,#4560,.T.);
#7900=EDGE_CURVE('',#6226,#6224,#467,.T.);
#7901=EDGE_CURVE('',#6223,#6225,#468,.T.);
#7902=EDGE_CURVE('',#6227,#6228,#4561,.T.);
#7903=EDGE_CURVE('',#6228,#6226,#469,.T.);
#7904=EDGE_CURVE('',#6225,#6227,#470,.T.);
#7905=EDGE_CURVE('',#6229,#6230,#4562,.T.);
#7906=EDGE_CURVE('',#6230,#6228,#471,.T.);
#7907=EDGE_CURVE('',#6227,#6229,#472,.T.);
#7908=EDGE_CURVE('',#6231,#6232,#4563,.T.);
#7909=EDGE_CURVE('',#6232,#6230,#473,.T.);
#7910=EDGE_CURVE('',#6229,#6231,#474,.T.);
#7911=EDGE_CURVE('',#6233,#6234,#4564,.T.);
#7912=EDGE_CURVE('',#6233,#6235,#475,.T.);
#7913=EDGE_CURVE('',#6236,#6235,#2430,.F.);
#7914=EDGE_CURVE('',#6236,#6234,#476,.T.);
#7915=EDGE_CURVE('',#6237,#6238,#4565,.T.);
#7916=EDGE_CURVE('',#6238,#6239,#477,.T.);
#7917=EDGE_CURVE('',#6240,#6239,#2431,.T.);
#7918=EDGE_CURVE('',#6237,#6240,#478,.T.);
#7919=EDGE_CURVE('',#6241,#6242,#4566,.T.);
#7920=EDGE_CURVE('',#6242,#6238,#479,.T.);
#7921=EDGE_CURVE('',#6241,#6237,#480,.T.);
#7922=EDGE_CURVE('',#6243,#6244,#4567,.T.);
#7923=EDGE_CURVE('',#6244,#6242,#481,.T.);
#7924=EDGE_CURVE('',#6243,#6241,#482,.T.);
#7925=EDGE_CURVE('',#6245,#6246,#4568,.T.);
#7926=EDGE_CURVE('',#6246,#6244,#483,.T.);
#7927=EDGE_CURVE('',#6245,#6243,#484,.T.);
#7928=EDGE_CURVE('',#6247,#6248,#4569,.T.);
#7929=EDGE_CURVE('',#6248,#6246,#485,.T.);
#7930=EDGE_CURVE('',#6247,#6245,#486,.T.);
#7931=EDGE_CURVE('',#6249,#6250,#4570,.T.);
#7932=EDGE_CURVE('',#6250,#6248,#487,.T.);
#7933=EDGE_CURVE('',#6249,#6247,#488,.T.);
#7934=EDGE_CURVE('',#6251,#6252,#4571,.T.);
#7935=EDGE_CURVE('',#6252,#6250,#489,.T.);
#7936=EDGE_CURVE('',#6251,#6249,#490,.T.);
#7937=EDGE_CURVE('',#6253,#6254,#4572,.T.);
#7938=EDGE_CURVE('',#6254,#6252,#491,.T.);
#7939=EDGE_CURVE('',#6253,#6251,#492,.T.);
#7940=EDGE_CURVE('',#6255,#6256,#4573,.T.);
#7941=EDGE_CURVE('',#6256,#6254,#493,.T.);
#7942=EDGE_CURVE('',#6255,#6253,#494,.T.);
#7943=EDGE_CURVE('',#6257,#6258,#4574,.T.);
#7944=EDGE_CURVE('',#6258,#6256,#495,.T.);
#7945=EDGE_CURVE('',#6257,#6255,#496,.T.);
#7946=EDGE_CURVE('',#6259,#6260,#4575,.T.);
#7947=EDGE_CURVE('',#6260,#6258,#497,.T.);
#7948=EDGE_CURVE('',#6259,#6257,#498,.T.);
#7949=EDGE_CURVE('',#6261,#6262,#4576,.T.);
#7950=EDGE_CURVE('',#6262,#6260,#499,.T.);
#7951=EDGE_CURVE('',#6261,#6259,#500,.T.);
#7952=EDGE_CURVE('',#6263,#6264,#4577,.T.);
#7953=EDGE_CURVE('',#6264,#6262,#501,.T.);
#7954=EDGE_CURVE('',#6263,#6261,#502,.T.);
#7955=EDGE_CURVE('',#6265,#6266,#4578,.T.);
#7956=EDGE_CURVE('',#6266,#6264,#503,.T.);
#7957=EDGE_CURVE('',#6265,#6263,#504,.T.);
#7958=EDGE_CURVE('',#6267,#6268,#4579,.T.);
#7959=EDGE_CURVE('',#6268,#6266,#505,.T.);
#7960=EDGE_CURVE('',#6267,#6265,#506,.T.);
#7961=EDGE_CURVE('',#6269,#6270,#4580,.T.);
#7962=EDGE_CURVE('',#6270,#6268,#507,.T.);
#7963=EDGE_CURVE('',#6269,#6267,#508,.T.);
#7964=EDGE_CURVE('',#6271,#6272,#4581,.T.);
#7965=EDGE_CURVE('',#6272,#6270,#509,.T.);
#7966=EDGE_CURVE('',#6271,#6269,#510,.T.);
#7967=EDGE_CURVE('',#6273,#6274,#4582,.T.);
#7968=EDGE_CURVE('',#6274,#6272,#511,.T.);
#7969=EDGE_CURVE('',#6273,#6271,#512,.T.);
#7970=EDGE_CURVE('',#6275,#6276,#4583,.T.);
#7971=EDGE_CURVE('',#6277,#6275,#513,.T.);
#7972=EDGE_CURVE('',#6278,#6277,#2432,.T.);
#7973=EDGE_CURVE('',#6278,#6276,#514,.T.);
#7974=EDGE_CURVE('',#6279,#6280,#4584,.T.);
#7975=EDGE_CURVE('',#6280,#6281,#515,.T.);
#7976=EDGE_CURVE('',#6281,#6282,#2433,.T.);
#7977=EDGE_CURVE('',#6282,#6283,#4585,.T.);
#7978=EDGE_CURVE('',#6283,#6283,#2434,.F.);
#7979=EDGE_CURVE('',#6282,#6284,#2435,.T.);
#7980=EDGE_CURVE('',#6284,#6279,#516,.T.);
#7981=EDGE_CURVE('',#6285,#6286,#4586,.T.);
#7982=EDGE_CURVE('',#6286,#6280,#517,.T.);
#7983=EDGE_CURVE('',#6279,#6285,#518,.T.);
#7984=EDGE_CURVE('',#6287,#6288,#4587,.T.);
#7985=EDGE_CURVE('',#6288,#6286,#519,.T.);
#7986=EDGE_CURVE('',#6285,#6287,#520,.T.);
#7987=EDGE_CURVE('',#6289,#6290,#4588,.T.);
#7988=EDGE_CURVE('',#6290,#6288,#521,.T.);
#7989=EDGE_CURVE('',#6287,#6289,#522,.T.);
#7990=EDGE_CURVE('',#6291,#6292,#4589,.T.);
#7991=EDGE_CURVE('',#6292,#6290,#523,.T.);
#7992=EDGE_CURVE('',#6289,#6291,#524,.T.);
#7993=EDGE_CURVE('',#6293,#6294,#4590,.T.);
#7994=EDGE_CURVE('',#6294,#6292,#525,.T.);
#7995=EDGE_CURVE('',#6291,#6293,#526,.T.);
#7996=EDGE_CURVE('',#6295,#6296,#4591,.T.);
#7997=EDGE_CURVE('',#6296,#6294,#527,.T.);
#7998=EDGE_CURVE('',#6293,#6295,#528,.T.);
#7999=EDGE_CURVE('',#6297,#6298,#4592,.T.);
#8000=EDGE_CURVE('',#6298,#6296,#529,.T.);
#8001=EDGE_CURVE('',#6295,#6297,#530,.T.);
#8002=EDGE_CURVE('',#6299,#6300,#4593,.T.);
#8003=EDGE_CURVE('',#6300,#6298,#531,.T.);
#8004=EDGE_CURVE('',#6297,#6299,#532,.T.);
#8005=EDGE_CURVE('',#6301,#6302,#4594,.T.);
#8006=EDGE_CURVE('',#6302,#6300,#533,.T.);
#8007=EDGE_CURVE('',#6299,#6301,#534,.T.);
#8008=EDGE_CURVE('',#6303,#6304,#4595,.T.);
#8009=EDGE_CURVE('',#6304,#6302,#535,.T.);
#8010=EDGE_CURVE('',#6301,#6303,#536,.T.);
#8011=EDGE_CURVE('',#6305,#6306,#4596,.T.);
#8012=EDGE_CURVE('',#6306,#6304,#537,.T.);
#8013=EDGE_CURVE('',#6303,#6305,#538,.T.);
#8014=EDGE_CURVE('',#6307,#6308,#4597,.T.);
#8015=EDGE_CURVE('',#6308,#6306,#539,.T.);
#8016=EDGE_CURVE('',#6305,#6307,#540,.T.);
#8017=EDGE_CURVE('',#6309,#6310,#4598,.T.);
#8018=EDGE_CURVE('',#6310,#6308,#541,.T.);
#8019=EDGE_CURVE('',#6307,#6309,#542,.T.);
#8020=EDGE_CURVE('',#6311,#6312,#4599,.T.);
#8021=EDGE_CURVE('',#6312,#6310,#543,.T.);
#8022=EDGE_CURVE('',#6309,#6311,#544,.T.);
#8023=EDGE_CURVE('',#6313,#6314,#4600,.T.);
#8024=EDGE_CURVE('',#6314,#6312,#545,.T.);
#8025=EDGE_CURVE('',#6311,#6313,#546,.T.);
#8026=EDGE_CURVE('',#6315,#6316,#4601,.T.);
#8027=EDGE_CURVE('',#6316,#6314,#547,.T.);
#8028=EDGE_CURVE('',#6313,#6315,#548,.T.);
#8029=EDGE_CURVE('',#6317,#6318,#4602,.T.);
#8030=EDGE_CURVE('',#6317,#6319,#549,.T.);
#8031=EDGE_CURVE('',#6320,#6319,#2436,.F.);
#8032=EDGE_CURVE('',#6320,#6318,#550,.T.);
#8033=EDGE_CURVE('',#6321,#6322,#4603,.T.);
#8034=EDGE_CURVE('',#6322,#6323,#551,.T.);
#8035=EDGE_CURVE('',#6324,#6323,#2437,.T.);
#8036=EDGE_CURVE('',#6321,#6324,#552,.T.);
#8037=EDGE_CURVE('',#6325,#6326,#4604,.T.);
#8038=EDGE_CURVE('',#6326,#6322,#553,.T.);
#8039=EDGE_CURVE('',#6325,#6321,#554,.T.);
#8040=EDGE_CURVE('',#6327,#6328,#4605,.T.);
#8041=EDGE_CURVE('',#6328,#6326,#555,.T.);
#8042=EDGE_CURVE('',#6327,#6325,#556,.T.);
#8043=EDGE_CURVE('',#6329,#6330,#4606,.T.);
#8044=EDGE_CURVE('',#6330,#6328,#557,.T.);
#8045=EDGE_CURVE('',#6329,#6327,#558,.T.);
#8046=EDGE_CURVE('',#6331,#6332,#4607,.T.);
#8047=EDGE_CURVE('',#6332,#6330,#559,.T.);
#8048=EDGE_CURVE('',#6331,#6329,#560,.T.);
#8049=EDGE_CURVE('',#6333,#6334,#4608,.T.);
#8050=EDGE_CURVE('',#6334,#6332,#561,.T.);
#8051=EDGE_CURVE('',#6333,#6331,#562,.T.);
#8052=EDGE_CURVE('',#6335,#6336,#4609,.T.);
#8053=EDGE_CURVE('',#6336,#6334,#563,.T.);
#8054=EDGE_CURVE('',#6335,#6333,#564,.T.);
#8055=EDGE_CURVE('',#6337,#6338,#4610,.T.);
#8056=EDGE_CURVE('',#6338,#6336,#565,.T.);
#8057=EDGE_CURVE('',#6337,#6335,#566,.T.);
#8058=EDGE_CURVE('',#6339,#6340,#4611,.T.);
#8059=EDGE_CURVE('',#6340,#6338,#567,.T.);
#8060=EDGE_CURVE('',#6339,#6337,#568,.T.);
#8061=EDGE_CURVE('',#6341,#6342,#4612,.T.);
#8062=EDGE_CURVE('',#6342,#6340,#569,.T.);
#8063=EDGE_CURVE('',#6341,#6339,#570,.T.);
#8064=EDGE_CURVE('',#6343,#6344,#4613,.T.);
#8065=EDGE_CURVE('',#6344,#6342,#571,.T.);
#8066=EDGE_CURVE('',#6343,#6341,#572,.T.);
#8067=EDGE_CURVE('',#6345,#6346,#4614,.T.);
#8068=EDGE_CURVE('',#6346,#6344,#573,.T.);
#8069=EDGE_CURVE('',#6345,#6343,#574,.T.);
#8070=EDGE_CURVE('',#6347,#6348,#4615,.T.);
#8071=EDGE_CURVE('',#6348,#6346,#575,.T.);
#8072=EDGE_CURVE('',#6347,#6345,#576,.T.);
#8073=EDGE_CURVE('',#6349,#6350,#4616,.T.);
#8074=EDGE_CURVE('',#6350,#6348,#577,.T.);
#8075=EDGE_CURVE('',#6349,#6347,#578,.T.);
#8076=EDGE_CURVE('',#6351,#6352,#4617,.T.);
#8077=EDGE_CURVE('',#6352,#6350,#579,.T.);
#8078=EDGE_CURVE('',#6351,#6349,#580,.T.);
#8079=EDGE_CURVE('',#6353,#6354,#4618,.T.);
#8080=EDGE_CURVE('',#6354,#6352,#581,.T.);
#8081=EDGE_CURVE('',#6353,#6351,#582,.T.);
#8082=EDGE_CURVE('',#6355,#6356,#4619,.T.);
#8083=EDGE_CURVE('',#6356,#6354,#583,.T.);
#8084=EDGE_CURVE('',#6355,#6353,#584,.T.);
#8085=EDGE_CURVE('',#6357,#6358,#4620,.T.);
#8086=EDGE_CURVE('',#6358,#6356,#585,.T.);
#8087=EDGE_CURVE('',#6357,#6355,#586,.T.);
#8088=EDGE_CURVE('',#6359,#6360,#4621,.T.);
#8089=EDGE_CURVE('',#6361,#6359,#587,.T.);
#8090=EDGE_CURVE('',#6362,#6361,#2438,.T.);
#8091=EDGE_CURVE('',#6362,#6360,#588,.T.);
#8092=EDGE_CURVE('',#6363,#6364,#4622,.T.);
#8093=EDGE_CURVE('',#6364,#6365,#589,.T.);
#8094=EDGE_CURVE('',#6365,#6366,#2439,.T.);
#8095=EDGE_CURVE('',#6366,#6367,#4623,.T.);
#8096=EDGE_CURVE('',#6367,#6367,#2440,.F.);
#8097=EDGE_CURVE('',#6366,#6368,#2441,.T.);
#8098=EDGE_CURVE('',#6368,#6363,#590,.T.);
#8099=EDGE_CURVE('',#6369,#6370,#4624,.T.);
#8100=EDGE_CURVE('',#6370,#6364,#591,.T.);
#8101=EDGE_CURVE('',#6363,#6369,#592,.T.);
#8102=EDGE_CURVE('',#6371,#6372,#4625,.T.);
#8103=EDGE_CURVE('',#6372,#6370,#593,.T.);
#8104=EDGE_CURVE('',#6369,#6371,#594,.T.);
#8105=EDGE_CURVE('',#6373,#6374,#4626,.T.);
#8106=EDGE_CURVE('',#6374,#6372,#595,.T.);
#8107=EDGE_CURVE('',#6371,#6373,#596,.T.);
#8108=EDGE_CURVE('',#6375,#6376,#4627,.T.);
#8109=EDGE_CURVE('',#6376,#6374,#597,.T.);
#8110=EDGE_CURVE('',#6373,#6375,#598,.T.);
#8111=EDGE_CURVE('',#6377,#6378,#4628,.T.);
#8112=EDGE_CURVE('',#6378,#6376,#599,.T.);
#8113=EDGE_CURVE('',#6375,#6377,#600,.T.);
#8114=EDGE_CURVE('',#6379,#6380,#4629,.T.);
#8115=EDGE_CURVE('',#6380,#6378,#601,.T.);
#8116=EDGE_CURVE('',#6377,#6379,#602,.T.);
#8117=EDGE_CURVE('',#6381,#6382,#4630,.T.);
#8118=EDGE_CURVE('',#6382,#6380,#603,.T.);
#8119=EDGE_CURVE('',#6379,#6381,#604,.T.);
#8120=EDGE_CURVE('',#6383,#6384,#4631,.T.);
#8121=EDGE_CURVE('',#6384,#6382,#605,.T.);
#8122=EDGE_CURVE('',#6381,#6383,#606,.T.);
#8123=EDGE_CURVE('',#6385,#6386,#4632,.T.);
#8124=EDGE_CURVE('',#6386,#6384,#607,.T.);
#8125=EDGE_CURVE('',#6383,#6385,#608,.T.);
#8126=EDGE_CURVE('',#6387,#6388,#4633,.T.);
#8127=EDGE_CURVE('',#6388,#6386,#609,.T.);
#8128=EDGE_CURVE('',#6385,#6387,#610,.T.);
#8129=EDGE_CURVE('',#6389,#6390,#4634,.T.);
#8130=EDGE_CURVE('',#6390,#6388,#611,.T.);
#8131=EDGE_CURVE('',#6387,#6389,#612,.T.);
#8132=EDGE_CURVE('',#6391,#6392,#4635,.T.);
#8133=EDGE_CURVE('',#6392,#6390,#613,.T.);
#8134=EDGE_CURVE('',#6389,#6391,#614,.T.);
#8135=EDGE_CURVE('',#6393,#6394,#4636,.T.);
#8136=EDGE_CURVE('',#6394,#6392,#615,.T.);
#8137=EDGE_CURVE('',#6391,#6393,#616,.T.);
#8138=EDGE_CURVE('',#6395,#6396,#4637,.T.);
#8139=EDGE_CURVE('',#6396,#6394,#617,.T.);
#8140=EDGE_CURVE('',#6393,#6395,#618,.T.);
#8141=EDGE_CURVE('',#6397,#6398,#4638,.T.);
#8142=EDGE_CURVE('',#6398,#6396,#619,.T.);
#8143=EDGE_CURVE('',#6395,#6397,#620,.T.);
#8144=EDGE_CURVE('',#6399,#6400,#4639,.T.);
#8145=EDGE_CURVE('',#6400,#6398,#621,.T.);
#8146=EDGE_CURVE('',#6397,#6399,#622,.T.);
#8147=EDGE_CURVE('',#6401,#6402,#4640,.T.);
#8148=EDGE_CURVE('',#6401,#6403,#623,.T.);
#8149=EDGE_CURVE('',#6404,#6403,#2442,.T.);
#8150=EDGE_CURVE('',#6404,#6402,#624,.T.);
#8151=EDGE_CURVE('',#6405,#6406,#4641,.T.);
#8152=EDGE_CURVE('',#6406,#6407,#625,.T.);
#8153=EDGE_CURVE('',#6408,#6407,#2443,.T.);
#8154=EDGE_CURVE('',#6405,#6408,#626,.T.);
#8155=EDGE_CURVE('',#6409,#6410,#4642,.T.);
#8156=EDGE_CURVE('',#6410,#6406,#627,.T.);
#8157=EDGE_CURVE('',#6409,#6405,#628,.T.);
#8158=EDGE_CURVE('',#6411,#6412,#4643,.T.);
#8159=EDGE_CURVE('',#6412,#6410,#629,.T.);
#8160=EDGE_CURVE('',#6411,#6409,#630,.T.);
#8161=EDGE_CURVE('',#6413,#6414,#4644,.T.);
#8162=EDGE_CURVE('',#6414,#6412,#631,.T.);
#8163=EDGE_CURVE('',#6413,#6411,#632,.T.);
#8164=EDGE_CURVE('',#6415,#6416,#4645,.T.);
#8165=EDGE_CURVE('',#6416,#6414,#633,.T.);
#8166=EDGE_CURVE('',#6415,#6413,#634,.T.);
#8167=EDGE_CURVE('',#6417,#6418,#4646,.T.);
#8168=EDGE_CURVE('',#6418,#6416,#635,.T.);
#8169=EDGE_CURVE('',#6417,#6415,#636,.T.);
#8170=EDGE_CURVE('',#6419,#6420,#4647,.T.);
#8171=EDGE_CURVE('',#6420,#6418,#637,.T.);
#8172=EDGE_CURVE('',#6419,#6417,#638,.T.);
#8173=EDGE_CURVE('',#6421,#6422,#4648,.T.);
#8174=EDGE_CURVE('',#6422,#6420,#639,.T.);
#8175=EDGE_CURVE('',#6421,#6419,#640,.T.);
#8176=EDGE_CURVE('',#6423,#6424,#4649,.T.);
#8177=EDGE_CURVE('',#6424,#6422,#641,.T.);
#8178=EDGE_CURVE('',#6423,#6421,#642,.T.);
#8179=EDGE_CURVE('',#6425,#6426,#4650,.T.);
#8180=EDGE_CURVE('',#6426,#6424,#643,.T.);
#8181=EDGE_CURVE('',#6425,#6423,#644,.T.);
#8182=EDGE_CURVE('',#6427,#6428,#4651,.T.);
#8183=EDGE_CURVE('',#6428,#6426,#645,.T.);
#8184=EDGE_CURVE('',#6427,#6425,#646,.T.);
#8185=EDGE_CURVE('',#6429,#6430,#4652,.T.);
#8186=EDGE_CURVE('',#6430,#6428,#647,.T.);
#8187=EDGE_CURVE('',#6429,#6427,#648,.T.);
#8188=EDGE_CURVE('',#6431,#6432,#4653,.T.);
#8189=EDGE_CURVE('',#6432,#6430,#649,.T.);
#8190=EDGE_CURVE('',#6431,#6429,#650,.T.);
#8191=EDGE_CURVE('',#6433,#6434,#4654,.T.);
#8192=EDGE_CURVE('',#6434,#6432,#651,.T.);
#8193=EDGE_CURVE('',#6433,#6431,#652,.T.);
#8194=EDGE_CURVE('',#6435,#6436,#4655,.T.);
#8195=EDGE_CURVE('',#6436,#6434,#653,.T.);
#8196=EDGE_CURVE('',#6435,#6433,#654,.T.);
#8197=EDGE_CURVE('',#6437,#6438,#4656,.T.);
#8198=EDGE_CURVE('',#6438,#6436,#655,.T.);
#8199=EDGE_CURVE('',#6437,#6435,#656,.T.);
#8200=EDGE_CURVE('',#6439,#6440,#4657,.T.);
#8201=EDGE_CURVE('',#6440,#6438,#657,.T.);
#8202=EDGE_CURVE('',#6439,#6437,#658,.T.);
#8203=EDGE_CURVE('',#6441,#6442,#4658,.T.);
#8204=EDGE_CURVE('',#6442,#6440,#659,.T.);
#8205=EDGE_CURVE('',#6441,#6439,#660,.T.);
#8206=EDGE_CURVE('',#6443,#6444,#4659,.T.);
#8207=EDGE_CURVE('',#6445,#6443,#661,.T.);
#8208=EDGE_CURVE('',#6446,#6445,#2444,.T.);
#8209=EDGE_CURVE('',#6446,#6444,#662,.T.);
#8210=EDGE_CURVE('',#6447,#6448,#4660,.T.);
#8211=EDGE_CURVE('',#6448,#6449,#663,.T.);
#8212=EDGE_CURVE('',#6449,#6450,#2445,.T.);
#8213=EDGE_CURVE('',#6450,#6451,#4661,.T.);
#8214=EDGE_CURVE('',#6451,#6451,#2446,.F.);
#8215=EDGE_CURVE('',#6450,#6452,#2447,.T.);
#8216=EDGE_CURVE('',#6452,#6447,#664,.T.);
#8217=EDGE_CURVE('',#6453,#6454,#4662,.T.);
#8218=EDGE_CURVE('',#6454,#6448,#665,.T.);
#8219=EDGE_CURVE('',#6447,#6453,#666,.T.);
#8220=EDGE_CURVE('',#6455,#6456,#4663,.T.);
#8221=EDGE_CURVE('',#6456,#6454,#667,.T.);
#8222=EDGE_CURVE('',#6453,#6455,#668,.T.);
#8223=EDGE_CURVE('',#6457,#6458,#4664,.T.);
#8224=EDGE_CURVE('',#6458,#6456,#669,.T.);
#8225=EDGE_CURVE('',#6455,#6457,#670,.T.);
#8226=EDGE_CURVE('',#6459,#6460,#4665,.T.);
#8227=EDGE_CURVE('',#6460,#6458,#671,.T.);
#8228=EDGE_CURVE('',#6457,#6459,#672,.T.);
#8229=EDGE_CURVE('',#6461,#6462,#4666,.T.);
#8230=EDGE_CURVE('',#6462,#6460,#673,.T.);
#8231=EDGE_CURVE('',#6459,#6461,#674,.T.);
#8232=EDGE_CURVE('',#6463,#6464,#4667,.T.);
#8233=EDGE_CURVE('',#6464,#6462,#675,.T.);
#8234=EDGE_CURVE('',#6461,#6463,#676,.T.);
#8235=EDGE_CURVE('',#6465,#6466,#4668,.T.);
#8236=EDGE_CURVE('',#6466,#6464,#677,.T.);
#8237=EDGE_CURVE('',#6463,#6465,#678,.T.);
#8238=EDGE_CURVE('',#6467,#6468,#4669,.T.);
#8239=EDGE_CURVE('',#6468,#6466,#679,.T.);
#8240=EDGE_CURVE('',#6465,#6467,#680,.T.);
#8241=EDGE_CURVE('',#6469,#6470,#4670,.T.);
#8242=EDGE_CURVE('',#6470,#6468,#681,.T.);
#8243=EDGE_CURVE('',#6467,#6469,#682,.T.);
#8244=EDGE_CURVE('',#6471,#6472,#4671,.T.);
#8245=EDGE_CURVE('',#6472,#6470,#683,.T.);
#8246=EDGE_CURVE('',#6469,#6471,#684,.T.);
#8247=EDGE_CURVE('',#6473,#6474,#4672,.T.);
#8248=EDGE_CURVE('',#6474,#6472,#685,.T.);
#8249=EDGE_CURVE('',#6471,#6473,#686,.T.);
#8250=EDGE_CURVE('',#6475,#6476,#4673,.T.);
#8251=EDGE_CURVE('',#6476,#6474,#687,.T.);
#8252=EDGE_CURVE('',#6473,#6475,#688,.T.);
#8253=EDGE_CURVE('',#6477,#6478,#4674,.T.);
#8254=EDGE_CURVE('',#6478,#6476,#689,.T.);
#8255=EDGE_CURVE('',#6475,#6477,#690,.T.);
#8256=EDGE_CURVE('',#6479,#6480,#4675,.T.);
#8257=EDGE_CURVE('',#6480,#6478,#691,.T.);
#8258=EDGE_CURVE('',#6477,#6479,#692,.T.);
#8259=EDGE_CURVE('',#6481,#6482,#4676,.T.);
#8260=EDGE_CURVE('',#6482,#6480,#693,.T.);
#8261=EDGE_CURVE('',#6479,#6481,#694,.T.);
#8262=EDGE_CURVE('',#6483,#6484,#4677,.T.);
#8263=EDGE_CURVE('',#6484,#6482,#695,.T.);
#8264=EDGE_CURVE('',#6481,#6483,#696,.T.);
#8265=EDGE_CURVE('',#6485,#6486,#4678,.T.);
#8266=EDGE_CURVE('',#6485,#6487,#697,.T.);
#8267=EDGE_CURVE('',#6488,#6487,#2448,.T.);
#8268=EDGE_CURVE('',#6488,#6486,#698,.T.);
#8269=EDGE_CURVE('',#6489,#6490,#4679,.T.);
#8270=EDGE_CURVE('',#6490,#6491,#699,.T.);
#8271=EDGE_CURVE('',#6492,#6491,#2449,.T.);
#8272=EDGE_CURVE('',#6489,#6492,#700,.T.);
#8273=EDGE_CURVE('',#6493,#6494,#4680,.T.);
#8274=EDGE_CURVE('',#6494,#6490,#701,.T.);
#8275=EDGE_CURVE('',#6493,#6489,#702,.T.);
#8276=EDGE_CURVE('',#6495,#6496,#4681,.T.);
#8277=EDGE_CURVE('',#6496,#6494,#703,.T.);
#8278=EDGE_CURVE('',#6495,#6493,#704,.T.);
#8279=EDGE_CURVE('',#6497,#6498,#4682,.T.);
#8280=EDGE_CURVE('',#6498,#6496,#705,.T.);
#8281=EDGE_CURVE('',#6497,#6495,#706,.T.);
#8282=EDGE_CURVE('',#6499,#6500,#4683,.T.);
#8283=EDGE_CURVE('',#6500,#6498,#707,.T.);
#8284=EDGE_CURVE('',#6499,#6497,#708,.T.);
#8285=EDGE_CURVE('',#6501,#6502,#4684,.T.);
#8286=EDGE_CURVE('',#6502,#6500,#709,.T.);
#8287=EDGE_CURVE('',#6501,#6499,#710,.T.);
#8288=EDGE_CURVE('',#6503,#6504,#4685,.T.);
#8289=EDGE_CURVE('',#6504,#6502,#711,.T.);
#8290=EDGE_CURVE('',#6503,#6501,#712,.T.);
#8291=EDGE_CURVE('',#6505,#6506,#4686,.T.);
#8292=EDGE_CURVE('',#6506,#6504,#713,.T.);
#8293=EDGE_CURVE('',#6505,#6503,#714,.T.);
#8294=EDGE_CURVE('',#6507,#6508,#4687,.T.);
#8295=EDGE_CURVE('',#6508,#6506,#715,.T.);
#8296=EDGE_CURVE('',#6507,#6505,#716,.T.);
#8297=EDGE_CURVE('',#6509,#6510,#4688,.T.);
#8298=EDGE_CURVE('',#6510,#6508,#717,.T.);
#8299=EDGE_CURVE('',#6509,#6507,#718,.T.);
#8300=EDGE_CURVE('',#6511,#6512,#4689,.T.);
#8301=EDGE_CURVE('',#6512,#6510,#719,.T.);
#8302=EDGE_CURVE('',#6511,#6509,#720,.T.);
#8303=EDGE_CURVE('',#6513,#6514,#4690,.T.);
#8304=EDGE_CURVE('',#6514,#6512,#721,.T.);
#8305=EDGE_CURVE('',#6513,#6511,#722,.T.);
#8306=EDGE_CURVE('',#6515,#6516,#4691,.T.);
#8307=EDGE_CURVE('',#6516,#6514,#723,.T.);
#8308=EDGE_CURVE('',#6515,#6513,#724,.T.);
#8309=EDGE_CURVE('',#6517,#6518,#4692,.T.);
#8310=EDGE_CURVE('',#6518,#6516,#725,.T.);
#8311=EDGE_CURVE('',#6517,#6515,#726,.T.);
#8312=EDGE_CURVE('',#6519,#6520,#4693,.T.);
#8313=EDGE_CURVE('',#6520,#6518,#727,.T.);
#8314=EDGE_CURVE('',#6519,#6517,#728,.T.);
#8315=EDGE_CURVE('',#6521,#6522,#4694,.T.);
#8316=EDGE_CURVE('',#6522,#6520,#729,.T.);
#8317=EDGE_CURVE('',#6521,#6519,#730,.T.);
#8318=EDGE_CURVE('',#6523,#6524,#4695,.T.);
#8319=EDGE_CURVE('',#6524,#6522,#731,.T.);
#8320=EDGE_CURVE('',#6523,#6521,#732,.T.);
#8321=EDGE_CURVE('',#6525,#6526,#4696,.T.);
#8322=EDGE_CURVE('',#6526,#6524,#733,.T.);
#8323=EDGE_CURVE('',#6525,#6523,#734,.T.);
#8324=EDGE_CURVE('',#6527,#6528,#4697,.T.);
#8325=EDGE_CURVE('',#6529,#6527,#735,.T.);
#8326=EDGE_CURVE('',#6530,#6529,#2450,.T.);
#8327=EDGE_CURVE('',#6530,#6528,#736,.T.);
#8328=EDGE_CURVE('',#6531,#6532,#4698,.T.);
#8329=EDGE_CURVE('',#6532,#6533,#737,.T.);
#8330=EDGE_CURVE('',#6533,#6534,#2451,.T.);
#8331=EDGE_CURVE('',#6534,#6535,#4699,.T.);
#8332=EDGE_CURVE('',#6535,#6535,#2452,.F.);
#8333=EDGE_CURVE('',#6534,#6536,#2453,.T.);
#8334=EDGE_CURVE('',#6536,#6531,#738,.T.);
#8335=EDGE_CURVE('',#6537,#6538,#4700,.T.);
#8336=EDGE_CURVE('',#6538,#6532,#739,.T.);
#8337=EDGE_CURVE('',#6531,#6537,#740,.T.);
#8338=EDGE_CURVE('',#6539,#6540,#4701,.T.);
#8339=EDGE_CURVE('',#6540,#6538,#741,.T.);
#8340=EDGE_CURVE('',#6537,#6539,#742,.T.);
#8341=EDGE_CURVE('',#6541,#6542,#4702,.T.);
#8342=EDGE_CURVE('',#6542,#6540,#743,.T.);
#8343=EDGE_CURVE('',#6539,#6541,#744,.T.);
#8344=EDGE_CURVE('',#6543,#6544,#4703,.T.);
#8345=EDGE_CURVE('',#6544,#6542,#745,.T.);
#8346=EDGE_CURVE('',#6541,#6543,#746,.T.);
#8347=EDGE_CURVE('',#6545,#6546,#4704,.T.);
#8348=EDGE_CURVE('',#6546,#6544,#747,.T.);
#8349=EDGE_CURVE('',#6543,#6545,#748,.T.);
#8350=EDGE_CURVE('',#6547,#6548,#4705,.T.);
#8351=EDGE_CURVE('',#6548,#6546,#749,.T.);
#8352=EDGE_CURVE('',#6545,#6547,#750,.T.);
#8353=EDGE_CURVE('',#6549,#6550,#4706,.T.);
#8354=EDGE_CURVE('',#6550,#6548,#751,.T.);
#8355=EDGE_CURVE('',#6547,#6549,#752,.T.);
#8356=EDGE_CURVE('',#6551,#6552,#4707,.T.);
#8357=EDGE_CURVE('',#6552,#6550,#753,.T.);
#8358=EDGE_CURVE('',#6549,#6551,#754,.T.);
#8359=EDGE_CURVE('',#6553,#6554,#4708,.T.);
#8360=EDGE_CURVE('',#6554,#6552,#755,.T.);
#8361=EDGE_CURVE('',#6551,#6553,#756,.T.);
#8362=EDGE_CURVE('',#6555,#6556,#4709,.T.);
#8363=EDGE_CURVE('',#6556,#6554,#757,.T.);
#8364=EDGE_CURVE('',#6553,#6555,#758,.T.);
#8365=EDGE_CURVE('',#6557,#6558,#4710,.T.);
#8366=EDGE_CURVE('',#6558,#6556,#759,.T.);
#8367=EDGE_CURVE('',#6555,#6557,#760,.T.);
#8368=EDGE_CURVE('',#6559,#6560,#4711,.T.);
#8369=EDGE_CURVE('',#6560,#6558,#761,.T.);
#8370=EDGE_CURVE('',#6557,#6559,#762,.T.);
#8371=EDGE_CURVE('',#6561,#6562,#4712,.T.);
#8372=EDGE_CURVE('',#6562,#6560,#763,.T.);
#8373=EDGE_CURVE('',#6559,#6561,#764,.T.);
#8374=EDGE_CURVE('',#6563,#6564,#4713,.T.);
#8375=EDGE_CURVE('',#6564,#6562,#765,.T.);
#8376=EDGE_CURVE('',#6561,#6563,#766,.T.);
#8377=EDGE_CURVE('',#6565,#6566,#4714,.T.);
#8378=EDGE_CURVE('',#6566,#6564,#767,.T.);
#8379=EDGE_CURVE('',#6563,#6565,#768,.T.);
#8380=EDGE_CURVE('',#6567,#6568,#4715,.T.);
#8381=EDGE_CURVE('',#6568,#6566,#769,.T.);
#8382=EDGE_CURVE('',#6565,#6567,#770,.T.);
#8383=EDGE_CURVE('',#6569,#6570,#4716,.T.);
#8384=EDGE_CURVE('',#6569,#6571,#771,.T.);
#8385=EDGE_CURVE('',#6572,#6571,#2454,.T.);
#8386=EDGE_CURVE('',#6572,#6570,#772,.T.);
#8387=EDGE_CURVE('',#6573,#6574,#4717,.T.);
#8388=EDGE_CURVE('',#6574,#6575,#773,.T.);
#8389=EDGE_CURVE('',#6576,#6575,#2455,.T.);
#8390=EDGE_CURVE('',#6573,#6576,#774,.T.);
#8391=EDGE_CURVE('',#6577,#6578,#4718,.T.);
#8392=EDGE_CURVE('',#6578,#6574,#775,.T.);
#8393=EDGE_CURVE('',#6577,#6573,#776,.T.);
#8394=EDGE_CURVE('',#6579,#6580,#4719,.T.);
#8395=EDGE_CURVE('',#6580,#6578,#777,.T.);
#8396=EDGE_CURVE('',#6579,#6577,#778,.T.);
#8397=EDGE_CURVE('',#6581,#6582,#4720,.T.);
#8398=EDGE_CURVE('',#6582,#6580,#779,.T.);
#8399=EDGE_CURVE('',#6581,#6579,#780,.T.);
#8400=EDGE_CURVE('',#6583,#6584,#4721,.T.);
#8401=EDGE_CURVE('',#6584,#6582,#781,.T.);
#8402=EDGE_CURVE('',#6583,#6581,#782,.T.);
#8403=EDGE_CURVE('',#6585,#6586,#4722,.T.);
#8404=EDGE_CURVE('',#6586,#6584,#783,.T.);
#8405=EDGE_CURVE('',#6585,#6583,#784,.T.);
#8406=EDGE_CURVE('',#6587,#6588,#4723,.T.);
#8407=EDGE_CURVE('',#6588,#6586,#785,.T.);
#8408=EDGE_CURVE('',#6587,#6585,#786,.T.);
#8409=EDGE_CURVE('',#6589,#6590,#4724,.T.);
#8410=EDGE_CURVE('',#6590,#6588,#787,.T.);
#8411=EDGE_CURVE('',#6589,#6587,#788,.T.);
#8412=EDGE_CURVE('',#6591,#6592,#4725,.T.);
#8413=EDGE_CURVE('',#6592,#6590,#789,.T.);
#8414=EDGE_CURVE('',#6591,#6589,#790,.T.);
#8415=EDGE_CURVE('',#6593,#6594,#4726,.T.);
#8416=EDGE_CURVE('',#6594,#6592,#791,.T.);
#8417=EDGE_CURVE('',#6593,#6591,#792,.T.);
#8418=EDGE_CURVE('',#6595,#6596,#4727,.T.);
#8419=EDGE_CURVE('',#6596,#6594,#793,.T.);
#8420=EDGE_CURVE('',#6595,#6593,#794,.T.);
#8421=EDGE_CURVE('',#6597,#6598,#4728,.T.);
#8422=EDGE_CURVE('',#6598,#6596,#795,.T.);
#8423=EDGE_CURVE('',#6597,#6595,#796,.T.);
#8424=EDGE_CURVE('',#6599,#6600,#4729,.T.);
#8425=EDGE_CURVE('',#6600,#6598,#797,.T.);
#8426=EDGE_CURVE('',#6599,#6597,#798,.T.);
#8427=EDGE_CURVE('',#6601,#6602,#4730,.T.);
#8428=EDGE_CURVE('',#6602,#6600,#799,.T.);
#8429=EDGE_CURVE('',#6601,#6599,#800,.T.);
#8430=EDGE_CURVE('',#6603,#6604,#4731,.T.);
#8431=EDGE_CURVE('',#6604,#6602,#801,.T.);
#8432=EDGE_CURVE('',#6603,#6601,#802,.T.);
#8433=EDGE_CURVE('',#6605,#6606,#4732,.T.);
#8434=EDGE_CURVE('',#6606,#6604,#803,.T.);
#8435=EDGE_CURVE('',#6605,#6603,#804,.T.);
#8436=EDGE_CURVE('',#6607,#6608,#4733,.T.);
#8437=EDGE_CURVE('',#6608,#6606,#805,.T.);
#8438=EDGE_CURVE('',#6607,#6605,#806,.T.);
#8439=EDGE_CURVE('',#6609,#6610,#4734,.T.);
#8440=EDGE_CURVE('',#6610,#6608,#807,.T.);
#8441=EDGE_CURVE('',#6609,#6607,#808,.T.);
#8442=EDGE_CURVE('',#6611,#6612,#4735,.T.);
#8443=EDGE_CURVE('',#6613,#6611,#809,.T.);
#8444=EDGE_CURVE('',#6614,#6613,#2456,.T.);
#8445=EDGE_CURVE('',#6614,#6612,#810,.T.);
#8446=EDGE_CURVE('',#6615,#6616,#4736,.T.);
#8447=EDGE_CURVE('',#6616,#6617,#811,.T.);
#8448=EDGE_CURVE('',#6617,#6618,#2457,.T.);
#8449=EDGE_CURVE('',#6618,#6619,#4737,.T.);
#8450=EDGE_CURVE('',#6619,#6619,#2458,.F.);
#8451=EDGE_CURVE('',#6618,#6620,#2459,.T.);
#8452=EDGE_CURVE('',#6620,#6615,#812,.T.);
#8453=EDGE_CURVE('',#6621,#6622,#4738,.T.);
#8454=EDGE_CURVE('',#6622,#6616,#813,.T.);
#8455=EDGE_CURVE('',#6615,#6621,#814,.T.);
#8456=EDGE_CURVE('',#6623,#6624,#4739,.T.);
#8457=EDGE_CURVE('',#6624,#6622,#815,.T.);
#8458=EDGE_CURVE('',#6621,#6623,#816,.T.);
#8459=EDGE_CURVE('',#6625,#6626,#4740,.T.);
#8460=EDGE_CURVE('',#6626,#6624,#817,.T.);
#8461=EDGE_CURVE('',#6623,#6625,#818,.T.);
#8462=EDGE_CURVE('',#6627,#6628,#4741,.T.);
#8463=EDGE_CURVE('',#6628,#6626,#819,.T.);
#8464=EDGE_CURVE('',#6625,#6627,#820,.T.);
#8465=EDGE_CURVE('',#6629,#6630,#4742,.T.);
#8466=EDGE_CURVE('',#6630,#6628,#821,.T.);
#8467=EDGE_CURVE('',#6627,#6629,#822,.T.);
#8468=EDGE_CURVE('',#6631,#6632,#4743,.T.);
#8469=EDGE_CURVE('',#6632,#6630,#823,.T.);
#8470=EDGE_CURVE('',#6629,#6631,#824,.T.);
#8471=EDGE_CURVE('',#6633,#6634,#4744,.T.);
#8472=EDGE_CURVE('',#6634,#6632,#825,.T.);
#8473=EDGE_CURVE('',#6631,#6633,#826,.T.);
#8474=EDGE_CURVE('',#6635,#6636,#4745,.T.);
#8475=EDGE_CURVE('',#6636,#6634,#827,.T.);
#8476=EDGE_CURVE('',#6633,#6635,#828,.T.);
#8477=EDGE_CURVE('',#6637,#6638,#4746,.T.);
#8478=EDGE_CURVE('',#6638,#6636,#829,.T.);
#8479=EDGE_CURVE('',#6635,#6637,#830,.T.);
#8480=EDGE_CURVE('',#6639,#6640,#4747,.T.);
#8481=EDGE_CURVE('',#6640,#6638,#831,.T.);
#8482=EDGE_CURVE('',#6637,#6639,#832,.T.);
#8483=EDGE_CURVE('',#6641,#6642,#4748,.T.);
#8484=EDGE_CURVE('',#6642,#6640,#833,.T.);
#8485=EDGE_CURVE('',#6639,#6641,#834,.T.);
#8486=EDGE_CURVE('',#6643,#6644,#4749,.T.);
#8487=EDGE_CURVE('',#6644,#6642,#835,.T.);
#8488=EDGE_CURVE('',#6641,#6643,#836,.T.);
#8489=EDGE_CURVE('',#6645,#6646,#4750,.T.);
#8490=EDGE_CURVE('',#6646,#6644,#837,.T.);
#8491=EDGE_CURVE('',#6643,#6645,#838,.T.);
#8492=EDGE_CURVE('',#6647,#6648,#4751,.T.);
#8493=EDGE_CURVE('',#6648,#6646,#839,.T.);
#8494=EDGE_CURVE('',#6645,#6647,#840,.T.);
#8495=EDGE_CURVE('',#6649,#6650,#4752,.T.);
#8496=EDGE_CURVE('',#6650,#6648,#841,.T.);
#8497=EDGE_CURVE('',#6647,#6649,#842,.T.);
#8498=EDGE_CURVE('',#6651,#6652,#4753,.T.);
#8499=EDGE_CURVE('',#6652,#6650,#843,.T.);
#8500=EDGE_CURVE('',#6649,#6651,#844,.T.);
#8501=EDGE_CURVE('',#6653,#6654,#4754,.T.);
#8502=EDGE_CURVE('',#6653,#6655,#845,.T.);
#8503=EDGE_CURVE('',#6656,#6655,#2460,.T.);
#8504=EDGE_CURVE('',#6656,#6654,#846,.T.);
#8505=EDGE_CURVE('',#6657,#6658,#4755,.T.);
#8506=EDGE_CURVE('',#6658,#6659,#847,.T.);
#8507=EDGE_CURVE('',#6660,#6659,#2461,.T.);
#8508=EDGE_CURVE('',#6657,#6660,#848,.T.);
#8509=EDGE_CURVE('',#6661,#6662,#4756,.T.);
#8510=EDGE_CURVE('',#6662,#6658,#849,.T.);
#8511=EDGE_CURVE('',#6661,#6657,#850,.T.);
#8512=EDGE_CURVE('',#6663,#6664,#4757,.T.);
#8513=EDGE_CURVE('',#6664,#6662,#851,.T.);
#8514=EDGE_CURVE('',#6663,#6661,#852,.T.);
#8515=EDGE_CURVE('',#6665,#6666,#4758,.T.);
#8516=EDGE_CURVE('',#6666,#6664,#853,.T.);
#8517=EDGE_CURVE('',#6665,#6663,#854,.T.);
#8518=EDGE_CURVE('',#6667,#6668,#4759,.T.);
#8519=EDGE_CURVE('',#6668,#6666,#855,.T.);
#8520=EDGE_CURVE('',#6667,#6665,#856,.T.);
#8521=EDGE_CURVE('',#6669,#6670,#4760,.T.);
#8522=EDGE_CURVE('',#6670,#6668,#857,.T.);
#8523=EDGE_CURVE('',#6669,#6667,#858,.T.);
#8524=EDGE_CURVE('',#6671,#6672,#4761,.T.);
#8525=EDGE_CURVE('',#6672,#6670,#859,.T.);
#8526=EDGE_CURVE('',#6671,#6669,#860,.T.);
#8527=EDGE_CURVE('',#6673,#6674,#4762,.T.);
#8528=EDGE_CURVE('',#6674,#6672,#861,.T.);
#8529=EDGE_CURVE('',#6673,#6671,#862,.T.);
#8530=EDGE_CURVE('',#6675,#6676,#4763,.T.);
#8531=EDGE_CURVE('',#6676,#6674,#863,.T.);
#8532=EDGE_CURVE('',#6675,#6673,#864,.T.);
#8533=EDGE_CURVE('',#6677,#6678,#4764,.T.);
#8534=EDGE_CURVE('',#6678,#6676,#865,.T.);
#8535=EDGE_CURVE('',#6677,#6675,#866,.T.);
#8536=EDGE_CURVE('',#6679,#6680,#4765,.T.);
#8537=EDGE_CURVE('',#6680,#6678,#867,.T.);
#8538=EDGE_CURVE('',#6679,#6677,#868,.T.);
#8539=EDGE_CURVE('',#6681,#6682,#4766,.T.);
#8540=EDGE_CURVE('',#6682,#6680,#869,.T.);
#8541=EDGE_CURVE('',#6681,#6679,#870,.T.);
#8542=EDGE_CURVE('',#6683,#6684,#4767,.T.);
#8543=EDGE_CURVE('',#6684,#6682,#871,.T.);
#8544=EDGE_CURVE('',#6683,#6681,#872,.T.);
#8545=EDGE_CURVE('',#6685,#6686,#4768,.T.);
#8546=EDGE_CURVE('',#6686,#6684,#873,.T.);
#8547=EDGE_CURVE('',#6685,#6683,#874,.T.);
#8548=EDGE_CURVE('',#6687,#6688,#4769,.T.);
#8549=EDGE_CURVE('',#6688,#6686,#875,.T.);
#8550=EDGE_CURVE('',#6687,#6685,#876,.T.);
#8551=EDGE_CURVE('',#6689,#6690,#4770,.T.);
#8552=EDGE_CURVE('',#6690,#6688,#877,.T.);
#8553=EDGE_CURVE('',#6689,#6687,#878,.T.);
#8554=EDGE_CURVE('',#6691,#6692,#4771,.T.);
#8555=EDGE_CURVE('',#6692,#6690,#879,.T.);
#8556=EDGE_CURVE('',#6691,#6689,#880,.T.);
#8557=EDGE_CURVE('',#6693,#6694,#4772,.T.);
#8558=EDGE_CURVE('',#6694,#6692,#881,.T.);
#8559=EDGE_CURVE('',#6693,#6691,#882,.T.);
#8560=EDGE_CURVE('',#6695,#6696,#4773,.T.);
#8561=EDGE_CURVE('',#6697,#6695,#883,.T.);
#8562=EDGE_CURVE('',#6698,#6697,#2462,.T.);
#8563=EDGE_CURVE('',#6698,#6696,#884,.T.);
#8564=EDGE_CURVE('',#6617,#6660,#885,.T.);
#8565=EDGE_CURVE('',#6659,#6620,#886,.T.);
#8566=EDGE_CURVE('',#6696,#6694,#887,.T.);
#8567=EDGE_CURVE('',#6695,#6693,#888,.T.);
#8568=EDGE_CURVE('',#6655,#6698,#889,.T.);
#8569=EDGE_CURVE('',#6651,#6653,#890,.T.);
#8570=EDGE_CURVE('',#6654,#6652,#891,.T.);
#8571=EDGE_CURVE('',#6697,#6656,#892,.T.);
#8572=EDGE_CURVE('',#6533,#6576,#893,.T.);
#8573=EDGE_CURVE('',#6575,#6536,#894,.T.);
#8574=EDGE_CURVE('',#6612,#6610,#895,.T.);
#8575=EDGE_CURVE('',#6611,#6609,#896,.T.);
#8576=EDGE_CURVE('',#6571,#6614,#897,.T.);
#8577=EDGE_CURVE('',#6567,#6569,#898,.T.);
#8578=EDGE_CURVE('',#6570,#6568,#899,.T.);
#8579=EDGE_CURVE('',#6613,#6572,#900,.T.);
#8580=EDGE_CURVE('',#6449,#6492,#901,.T.);
#8581=EDGE_CURVE('',#6491,#6452,#902,.T.);
#8582=EDGE_CURVE('',#6528,#6526,#903,.T.);
#8583=EDGE_CURVE('',#6527,#6525,#904,.T.);
#8584=EDGE_CURVE('',#6487,#6530,#905,.T.);
#8585=EDGE_CURVE('',#6483,#6485,#906,.T.);
#8586=EDGE_CURVE('',#6486,#6484,#907,.T.);
#8587=EDGE_CURVE('',#6529,#6488,#908,.T.);
#8588=EDGE_CURVE('',#6365,#6408,#909,.T.);
#8589=EDGE_CURVE('',#6407,#6368,#910,.T.);
#8590=EDGE_CURVE('',#6444,#6442,#911,.T.);
#8591=EDGE_CURVE('',#6443,#6441,#912,.T.);
#8592=EDGE_CURVE('',#6403,#6446,#913,.T.);
#8593=EDGE_CURVE('',#6399,#6401,#914,.T.);
#8594=EDGE_CURVE('',#6402,#6400,#915,.T.);
#8595=EDGE_CURVE('',#6445,#6404,#916,.T.);
#8596=EDGE_CURVE('',#6281,#6324,#917,.T.);
#8597=EDGE_CURVE('',#6323,#6284,#918,.T.);
#8598=EDGE_CURVE('',#6360,#6358,#919,.T.);
#8599=EDGE_CURVE('',#6359,#6357,#920,.T.);
#8600=EDGE_CURVE('',#6319,#6362,#921,.T.);
#8601=EDGE_CURVE('',#6315,#6317,#922,.T.);
#8602=EDGE_CURVE('',#6318,#6316,#923,.T.);
#8603=EDGE_CURVE('',#6361,#6320,#924,.T.);
#8604=EDGE_CURVE('',#6197,#6240,#925,.T.);
#8605=EDGE_CURVE('',#6239,#6200,#926,.T.);
#8606=EDGE_CURVE('',#6276,#6274,#927,.T.);
#8607=EDGE_CURVE('',#6275,#6273,#928,.T.);
#8608=EDGE_CURVE('',#6235,#6278,#929,.T.);
#8609=EDGE_CURVE('',#6231,#6233,#930,.T.);
#8610=EDGE_CURVE('',#6234,#6232,#931,.T.);
#8611=EDGE_CURVE('',#6277,#6236,#932,.T.);
#8612=EDGE_CURVE('',#6113,#6156,#933,.T.);
#8613=EDGE_CURVE('',#6155,#6116,#934,.T.);
#8614=EDGE_CURVE('',#6192,#6190,#935,.T.);
#8615=EDGE_CURVE('',#6191,#6189,#936,.T.);
#8616=EDGE_CURVE('',#6151,#6194,#937,.T.);
#8617=EDGE_CURVE('',#6147,#6149,#938,.T.);
#8618=EDGE_CURVE('',#6150,#6148,#939,.T.);
#8619=EDGE_CURVE('',#6193,#6152,#940,.T.);
#8620=EDGE_CURVE('',#6029,#6072,#941,.T.);
#8621=EDGE_CURVE('',#6071,#6032,#942,.T.);
#8622=EDGE_CURVE('',#6108,#6106,#943,.T.);
#8623=EDGE_CURVE('',#6107,#6105,#944,.T.);
#8624=EDGE_CURVE('',#6067,#6110,#945,.T.);
#8625=EDGE_CURVE('',#6063,#6065,#946,.T.);
#8626=EDGE_CURVE('',#6066,#6064,#947,.T.);
#8627=EDGE_CURVE('',#6109,#6068,#948,.T.);
#8628=EDGE_CURVE('',#6699,#6700,#4774,.T.);
#8629=EDGE_CURVE('',#6701,#6699,#4775,.T.);
#8630=EDGE_CURVE('',#6701,#6702,#4776,.T.);
#8631=EDGE_CURVE('',#6700,#6702,#4777,.T.);
#8632=EDGE_CURVE('',#6703,#6701,#4778,.T.);
#8633=EDGE_CURVE('',#6703,#6704,#4779,.T.);
#8634=EDGE_CURVE('',#6702,#6704,#4780,.T.);
#8635=EDGE_CURVE('',#6705,#6706,#4781,.T.);
#8636=EDGE_CURVE('',#6704,#6705,#4782,.T.);
#8637=EDGE_CURVE('',#6706,#6703,#4783,.T.);
#8638=EDGE_CURVE('',#6700,#6705,#2463,.T.);
#8639=EDGE_CURVE('',#6707,#6707,#2464,.T.);
#8640=EDGE_CURVE('',#6024,#6022,#949,.T.);
#8641=EDGE_CURVE('',#6023,#6021,#950,.T.);
#8642=EDGE_CURVE('',#6011,#5993,#951,.T.);
#8643=EDGE_CURVE('',#6007,#6026,#952,.T.);
#8644=EDGE_CURVE('',#6003,#6005,#953,.T.);
#8645=EDGE_CURVE('',#5996,#6012,#954,.T.);
#8646=EDGE_CURVE('',#6006,#6004,#955,.T.);
#8647=EDGE_CURVE('',#6025,#6008,#956,.T.);
#8648=EDGE_CURVE('',#6708,#6709,#2465,.T.);
#8649=EDGE_CURVE('',#6708,#6710,#4784,.T.);
#8650=EDGE_CURVE('',#6710,#6711,#4785,.T.);
#8651=EDGE_CURVE('',#6711,#6709,#4786,.T.);
#8652=EDGE_CURVE('',#6712,#6708,#4787,.T.);
#8653=EDGE_CURVE('',#6712,#6713,#4788,.T.);
#8654=EDGE_CURVE('',#6713,#6710,#4789,.T.);
#8655=EDGE_CURVE('',#6709,#6714,#4790,.T.);
#8656=EDGE_CURVE('',#6715,#6711,#4791,.T.);
#8657=EDGE_CURVE('',#6715,#6714,#4792,.T.);
#8658=EDGE_CURVE('',#6713,#6715,#4793,.T.);
#8659=EDGE_CURVE('',#6714,#6712,#2466,.T.);
#8660=EDGE_CURVE('',#6716,#6716,#2467,.T.);
#8661=EDGE_CURVE('',#6717,#6717,#2468,.T.);
#8662=EDGE_CURVE('',#6718,#6718,#2469,.T.);
#8663=EDGE_CURVE('',#6719,#6719,#2470,.T.);
#8664=EDGE_CURVE('',#6717,#6719,#4794,.T.);
#8665=EDGE_CURVE('',#6718,#6720,#4795,.T.);
#8666=EDGE_CURVE('',#6720,#6720,#2471,.T.);
#8667=EDGE_CURVE('',#6721,#6721,#2472,.T.);
#8668=EDGE_CURVE('',#6722,#6722,#2473,.T.);
#8669=EDGE_CURVE('',#6723,#6723,#2474,.T.);
#8670=EDGE_CURVE('',#6721,#6723,#4796,.T.);
#8671=EDGE_CURVE('',#6722,#6707,#4797,.T.);
#8672=EDGE_CURVE('',#6724,#6724,#2475,.T.);
#8673=EDGE_CURVE('',#6724,#6716,#4798,.T.);
#8674=EDGE_CURVE('',#6699,#6706,#2476,.T.);
#9970=ORIENTED_EDGE('',*,*,#7574,.T.);
#9971=ORIENTED_EDGE('',*,*,#7575,.F.);
#9972=ORIENTED_EDGE('',*,*,#7576,.T.);
#9973=ORIENTED_EDGE('',*,*,#7577,.T.);
#9974=ORIENTED_EDGE('',*,*,#7578,.T.);
#9975=ORIENTED_EDGE('',*,*,#7579,.F.);
#9976=ORIENTED_EDGE('',*,*,#7574,.F.);
#9977=ORIENTED_EDGE('',*,*,#7580,.T.);
#9978=ORIENTED_EDGE('',*,*,#7581,.T.);
#9979=ORIENTED_EDGE('',*,*,#7582,.T.);
#9980=ORIENTED_EDGE('',*,*,#7577,.F.);
#9981=ORIENTED_EDGE('',*,*,#7583,.T.);
#9982=ORIENTED_EDGE('',*,*,#7584,.T.);
#9983=ORIENTED_EDGE('',*,*,#7585,.T.);
#9984=ORIENTED_EDGE('',*,*,#7581,.F.);
#9985=ORIENTED_EDGE('',*,*,#7586,.T.);
#9986=ORIENTED_EDGE('',*,*,#7587,.T.);
#9987=ORIENTED_EDGE('',*,*,#7588,.T.);
#9988=ORIENTED_EDGE('',*,*,#7584,.F.);
#9989=ORIENTED_EDGE('',*,*,#7589,.T.);
#9990=ORIENTED_EDGE('',*,*,#7590,.T.);
#9991=ORIENTED_EDGE('',*,*,#7591,.T.);
#9992=ORIENTED_EDGE('',*,*,#7587,.F.);
#9993=ORIENTED_EDGE('',*,*,#7592,.T.);
#9994=ORIENTED_EDGE('',*,*,#7593,.F.);
#9995=ORIENTED_EDGE('',*,*,#7594,.T.);
#9996=ORIENTED_EDGE('',*,*,#7595,.F.);
#9997=ORIENTED_EDGE('',*,*,#7596,.T.);
#9998=ORIENTED_EDGE('',*,*,#7597,.T.);
#9999=ORIENTED_EDGE('',*,*,#7598,.T.);
#10000=ORIENTED_EDGE('',*,*,#7599,.F.);
#10001=ORIENTED_EDGE('',*,*,#7600,.F.);
#10002=ORIENTED_EDGE('',*,*,#7601,.T.);
#10003=ORIENTED_EDGE('',*,*,#7602,.T.);
#10004=ORIENTED_EDGE('',*,*,#7597,.F.);
#10005=ORIENTED_EDGE('',*,*,#7603,.F.);
#10006=ORIENTED_EDGE('',*,*,#7604,.T.);
#10007=ORIENTED_EDGE('',*,*,#7605,.T.);
#10008=ORIENTED_EDGE('',*,*,#7601,.F.);
#10009=ORIENTED_EDGE('',*,*,#7606,.F.);
#10010=ORIENTED_EDGE('',*,*,#7607,.T.);
#10011=ORIENTED_EDGE('',*,*,#7608,.T.);
#10012=ORIENTED_EDGE('',*,*,#7604,.F.);
#10013=ORIENTED_EDGE('',*,*,#7609,.F.);
#10014=ORIENTED_EDGE('',*,*,#7610,.T.);
#10015=ORIENTED_EDGE('',*,*,#7611,.T.);
#10016=ORIENTED_EDGE('',*,*,#7607,.F.);
#10017=ORIENTED_EDGE('',*,*,#7612,.F.);
#10018=ORIENTED_EDGE('',*,*,#7613,.T.);
#10019=ORIENTED_EDGE('',*,*,#7614,.T.);
#10020=ORIENTED_EDGE('',*,*,#7610,.F.);
#10021=ORIENTED_EDGE('',*,*,#7615,.F.);
#10022=ORIENTED_EDGE('',*,*,#7616,.F.);
#10023=ORIENTED_EDGE('',*,*,#7617,.F.);
#10024=ORIENTED_EDGE('',*,*,#7618,.F.);
#10025=ORIENTED_EDGE('',*,*,#7619,.T.);
#10026=ORIENTED_EDGE('',*,*,#7620,.T.);
#10027=ORIENTED_EDGE('',*,*,#7621,.T.);
#10028=ORIENTED_EDGE('',*,*,#7622,.T.);
#10029=ORIENTED_EDGE('',*,*,#7623,.T.);
#10030=ORIENTED_EDGE('',*,*,#7624,.T.);
#10031=ORIENTED_EDGE('',*,*,#7623,.F.);
#10032=ORIENTED_EDGE('',*,*,#7625,.T.);
#10033=ORIENTED_EDGE('',*,*,#7626,.T.);
#10034=ORIENTED_EDGE('',*,*,#7627,.T.);
#10035=ORIENTED_EDGE('',*,*,#7628,.T.);
#10036=ORIENTED_EDGE('',*,*,#7620,.F.);
#10037=ORIENTED_EDGE('',*,*,#7629,.T.);
#10038=ORIENTED_EDGE('',*,*,#7630,.T.);
#10039=ORIENTED_EDGE('',*,*,#7631,.T.);
#10040=ORIENTED_EDGE('',*,*,#7627,.F.);
#10041=ORIENTED_EDGE('',*,*,#7632,.T.);
#10042=ORIENTED_EDGE('',*,*,#7633,.T.);
#10043=ORIENTED_EDGE('',*,*,#7634,.T.);
#10044=ORIENTED_EDGE('',*,*,#7630,.F.);
#10045=ORIENTED_EDGE('',*,*,#7635,.T.);
#10046=ORIENTED_EDGE('',*,*,#7636,.T.);
#10047=ORIENTED_EDGE('',*,*,#7637,.T.);
#10048=ORIENTED_EDGE('',*,*,#7633,.F.);
#10049=ORIENTED_EDGE('',*,*,#7638,.T.);
#10050=ORIENTED_EDGE('',*,*,#7639,.T.);
#10051=ORIENTED_EDGE('',*,*,#7640,.T.);
#10052=ORIENTED_EDGE('',*,*,#7636,.F.);
#10053=ORIENTED_EDGE('',*,*,#7641,.T.);
#10054=ORIENTED_EDGE('',*,*,#7642,.T.);
#10055=ORIENTED_EDGE('',*,*,#7643,.T.);
#10056=ORIENTED_EDGE('',*,*,#7639,.F.);
#10057=ORIENTED_EDGE('',*,*,#7644,.T.);
#10058=ORIENTED_EDGE('',*,*,#7645,.T.);
#10059=ORIENTED_EDGE('',*,*,#7646,.T.);
#10060=ORIENTED_EDGE('',*,*,#7642,.F.);
#10061=ORIENTED_EDGE('',*,*,#7647,.T.);
#10062=ORIENTED_EDGE('',*,*,#7648,.T.);
#10063=ORIENTED_EDGE('',*,*,#7649,.T.);
#10064=ORIENTED_EDGE('',*,*,#7645,.F.);
#10065=ORIENTED_EDGE('',*,*,#7650,.T.);
#10066=ORIENTED_EDGE('',*,*,#7651,.T.);
#10067=ORIENTED_EDGE('',*,*,#7652,.T.);
#10068=ORIENTED_EDGE('',*,*,#7648,.F.);
#10069=ORIENTED_EDGE('',*,*,#7653,.T.);
#10070=ORIENTED_EDGE('',*,*,#7654,.T.);
#10071=ORIENTED_EDGE('',*,*,#7655,.T.);
#10072=ORIENTED_EDGE('',*,*,#7651,.F.);
#10073=ORIENTED_EDGE('',*,*,#7656,.T.);
#10074=ORIENTED_EDGE('',*,*,#7657,.T.);
#10075=ORIENTED_EDGE('',*,*,#7658,.T.);
#10076=ORIENTED_EDGE('',*,*,#7654,.F.);
#10077=ORIENTED_EDGE('',*,*,#7659,.T.);
#10078=ORIENTED_EDGE('',*,*,#7660,.T.);
#10079=ORIENTED_EDGE('',*,*,#7661,.T.);
#10080=ORIENTED_EDGE('',*,*,#7657,.F.);
#10081=ORIENTED_EDGE('',*,*,#7662,.T.);
#10082=ORIENTED_EDGE('',*,*,#7663,.T.);
#10083=ORIENTED_EDGE('',*,*,#7664,.T.);
#10084=ORIENTED_EDGE('',*,*,#7660,.F.);
#10085=ORIENTED_EDGE('',*,*,#7665,.T.);
#10086=ORIENTED_EDGE('',*,*,#7666,.T.);
#10087=ORIENTED_EDGE('',*,*,#7667,.T.);
#10088=ORIENTED_EDGE('',*,*,#7663,.F.);
#10089=ORIENTED_EDGE('',*,*,#7668,.T.);
#10090=ORIENTED_EDGE('',*,*,#7669,.T.);
#10091=ORIENTED_EDGE('',*,*,#7670,.T.);
#10092=ORIENTED_EDGE('',*,*,#7666,.F.);
#10093=ORIENTED_EDGE('',*,*,#7671,.T.);
#10094=ORIENTED_EDGE('',*,*,#7672,.T.);
#10095=ORIENTED_EDGE('',*,*,#7673,.T.);
#10096=ORIENTED_EDGE('',*,*,#7669,.F.);
#10097=ORIENTED_EDGE('',*,*,#7674,.T.);
#10098=ORIENTED_EDGE('',*,*,#7675,.F.);
#10099=ORIENTED_EDGE('',*,*,#7676,.T.);
#10100=ORIENTED_EDGE('',*,*,#7677,.F.);
#10101=ORIENTED_EDGE('',*,*,#7678,.T.);
#10102=ORIENTED_EDGE('',*,*,#7679,.T.);
#10103=ORIENTED_EDGE('',*,*,#7680,.T.);
#10104=ORIENTED_EDGE('',*,*,#7681,.F.);
#10105=ORIENTED_EDGE('',*,*,#7682,.F.);
#10106=ORIENTED_EDGE('',*,*,#7683,.T.);
#10107=ORIENTED_EDGE('',*,*,#7684,.T.);
#10108=ORIENTED_EDGE('',*,*,#7679,.F.);
#10109=ORIENTED_EDGE('',*,*,#7685,.F.);
#10110=ORIENTED_EDGE('',*,*,#7686,.T.);
#10111=ORIENTED_EDGE('',*,*,#7687,.T.);
#10112=ORIENTED_EDGE('',*,*,#7683,.F.);
#10113=ORIENTED_EDGE('',*,*,#7688,.F.);
#10114=ORIENTED_EDGE('',*,*,#7689,.T.);
#10115=ORIENTED_EDGE('',*,*,#7690,.T.);
#10116=ORIENTED_EDGE('',*,*,#7686,.F.);
#10117=ORIENTED_EDGE('',*,*,#7691,.F.);
#10118=ORIENTED_EDGE('',*,*,#7692,.T.);
#10119=ORIENTED_EDGE('',*,*,#7693,.T.);
#10120=ORIENTED_EDGE('',*,*,#7689,.F.);
#10121=ORIENTED_EDGE('',*,*,#7694,.F.);
#10122=ORIENTED_EDGE('',*,*,#7695,.T.);
#10123=ORIENTED_EDGE('',*,*,#7696,.T.);
#10124=ORIENTED_EDGE('',*,*,#7692,.F.);
#10125=ORIENTED_EDGE('',*,*,#7697,.F.);
#10126=ORIENTED_EDGE('',*,*,#7698,.T.);
#10127=ORIENTED_EDGE('',*,*,#7699,.T.);
#10128=ORIENTED_EDGE('',*,*,#7695,.F.);
#10129=ORIENTED_EDGE('',*,*,#7700,.F.);
#10130=ORIENTED_EDGE('',*,*,#7701,.T.);
#10131=ORIENTED_EDGE('',*,*,#7702,.T.);
#10132=ORIENTED_EDGE('',*,*,#7698,.F.);
#10133=ORIENTED_EDGE('',*,*,#7703,.F.);
#10134=ORIENTED_EDGE('',*,*,#7704,.T.);
#10135=ORIENTED_EDGE('',*,*,#7705,.T.);
#10136=ORIENTED_EDGE('',*,*,#7701,.F.);
#10137=ORIENTED_EDGE('',*,*,#7706,.F.);
#10138=ORIENTED_EDGE('',*,*,#7707,.T.);
#10139=ORIENTED_EDGE('',*,*,#7708,.T.);
#10140=ORIENTED_EDGE('',*,*,#7704,.F.);
#10141=ORIENTED_EDGE('',*,*,#7709,.F.);
#10142=ORIENTED_EDGE('',*,*,#7710,.T.);
#10143=ORIENTED_EDGE('',*,*,#7711,.T.);
#10144=ORIENTED_EDGE('',*,*,#7707,.F.);
#10145=ORIENTED_EDGE('',*,*,#7712,.F.);
#10146=ORIENTED_EDGE('',*,*,#7713,.T.);
#10147=ORIENTED_EDGE('',*,*,#7714,.T.);
#10148=ORIENTED_EDGE('',*,*,#7710,.F.);
#10149=ORIENTED_EDGE('',*,*,#7715,.F.);
#10150=ORIENTED_EDGE('',*,*,#7716,.T.);
#10151=ORIENTED_EDGE('',*,*,#7717,.T.);
#10152=ORIENTED_EDGE('',*,*,#7713,.F.);
#10153=ORIENTED_EDGE('',*,*,#7718,.F.);
#10154=ORIENTED_EDGE('',*,*,#7719,.T.);
#10155=ORIENTED_EDGE('',*,*,#7720,.T.);
#10156=ORIENTED_EDGE('',*,*,#7716,.F.);
#10157=ORIENTED_EDGE('',*,*,#7721,.F.);
#10158=ORIENTED_EDGE('',*,*,#7722,.T.);
#10159=ORIENTED_EDGE('',*,*,#7723,.T.);
#10160=ORIENTED_EDGE('',*,*,#7719,.F.);
#10161=ORIENTED_EDGE('',*,*,#7724,.F.);
#10162=ORIENTED_EDGE('',*,*,#7725,.T.);
#10163=ORIENTED_EDGE('',*,*,#7726,.T.);
#10164=ORIENTED_EDGE('',*,*,#7722,.F.);
#10165=ORIENTED_EDGE('',*,*,#7727,.F.);
#10166=ORIENTED_EDGE('',*,*,#7728,.T.);
#10167=ORIENTED_EDGE('',*,*,#7729,.T.);
#10168=ORIENTED_EDGE('',*,*,#7725,.F.);
#10169=ORIENTED_EDGE('',*,*,#7730,.F.);
#10170=ORIENTED_EDGE('',*,*,#7731,.T.);
#10171=ORIENTED_EDGE('',*,*,#7732,.T.);
#10172=ORIENTED_EDGE('',*,*,#7728,.F.);
#10173=ORIENTED_EDGE('',*,*,#7733,.F.);
#10174=ORIENTED_EDGE('',*,*,#7734,.F.);
#10175=ORIENTED_EDGE('',*,*,#7735,.F.);
#10176=ORIENTED_EDGE('',*,*,#7736,.F.);
#10177=ORIENTED_EDGE('',*,*,#7737,.T.);
#10178=ORIENTED_EDGE('',*,*,#7738,.T.);
#10179=ORIENTED_EDGE('',*,*,#7739,.T.);
#10180=ORIENTED_EDGE('',*,*,#7740,.T.);
#10181=ORIENTED_EDGE('',*,*,#7741,.T.);
#10182=ORIENTED_EDGE('',*,*,#7742,.T.);
#10183=ORIENTED_EDGE('',*,*,#7741,.F.);
#10184=ORIENTED_EDGE('',*,*,#7743,.T.);
#10185=ORIENTED_EDGE('',*,*,#7744,.T.);
#10186=ORIENTED_EDGE('',*,*,#7745,.T.);
#10187=ORIENTED_EDGE('',*,*,#7746,.T.);
#10188=ORIENTED_EDGE('',*,*,#7738,.F.);
#10189=ORIENTED_EDGE('',*,*,#7747,.T.);
#10190=ORIENTED_EDGE('',*,*,#7748,.T.);
#10191=ORIENTED_EDGE('',*,*,#7749,.T.);
#10192=ORIENTED_EDGE('',*,*,#7745,.F.);
#10193=ORIENTED_EDGE('',*,*,#7750,.T.);
#10194=ORIENTED_EDGE('',*,*,#7751,.T.);
#10195=ORIENTED_EDGE('',*,*,#7752,.T.);
#10196=ORIENTED_EDGE('',*,*,#7748,.F.);
#10197=ORIENTED_EDGE('',*,*,#7753,.T.);
#10198=ORIENTED_EDGE('',*,*,#7754,.T.);
#10199=ORIENTED_EDGE('',*,*,#7755,.T.);
#10200=ORIENTED_EDGE('',*,*,#7751,.F.);
#10201=ORIENTED_EDGE('',*,*,#7756,.T.);
#10202=ORIENTED_EDGE('',*,*,#7757,.T.);
#10203=ORIENTED_EDGE('',*,*,#7758,.T.);
#10204=ORIENTED_EDGE('',*,*,#7754,.F.);
#10205=ORIENTED_EDGE('',*,*,#7759,.T.);
#10206=ORIENTED_EDGE('',*,*,#7760,.T.);
#10207=ORIENTED_EDGE('',*,*,#7761,.T.);
#10208=ORIENTED_EDGE('',*,*,#7757,.F.);
#10209=ORIENTED_EDGE('',*,*,#7762,.T.);
#10210=ORIENTED_EDGE('',*,*,#7763,.T.);
#10211=ORIENTED_EDGE('',*,*,#7764,.T.);
#10212=ORIENTED_EDGE('',*,*,#7760,.F.);
#10213=ORIENTED_EDGE('',*,*,#7765,.T.);
#10214=ORIENTED_EDGE('',*,*,#7766,.T.);
#10215=ORIENTED_EDGE('',*,*,#7767,.T.);
#10216=ORIENTED_EDGE('',*,*,#7763,.F.);
#10217=ORIENTED_EDGE('',*,*,#7768,.T.);
#10218=ORIENTED_EDGE('',*,*,#7769,.T.);
#10219=ORIENTED_EDGE('',*,*,#7770,.T.);
#10220=ORIENTED_EDGE('',*,*,#7766,.F.);
#10221=ORIENTED_EDGE('',*,*,#7771,.T.);
#10222=ORIENTED_EDGE('',*,*,#7772,.T.);
#10223=ORIENTED_EDGE('',*,*,#7773,.T.);
#10224=ORIENTED_EDGE('',*,*,#7769,.F.);
#10225=ORIENTED_EDGE('',*,*,#7774,.T.);
#10226=ORIENTED_EDGE('',*,*,#7775,.T.);
#10227=ORIENTED_EDGE('',*,*,#7776,.T.);
#10228=ORIENTED_EDGE('',*,*,#7772,.F.);
#10229=ORIENTED_EDGE('',*,*,#7777,.T.);
#10230=ORIENTED_EDGE('',*,*,#7778,.T.);
#10231=ORIENTED_EDGE('',*,*,#7779,.T.);
#10232=ORIENTED_EDGE('',*,*,#7775,.F.);
#10233=ORIENTED_EDGE('',*,*,#7780,.T.);
#10234=ORIENTED_EDGE('',*,*,#7781,.T.);
#10235=ORIENTED_EDGE('',*,*,#7782,.T.);
#10236=ORIENTED_EDGE('',*,*,#7778,.F.);
#10237=ORIENTED_EDGE('',*,*,#7783,.T.);
#10238=ORIENTED_EDGE('',*,*,#7784,.T.);
#10239=ORIENTED_EDGE('',*,*,#7785,.T.);
#10240=ORIENTED_EDGE('',*,*,#7781,.F.);
#10241=ORIENTED_EDGE('',*,*,#7786,.T.);
#10242=ORIENTED_EDGE('',*,*,#7787,.T.);
#10243=ORIENTED_EDGE('',*,*,#7788,.T.);
#10244=ORIENTED_EDGE('',*,*,#7784,.F.);
#10245=ORIENTED_EDGE('',*,*,#7789,.T.);
#10246=ORIENTED_EDGE('',*,*,#7790,.T.);
#10247=ORIENTED_EDGE('',*,*,#7791,.T.);
#10248=ORIENTED_EDGE('',*,*,#7787,.F.);
#10249=ORIENTED_EDGE('',*,*,#7792,.T.);
#10250=ORIENTED_EDGE('',*,*,#7793,.F.);
#10251=ORIENTED_EDGE('',*,*,#7794,.T.);
#10252=ORIENTED_EDGE('',*,*,#7795,.F.);
#10253=ORIENTED_EDGE('',*,*,#7796,.T.);
#10254=ORIENTED_EDGE('',*,*,#7797,.T.);
#10255=ORIENTED_EDGE('',*,*,#7798,.T.);
#10256=ORIENTED_EDGE('',*,*,#7799,.F.);
#10257=ORIENTED_EDGE('',*,*,#7800,.F.);
#10258=ORIENTED_EDGE('',*,*,#7801,.T.);
#10259=ORIENTED_EDGE('',*,*,#7802,.T.);
#10260=ORIENTED_EDGE('',*,*,#7797,.F.);
#10261=ORIENTED_EDGE('',*,*,#7803,.F.);
#10262=ORIENTED_EDGE('',*,*,#7804,.T.);
#10263=ORIENTED_EDGE('',*,*,#7805,.T.);
#10264=ORIENTED_EDGE('',*,*,#7801,.F.);
#10265=ORIENTED_EDGE('',*,*,#7806,.F.);
#10266=ORIENTED_EDGE('',*,*,#7807,.T.);
#10267=ORIENTED_EDGE('',*,*,#7808,.T.);
#10268=ORIENTED_EDGE('',*,*,#7804,.F.);
#10269=ORIENTED_EDGE('',*,*,#7809,.F.);
#10270=ORIENTED_EDGE('',*,*,#7810,.T.);
#10271=ORIENTED_EDGE('',*,*,#7811,.T.);
#10272=ORIENTED_EDGE('',*,*,#7807,.F.);
#10273=ORIENTED_EDGE('',*,*,#7812,.F.);
#10274=ORIENTED_EDGE('',*,*,#7813,.T.);
#10275=ORIENTED_EDGE('',*,*,#7814,.T.);
#10276=ORIENTED_EDGE('',*,*,#7810,.F.);
#10277=ORIENTED_EDGE('',*,*,#7815,.F.);
#10278=ORIENTED_EDGE('',*,*,#7816,.T.);
#10279=ORIENTED_EDGE('',*,*,#7817,.T.);
#10280=ORIENTED_EDGE('',*,*,#7813,.F.);
#10281=ORIENTED_EDGE('',*,*,#7818,.F.);
#10282=ORIENTED_EDGE('',*,*,#7819,.T.);
#10283=ORIENTED_EDGE('',*,*,#7820,.T.);
#10284=ORIENTED_EDGE('',*,*,#7816,.F.);
#10285=ORIENTED_EDGE('',*,*,#7821,.F.);
#10286=ORIENTED_EDGE('',*,*,#7822,.T.);
#10287=ORIENTED_EDGE('',*,*,#7823,.T.);
#10288=ORIENTED_EDGE('',*,*,#7819,.F.);
#10289=ORIENTED_EDGE('',*,*,#7824,.F.);
#10290=ORIENTED_EDGE('',*,*,#7825,.T.);
#10291=ORIENTED_EDGE('',*,*,#7826,.T.);
#10292=ORIENTED_EDGE('',*,*,#7822,.F.);
#10293=ORIENTED_EDGE('',*,*,#7827,.F.);
#10294=ORIENTED_EDGE('',*,*,#7828,.T.);
#10295=ORIENTED_EDGE('',*,*,#7829,.T.);
#10296=ORIENTED_EDGE('',*,*,#7825,.F.);
#10297=ORIENTED_EDGE('',*,*,#7830,.F.);
#10298=ORIENTED_EDGE('',*,*,#7831,.T.);
#10299=ORIENTED_EDGE('',*,*,#7832,.T.);
#10300=ORIENTED_EDGE('',*,*,#7828,.F.);
#10301=ORIENTED_EDGE('',*,*,#7833,.F.);
#10302=ORIENTED_EDGE('',*,*,#7834,.T.);
#10303=ORIENTED_EDGE('',*,*,#7835,.T.);
#10304=ORIENTED_EDGE('',*,*,#7831,.F.);
#10305=ORIENTED_EDGE('',*,*,#7836,.F.);
#10306=ORIENTED_EDGE('',*,*,#7837,.T.);
#10307=ORIENTED_EDGE('',*,*,#7838,.T.);
#10308=ORIENTED_EDGE('',*,*,#7834,.F.);
#10309=ORIENTED_EDGE('',*,*,#7839,.F.);
#10310=ORIENTED_EDGE('',*,*,#7840,.T.);
#10311=ORIENTED_EDGE('',*,*,#7841,.T.);
#10312=ORIENTED_EDGE('',*,*,#7837,.F.);
#10313=ORIENTED_EDGE('',*,*,#7842,.F.);
#10314=ORIENTED_EDGE('',*,*,#7843,.T.);
#10315=ORIENTED_EDGE('',*,*,#7844,.T.);
#10316=ORIENTED_EDGE('',*,*,#7840,.F.);
#10317=ORIENTED_EDGE('',*,*,#7845,.F.);
#10318=ORIENTED_EDGE('',*,*,#7846,.T.);
#10319=ORIENTED_EDGE('',*,*,#7847,.T.);
#10320=ORIENTED_EDGE('',*,*,#7843,.F.);
#10321=ORIENTED_EDGE('',*,*,#7848,.F.);
#10322=ORIENTED_EDGE('',*,*,#7849,.T.);
#10323=ORIENTED_EDGE('',*,*,#7850,.T.);
#10324=ORIENTED_EDGE('',*,*,#7846,.F.);
#10325=ORIENTED_EDGE('',*,*,#7851,.F.);
#10326=ORIENTED_EDGE('',*,*,#7852,.F.);
#10327=ORIENTED_EDGE('',*,*,#7853,.F.);
#10328=ORIENTED_EDGE('',*,*,#7854,.F.);
#10329=ORIENTED_EDGE('',*,*,#7855,.T.);
#10330=ORIENTED_EDGE('',*,*,#7856,.T.);
#10331=ORIENTED_EDGE('',*,*,#7857,.T.);
#10332=ORIENTED_EDGE('',*,*,#7858,.T.);
#10333=ORIENTED_EDGE('',*,*,#7859,.T.);
#10334=ORIENTED_EDGE('',*,*,#7860,.T.);
#10335=ORIENTED_EDGE('',*,*,#7859,.F.);
#10336=ORIENTED_EDGE('',*,*,#7861,.T.);
#10337=ORIENTED_EDGE('',*,*,#7862,.T.);
#10338=ORIENTED_EDGE('',*,*,#7863,.T.);
#10339=ORIENTED_EDGE('',*,*,#7864,.T.);
#10340=ORIENTED_EDGE('',*,*,#7856,.F.);
#10341=ORIENTED_EDGE('',*,*,#7865,.T.);
#10342=ORIENTED_EDGE('',*,*,#7866,.T.);
#10343=ORIENTED_EDGE('',*,*,#7867,.T.);
#10344=ORIENTED_EDGE('',*,*,#7863,.F.);
#10345=ORIENTED_EDGE('',*,*,#7868,.T.);
#10346=ORIENTED_EDGE('',*,*,#7869,.T.);
#10347=ORIENTED_EDGE('',*,*,#7870,.T.);
#10348=ORIENTED_EDGE('',*,*,#7866,.F.);
#10349=ORIENTED_EDGE('',*,*,#7871,.T.);
#10350=ORIENTED_EDGE('',*,*,#7872,.T.);
#10351=ORIENTED_EDGE('',*,*,#7873,.T.);
#10352=ORIENTED_EDGE('',*,*,#7869,.F.);
#10353=ORIENTED_EDGE('',*,*,#7874,.T.);
#10354=ORIENTED_EDGE('',*,*,#7875,.T.);
#10355=ORIENTED_EDGE('',*,*,#7876,.T.);
#10356=ORIENTED_EDGE('',*,*,#7872,.F.);
#10357=ORIENTED_EDGE('',*,*,#7877,.T.);
#10358=ORIENTED_EDGE('',*,*,#7878,.T.);
#10359=ORIENTED_EDGE('',*,*,#7879,.T.);
#10360=ORIENTED_EDGE('',*,*,#7875,.F.);
#10361=ORIENTED_EDGE('',*,*,#7880,.T.);
#10362=ORIENTED_EDGE('',*,*,#7881,.T.);
#10363=ORIENTED_EDGE('',*,*,#7882,.T.);
#10364=ORIENTED_EDGE('',*,*,#7878,.F.);
#10365=ORIENTED_EDGE('',*,*,#7883,.T.);
#10366=ORIENTED_EDGE('',*,*,#7884,.T.);
#10367=ORIENTED_EDGE('',*,*,#7885,.T.);
#10368=ORIENTED_EDGE('',*,*,#7881,.F.);
#10369=ORIENTED_EDGE('',*,*,#7886,.T.);
#10370=ORIENTED_EDGE('',*,*,#7887,.T.);
#10371=ORIENTED_EDGE('',*,*,#7888,.T.);
#10372=ORIENTED_EDGE('',*,*,#7884,.F.);
#10373=ORIENTED_EDGE('',*,*,#7889,.T.);
#10374=ORIENTED_EDGE('',*,*,#7890,.T.);
#10375=ORIENTED_EDGE('',*,*,#7891,.T.);
#10376=ORIENTED_EDGE('',*,*,#7887,.F.);
#10377=ORIENTED_EDGE('',*,*,#7892,.T.);
#10378=ORIENTED_EDGE('',*,*,#7893,.T.);
#10379=ORIENTED_EDGE('',*,*,#7894,.T.);
#10380=ORIENTED_EDGE('',*,*,#7890,.F.);
#10381=ORIENTED_EDGE('',*,*,#7895,.T.);
#10382=ORIENTED_EDGE('',*,*,#7896,.T.);
#10383=ORIENTED_EDGE('',*,*,#7897,.T.);
#10384=ORIENTED_EDGE('',*,*,#7893,.F.);
#10385=ORIENTED_EDGE('',*,*,#7898,.T.);
#10386=ORIENTED_EDGE('',*,*,#7899,.T.);
#10387=ORIENTED_EDGE('',*,*,#7900,.T.);
#10388=ORIENTED_EDGE('',*,*,#7896,.F.);
#10389=ORIENTED_EDGE('',*,*,#7901,.T.);
#10390=ORIENTED_EDGE('',*,*,#7902,.T.);
#10391=ORIENTED_EDGE('',*,*,#7903,.T.);
#10392=ORIENTED_EDGE('',*,*,#7899,.F.);
#10393=ORIENTED_EDGE('',*,*,#7904,.T.);
#10394=ORIENTED_EDGE('',*,*,#7905,.T.);
#10395=ORIENTED_EDGE('',*,*,#7906,.T.);
#10396=ORIENTED_EDGE('',*,*,#7902,.F.);
#10397=ORIENTED_EDGE('',*,*,#7907,.T.);
#10398=ORIENTED_EDGE('',*,*,#7908,.T.);
#10399=ORIENTED_EDGE('',*,*,#7909,.T.);
#10400=ORIENTED_EDGE('',*,*,#7905,.F.);
#10401=ORIENTED_EDGE('',*,*,#7910,.T.);
#10402=ORIENTED_EDGE('',*,*,#7911,.F.);
#10403=ORIENTED_EDGE('',*,*,#7912,.T.);
#10404=ORIENTED_EDGE('',*,*,#7913,.F.);
#10405=ORIENTED_EDGE('',*,*,#7914,.T.);
#10406=ORIENTED_EDGE('',*,*,#7915,.T.);
#10407=ORIENTED_EDGE('',*,*,#7916,.T.);
#10408=ORIENTED_EDGE('',*,*,#7917,.F.);
#10409=ORIENTED_EDGE('',*,*,#7918,.F.);
#10410=ORIENTED_EDGE('',*,*,#7919,.T.);
#10411=ORIENTED_EDGE('',*,*,#7920,.T.);
#10412=ORIENTED_EDGE('',*,*,#7915,.F.);
#10413=ORIENTED_EDGE('',*,*,#7921,.F.);
#10414=ORIENTED_EDGE('',*,*,#7922,.T.);
#10415=ORIENTED_EDGE('',*,*,#7923,.T.);
#10416=ORIENTED_EDGE('',*,*,#7919,.F.);
#10417=ORIENTED_EDGE('',*,*,#7924,.F.);
#10418=ORIENTED_EDGE('',*,*,#7925,.T.);
#10419=ORIENTED_EDGE('',*,*,#7926,.T.);
#10420=ORIENTED_EDGE('',*,*,#7922,.F.);
#10421=ORIENTED_EDGE('',*,*,#7927,.F.);
#10422=ORIENTED_EDGE('',*,*,#7928,.T.);
#10423=ORIENTED_EDGE('',*,*,#7929,.T.);
#10424=ORIENTED_EDGE('',*,*,#7925,.F.);
#10425=ORIENTED_EDGE('',*,*,#7930,.F.);
#10426=ORIENTED_EDGE('',*,*,#7931,.T.);
#10427=ORIENTED_EDGE('',*,*,#7932,.T.);
#10428=ORIENTED_EDGE('',*,*,#7928,.F.);
#10429=ORIENTED_EDGE('',*,*,#7933,.F.);
#10430=ORIENTED_EDGE('',*,*,#7934,.T.);
#10431=ORIENTED_EDGE('',*,*,#7935,.T.);
#10432=ORIENTED_EDGE('',*,*,#7931,.F.);
#10433=ORIENTED_EDGE('',*,*,#7936,.F.);
#10434=ORIENTED_EDGE('',*,*,#7937,.T.);
#10435=ORIENTED_EDGE('',*,*,#7938,.T.);
#10436=ORIENTED_EDGE('',*,*,#7934,.F.);
#10437=ORIENTED_EDGE('',*,*,#7939,.F.);
#10438=ORIENTED_EDGE('',*,*,#7940,.T.);
#10439=ORIENTED_EDGE('',*,*,#7941,.T.);
#10440=ORIENTED_EDGE('',*,*,#7937,.F.);
#10441=ORIENTED_EDGE('',*,*,#7942,.F.);
#10442=ORIENTED_EDGE('',*,*,#7943,.T.);
#10443=ORIENTED_EDGE('',*,*,#7944,.T.);
#10444=ORIENTED_EDGE('',*,*,#7940,.F.);
#10445=ORIENTED_EDGE('',*,*,#7945,.F.);
#10446=ORIENTED_EDGE('',*,*,#7946,.T.);
#10447=ORIENTED_EDGE('',*,*,#7947,.T.);
#10448=ORIENTED_EDGE('',*,*,#7943,.F.);
#10449=ORIENTED_EDGE('',*,*,#7948,.F.);
#10450=ORIENTED_EDGE('',*,*,#7949,.T.);
#10451=ORIENTED_EDGE('',*,*,#7950,.T.);
#10452=ORIENTED_EDGE('',*,*,#7946,.F.);
#10453=ORIENTED_EDGE('',*,*,#7951,.F.);
#10454=ORIENTED_EDGE('',*,*,#7952,.T.);
#10455=ORIENTED_EDGE('',*,*,#7953,.T.);
#10456=ORIENTED_EDGE('',*,*,#7949,.F.);
#10457=ORIENTED_EDGE('',*,*,#7954,.F.);
#10458=ORIENTED_EDGE('',*,*,#7955,.T.);
#10459=ORIENTED_EDGE('',*,*,#7956,.T.);
#10460=ORIENTED_EDGE('',*,*,#7952,.F.);
#10461=ORIENTED_EDGE('',*,*,#7957,.F.);
#10462=ORIENTED_EDGE('',*,*,#7958,.T.);
#10463=ORIENTED_EDGE('',*,*,#7959,.T.);
#10464=ORIENTED_EDGE('',*,*,#7955,.F.);
#10465=ORIENTED_EDGE('',*,*,#7960,.F.);
#10466=ORIENTED_EDGE('',*,*,#7961,.T.);
#10467=ORIENTED_EDGE('',*,*,#7962,.T.);
#10468=ORIENTED_EDGE('',*,*,#7958,.F.);
#10469=ORIENTED_EDGE('',*,*,#7963,.F.);
#10470=ORIENTED_EDGE('',*,*,#7964,.T.);
#10471=ORIENTED_EDGE('',*,*,#7965,.T.);
#10472=ORIENTED_EDGE('',*,*,#7961,.F.);
#10473=ORIENTED_EDGE('',*,*,#7966,.F.);
#10474=ORIENTED_EDGE('',*,*,#7967,.T.);
#10475=ORIENTED_EDGE('',*,*,#7968,.T.);
#10476=ORIENTED_EDGE('',*,*,#7964,.F.);
#10477=ORIENTED_EDGE('',*,*,#7969,.F.);
#10478=ORIENTED_EDGE('',*,*,#7970,.F.);
#10479=ORIENTED_EDGE('',*,*,#7971,.F.);
#10480=ORIENTED_EDGE('',*,*,#7972,.F.);
#10481=ORIENTED_EDGE('',*,*,#7973,.T.);
#10482=ORIENTED_EDGE('',*,*,#7974,.T.);
#10483=ORIENTED_EDGE('',*,*,#7975,.T.);
#10484=ORIENTED_EDGE('',*,*,#7976,.T.);
#10485=ORIENTED_EDGE('',*,*,#7977,.T.);
#10486=ORIENTED_EDGE('',*,*,#7978,.T.);
#10487=ORIENTED_EDGE('',*,*,#7977,.F.);
#10488=ORIENTED_EDGE('',*,*,#7979,.T.);
#10489=ORIENTED_EDGE('',*,*,#7980,.T.);
#10490=ORIENTED_EDGE('',*,*,#7981,.T.);
#10491=ORIENTED_EDGE('',*,*,#7982,.T.);
#10492=ORIENTED_EDGE('',*,*,#7974,.F.);
#10493=ORIENTED_EDGE('',*,*,#7983,.T.);
#10494=ORIENTED_EDGE('',*,*,#7984,.T.);
#10495=ORIENTED_EDGE('',*,*,#7985,.T.);
#10496=ORIENTED_EDGE('',*,*,#7981,.F.);
#10497=ORIENTED_EDGE('',*,*,#7986,.T.);
#10498=ORIENTED_EDGE('',*,*,#7987,.T.);
#10499=ORIENTED_EDGE('',*,*,#7988,.T.);
#10500=ORIENTED_EDGE('',*,*,#7984,.F.);
#10501=ORIENTED_EDGE('',*,*,#7989,.T.);
#10502=ORIENTED_EDGE('',*,*,#7990,.T.);
#10503=ORIENTED_EDGE('',*,*,#7991,.T.);
#10504=ORIENTED_EDGE('',*,*,#7987,.F.);
#10505=ORIENTED_EDGE('',*,*,#7992,.T.);
#10506=ORIENTED_EDGE('',*,*,#7993,.T.);
#10507=ORIENTED_EDGE('',*,*,#7994,.T.);
#10508=ORIENTED_EDGE('',*,*,#7990,.F.);
#10509=ORIENTED_EDGE('',*,*,#7995,.T.);
#10510=ORIENTED_EDGE('',*,*,#7996,.T.);
#10511=ORIENTED_EDGE('',*,*,#7997,.T.);
#10512=ORIENTED_EDGE('',*,*,#7993,.F.);
#10513=ORIENTED_EDGE('',*,*,#7998,.T.);
#10514=ORIENTED_EDGE('',*,*,#7999,.T.);
#10515=ORIENTED_EDGE('',*,*,#8000,.T.);
#10516=ORIENTED_EDGE('',*,*,#7996,.F.);
#10517=ORIENTED_EDGE('',*,*,#8001,.T.);
#10518=ORIENTED_EDGE('',*,*,#8002,.T.);
#10519=ORIENTED_EDGE('',*,*,#8003,.T.);
#10520=ORIENTED_EDGE('',*,*,#7999,.F.);
#10521=ORIENTED_EDGE('',*,*,#8004,.T.);
#10522=ORIENTED_EDGE('',*,*,#8005,.T.);
#10523=ORIENTED_EDGE('',*,*,#8006,.T.);
#10524=ORIENTED_EDGE('',*,*,#8002,.F.);
#10525=ORIENTED_EDGE('',*,*,#8007,.T.);
#10526=ORIENTED_EDGE('',*,*,#8008,.T.);
#10527=ORIENTED_EDGE('',*,*,#8009,.T.);
#10528=ORIENTED_EDGE('',*,*,#8005,.F.);
#10529=ORIENTED_EDGE('',*,*,#8010,.T.);
#10530=ORIENTED_EDGE('',*,*,#8011,.T.);
#10531=ORIENTED_EDGE('',*,*,#8012,.T.);
#10532=ORIENTED_EDGE('',*,*,#8008,.F.);
#10533=ORIENTED_EDGE('',*,*,#8013,.T.);
#10534=ORIENTED_EDGE('',*,*,#8014,.T.);
#10535=ORIENTED_EDGE('',*,*,#8015,.T.);
#10536=ORIENTED_EDGE('',*,*,#8011,.F.);
#10537=ORIENTED_EDGE('',*,*,#8016,.T.);
#10538=ORIENTED_EDGE('',*,*,#8017,.T.);
#10539=ORIENTED_EDGE('',*,*,#8018,.T.);
#10540=ORIENTED_EDGE('',*,*,#8014,.F.);
#10541=ORIENTED_EDGE('',*,*,#8019,.T.);
#10542=ORIENTED_EDGE('',*,*,#8020,.T.);
#10543=ORIENTED_EDGE('',*,*,#8021,.T.);
#10544=ORIENTED_EDGE('',*,*,#8017,.F.);
#10545=ORIENTED_EDGE('',*,*,#8022,.T.);
#10546=ORIENTED_EDGE('',*,*,#8023,.T.);
#10547=ORIENTED_EDGE('',*,*,#8024,.T.);
#10548=ORIENTED_EDGE('',*,*,#8020,.F.);
#10549=ORIENTED_EDGE('',*,*,#8025,.T.);
#10550=ORIENTED_EDGE('',*,*,#8026,.T.);
#10551=ORIENTED_EDGE('',*,*,#8027,.T.);
#10552=ORIENTED_EDGE('',*,*,#8023,.F.);
#10553=ORIENTED_EDGE('',*,*,#8028,.T.);
#10554=ORIENTED_EDGE('',*,*,#8029,.F.);
#10555=ORIENTED_EDGE('',*,*,#8030,.T.);
#10556=ORIENTED_EDGE('',*,*,#8031,.F.);
#10557=ORIENTED_EDGE('',*,*,#8032,.T.);
#10558=ORIENTED_EDGE('',*,*,#8033,.T.);
#10559=ORIENTED_EDGE('',*,*,#8034,.T.);
#10560=ORIENTED_EDGE('',*,*,#8035,.F.);
#10561=ORIENTED_EDGE('',*,*,#8036,.F.);
#10562=ORIENTED_EDGE('',*,*,#8037,.T.);
#10563=ORIENTED_EDGE('',*,*,#8038,.T.);
#10564=ORIENTED_EDGE('',*,*,#8033,.F.);
#10565=ORIENTED_EDGE('',*,*,#8039,.F.);
#10566=ORIENTED_EDGE('',*,*,#8040,.T.);
#10567=ORIENTED_EDGE('',*,*,#8041,.T.);
#10568=ORIENTED_EDGE('',*,*,#8037,.F.);
#10569=ORIENTED_EDGE('',*,*,#8042,.F.);
#10570=ORIENTED_EDGE('',*,*,#8043,.T.);
#10571=ORIENTED_EDGE('',*,*,#8044,.T.);
#10572=ORIENTED_EDGE('',*,*,#8040,.F.);
#10573=ORIENTED_EDGE('',*,*,#8045,.F.);
#10574=ORIENTED_EDGE('',*,*,#8046,.T.);
#10575=ORIENTED_EDGE('',*,*,#8047,.T.);
#10576=ORIENTED_EDGE('',*,*,#8043,.F.);
#10577=ORIENTED_EDGE('',*,*,#8048,.F.);
#10578=ORIENTED_EDGE('',*,*,#8049,.T.);
#10579=ORIENTED_EDGE('',*,*,#8050,.T.);
#10580=ORIENTED_EDGE('',*,*,#8046,.F.);
#10581=ORIENTED_EDGE('',*,*,#8051,.F.);
#10582=ORIENTED_EDGE('',*,*,#8052,.T.);
#10583=ORIENTED_EDGE('',*,*,#8053,.T.);
#10584=ORIENTED_EDGE('',*,*,#8049,.F.);
#10585=ORIENTED_EDGE('',*,*,#8054,.F.);
#10586=ORIENTED_EDGE('',*,*,#8055,.T.);
#10587=ORIENTED_EDGE('',*,*,#8056,.T.);
#10588=ORIENTED_EDGE('',*,*,#8052,.F.);
#10589=ORIENTED_EDGE('',*,*,#8057,.F.);
#10590=ORIENTED_EDGE('',*,*,#8058,.T.);
#10591=ORIENTED_EDGE('',*,*,#8059,.T.);
#10592=ORIENTED_EDGE('',*,*,#8055,.F.);
#10593=ORIENTED_EDGE('',*,*,#8060,.F.);
#10594=ORIENTED_EDGE('',*,*,#8061,.T.);
#10595=ORIENTED_EDGE('',*,*,#8062,.T.);
#10596=ORIENTED_EDGE('',*,*,#8058,.F.);
#10597=ORIENTED_EDGE('',*,*,#8063,.F.);
#10598=ORIENTED_EDGE('',*,*,#8064,.T.);
#10599=ORIENTED_EDGE('',*,*,#8065,.T.);
#10600=ORIENTED_EDGE('',*,*,#8061,.F.);
#10601=ORIENTED_EDGE('',*,*,#8066,.F.);
#10602=ORIENTED_EDGE('',*,*,#8067,.T.);
#10603=ORIENTED_EDGE('',*,*,#8068,.T.);
#10604=ORIENTED_EDGE('',*,*,#8064,.F.);
#10605=ORIENTED_EDGE('',*,*,#8069,.F.);
#10606=ORIENTED_EDGE('',*,*,#8070,.T.);
#10607=ORIENTED_EDGE('',*,*,#8071,.T.);
#10608=ORIENTED_EDGE('',*,*,#8067,.F.);
#10609=ORIENTED_EDGE('',*,*,#8072,.F.);
#10610=ORIENTED_EDGE('',*,*,#8073,.T.);
#10611=ORIENTED_EDGE('',*,*,#8074,.T.);
#10612=ORIENTED_EDGE('',*,*,#8070,.F.);
#10613=ORIENTED_EDGE('',*,*,#8075,.F.);
#10614=ORIENTED_EDGE('',*,*,#8076,.T.);
#10615=ORIENTED_EDGE('',*,*,#8077,.T.);
#10616=ORIENTED_EDGE('',*,*,#8073,.F.);
#10617=ORIENTED_EDGE('',*,*,#8078,.F.);
#10618=ORIENTED_EDGE('',*,*,#8079,.T.);
#10619=ORIENTED_EDGE('',*,*,#8080,.T.);
#10620=ORIENTED_EDGE('',*,*,#8076,.F.);
#10621=ORIENTED_EDGE('',*,*,#8081,.F.);
#10622=ORIENTED_EDGE('',*,*,#8082,.T.);
#10623=ORIENTED_EDGE('',*,*,#8083,.T.);
#10624=ORIENTED_EDGE('',*,*,#8079,.F.);
#10625=ORIENTED_EDGE('',*,*,#8084,.F.);
#10626=ORIENTED_EDGE('',*,*,#8085,.T.);
#10627=ORIENTED_EDGE('',*,*,#8086,.T.);
#10628=ORIENTED_EDGE('',*,*,#8082,.F.);
#10629=ORIENTED_EDGE('',*,*,#8087,.F.);
#10630=ORIENTED_EDGE('',*,*,#8088,.F.);
#10631=ORIENTED_EDGE('',*,*,#8089,.F.);
#10632=ORIENTED_EDGE('',*,*,#8090,.F.);
#10633=ORIENTED_EDGE('',*,*,#8091,.T.);
#10634=ORIENTED_EDGE('',*,*,#8092,.T.);
#10635=ORIENTED_EDGE('',*,*,#8093,.T.);
#10636=ORIENTED_EDGE('',*,*,#8094,.T.);
#10637=ORIENTED_EDGE('',*,*,#8095,.T.);
#10638=ORIENTED_EDGE('',*,*,#8096,.T.);
#10639=ORIENTED_EDGE('',*,*,#8095,.F.);
#10640=ORIENTED_EDGE('',*,*,#8097,.T.);
#10641=ORIENTED_EDGE('',*,*,#8098,.T.);
#10642=ORIENTED_EDGE('',*,*,#8099,.T.);
#10643=ORIENTED_EDGE('',*,*,#8100,.T.);
#10644=ORIENTED_EDGE('',*,*,#8092,.F.);
#10645=ORIENTED_EDGE('',*,*,#8101,.T.);
#10646=ORIENTED_EDGE('',*,*,#8102,.T.);
#10647=ORIENTED_EDGE('',*,*,#8103,.T.);
#10648=ORIENTED_EDGE('',*,*,#8099,.F.);
#10649=ORIENTED_EDGE('',*,*,#8104,.T.);
#10650=ORIENTED_EDGE('',*,*,#8105,.T.);
#10651=ORIENTED_EDGE('',*,*,#8106,.T.);
#10652=ORIENTED_EDGE('',*,*,#8102,.F.);
#10653=ORIENTED_EDGE('',*,*,#8107,.T.);
#10654=ORIENTED_EDGE('',*,*,#8108,.T.);
#10655=ORIENTED_EDGE('',*,*,#8109,.T.);
#10656=ORIENTED_EDGE('',*,*,#8105,.F.);
#10657=ORIENTED_EDGE('',*,*,#8110,.T.);
#10658=ORIENTED_EDGE('',*,*,#8111,.T.);
#10659=ORIENTED_EDGE('',*,*,#8112,.T.);
#10660=ORIENTED_EDGE('',*,*,#8108,.F.);
#10661=ORIENTED_EDGE('',*,*,#8113,.T.);
#10662=ORIENTED_EDGE('',*,*,#8114,.T.);
#10663=ORIENTED_EDGE('',*,*,#8115,.T.);
#10664=ORIENTED_EDGE('',*,*,#8111,.F.);
#10665=ORIENTED_EDGE('',*,*,#8116,.T.);
#10666=ORIENTED_EDGE('',*,*,#8117,.T.);
#10667=ORIENTED_EDGE('',*,*,#8118,.T.);
#10668=ORIENTED_EDGE('',*,*,#8114,.F.);
#10669=ORIENTED_EDGE('',*,*,#8119,.T.);
#10670=ORIENTED_EDGE('',*,*,#8120,.T.);
#10671=ORIENTED_EDGE('',*,*,#8121,.T.);
#10672=ORIENTED_EDGE('',*,*,#8117,.F.);
#10673=ORIENTED_EDGE('',*,*,#8122,.T.);
#10674=ORIENTED_EDGE('',*,*,#8123,.T.);
#10675=ORIENTED_EDGE('',*,*,#8124,.T.);
#10676=ORIENTED_EDGE('',*,*,#8120,.F.);
#10677=ORIENTED_EDGE('',*,*,#8125,.T.);
#10678=ORIENTED_EDGE('',*,*,#8126,.T.);
#10679=ORIENTED_EDGE('',*,*,#8127,.T.);
#10680=ORIENTED_EDGE('',*,*,#8123,.F.);
#10681=ORIENTED_EDGE('',*,*,#8128,.T.);
#10682=ORIENTED_EDGE('',*,*,#8129,.T.);
#10683=ORIENTED_EDGE('',*,*,#8130,.T.);
#10684=ORIENTED_EDGE('',*,*,#8126,.F.);
#10685=ORIENTED_EDGE('',*,*,#8131,.T.);
#10686=ORIENTED_EDGE('',*,*,#8132,.T.);
#10687=ORIENTED_EDGE('',*,*,#8133,.T.);
#10688=ORIENTED_EDGE('',*,*,#8129,.F.);
#10689=ORIENTED_EDGE('',*,*,#8134,.T.);
#10690=ORIENTED_EDGE('',*,*,#8135,.T.);
#10691=ORIENTED_EDGE('',*,*,#8136,.T.);
#10692=ORIENTED_EDGE('',*,*,#8132,.F.);
#10693=ORIENTED_EDGE('',*,*,#8137,.T.);
#10694=ORIENTED_EDGE('',*,*,#8138,.T.);
#10695=ORIENTED_EDGE('',*,*,#8139,.T.);
#10696=ORIENTED_EDGE('',*,*,#8135,.F.);
#10697=ORIENTED_EDGE('',*,*,#8140,.T.);
#10698=ORIENTED_EDGE('',*,*,#8141,.T.);
#10699=ORIENTED_EDGE('',*,*,#8142,.T.);
#10700=ORIENTED_EDGE('',*,*,#8138,.F.);
#10701=ORIENTED_EDGE('',*,*,#8143,.T.);
#10702=ORIENTED_EDGE('',*,*,#8144,.T.);
#10703=ORIENTED_EDGE('',*,*,#8145,.T.);
#10704=ORIENTED_EDGE('',*,*,#8141,.F.);
#10705=ORIENTED_EDGE('',*,*,#8146,.T.);
#10706=ORIENTED_EDGE('',*,*,#8147,.F.);
#10707=ORIENTED_EDGE('',*,*,#8148,.T.);
#10708=ORIENTED_EDGE('',*,*,#8149,.F.);
#10709=ORIENTED_EDGE('',*,*,#8150,.T.);
#10710=ORIENTED_EDGE('',*,*,#8151,.T.);
#10711=ORIENTED_EDGE('',*,*,#8152,.T.);
#10712=ORIENTED_EDGE('',*,*,#8153,.F.);
#10713=ORIENTED_EDGE('',*,*,#8154,.F.);
#10714=ORIENTED_EDGE('',*,*,#8155,.T.);
#10715=ORIENTED_EDGE('',*,*,#8156,.T.);
#10716=ORIENTED_EDGE('',*,*,#8151,.F.);
#10717=ORIENTED_EDGE('',*,*,#8157,.F.);
#10718=ORIENTED_EDGE('',*,*,#8158,.T.);
#10719=ORIENTED_EDGE('',*,*,#8159,.T.);
#10720=ORIENTED_EDGE('',*,*,#8155,.F.);
#10721=ORIENTED_EDGE('',*,*,#8160,.F.);
#10722=ORIENTED_EDGE('',*,*,#8161,.T.);
#10723=ORIENTED_EDGE('',*,*,#8162,.T.);
#10724=ORIENTED_EDGE('',*,*,#8158,.F.);
#10725=ORIENTED_EDGE('',*,*,#8163,.F.);
#10726=ORIENTED_EDGE('',*,*,#8164,.T.);
#10727=ORIENTED_EDGE('',*,*,#8165,.T.);
#10728=ORIENTED_EDGE('',*,*,#8161,.F.);
#10729=ORIENTED_EDGE('',*,*,#8166,.F.);
#10730=ORIENTED_EDGE('',*,*,#8167,.T.);
#10731=ORIENTED_EDGE('',*,*,#8168,.T.);
#10732=ORIENTED_EDGE('',*,*,#8164,.F.);
#10733=ORIENTED_EDGE('',*,*,#8169,.F.);
#10734=ORIENTED_EDGE('',*,*,#8170,.T.);
#10735=ORIENTED_EDGE('',*,*,#8171,.T.);
#10736=ORIENTED_EDGE('',*,*,#8167,.F.);
#10737=ORIENTED_EDGE('',*,*,#8172,.F.);
#10738=ORIENTED_EDGE('',*,*,#8173,.T.);
#10739=ORIENTED_EDGE('',*,*,#8174,.T.);
#10740=ORIENTED_EDGE('',*,*,#8170,.F.);
#10741=ORIENTED_EDGE('',*,*,#8175,.F.);
#10742=ORIENTED_EDGE('',*,*,#8176,.T.);
#10743=ORIENTED_EDGE('',*,*,#8177,.T.);
#10744=ORIENTED_EDGE('',*,*,#8173,.F.);
#10745=ORIENTED_EDGE('',*,*,#8178,.F.);
#10746=ORIENTED_EDGE('',*,*,#8179,.T.);
#10747=ORIENTED_EDGE('',*,*,#8180,.T.);
#10748=ORIENTED_EDGE('',*,*,#8176,.F.);
#10749=ORIENTED_EDGE('',*,*,#8181,.F.);
#10750=ORIENTED_EDGE('',*,*,#8182,.T.);
#10751=ORIENTED_EDGE('',*,*,#8183,.T.);
#10752=ORIENTED_EDGE('',*,*,#8179,.F.);
#10753=ORIENTED_EDGE('',*,*,#8184,.F.);
#10754=ORIENTED_EDGE('',*,*,#8185,.T.);
#10755=ORIENTED_EDGE('',*,*,#8186,.T.);
#10756=ORIENTED_EDGE('',*,*,#8182,.F.);
#10757=ORIENTED_EDGE('',*,*,#8187,.F.);
#10758=ORIENTED_EDGE('',*,*,#8188,.T.);
#10759=ORIENTED_EDGE('',*,*,#8189,.T.);
#10760=ORIENTED_EDGE('',*,*,#8185,.F.);
#10761=ORIENTED_EDGE('',*,*,#8190,.F.);
#10762=ORIENTED_EDGE('',*,*,#8191,.T.);
#10763=ORIENTED_EDGE('',*,*,#8192,.T.);
#10764=ORIENTED_EDGE('',*,*,#8188,.F.);
#10765=ORIENTED_EDGE('',*,*,#8193,.F.);
#10766=ORIENTED_EDGE('',*,*,#8194,.T.);
#10767=ORIENTED_EDGE('',*,*,#8195,.T.);
#10768=ORIENTED_EDGE('',*,*,#8191,.F.);
#10769=ORIENTED_EDGE('',*,*,#8196,.F.);
#10770=ORIENTED_EDGE('',*,*,#8197,.T.);
#10771=ORIENTED_EDGE('',*,*,#8198,.T.);
#10772=ORIENTED_EDGE('',*,*,#8194,.F.);
#10773=ORIENTED_EDGE('',*,*,#8199,.F.);
#10774=ORIENTED_EDGE('',*,*,#8200,.T.);
#10775=ORIENTED_EDGE('',*,*,#8201,.T.);
#10776=ORIENTED_EDGE('',*,*,#8197,.F.);
#10777=ORIENTED_EDGE('',*,*,#8202,.F.);
#10778=ORIENTED_EDGE('',*,*,#8203,.T.);
#10779=ORIENTED_EDGE('',*,*,#8204,.T.);
#10780=ORIENTED_EDGE('',*,*,#8200,.F.);
#10781=ORIENTED_EDGE('',*,*,#8205,.F.);
#10782=ORIENTED_EDGE('',*,*,#8206,.F.);
#10783=ORIENTED_EDGE('',*,*,#8207,.F.);
#10784=ORIENTED_EDGE('',*,*,#8208,.F.);
#10785=ORIENTED_EDGE('',*,*,#8209,.T.);
#10786=ORIENTED_EDGE('',*,*,#8210,.T.);
#10787=ORIENTED_EDGE('',*,*,#8211,.T.);
#10788=ORIENTED_EDGE('',*,*,#8212,.T.);
#10789=ORIENTED_EDGE('',*,*,#8213,.T.);
#10790=ORIENTED_EDGE('',*,*,#8214,.T.);
#10791=ORIENTED_EDGE('',*,*,#8213,.F.);
#10792=ORIENTED_EDGE('',*,*,#8215,.T.);
#10793=ORIENTED_EDGE('',*,*,#8216,.T.);
#10794=ORIENTED_EDGE('',*,*,#8217,.T.);
#10795=ORIENTED_EDGE('',*,*,#8218,.T.);
#10796=ORIENTED_EDGE('',*,*,#8210,.F.);
#10797=ORIENTED_EDGE('',*,*,#8219,.T.);
#10798=ORIENTED_EDGE('',*,*,#8220,.T.);
#10799=ORIENTED_EDGE('',*,*,#8221,.T.);
#10800=ORIENTED_EDGE('',*,*,#8217,.F.);
#10801=ORIENTED_EDGE('',*,*,#8222,.T.);
#10802=ORIENTED_EDGE('',*,*,#8223,.T.);
#10803=ORIENTED_EDGE('',*,*,#8224,.T.);
#10804=ORIENTED_EDGE('',*,*,#8220,.F.);
#10805=ORIENTED_EDGE('',*,*,#8225,.T.);
#10806=ORIENTED_EDGE('',*,*,#8226,.T.);
#10807=ORIENTED_EDGE('',*,*,#8227,.T.);
#10808=ORIENTED_EDGE('',*,*,#8223,.F.);
#10809=ORIENTED_EDGE('',*,*,#8228,.T.);
#10810=ORIENTED_EDGE('',*,*,#8229,.T.);
#10811=ORIENTED_EDGE('',*,*,#8230,.T.);
#10812=ORIENTED_EDGE('',*,*,#8226,.F.);
#10813=ORIENTED_EDGE('',*,*,#8231,.T.);
#10814=ORIENTED_EDGE('',*,*,#8232,.T.);
#10815=ORIENTED_EDGE('',*,*,#8233,.T.);
#10816=ORIENTED_EDGE('',*,*,#8229,.F.);
#10817=ORIENTED_EDGE('',*,*,#8234,.T.);
#10818=ORIENTED_EDGE('',*,*,#8235,.T.);
#10819=ORIENTED_EDGE('',*,*,#8236,.T.);
#10820=ORIENTED_EDGE('',*,*,#8232,.F.);
#10821=ORIENTED_EDGE('',*,*,#8237,.T.);
#10822=ORIENTED_EDGE('',*,*,#8238,.T.);
#10823=ORIENTED_EDGE('',*,*,#8239,.T.);
#10824=ORIENTED_EDGE('',*,*,#8235,.F.);
#10825=ORIENTED_EDGE('',*,*,#8240,.T.);
#10826=ORIENTED_EDGE('',*,*,#8241,.T.);
#10827=ORIENTED_EDGE('',*,*,#8242,.T.);
#10828=ORIENTED_EDGE('',*,*,#8238,.F.);
#10829=ORIENTED_EDGE('',*,*,#8243,.T.);
#10830=ORIENTED_EDGE('',*,*,#8244,.T.);
#10831=ORIENTED_EDGE('',*,*,#8245,.T.);
#10832=ORIENTED_EDGE('',*,*,#8241,.F.);
#10833=ORIENTED_EDGE('',*,*,#8246,.T.);
#10834=ORIENTED_EDGE('',*,*,#8247,.T.);
#10835=ORIENTED_EDGE('',*,*,#8248,.T.);
#10836=ORIENTED_EDGE('',*,*,#8244,.F.);
#10837=ORIENTED_EDGE('',*,*,#8249,.T.);
#10838=ORIENTED_EDGE('',*,*,#8250,.T.);
#10839=ORIENTED_EDGE('',*,*,#8251,.T.);
#10840=ORIENTED_EDGE('',*,*,#8247,.F.);
#10841=ORIENTED_EDGE('',*,*,#8252,.T.);
#10842=ORIENTED_EDGE('',*,*,#8253,.T.);
#10843=ORIENTED_EDGE('',*,*,#8254,.T.);
#10844=ORIENTED_EDGE('',*,*,#8250,.F.);
#10845=ORIENTED_EDGE('',*,*,#8255,.T.);
#10846=ORIENTED_EDGE('',*,*,#8256,.T.);
#10847=ORIENTED_EDGE('',*,*,#8257,.T.);
#10848=ORIENTED_EDGE('',*,*,#8253,.F.);
#10849=ORIENTED_EDGE('',*,*,#8258,.T.);
#10850=ORIENTED_EDGE('',*,*,#8259,.T.);
#10851=ORIENTED_EDGE('',*,*,#8260,.T.);
#10852=ORIENTED_EDGE('',*,*,#8256,.F.);
#10853=ORIENTED_EDGE('',*,*,#8261,.T.);
#10854=ORIENTED_EDGE('',*,*,#8262,.T.);
#10855=ORIENTED_EDGE('',*,*,#8263,.T.);
#10856=ORIENTED_EDGE('',*,*,#8259,.F.);
#10857=ORIENTED_EDGE('',*,*,#8264,.T.);
#10858=ORIENTED_EDGE('',*,*,#8265,.F.);
#10859=ORIENTED_EDGE('',*,*,#8266,.T.);
#10860=ORIENTED_EDGE('',*,*,#8267,.F.);
#10861=ORIENTED_EDGE('',*,*,#8268,.T.);
#10862=ORIENTED_EDGE('',*,*,#8269,.T.);
#10863=ORIENTED_EDGE('',*,*,#8270,.T.);
#10864=ORIENTED_EDGE('',*,*,#8271,.F.);
#10865=ORIENTED_EDGE('',*,*,#8272,.F.);
#10866=ORIENTED_EDGE('',*,*,#8273,.T.);
#10867=ORIENTED_EDGE('',*,*,#8274,.T.);
#10868=ORIENTED_EDGE('',*,*,#8269,.F.);
#10869=ORIENTED_EDGE('',*,*,#8275,.F.);
#10870=ORIENTED_EDGE('',*,*,#8276,.T.);
#10871=ORIENTED_EDGE('',*,*,#8277,.T.);
#10872=ORIENTED_EDGE('',*,*,#8273,.F.);
#10873=ORIENTED_EDGE('',*,*,#8278,.F.);
#10874=ORIENTED_EDGE('',*,*,#8279,.T.);
#10875=ORIENTED_EDGE('',*,*,#8280,.T.);
#10876=ORIENTED_EDGE('',*,*,#8276,.F.);
#10877=ORIENTED_EDGE('',*,*,#8281,.F.);
#10878=ORIENTED_EDGE('',*,*,#8282,.T.);
#10879=ORIENTED_EDGE('',*,*,#8283,.T.);
#10880=ORIENTED_EDGE('',*,*,#8279,.F.);
#10881=ORIENTED_EDGE('',*,*,#8284,.F.);
#10882=ORIENTED_EDGE('',*,*,#8285,.T.);
#10883=ORIENTED_EDGE('',*,*,#8286,.T.);
#10884=ORIENTED_EDGE('',*,*,#8282,.F.);
#10885=ORIENTED_EDGE('',*,*,#8287,.F.);
#10886=ORIENTED_EDGE('',*,*,#8288,.T.);
#10887=ORIENTED_EDGE('',*,*,#8289,.T.);
#10888=ORIENTED_EDGE('',*,*,#8285,.F.);
#10889=ORIENTED_EDGE('',*,*,#8290,.F.);
#10890=ORIENTED_EDGE('',*,*,#8291,.T.);
#10891=ORIENTED_EDGE('',*,*,#8292,.T.);
#10892=ORIENTED_EDGE('',*,*,#8288,.F.);
#10893=ORIENTED_EDGE('',*,*,#8293,.F.);
#10894=ORIENTED_EDGE('',*,*,#8294,.T.);
#10895=ORIENTED_EDGE('',*,*,#8295,.T.);
#10896=ORIENTED_EDGE('',*,*,#8291,.F.);
#10897=ORIENTED_EDGE('',*,*,#8296,.F.);
#10898=ORIENTED_EDGE('',*,*,#8297,.T.);
#10899=ORIENTED_EDGE('',*,*,#8298,.T.);
#10900=ORIENTED_EDGE('',*,*,#8294,.F.);
#10901=ORIENTED_EDGE('',*,*,#8299,.F.);
#10902=ORIENTED_EDGE('',*,*,#8300,.T.);
#10903=ORIENTED_EDGE('',*,*,#8301,.T.);
#10904=ORIENTED_EDGE('',*,*,#8297,.F.);
#10905=ORIENTED_EDGE('',*,*,#8302,.F.);
#10906=ORIENTED_EDGE('',*,*,#8303,.T.);
#10907=ORIENTED_EDGE('',*,*,#8304,.T.);
#10908=ORIENTED_EDGE('',*,*,#8300,.F.);
#10909=ORIENTED_EDGE('',*,*,#8305,.F.);
#10910=ORIENTED_EDGE('',*,*,#8306,.T.);
#10911=ORIENTED_EDGE('',*,*,#8307,.T.);
#10912=ORIENTED_EDGE('',*,*,#8303,.F.);
#10913=ORIENTED_EDGE('',*,*,#8308,.F.);
#10914=ORIENTED_EDGE('',*,*,#8309,.T.);
#10915=ORIENTED_EDGE('',*,*,#8310,.T.);
#10916=ORIENTED_EDGE('',*,*,#8306,.F.);
#10917=ORIENTED_EDGE('',*,*,#8311,.F.);
#10918=ORIENTED_EDGE('',*,*,#8312,.T.);
#10919=ORIENTED_EDGE('',*,*,#8313,.T.);
#10920=ORIENTED_EDGE('',*,*,#8309,.F.);
#10921=ORIENTED_EDGE('',*,*,#8314,.F.);
#10922=ORIENTED_EDGE('',*,*,#8315,.T.);
#10923=ORIENTED_EDGE('',*,*,#8316,.T.);
#10924=ORIENTED_EDGE('',*,*,#8312,.F.);
#10925=ORIENTED_EDGE('',*,*,#8317,.F.);
#10926=ORIENTED_EDGE('',*,*,#8318,.T.);
#10927=ORIENTED_EDGE('',*,*,#8319,.T.);
#10928=ORIENTED_EDGE('',*,*,#8315,.F.);
#10929=ORIENTED_EDGE('',*,*,#8320,.F.);
#10930=ORIENTED_EDGE('',*,*,#8321,.T.);
#10931=ORIENTED_EDGE('',*,*,#8322,.T.);
#10932=ORIENTED_EDGE('',*,*,#8318,.F.);
#10933=ORIENTED_EDGE('',*,*,#8323,.F.);
#10934=ORIENTED_EDGE('',*,*,#8324,.F.);
#10935=ORIENTED_EDGE('',*,*,#8325,.F.);
#10936=ORIENTED_EDGE('',*,*,#8326,.F.);
#10937=ORIENTED_EDGE('',*,*,#8327,.T.);
#10938=ORIENTED_EDGE('',*,*,#8328,.T.);
#10939=ORIENTED_EDGE('',*,*,#8329,.T.);
#10940=ORIENTED_EDGE('',*,*,#8330,.T.);
#10941=ORIENTED_EDGE('',*,*,#8331,.T.);
#10942=ORIENTED_EDGE('',*,*,#8332,.T.);
#10943=ORIENTED_EDGE('',*,*,#8331,.F.);
#10944=ORIENTED_EDGE('',*,*,#8333,.T.);
#10945=ORIENTED_EDGE('',*,*,#8334,.T.);
#10946=ORIENTED_EDGE('',*,*,#8335,.T.);
#10947=ORIENTED_EDGE('',*,*,#8336,.T.);
#10948=ORIENTED_EDGE('',*,*,#8328,.F.);
#10949=ORIENTED_EDGE('',*,*,#8337,.T.);
#10950=ORIENTED_EDGE('',*,*,#8338,.T.);
#10951=ORIENTED_EDGE('',*,*,#8339,.T.);
#10952=ORIENTED_EDGE('',*,*,#8335,.F.);
#10953=ORIENTED_EDGE('',*,*,#8340,.T.);
#10954=ORIENTED_EDGE('',*,*,#8341,.T.);
#10955=ORIENTED_EDGE('',*,*,#8342,.T.);
#10956=ORIENTED_EDGE('',*,*,#8338,.F.);
#10957=ORIENTED_EDGE('',*,*,#8343,.T.);
#10958=ORIENTED_EDGE('',*,*,#8344,.T.);
#10959=ORIENTED_EDGE('',*,*,#8345,.T.);
#10960=ORIENTED_EDGE('',*,*,#8341,.F.);
#10961=ORIENTED_EDGE('',*,*,#8346,.T.);
#10962=ORIENTED_EDGE('',*,*,#8347,.T.);
#10963=ORIENTED_EDGE('',*,*,#8348,.T.);
#10964=ORIENTED_EDGE('',*,*,#8344,.F.);
#10965=ORIENTED_EDGE('',*,*,#8349,.T.);
#10966=ORIENTED_EDGE('',*,*,#8350,.T.);
#10967=ORIENTED_EDGE('',*,*,#8351,.T.);
#10968=ORIENTED_EDGE('',*,*,#8347,.F.);
#10969=ORIENTED_EDGE('',*,*,#8352,.T.);
#10970=ORIENTED_EDGE('',*,*,#8353,.T.);
#10971=ORIENTED_EDGE('',*,*,#8354,.T.);
#10972=ORIENTED_EDGE('',*,*,#8350,.F.);
#10973=ORIENTED_EDGE('',*,*,#8355,.T.);
#10974=ORIENTED_EDGE('',*,*,#8356,.T.);
#10975=ORIENTED_EDGE('',*,*,#8357,.T.);
#10976=ORIENTED_EDGE('',*,*,#8353,.F.);
#10977=ORIENTED_EDGE('',*,*,#8358,.T.);
#10978=ORIENTED_EDGE('',*,*,#8359,.T.);
#10979=ORIENTED_EDGE('',*,*,#8360,.T.);
#10980=ORIENTED_EDGE('',*,*,#8356,.F.);
#10981=ORIENTED_EDGE('',*,*,#8361,.T.);
#10982=ORIENTED_EDGE('',*,*,#8362,.T.);
#10983=ORIENTED_EDGE('',*,*,#8363,.T.);
#10984=ORIENTED_EDGE('',*,*,#8359,.F.);
#10985=ORIENTED_EDGE('',*,*,#8364,.T.);
#10986=ORIENTED_EDGE('',*,*,#8365,.T.);
#10987=ORIENTED_EDGE('',*,*,#8366,.T.);
#10988=ORIENTED_EDGE('',*,*,#8362,.F.);
#10989=ORIENTED_EDGE('',*,*,#8367,.T.);
#10990=ORIENTED_EDGE('',*,*,#8368,.T.);
#10991=ORIENTED_EDGE('',*,*,#8369,.T.);
#10992=ORIENTED_EDGE('',*,*,#8365,.F.);
#10993=ORIENTED_EDGE('',*,*,#8370,.T.);
#10994=ORIENTED_EDGE('',*,*,#8371,.T.);
#10995=ORIENTED_EDGE('',*,*,#8372,.T.);
#10996=ORIENTED_EDGE('',*,*,#8368,.F.);
#10997=ORIENTED_EDGE('',*,*,#8373,.T.);
#10998=ORIENTED_EDGE('',*,*,#8374,.T.);
#10999=ORIENTED_EDGE('',*,*,#8375,.T.);
#11000=ORIENTED_EDGE('',*,*,#8371,.F.);
#11001=ORIENTED_EDGE('',*,*,#8376,.T.);
#11002=ORIENTED_EDGE('',*,*,#8377,.T.);
#11003=ORIENTED_EDGE('',*,*,#8378,.T.);
#11004=ORIENTED_EDGE('',*,*,#8374,.F.);
#11005=ORIENTED_EDGE('',*,*,#8379,.T.);
#11006=ORIENTED_EDGE('',*,*,#8380,.T.);
#11007=ORIENTED_EDGE('',*,*,#8381,.T.);
#11008=ORIENTED_EDGE('',*,*,#8377,.F.);
#11009=ORIENTED_EDGE('',*,*,#8382,.T.);
#11010=ORIENTED_EDGE('',*,*,#8383,.F.);
#11011=ORIENTED_EDGE('',*,*,#8384,.T.);
#11012=ORIENTED_EDGE('',*,*,#8385,.F.);
#11013=ORIENTED_EDGE('',*,*,#8386,.T.);
#11014=ORIENTED_EDGE('',*,*,#8387,.T.);
#11015=ORIENTED_EDGE('',*,*,#8388,.T.);
#11016=ORIENTED_EDGE('',*,*,#8389,.F.);
#11017=ORIENTED_EDGE('',*,*,#8390,.F.);
#11018=ORIENTED_EDGE('',*,*,#8391,.T.);
#11019=ORIENTED_EDGE('',*,*,#8392,.T.);
#11020=ORIENTED_EDGE('',*,*,#8387,.F.);
#11021=ORIENTED_EDGE('',*,*,#8393,.F.);
#11022=ORIENTED_EDGE('',*,*,#8394,.T.);
#11023=ORIENTED_EDGE('',*,*,#8395,.T.);
#11024=ORIENTED_EDGE('',*,*,#8391,.F.);
#11025=ORIENTED_EDGE('',*,*,#8396,.F.);
#11026=ORIENTED_EDGE('',*,*,#8397,.T.);
#11027=ORIENTED_EDGE('',*,*,#8398,.T.);
#11028=ORIENTED_EDGE('',*,*,#8394,.F.);
#11029=ORIENTED_EDGE('',*,*,#8399,.F.);
#11030=ORIENTED_EDGE('',*,*,#8400,.T.);
#11031=ORIENTED_EDGE('',*,*,#8401,.T.);
#11032=ORIENTED_EDGE('',*,*,#8397,.F.);
#11033=ORIENTED_EDGE('',*,*,#8402,.F.);
#11034=ORIENTED_EDGE('',*,*,#8403,.T.);
#11035=ORIENTED_EDGE('',*,*,#8404,.T.);
#11036=ORIENTED_EDGE('',*,*,#8400,.F.);
#11037=ORIENTED_EDGE('',*,*,#8405,.F.);
#11038=ORIENTED_EDGE('',*,*,#8406,.T.);
#11039=ORIENTED_EDGE('',*,*,#8407,.T.);
#11040=ORIENTED_EDGE('',*,*,#8403,.F.);
#11041=ORIENTED_EDGE('',*,*,#8408,.F.);
#11042=ORIENTED_EDGE('',*,*,#8409,.T.);
#11043=ORIENTED_EDGE('',*,*,#8410,.T.);
#11044=ORIENTED_EDGE('',*,*,#8406,.F.);
#11045=ORIENTED_EDGE('',*,*,#8411,.F.);
#11046=ORIENTED_EDGE('',*,*,#8412,.T.);
#11047=ORIENTED_EDGE('',*,*,#8413,.T.);
#11048=ORIENTED_EDGE('',*,*,#8409,.F.);
#11049=ORIENTED_EDGE('',*,*,#8414,.F.);
#11050=ORIENTED_EDGE('',*,*,#8415,.T.);
#11051=ORIENTED_EDGE('',*,*,#8416,.T.);
#11052=ORIENTED_EDGE('',*,*,#8412,.F.);
#11053=ORIENTED_EDGE('',*,*,#8417,.F.);
#11054=ORIENTED_EDGE('',*,*,#8418,.T.);
#11055=ORIENTED_EDGE('',*,*,#8419,.T.);
#11056=ORIENTED_EDGE('',*,*,#8415,.F.);
#11057=ORIENTED_EDGE('',*,*,#8420,.F.);
#11058=ORIENTED_EDGE('',*,*,#8421,.T.);
#11059=ORIENTED_EDGE('',*,*,#8422,.T.);
#11060=ORIENTED_EDGE('',*,*,#8418,.F.);
#11061=ORIENTED_EDGE('',*,*,#8423,.F.);
#11062=ORIENTED_EDGE('',*,*,#8424,.T.);
#11063=ORIENTED_EDGE('',*,*,#8425,.T.);
#11064=ORIENTED_EDGE('',*,*,#8421,.F.);
#11065=ORIENTED_EDGE('',*,*,#8426,.F.);
#11066=ORIENTED_EDGE('',*,*,#8427,.T.);
#11067=ORIENTED_EDGE('',*,*,#8428,.T.);
#11068=ORIENTED_EDGE('',*,*,#8424,.F.);
#11069=ORIENTED_EDGE('',*,*,#8429,.F.);
#11070=ORIENTED_EDGE('',*,*,#8430,.T.);
#11071=ORIENTED_EDGE('',*,*,#8431,.T.);
#11072=ORIENTED_EDGE('',*,*,#8427,.F.);
#11073=ORIENTED_EDGE('',*,*,#8432,.F.);
#11074=ORIENTED_EDGE('',*,*,#8433,.T.);
#11075=ORIENTED_EDGE('',*,*,#8434,.T.);
#11076=ORIENTED_EDGE('',*,*,#8430,.F.);
#11077=ORIENTED_EDGE('',*,*,#8435,.F.);
#11078=ORIENTED_EDGE('',*,*,#8436,.T.);
#11079=ORIENTED_EDGE('',*,*,#8437,.T.);
#11080=ORIENTED_EDGE('',*,*,#8433,.F.);
#11081=ORIENTED_EDGE('',*,*,#8438,.F.);
#11082=ORIENTED_EDGE('',*,*,#8439,.T.);
#11083=ORIENTED_EDGE('',*,*,#8440,.T.);
#11084=ORIENTED_EDGE('',*,*,#8436,.F.);
#11085=ORIENTED_EDGE('',*,*,#8441,.F.);
#11086=ORIENTED_EDGE('',*,*,#8442,.F.);
#11087=ORIENTED_EDGE('',*,*,#8443,.F.);
#11088=ORIENTED_EDGE('',*,*,#8444,.F.);
#11089=ORIENTED_EDGE('',*,*,#8445,.T.);
#11090=ORIENTED_EDGE('',*,*,#8446,.T.);
#11091=ORIENTED_EDGE('',*,*,#8447,.T.);
#11092=ORIENTED_EDGE('',*,*,#8448,.T.);
#11093=ORIENTED_EDGE('',*,*,#8449,.T.);
#11094=ORIENTED_EDGE('',*,*,#8450,.T.);
#11095=ORIENTED_EDGE('',*,*,#8449,.F.);
#11096=ORIENTED_EDGE('',*,*,#8451,.T.);
#11097=ORIENTED_EDGE('',*,*,#8452,.T.);
#11098=ORIENTED_EDGE('',*,*,#8453,.T.);
#11099=ORIENTED_EDGE('',*,*,#8454,.T.);
#11100=ORIENTED_EDGE('',*,*,#8446,.F.);
#11101=ORIENTED_EDGE('',*,*,#8455,.T.);
#11102=ORIENTED_EDGE('',*,*,#8456,.T.);
#11103=ORIENTED_EDGE('',*,*,#8457,.T.);
#11104=ORIENTED_EDGE('',*,*,#8453,.F.);
#11105=ORIENTED_EDGE('',*,*,#8458,.T.);
#11106=ORIENTED_EDGE('',*,*,#8459,.T.);
#11107=ORIENTED_EDGE('',*,*,#8460,.T.);
#11108=ORIENTED_EDGE('',*,*,#8456,.F.);
#11109=ORIENTED_EDGE('',*,*,#8461,.T.);
#11110=ORIENTED_EDGE('',*,*,#8462,.T.);
#11111=ORIENTED_EDGE('',*,*,#8463,.T.);
#11112=ORIENTED_EDGE('',*,*,#8459,.F.);
#11113=ORIENTED_EDGE('',*,*,#8464,.T.);
#11114=ORIENTED_EDGE('',*,*,#8465,.T.);
#11115=ORIENTED_EDGE('',*,*,#8466,.T.);
#11116=ORIENTED_EDGE('',*,*,#8462,.F.);
#11117=ORIENTED_EDGE('',*,*,#8467,.T.);
#11118=ORIENTED_EDGE('',*,*,#8468,.T.);
#11119=ORIENTED_EDGE('',*,*,#8469,.T.);
#11120=ORIENTED_EDGE('',*,*,#8465,.F.);
#11121=ORIENTED_EDGE('',*,*,#8470,.T.);
#11122=ORIENTED_EDGE('',*,*,#8471,.T.);
#11123=ORIENTED_EDGE('',*,*,#8472,.T.);
#11124=ORIENTED_EDGE('',*,*,#8468,.F.);
#11125=ORIENTED_EDGE('',*,*,#8473,.T.);
#11126=ORIENTED_EDGE('',*,*,#8474,.T.);
#11127=ORIENTED_EDGE('',*,*,#8475,.T.);
#11128=ORIENTED_EDGE('',*,*,#8471,.F.);
#11129=ORIENTED_EDGE('',*,*,#8476,.T.);
#11130=ORIENTED_EDGE('',*,*,#8477,.T.);
#11131=ORIENTED_EDGE('',*,*,#8478,.T.);
#11132=ORIENTED_EDGE('',*,*,#8474,.F.);
#11133=ORIENTED_EDGE('',*,*,#8479,.T.);
#11134=ORIENTED_EDGE('',*,*,#8480,.T.);
#11135=ORIENTED_EDGE('',*,*,#8481,.T.);
#11136=ORIENTED_EDGE('',*,*,#8477,.F.);
#11137=ORIENTED_EDGE('',*,*,#8482,.T.);
#11138=ORIENTED_EDGE('',*,*,#8483,.T.);
#11139=ORIENTED_EDGE('',*,*,#8484,.T.);
#11140=ORIENTED_EDGE('',*,*,#8480,.F.);
#11141=ORIENTED_EDGE('',*,*,#8485,.T.);
#11142=ORIENTED_EDGE('',*,*,#8486,.T.);
#11143=ORIENTED_EDGE('',*,*,#8487,.T.);
#11144=ORIENTED_EDGE('',*,*,#8483,.F.);
#11145=ORIENTED_EDGE('',*,*,#8488,.T.);
#11146=ORIENTED_EDGE('',*,*,#8489,.T.);
#11147=ORIENTED_EDGE('',*,*,#8490,.T.);
#11148=ORIENTED_EDGE('',*,*,#8486,.F.);
#11149=ORIENTED_EDGE('',*,*,#8491,.T.);
#11150=ORIENTED_EDGE('',*,*,#8492,.T.);
#11151=ORIENTED_EDGE('',*,*,#8493,.T.);
#11152=ORIENTED_EDGE('',*,*,#8489,.F.);
#11153=ORIENTED_EDGE('',*,*,#8494,.T.);
#11154=ORIENTED_EDGE('',*,*,#8495,.T.);
#11155=ORIENTED_EDGE('',*,*,#8496,.T.);
#11156=ORIENTED_EDGE('',*,*,#8492,.F.);
#11157=ORIENTED_EDGE('',*,*,#8497,.T.);
#11158=ORIENTED_EDGE('',*,*,#8498,.T.);
#11159=ORIENTED_EDGE('',*,*,#8499,.T.);
#11160=ORIENTED_EDGE('',*,*,#8495,.F.);
#11161=ORIENTED_EDGE('',*,*,#8500,.T.);
#11162=ORIENTED_EDGE('',*,*,#8501,.F.);
#11163=ORIENTED_EDGE('',*,*,#8502,.T.);
#11164=ORIENTED_EDGE('',*,*,#8503,.F.);
#11165=ORIENTED_EDGE('',*,*,#8504,.T.);
#11166=ORIENTED_EDGE('',*,*,#8505,.T.);
#11167=ORIENTED_EDGE('',*,*,#8506,.T.);
#11168=ORIENTED_EDGE('',*,*,#8507,.F.);
#11169=ORIENTED_EDGE('',*,*,#8508,.F.);
#11170=ORIENTED_EDGE('',*,*,#8509,.T.);
#11171=ORIENTED_EDGE('',*,*,#8510,.T.);
#11172=ORIENTED_EDGE('',*,*,#8505,.F.);
#11173=ORIENTED_EDGE('',*,*,#8511,.F.);
#11174=ORIENTED_EDGE('',*,*,#8512,.T.);
#11175=ORIENTED_EDGE('',*,*,#8513,.T.);
#11176=ORIENTED_EDGE('',*,*,#8509,.F.);
#11177=ORIENTED_EDGE('',*,*,#8514,.F.);
#11178=ORIENTED_EDGE('',*,*,#8515,.T.);
#11179=ORIENTED_EDGE('',*,*,#8516,.T.);
#11180=ORIENTED_EDGE('',*,*,#8512,.F.);
#11181=ORIENTED_EDGE('',*,*,#8517,.F.);
#11182=ORIENTED_EDGE('',*,*,#8518,.T.);
#11183=ORIENTED_EDGE('',*,*,#8519,.T.);
#11184=ORIENTED_EDGE('',*,*,#8515,.F.);
#11185=ORIENTED_EDGE('',*,*,#8520,.F.);
#11186=ORIENTED_EDGE('',*,*,#8521,.T.);
#11187=ORIENTED_EDGE('',*,*,#8522,.T.);
#11188=ORIENTED_EDGE('',*,*,#8518,.F.);
#11189=ORIENTED_EDGE('',*,*,#8523,.F.);
#11190=ORIENTED_EDGE('',*,*,#8524,.T.);
#11191=ORIENTED_EDGE('',*,*,#8525,.T.);
#11192=ORIENTED_EDGE('',*,*,#8521,.F.);
#11193=ORIENTED_EDGE('',*,*,#8526,.F.);
#11194=ORIENTED_EDGE('',*,*,#8527,.T.);
#11195=ORIENTED_EDGE('',*,*,#8528,.T.);
#11196=ORIENTED_EDGE('',*,*,#8524,.F.);
#11197=ORIENTED_EDGE('',*,*,#8529,.F.);
#11198=ORIENTED_EDGE('',*,*,#8530,.T.);
#11199=ORIENTED_EDGE('',*,*,#8531,.T.);
#11200=ORIENTED_EDGE('',*,*,#8527,.F.);
#11201=ORIENTED_EDGE('',*,*,#8532,.F.);
#11202=ORIENTED_EDGE('',*,*,#8533,.T.);
#11203=ORIENTED_EDGE('',*,*,#8534,.T.);
#11204=ORIENTED_EDGE('',*,*,#8530,.F.);
#11205=ORIENTED_EDGE('',*,*,#8535,.F.);
#11206=ORIENTED_EDGE('',*,*,#8536,.T.);
#11207=ORIENTED_EDGE('',*,*,#8537,.T.);
#11208=ORIENTED_EDGE('',*,*,#8533,.F.);
#11209=ORIENTED_EDGE('',*,*,#8538,.F.);
#11210=ORIENTED_EDGE('',*,*,#8539,.T.);
#11211=ORIENTED_EDGE('',*,*,#8540,.T.);
#11212=ORIENTED_EDGE('',*,*,#8536,.F.);
#11213=ORIENTED_EDGE('',*,*,#8541,.F.);
#11214=ORIENTED_EDGE('',*,*,#8542,.T.);
#11215=ORIENTED_EDGE('',*,*,#8543,.T.);
#11216=ORIENTED_EDGE('',*,*,#8539,.F.);
#11217=ORIENTED_EDGE('',*,*,#8544,.F.);
#11218=ORIENTED_EDGE('',*,*,#8545,.T.);
#11219=ORIENTED_EDGE('',*,*,#8546,.T.);
#11220=ORIENTED_EDGE('',*,*,#8542,.F.);
#11221=ORIENTED_EDGE('',*,*,#8547,.F.);
#11222=ORIENTED_EDGE('',*,*,#8548,.T.);
#11223=ORIENTED_EDGE('',*,*,#8549,.T.);
#11224=ORIENTED_EDGE('',*,*,#8545,.F.);
#11225=ORIENTED_EDGE('',*,*,#8550,.F.);
#11226=ORIENTED_EDGE('',*,*,#8551,.T.);
#11227=ORIENTED_EDGE('',*,*,#8552,.T.);
#11228=ORIENTED_EDGE('',*,*,#8548,.F.);
#11229=ORIENTED_EDGE('',*,*,#8553,.F.);
#11230=ORIENTED_EDGE('',*,*,#8554,.T.);
#11231=ORIENTED_EDGE('',*,*,#8555,.T.);
#11232=ORIENTED_EDGE('',*,*,#8551,.F.);
#11233=ORIENTED_EDGE('',*,*,#8556,.F.);
#11234=ORIENTED_EDGE('',*,*,#8557,.T.);
#11235=ORIENTED_EDGE('',*,*,#8558,.T.);
#11236=ORIENTED_EDGE('',*,*,#8554,.F.);
#11237=ORIENTED_EDGE('',*,*,#8559,.F.);
#11238=ORIENTED_EDGE('',*,*,#8560,.F.);
#11239=ORIENTED_EDGE('',*,*,#8561,.F.);
#11240=ORIENTED_EDGE('',*,*,#8562,.F.);
#11241=ORIENTED_EDGE('',*,*,#8563,.T.);
#11242=ORIENTED_EDGE('',*,*,#8448,.F.);
#11243=ORIENTED_EDGE('',*,*,#8564,.T.);
#11244=ORIENTED_EDGE('',*,*,#8507,.T.);
#11245=ORIENTED_EDGE('',*,*,#8565,.T.);
#11246=ORIENTED_EDGE('',*,*,#8451,.F.);
#11247=ORIENTED_EDGE('',*,*,#8560,.T.);
#11248=ORIENTED_EDGE('',*,*,#8566,.T.);
#11249=ORIENTED_EDGE('',*,*,#8557,.F.);
#11250=ORIENTED_EDGE('',*,*,#8567,.F.);
#11251=ORIENTED_EDGE('',*,*,#8565,.F.);
#11252=ORIENTED_EDGE('',*,*,#8506,.F.);
#11253=ORIENTED_EDGE('',*,*,#8510,.F.);
#11254=ORIENTED_EDGE('',*,*,#8513,.F.);
#11255=ORIENTED_EDGE('',*,*,#8516,.F.);
#11256=ORIENTED_EDGE('',*,*,#8519,.F.);
#11257=ORIENTED_EDGE('',*,*,#8522,.F.);
#11258=ORIENTED_EDGE('',*,*,#8525,.F.);
#11259=ORIENTED_EDGE('',*,*,#8528,.F.);
#11260=ORIENTED_EDGE('',*,*,#8531,.F.);
#11261=ORIENTED_EDGE('',*,*,#8534,.F.);
#11262=ORIENTED_EDGE('',*,*,#8537,.F.);
#11263=ORIENTED_EDGE('',*,*,#8540,.F.);
#11264=ORIENTED_EDGE('',*,*,#8543,.F.);
#11265=ORIENTED_EDGE('',*,*,#8546,.F.);
#11266=ORIENTED_EDGE('',*,*,#8549,.F.);
#11267=ORIENTED_EDGE('',*,*,#8552,.F.);
#11268=ORIENTED_EDGE('',*,*,#8555,.F.);
#11269=ORIENTED_EDGE('',*,*,#8558,.F.);
#11270=ORIENTED_EDGE('',*,*,#8566,.F.);
#11271=ORIENTED_EDGE('',*,*,#8563,.F.);
#11272=ORIENTED_EDGE('',*,*,#8568,.F.);
#11273=ORIENTED_EDGE('',*,*,#8502,.F.);
#11274=ORIENTED_EDGE('',*,*,#8569,.F.);
#11275=ORIENTED_EDGE('',*,*,#8500,.F.);
#11276=ORIENTED_EDGE('',*,*,#8497,.F.);
#11277=ORIENTED_EDGE('',*,*,#8494,.F.);
#11278=ORIENTED_EDGE('',*,*,#8491,.F.);
#11279=ORIENTED_EDGE('',*,*,#8488,.F.);
#11280=ORIENTED_EDGE('',*,*,#8485,.F.);
#11281=ORIENTED_EDGE('',*,*,#8482,.F.);
#11282=ORIENTED_EDGE('',*,*,#8479,.F.);
#11283=ORIENTED_EDGE('',*,*,#8476,.F.);
#11284=ORIENTED_EDGE('',*,*,#8473,.F.);
#11285=ORIENTED_EDGE('',*,*,#8470,.F.);
#11286=ORIENTED_EDGE('',*,*,#8467,.F.);
#11287=ORIENTED_EDGE('',*,*,#8464,.F.);
#11288=ORIENTED_EDGE('',*,*,#8461,.F.);
#11289=ORIENTED_EDGE('',*,*,#8458,.F.);
#11290=ORIENTED_EDGE('',*,*,#8455,.F.);
#11291=ORIENTED_EDGE('',*,*,#8452,.F.);
#11292=ORIENTED_EDGE('',*,*,#8564,.F.);
#11293=ORIENTED_EDGE('',*,*,#8447,.F.);
#11294=ORIENTED_EDGE('',*,*,#8454,.F.);
#11295=ORIENTED_EDGE('',*,*,#8457,.F.);
#11296=ORIENTED_EDGE('',*,*,#8460,.F.);
#11297=ORIENTED_EDGE('',*,*,#8463,.F.);
#11298=ORIENTED_EDGE('',*,*,#8466,.F.);
#11299=ORIENTED_EDGE('',*,*,#8469,.F.);
#11300=ORIENTED_EDGE('',*,*,#8472,.F.);
#11301=ORIENTED_EDGE('',*,*,#8475,.F.);
#11302=ORIENTED_EDGE('',*,*,#8478,.F.);
#11303=ORIENTED_EDGE('',*,*,#8481,.F.);
#11304=ORIENTED_EDGE('',*,*,#8484,.F.);
#11305=ORIENTED_EDGE('',*,*,#8487,.F.);
#11306=ORIENTED_EDGE('',*,*,#8490,.F.);
#11307=ORIENTED_EDGE('',*,*,#8493,.F.);
#11308=ORIENTED_EDGE('',*,*,#8496,.F.);
#11309=ORIENTED_EDGE('',*,*,#8499,.F.);
#11310=ORIENTED_EDGE('',*,*,#8570,.F.);
#11311=ORIENTED_EDGE('',*,*,#8504,.F.);
#11312=ORIENTED_EDGE('',*,*,#8571,.F.);
#11313=ORIENTED_EDGE('',*,*,#8561,.T.);
#11314=ORIENTED_EDGE('',*,*,#8567,.T.);
#11315=ORIENTED_EDGE('',*,*,#8559,.T.);
#11316=ORIENTED_EDGE('',*,*,#8556,.T.);
#11317=ORIENTED_EDGE('',*,*,#8553,.T.);
#11318=ORIENTED_EDGE('',*,*,#8550,.T.);
#11319=ORIENTED_EDGE('',*,*,#8547,.T.);
#11320=ORIENTED_EDGE('',*,*,#8544,.T.);
#11321=ORIENTED_EDGE('',*,*,#8541,.T.);
#11322=ORIENTED_EDGE('',*,*,#8538,.T.);
#11323=ORIENTED_EDGE('',*,*,#8535,.T.);
#11324=ORIENTED_EDGE('',*,*,#8532,.T.);
#11325=ORIENTED_EDGE('',*,*,#8529,.T.);
#11326=ORIENTED_EDGE('',*,*,#8526,.T.);
#11327=ORIENTED_EDGE('',*,*,#8523,.T.);
#11328=ORIENTED_EDGE('',*,*,#8520,.T.);
#11329=ORIENTED_EDGE('',*,*,#8517,.T.);
#11330=ORIENTED_EDGE('',*,*,#8514,.T.);
#11331=ORIENTED_EDGE('',*,*,#8511,.T.);
#11332=ORIENTED_EDGE('',*,*,#8508,.T.);
#11333=ORIENTED_EDGE('',*,*,#8501,.T.);
#11334=ORIENTED_EDGE('',*,*,#8570,.T.);
#11335=ORIENTED_EDGE('',*,*,#8498,.F.);
#11336=ORIENTED_EDGE('',*,*,#8569,.T.);
#11337=ORIENTED_EDGE('',*,*,#8330,.F.);
#11338=ORIENTED_EDGE('',*,*,#8572,.T.);
#11339=ORIENTED_EDGE('',*,*,#8389,.T.);
#11340=ORIENTED_EDGE('',*,*,#8573,.T.);
#11341=ORIENTED_EDGE('',*,*,#8333,.F.);
#11342=ORIENTED_EDGE('',*,*,#8442,.T.);
#11343=ORIENTED_EDGE('',*,*,#8574,.T.);
#11344=ORIENTED_EDGE('',*,*,#8439,.F.);
#11345=ORIENTED_EDGE('',*,*,#8575,.F.);
#11346=ORIENTED_EDGE('',*,*,#8573,.F.);
#11347=ORIENTED_EDGE('',*,*,#8388,.F.);
#11348=ORIENTED_EDGE('',*,*,#8392,.F.);
#11349=ORIENTED_EDGE('',*,*,#8395,.F.);
#11350=ORIENTED_EDGE('',*,*,#8398,.F.);
#11351=ORIENTED_EDGE('',*,*,#8401,.F.);
#11352=ORIENTED_EDGE('',*,*,#8404,.F.);
#11353=ORIENTED_EDGE('',*,*,#8407,.F.);
#11354=ORIENTED_EDGE('',*,*,#8410,.F.);
#11355=ORIENTED_EDGE('',*,*,#8413,.F.);
#11356=ORIENTED_EDGE('',*,*,#8416,.F.);
#11357=ORIENTED_EDGE('',*,*,#8419,.F.);
#11358=ORIENTED_EDGE('',*,*,#8422,.F.);
#11359=ORIENTED_EDGE('',*,*,#8425,.F.);
#11360=ORIENTED_EDGE('',*,*,#8428,.F.);
#11361=ORIENTED_EDGE('',*,*,#8431,.F.);
#11362=ORIENTED_EDGE('',*,*,#8434,.F.);
#11363=ORIENTED_EDGE('',*,*,#8437,.F.);
#11364=ORIENTED_EDGE('',*,*,#8440,.F.);
#11365=ORIENTED_EDGE('',*,*,#8574,.F.);
#11366=ORIENTED_EDGE('',*,*,#8445,.F.);
#11367=ORIENTED_EDGE('',*,*,#8576,.F.);
#11368=ORIENTED_EDGE('',*,*,#8384,.F.);
#11369=ORIENTED_EDGE('',*,*,#8577,.F.);
#11370=ORIENTED_EDGE('',*,*,#8382,.F.);
#11371=ORIENTED_EDGE('',*,*,#8379,.F.);
#11372=ORIENTED_EDGE('',*,*,#8376,.F.);
#11373=ORIENTED_EDGE('',*,*,#8373,.F.);
#11374=ORIENTED_EDGE('',*,*,#8370,.F.);
#11375=ORIENTED_EDGE('',*,*,#8367,.F.);
#11376=ORIENTED_EDGE('',*,*,#8364,.F.);
#11377=ORIENTED_EDGE('',*,*,#8361,.F.);
#11378=ORIENTED_EDGE('',*,*,#8358,.F.);
#11379=ORIENTED_EDGE('',*,*,#8355,.F.);
#11380=ORIENTED_EDGE('',*,*,#8352,.F.);
#11381=ORIENTED_EDGE('',*,*,#8349,.F.);
#11382=ORIENTED_EDGE('',*,*,#8346,.F.);
#11383=ORIENTED_EDGE('',*,*,#8343,.F.);
#11384=ORIENTED_EDGE('',*,*,#8340,.F.);
#11385=ORIENTED_EDGE('',*,*,#8337,.F.);
#11386=ORIENTED_EDGE('',*,*,#8334,.F.);
#11387=ORIENTED_EDGE('',*,*,#8572,.F.);
#11388=ORIENTED_EDGE('',*,*,#8329,.F.);
#11389=ORIENTED_EDGE('',*,*,#8336,.F.);
#11390=ORIENTED_EDGE('',*,*,#8339,.F.);
#11391=ORIENTED_EDGE('',*,*,#8342,.F.);
#11392=ORIENTED_EDGE('',*,*,#8345,.F.);
#11393=ORIENTED_EDGE('',*,*,#8348,.F.);
#11394=ORIENTED_EDGE('',*,*,#8351,.F.);
#11395=ORIENTED_EDGE('',*,*,#8354,.F.);
#11396=ORIENTED_EDGE('',*,*,#8357,.F.);
#11397=ORIENTED_EDGE('',*,*,#8360,.F.);
#11398=ORIENTED_EDGE('',*,*,#8363,.F.);
#11399=ORIENTED_EDGE('',*,*,#8366,.F.);
#11400=ORIENTED_EDGE('',*,*,#8369,.F.);
#11401=ORIENTED_EDGE('',*,*,#8372,.F.);
#11402=ORIENTED_EDGE('',*,*,#8375,.F.);
#11403=ORIENTED_EDGE('',*,*,#8378,.F.);
#11404=ORIENTED_EDGE('',*,*,#8381,.F.);
#11405=ORIENTED_EDGE('',*,*,#8578,.F.);
#11406=ORIENTED_EDGE('',*,*,#8386,.F.);
#11407=ORIENTED_EDGE('',*,*,#8579,.F.);
#11408=ORIENTED_EDGE('',*,*,#8443,.T.);
#11409=ORIENTED_EDGE('',*,*,#8575,.T.);
#11410=ORIENTED_EDGE('',*,*,#8441,.T.);
#11411=ORIENTED_EDGE('',*,*,#8438,.T.);
#11412=ORIENTED_EDGE('',*,*,#8435,.T.);
#11413=ORIENTED_EDGE('',*,*,#8432,.T.);
#11414=ORIENTED_EDGE('',*,*,#8429,.T.);
#11415=ORIENTED_EDGE('',*,*,#8426,.T.);
#11416=ORIENTED_EDGE('',*,*,#8423,.T.);
#11417=ORIENTED_EDGE('',*,*,#8420,.T.);
#11418=ORIENTED_EDGE('',*,*,#8417,.T.);
#11419=ORIENTED_EDGE('',*,*,#8414,.T.);
#11420=ORIENTED_EDGE('',*,*,#8411,.T.);
#11421=ORIENTED_EDGE('',*,*,#8408,.T.);
#11422=ORIENTED_EDGE('',*,*,#8405,.T.);
#11423=ORIENTED_EDGE('',*,*,#8402,.T.);
#11424=ORIENTED_EDGE('',*,*,#8399,.T.);
#11425=ORIENTED_EDGE('',*,*,#8396,.T.);
#11426=ORIENTED_EDGE('',*,*,#8393,.T.);
#11427=ORIENTED_EDGE('',*,*,#8390,.T.);
#11428=ORIENTED_EDGE('',*,*,#8383,.T.);
#11429=ORIENTED_EDGE('',*,*,#8578,.T.);
#11430=ORIENTED_EDGE('',*,*,#8380,.F.);
#11431=ORIENTED_EDGE('',*,*,#8577,.T.);
#11432=ORIENTED_EDGE('',*,*,#8212,.F.);
#11433=ORIENTED_EDGE('',*,*,#8580,.T.);
#11434=ORIENTED_EDGE('',*,*,#8271,.T.);
#11435=ORIENTED_EDGE('',*,*,#8581,.T.);
#11436=ORIENTED_EDGE('',*,*,#8215,.F.);
#11437=ORIENTED_EDGE('',*,*,#8324,.T.);
#11438=ORIENTED_EDGE('',*,*,#8582,.T.);
#11439=ORIENTED_EDGE('',*,*,#8321,.F.);
#11440=ORIENTED_EDGE('',*,*,#8583,.F.);
#11441=ORIENTED_EDGE('',*,*,#8581,.F.);
#11442=ORIENTED_EDGE('',*,*,#8270,.F.);
#11443=ORIENTED_EDGE('',*,*,#8274,.F.);
#11444=ORIENTED_EDGE('',*,*,#8277,.F.);
#11445=ORIENTED_EDGE('',*,*,#8280,.F.);
#11446=ORIENTED_EDGE('',*,*,#8283,.F.);
#11447=ORIENTED_EDGE('',*,*,#8286,.F.);
#11448=ORIENTED_EDGE('',*,*,#8289,.F.);
#11449=ORIENTED_EDGE('',*,*,#8292,.F.);
#11450=ORIENTED_EDGE('',*,*,#8295,.F.);
#11451=ORIENTED_EDGE('',*,*,#8298,.F.);
#11452=ORIENTED_EDGE('',*,*,#8301,.F.);
#11453=ORIENTED_EDGE('',*,*,#8304,.F.);
#11454=ORIENTED_EDGE('',*,*,#8307,.F.);
#11455=ORIENTED_EDGE('',*,*,#8310,.F.);
#11456=ORIENTED_EDGE('',*,*,#8313,.F.);
#11457=ORIENTED_EDGE('',*,*,#8316,.F.);
#11458=ORIENTED_EDGE('',*,*,#8319,.F.);
#11459=ORIENTED_EDGE('',*,*,#8322,.F.);
#11460=ORIENTED_EDGE('',*,*,#8582,.F.);
#11461=ORIENTED_EDGE('',*,*,#8327,.F.);
#11462=ORIENTED_EDGE('',*,*,#8584,.F.);
#11463=ORIENTED_EDGE('',*,*,#8266,.F.);
#11464=ORIENTED_EDGE('',*,*,#8585,.F.);
#11465=ORIENTED_EDGE('',*,*,#8264,.F.);
#11466=ORIENTED_EDGE('',*,*,#8261,.F.);
#11467=ORIENTED_EDGE('',*,*,#8258,.F.);
#11468=ORIENTED_EDGE('',*,*,#8255,.F.);
#11469=ORIENTED_EDGE('',*,*,#8252,.F.);
#11470=ORIENTED_EDGE('',*,*,#8249,.F.);
#11471=ORIENTED_EDGE('',*,*,#8246,.F.);
#11472=ORIENTED_EDGE('',*,*,#8243,.F.);
#11473=ORIENTED_EDGE('',*,*,#8240,.F.);
#11474=ORIENTED_EDGE('',*,*,#8237,.F.);
#11475=ORIENTED_EDGE('',*,*,#8234,.F.);
#11476=ORIENTED_EDGE('',*,*,#8231,.F.);
#11477=ORIENTED_EDGE('',*,*,#8228,.F.);
#11478=ORIENTED_EDGE('',*,*,#8225,.F.);
#11479=ORIENTED_EDGE('',*,*,#8222,.F.);
#11480=ORIENTED_EDGE('',*,*,#8219,.F.);
#11481=ORIENTED_EDGE('',*,*,#8216,.F.);
#11482=ORIENTED_EDGE('',*,*,#8580,.F.);
#11483=ORIENTED_EDGE('',*,*,#8211,.F.);
#11484=ORIENTED_EDGE('',*,*,#8218,.F.);
#11485=ORIENTED_EDGE('',*,*,#8221,.F.);
#11486=ORIENTED_EDGE('',*,*,#8224,.F.);
#11487=ORIENTED_EDGE('',*,*,#8227,.F.);
#11488=ORIENTED_EDGE('',*,*,#8230,.F.);
#11489=ORIENTED_EDGE('',*,*,#8233,.F.);
#11490=ORIENTED_EDGE('',*,*,#8236,.F.);
#11491=ORIENTED_EDGE('',*,*,#8239,.F.);
#11492=ORIENTED_EDGE('',*,*,#8242,.F.);
#11493=ORIENTED_EDGE('',*,*,#8245,.F.);
#11494=ORIENTED_EDGE('',*,*,#8248,.F.);
#11495=ORIENTED_EDGE('',*,*,#8251,.F.);
#11496=ORIENTED_EDGE('',*,*,#8254,.F.);
#11497=ORIENTED_EDGE('',*,*,#8257,.F.);
#11498=ORIENTED_EDGE('',*,*,#8260,.F.);
#11499=ORIENTED_EDGE('',*,*,#8263,.F.);
#11500=ORIENTED_EDGE('',*,*,#8586,.F.);
#11501=ORIENTED_EDGE('',*,*,#8268,.F.);
#11502=ORIENTED_EDGE('',*,*,#8587,.F.);
#11503=ORIENTED_EDGE('',*,*,#8325,.T.);
#11504=ORIENTED_EDGE('',*,*,#8583,.T.);
#11505=ORIENTED_EDGE('',*,*,#8323,.T.);
#11506=ORIENTED_EDGE('',*,*,#8320,.T.);
#11507=ORIENTED_EDGE('',*,*,#8317,.T.);
#11508=ORIENTED_EDGE('',*,*,#8314,.T.);
#11509=ORIENTED_EDGE('',*,*,#8311,.T.);
#11510=ORIENTED_EDGE('',*,*,#8308,.T.);
#11511=ORIENTED_EDGE('',*,*,#8305,.T.);
#11512=ORIENTED_EDGE('',*,*,#8302,.T.);
#11513=ORIENTED_EDGE('',*,*,#8299,.T.);
#11514=ORIENTED_EDGE('',*,*,#8296,.T.);
#11515=ORIENTED_EDGE('',*,*,#8293,.T.);
#11516=ORIENTED_EDGE('',*,*,#8290,.T.);
#11517=ORIENTED_EDGE('',*,*,#8287,.T.);
#11518=ORIENTED_EDGE('',*,*,#8284,.T.);
#11519=ORIENTED_EDGE('',*,*,#8281,.T.);
#11520=ORIENTED_EDGE('',*,*,#8278,.T.);
#11521=ORIENTED_EDGE('',*,*,#8275,.T.);
#11522=ORIENTED_EDGE('',*,*,#8272,.T.);
#11523=ORIENTED_EDGE('',*,*,#8265,.T.);
#11524=ORIENTED_EDGE('',*,*,#8586,.T.);
#11525=ORIENTED_EDGE('',*,*,#8262,.F.);
#11526=ORIENTED_EDGE('',*,*,#8585,.T.);
#11527=ORIENTED_EDGE('',*,*,#8094,.F.);
#11528=ORIENTED_EDGE('',*,*,#8588,.T.);
#11529=ORIENTED_EDGE('',*,*,#8153,.T.);
#11530=ORIENTED_EDGE('',*,*,#8589,.T.);
#11531=ORIENTED_EDGE('',*,*,#8097,.F.);
#11532=ORIENTED_EDGE('',*,*,#8206,.T.);
#11533=ORIENTED_EDGE('',*,*,#8590,.T.);
#11534=ORIENTED_EDGE('',*,*,#8203,.F.);
#11535=ORIENTED_EDGE('',*,*,#8591,.F.);
#11536=ORIENTED_EDGE('',*,*,#8589,.F.);
#11537=ORIENTED_EDGE('',*,*,#8152,.F.);
#11538=ORIENTED_EDGE('',*,*,#8156,.F.);
#11539=ORIENTED_EDGE('',*,*,#8159,.F.);
#11540=ORIENTED_EDGE('',*,*,#8162,.F.);
#11541=ORIENTED_EDGE('',*,*,#8165,.F.);
#11542=ORIENTED_EDGE('',*,*,#8168,.F.);
#11543=ORIENTED_EDGE('',*,*,#8171,.F.);
#11544=ORIENTED_EDGE('',*,*,#8174,.F.);
#11545=ORIENTED_EDGE('',*,*,#8177,.F.);
#11546=ORIENTED_EDGE('',*,*,#8180,.F.);
#11547=ORIENTED_EDGE('',*,*,#8183,.F.);
#11548=ORIENTED_EDGE('',*,*,#8186,.F.);
#11549=ORIENTED_EDGE('',*,*,#8189,.F.);
#11550=ORIENTED_EDGE('',*,*,#8192,.F.);
#11551=ORIENTED_EDGE('',*,*,#8195,.F.);
#11552=ORIENTED_EDGE('',*,*,#8198,.F.);
#11553=ORIENTED_EDGE('',*,*,#8201,.F.);
#11554=ORIENTED_EDGE('',*,*,#8204,.F.);
#11555=ORIENTED_EDGE('',*,*,#8590,.F.);
#11556=ORIENTED_EDGE('',*,*,#8209,.F.);
#11557=ORIENTED_EDGE('',*,*,#8592,.F.);
#11558=ORIENTED_EDGE('',*,*,#8148,.F.);
#11559=ORIENTED_EDGE('',*,*,#8593,.F.);
#11560=ORIENTED_EDGE('',*,*,#8146,.F.);
#11561=ORIENTED_EDGE('',*,*,#8143,.F.);
#11562=ORIENTED_EDGE('',*,*,#8140,.F.);
#11563=ORIENTED_EDGE('',*,*,#8137,.F.);
#11564=ORIENTED_EDGE('',*,*,#8134,.F.);
#11565=ORIENTED_EDGE('',*,*,#8131,.F.);
#11566=ORIENTED_EDGE('',*,*,#8128,.F.);
#11567=ORIENTED_EDGE('',*,*,#8125,.F.);
#11568=ORIENTED_EDGE('',*,*,#8122,.F.);
#11569=ORIENTED_EDGE('',*,*,#8119,.F.);
#11570=ORIENTED_EDGE('',*,*,#8116,.F.);
#11571=ORIENTED_EDGE('',*,*,#8113,.F.);
#11572=ORIENTED_EDGE('',*,*,#8110,.F.);
#11573=ORIENTED_EDGE('',*,*,#8107,.F.);
#11574=ORIENTED_EDGE('',*,*,#8104,.F.);
#11575=ORIENTED_EDGE('',*,*,#8101,.F.);
#11576=ORIENTED_EDGE('',*,*,#8098,.F.);
#11577=ORIENTED_EDGE('',*,*,#8588,.F.);
#11578=ORIENTED_EDGE('',*,*,#8093,.F.);
#11579=ORIENTED_EDGE('',*,*,#8100,.F.);
#11580=ORIENTED_EDGE('',*,*,#8103,.F.);
#11581=ORIENTED_EDGE('',*,*,#8106,.F.);
#11582=ORIENTED_EDGE('',*,*,#8109,.F.);
#11583=ORIENTED_EDGE('',*,*,#8112,.F.);
#11584=ORIENTED_EDGE('',*,*,#8115,.F.);
#11585=ORIENTED_EDGE('',*,*,#8118,.F.);
#11586=ORIENTED_EDGE('',*,*,#8121,.F.);
#11587=ORIENTED_EDGE('',*,*,#8124,.F.);
#11588=ORIENTED_EDGE('',*,*,#8127,.F.);
#11589=ORIENTED_EDGE('',*,*,#8130,.F.);
#11590=ORIENTED_EDGE('',*,*,#8133,.F.);
#11591=ORIENTED_EDGE('',*,*,#8136,.F.);
#11592=ORIENTED_EDGE('',*,*,#8139,.F.);
#11593=ORIENTED_EDGE('',*,*,#8142,.F.);
#11594=ORIENTED_EDGE('',*,*,#8145,.F.);
#11595=ORIENTED_EDGE('',*,*,#8594,.F.);
#11596=ORIENTED_EDGE('',*,*,#8150,.F.);
#11597=ORIENTED_EDGE('',*,*,#8595,.F.);
#11598=ORIENTED_EDGE('',*,*,#8207,.T.);
#11599=ORIENTED_EDGE('',*,*,#8591,.T.);
#11600=ORIENTED_EDGE('',*,*,#8205,.T.);
#11601=ORIENTED_EDGE('',*,*,#8202,.T.);
#11602=ORIENTED_EDGE('',*,*,#8199,.T.);
#11603=ORIENTED_EDGE('',*,*,#8196,.T.);
#11604=ORIENTED_EDGE('',*,*,#8193,.T.);
#11605=ORIENTED_EDGE('',*,*,#8190,.T.);
#11606=ORIENTED_EDGE('',*,*,#8187,.T.);
#11607=ORIENTED_EDGE('',*,*,#8184,.T.);
#11608=ORIENTED_EDGE('',*,*,#8181,.T.);
#11609=ORIENTED_EDGE('',*,*,#8178,.T.);
#11610=ORIENTED_EDGE('',*,*,#8175,.T.);
#11611=ORIENTED_EDGE('',*,*,#8172,.T.);
#11612=ORIENTED_EDGE('',*,*,#8169,.T.);
#11613=ORIENTED_EDGE('',*,*,#8166,.T.);
#11614=ORIENTED_EDGE('',*,*,#8163,.T.);
#11615=ORIENTED_EDGE('',*,*,#8160,.T.);
#11616=ORIENTED_EDGE('',*,*,#8157,.T.);
#11617=ORIENTED_EDGE('',*,*,#8154,.T.);
#11618=ORIENTED_EDGE('',*,*,#8147,.T.);
#11619=ORIENTED_EDGE('',*,*,#8594,.T.);
#11620=ORIENTED_EDGE('',*,*,#8144,.F.);
#11621=ORIENTED_EDGE('',*,*,#8593,.T.);
#11622=ORIENTED_EDGE('',*,*,#8096,.F.);
#11623=ORIENTED_EDGE('',*,*,#8332,.F.);
#11624=ORIENTED_EDGE('',*,*,#8214,.F.);
#11625=ORIENTED_EDGE('',*,*,#8450,.F.);
#11626=ORIENTED_EDGE('',*,*,#7976,.F.);
#11627=ORIENTED_EDGE('',*,*,#8596,.T.);
#11628=ORIENTED_EDGE('',*,*,#8035,.T.);
#11629=ORIENTED_EDGE('',*,*,#8597,.T.);
#11630=ORIENTED_EDGE('',*,*,#7979,.F.);
#11631=ORIENTED_EDGE('',*,*,#8088,.T.);
#11632=ORIENTED_EDGE('',*,*,#8598,.T.);
#11633=ORIENTED_EDGE('',*,*,#8085,.F.);
#11634=ORIENTED_EDGE('',*,*,#8599,.F.);
#11635=ORIENTED_EDGE('',*,*,#8597,.F.);
#11636=ORIENTED_EDGE('',*,*,#8034,.F.);
#11637=ORIENTED_EDGE('',*,*,#8038,.F.);
#11638=ORIENTED_EDGE('',*,*,#8041,.F.);
#11639=ORIENTED_EDGE('',*,*,#8044,.F.);
#11640=ORIENTED_EDGE('',*,*,#8047,.F.);
#11641=ORIENTED_EDGE('',*,*,#8050,.F.);
#11642=ORIENTED_EDGE('',*,*,#8053,.F.);
#11643=ORIENTED_EDGE('',*,*,#8056,.F.);
#11644=ORIENTED_EDGE('',*,*,#8059,.F.);
#11645=ORIENTED_EDGE('',*,*,#8062,.F.);
#11646=ORIENTED_EDGE('',*,*,#8065,.F.);
#11647=ORIENTED_EDGE('',*,*,#8068,.F.);
#11648=ORIENTED_EDGE('',*,*,#8071,.F.);
#11649=ORIENTED_EDGE('',*,*,#8074,.F.);
#11650=ORIENTED_EDGE('',*,*,#8077,.F.);
#11651=ORIENTED_EDGE('',*,*,#8080,.F.);
#11652=ORIENTED_EDGE('',*,*,#8083,.F.);
#11653=ORIENTED_EDGE('',*,*,#8086,.F.);
#11654=ORIENTED_EDGE('',*,*,#8598,.F.);
#11655=ORIENTED_EDGE('',*,*,#8091,.F.);
#11656=ORIENTED_EDGE('',*,*,#8600,.F.);
#11657=ORIENTED_EDGE('',*,*,#8030,.F.);
#11658=ORIENTED_EDGE('',*,*,#8601,.F.);
#11659=ORIENTED_EDGE('',*,*,#8028,.F.);
#11660=ORIENTED_EDGE('',*,*,#8025,.F.);
#11661=ORIENTED_EDGE('',*,*,#8022,.F.);
#11662=ORIENTED_EDGE('',*,*,#8019,.F.);
#11663=ORIENTED_EDGE('',*,*,#8016,.F.);
#11664=ORIENTED_EDGE('',*,*,#8013,.F.);
#11665=ORIENTED_EDGE('',*,*,#8010,.F.);
#11666=ORIENTED_EDGE('',*,*,#8007,.F.);
#11667=ORIENTED_EDGE('',*,*,#8004,.F.);
#11668=ORIENTED_EDGE('',*,*,#8001,.F.);
#11669=ORIENTED_EDGE('',*,*,#7998,.F.);
#11670=ORIENTED_EDGE('',*,*,#7995,.F.);
#11671=ORIENTED_EDGE('',*,*,#7992,.F.);
#11672=ORIENTED_EDGE('',*,*,#7989,.F.);
#11673=ORIENTED_EDGE('',*,*,#7986,.F.);
#11674=ORIENTED_EDGE('',*,*,#7983,.F.);
#11675=ORIENTED_EDGE('',*,*,#7980,.F.);
#11676=ORIENTED_EDGE('',*,*,#8596,.F.);
#11677=ORIENTED_EDGE('',*,*,#7975,.F.);
#11678=ORIENTED_EDGE('',*,*,#7982,.F.);
#11679=ORIENTED_EDGE('',*,*,#7985,.F.);
#11680=ORIENTED_EDGE('',*,*,#7988,.F.);
#11681=ORIENTED_EDGE('',*,*,#7991,.F.);
#11682=ORIENTED_EDGE('',*,*,#7994,.F.);
#11683=ORIENTED_EDGE('',*,*,#7997,.F.);
#11684=ORIENTED_EDGE('',*,*,#8000,.F.);
#11685=ORIENTED_EDGE('',*,*,#8003,.F.);
#11686=ORIENTED_EDGE('',*,*,#8006,.F.);
#11687=ORIENTED_EDGE('',*,*,#8009,.F.);
#11688=ORIENTED_EDGE('',*,*,#8012,.F.);
#11689=ORIENTED_EDGE('',*,*,#8015,.F.);
#11690=ORIENTED_EDGE('',*,*,#8018,.F.);
#11691=ORIENTED_EDGE('',*,*,#8021,.F.);
#11692=ORIENTED_EDGE('',*,*,#8024,.F.);
#11693=ORIENTED_EDGE('',*,*,#8027,.F.);
#11694=ORIENTED_EDGE('',*,*,#8602,.F.);
#11695=ORIENTED_EDGE('',*,*,#8032,.F.);
#11696=ORIENTED_EDGE('',*,*,#8603,.F.);
#11697=ORIENTED_EDGE('',*,*,#8089,.T.);
#11698=ORIENTED_EDGE('',*,*,#8599,.T.);
#11699=ORIENTED_EDGE('',*,*,#8087,.T.);
#11700=ORIENTED_EDGE('',*,*,#8084,.T.);
#11701=ORIENTED_EDGE('',*,*,#8081,.T.);
#11702=ORIENTED_EDGE('',*,*,#8078,.T.);
#11703=ORIENTED_EDGE('',*,*,#8075,.T.);
#11704=ORIENTED_EDGE('',*,*,#8072,.T.);
#11705=ORIENTED_EDGE('',*,*,#8069,.T.);
#11706=ORIENTED_EDGE('',*,*,#8066,.T.);
#11707=ORIENTED_EDGE('',*,*,#8063,.T.);
#11708=ORIENTED_EDGE('',*,*,#8060,.T.);
#11709=ORIENTED_EDGE('',*,*,#8057,.T.);
#11710=ORIENTED_EDGE('',*,*,#8054,.T.);
#11711=ORIENTED_EDGE('',*,*,#8051,.T.);
#11712=ORIENTED_EDGE('',*,*,#8048,.T.);
#11713=ORIENTED_EDGE('',*,*,#8045,.T.);
#11714=ORIENTED_EDGE('',*,*,#8042,.T.);
#11715=ORIENTED_EDGE('',*,*,#8039,.T.);
#11716=ORIENTED_EDGE('',*,*,#8036,.T.);
#11717=ORIENTED_EDGE('',*,*,#8029,.T.);
#11718=ORIENTED_EDGE('',*,*,#8602,.T.);
#11719=ORIENTED_EDGE('',*,*,#8026,.F.);
#11720=ORIENTED_EDGE('',*,*,#8601,.T.);
#11721=ORIENTED_EDGE('',*,*,#7858,.F.);
#11722=ORIENTED_EDGE('',*,*,#8604,.T.);
#11723=ORIENTED_EDGE('',*,*,#7917,.T.);
#11724=ORIENTED_EDGE('',*,*,#8605,.T.);
#11725=ORIENTED_EDGE('',*,*,#7861,.F.);
#11726=ORIENTED_EDGE('',*,*,#7970,.T.);
#11727=ORIENTED_EDGE('',*,*,#8606,.T.);
#11728=ORIENTED_EDGE('',*,*,#7967,.F.);
#11729=ORIENTED_EDGE('',*,*,#8607,.F.);
#11730=ORIENTED_EDGE('',*,*,#8605,.F.);
#11731=ORIENTED_EDGE('',*,*,#7916,.F.);
#11732=ORIENTED_EDGE('',*,*,#7920,.F.);
#11733=ORIENTED_EDGE('',*,*,#7923,.F.);
#11734=ORIENTED_EDGE('',*,*,#7926,.F.);
#11735=ORIENTED_EDGE('',*,*,#7929,.F.);
#11736=ORIENTED_EDGE('',*,*,#7932,.F.);
#11737=ORIENTED_EDGE('',*,*,#7935,.F.);
#11738=ORIENTED_EDGE('',*,*,#7938,.F.);
#11739=ORIENTED_EDGE('',*,*,#7941,.F.);
#11740=ORIENTED_EDGE('',*,*,#7944,.F.);
#11741=ORIENTED_EDGE('',*,*,#7947,.F.);
#11742=ORIENTED_EDGE('',*,*,#7950,.F.);
#11743=ORIENTED_EDGE('',*,*,#7953,.F.);
#11744=ORIENTED_EDGE('',*,*,#7956,.F.);
#11745=ORIENTED_EDGE('',*,*,#7959,.F.);
#11746=ORIENTED_EDGE('',*,*,#7962,.F.);
#11747=ORIENTED_EDGE('',*,*,#7965,.F.);
#11748=ORIENTED_EDGE('',*,*,#7968,.F.);
#11749=ORIENTED_EDGE('',*,*,#8606,.F.);
#11750=ORIENTED_EDGE('',*,*,#7973,.F.);
#11751=ORIENTED_EDGE('',*,*,#8608,.F.);
#11752=ORIENTED_EDGE('',*,*,#7912,.F.);
#11753=ORIENTED_EDGE('',*,*,#8609,.F.);
#11754=ORIENTED_EDGE('',*,*,#7910,.F.);
#11755=ORIENTED_EDGE('',*,*,#7907,.F.);
#11756=ORIENTED_EDGE('',*,*,#7904,.F.);
#11757=ORIENTED_EDGE('',*,*,#7901,.F.);
#11758=ORIENTED_EDGE('',*,*,#7898,.F.);
#11759=ORIENTED_EDGE('',*,*,#7895,.F.);
#11760=ORIENTED_EDGE('',*,*,#7892,.F.);
#11761=ORIENTED_EDGE('',*,*,#7889,.F.);
#11762=ORIENTED_EDGE('',*,*,#7886,.F.);
#11763=ORIENTED_EDGE('',*,*,#7883,.F.);
#11764=ORIENTED_EDGE('',*,*,#7880,.F.);
#11765=ORIENTED_EDGE('',*,*,#7877,.F.);
#11766=ORIENTED_EDGE('',*,*,#7874,.F.);
#11767=ORIENTED_EDGE('',*,*,#7871,.F.);
#11768=ORIENTED_EDGE('',*,*,#7868,.F.);
#11769=ORIENTED_EDGE('',*,*,#7865,.F.);
#11770=ORIENTED_EDGE('',*,*,#7862,.F.);
#11771=ORIENTED_EDGE('',*,*,#8604,.F.);
#11772=ORIENTED_EDGE('',*,*,#7857,.F.);
#11773=ORIENTED_EDGE('',*,*,#7864,.F.);
#11774=ORIENTED_EDGE('',*,*,#7867,.F.);
#11775=ORIENTED_EDGE('',*,*,#7870,.F.);
#11776=ORIENTED_EDGE('',*,*,#7873,.F.);
#11777=ORIENTED_EDGE('',*,*,#7876,.F.);
#11778=ORIENTED_EDGE('',*,*,#7879,.F.);
#11779=ORIENTED_EDGE('',*,*,#7882,.F.);
#11780=ORIENTED_EDGE('',*,*,#7885,.F.);
#11781=ORIENTED_EDGE('',*,*,#7888,.F.);
#11782=ORIENTED_EDGE('',*,*,#7891,.F.);
#11783=ORIENTED_EDGE('',*,*,#7894,.F.);
#11784=ORIENTED_EDGE('',*,*,#7897,.F.);
#11785=ORIENTED_EDGE('',*,*,#7900,.F.);
#11786=ORIENTED_EDGE('',*,*,#7903,.F.);
#11787=ORIENTED_EDGE('',*,*,#7906,.F.);
#11788=ORIENTED_EDGE('',*,*,#7909,.F.);
#11789=ORIENTED_EDGE('',*,*,#8610,.F.);
#11790=ORIENTED_EDGE('',*,*,#7914,.F.);
#11791=ORIENTED_EDGE('',*,*,#8611,.F.);
#11792=ORIENTED_EDGE('',*,*,#7971,.T.);
#11793=ORIENTED_EDGE('',*,*,#8607,.T.);
#11794=ORIENTED_EDGE('',*,*,#7969,.T.);
#11795=ORIENTED_EDGE('',*,*,#7966,.T.);
#11796=ORIENTED_EDGE('',*,*,#7963,.T.);
#11797=ORIENTED_EDGE('',*,*,#7960,.T.);
#11798=ORIENTED_EDGE('',*,*,#7957,.T.);
#11799=ORIENTED_EDGE('',*,*,#7954,.T.);
#11800=ORIENTED_EDGE('',*,*,#7951,.T.);
#11801=ORIENTED_EDGE('',*,*,#7948,.T.);
#11802=ORIENTED_EDGE('',*,*,#7945,.T.);
#11803=ORIENTED_EDGE('',*,*,#7942,.T.);
#11804=ORIENTED_EDGE('',*,*,#7939,.T.);
#11805=ORIENTED_EDGE('',*,*,#7936,.T.);
#11806=ORIENTED_EDGE('',*,*,#7933,.T.);
#11807=ORIENTED_EDGE('',*,*,#7930,.T.);
#11808=ORIENTED_EDGE('',*,*,#7927,.T.);
#11809=ORIENTED_EDGE('',*,*,#7924,.T.);
#11810=ORIENTED_EDGE('',*,*,#7921,.T.);
#11811=ORIENTED_EDGE('',*,*,#7918,.T.);
#11812=ORIENTED_EDGE('',*,*,#7911,.T.);
#11813=ORIENTED_EDGE('',*,*,#8610,.T.);
#11814=ORIENTED_EDGE('',*,*,#7908,.F.);
#11815=ORIENTED_EDGE('',*,*,#8609,.T.);
#11816=ORIENTED_EDGE('',*,*,#7740,.F.);
#11817=ORIENTED_EDGE('',*,*,#8612,.T.);
#11818=ORIENTED_EDGE('',*,*,#7799,.T.);
#11819=ORIENTED_EDGE('',*,*,#8613,.T.);
#11820=ORIENTED_EDGE('',*,*,#7743,.F.);
#11821=ORIENTED_EDGE('',*,*,#7852,.T.);
#11822=ORIENTED_EDGE('',*,*,#8614,.T.);
#11823=ORIENTED_EDGE('',*,*,#7849,.F.);
#11824=ORIENTED_EDGE('',*,*,#8615,.F.);
#11825=ORIENTED_EDGE('',*,*,#8613,.F.);
#11826=ORIENTED_EDGE('',*,*,#7798,.F.);
#11827=ORIENTED_EDGE('',*,*,#7802,.F.);
#11828=ORIENTED_EDGE('',*,*,#7805,.F.);
#11829=ORIENTED_EDGE('',*,*,#7808,.F.);
#11830=ORIENTED_EDGE('',*,*,#7811,.F.);
#11831=ORIENTED_EDGE('',*,*,#7814,.F.);
#11832=ORIENTED_EDGE('',*,*,#7817,.F.);
#11833=ORIENTED_EDGE('',*,*,#7820,.F.);
#11834=ORIENTED_EDGE('',*,*,#7823,.F.);
#11835=ORIENTED_EDGE('',*,*,#7826,.F.);
#11836=ORIENTED_EDGE('',*,*,#7829,.F.);
#11837=ORIENTED_EDGE('',*,*,#7832,.F.);
#11838=ORIENTED_EDGE('',*,*,#7835,.F.);
#11839=ORIENTED_EDGE('',*,*,#7838,.F.);
#11840=ORIENTED_EDGE('',*,*,#7841,.F.);
#11841=ORIENTED_EDGE('',*,*,#7844,.F.);
#11842=ORIENTED_EDGE('',*,*,#7847,.F.);
#11843=ORIENTED_EDGE('',*,*,#7850,.F.);
#11844=ORIENTED_EDGE('',*,*,#8614,.F.);
#11845=ORIENTED_EDGE('',*,*,#7855,.F.);
#11846=ORIENTED_EDGE('',*,*,#8616,.F.);
#11847=ORIENTED_EDGE('',*,*,#7794,.F.);
#11848=ORIENTED_EDGE('',*,*,#8617,.F.);
#11849=ORIENTED_EDGE('',*,*,#7792,.F.);
#11850=ORIENTED_EDGE('',*,*,#7789,.F.);
#11851=ORIENTED_EDGE('',*,*,#7786,.F.);
#11852=ORIENTED_EDGE('',*,*,#7783,.F.);
#11853=ORIENTED_EDGE('',*,*,#7780,.F.);
#11854=ORIENTED_EDGE('',*,*,#7777,.F.);
#11855=ORIENTED_EDGE('',*,*,#7774,.F.);
#11856=ORIENTED_EDGE('',*,*,#7771,.F.);
#11857=ORIENTED_EDGE('',*,*,#7768,.F.);
#11858=ORIENTED_EDGE('',*,*,#7765,.F.);
#11859=ORIENTED_EDGE('',*,*,#7762,.F.);
#11860=ORIENTED_EDGE('',*,*,#7759,.F.);
#11861=ORIENTED_EDGE('',*,*,#7756,.F.);
#11862=ORIENTED_EDGE('',*,*,#7753,.F.);
#11863=ORIENTED_EDGE('',*,*,#7750,.F.);
#11864=ORIENTED_EDGE('',*,*,#7747,.F.);
#11865=ORIENTED_EDGE('',*,*,#7744,.F.);
#11866=ORIENTED_EDGE('',*,*,#8612,.F.);
#11867=ORIENTED_EDGE('',*,*,#7739,.F.);
#11868=ORIENTED_EDGE('',*,*,#7746,.F.);
#11869=ORIENTED_EDGE('',*,*,#7749,.F.);
#11870=ORIENTED_EDGE('',*,*,#7752,.F.);
#11871=ORIENTED_EDGE('',*,*,#7755,.F.);
#11872=ORIENTED_EDGE('',*,*,#7758,.F.);
#11873=ORIENTED_EDGE('',*,*,#7761,.F.);
#11874=ORIENTED_EDGE('',*,*,#7764,.F.);
#11875=ORIENTED_EDGE('',*,*,#7767,.F.);
#11876=ORIENTED_EDGE('',*,*,#7770,.F.);
#11877=ORIENTED_EDGE('',*,*,#7773,.F.);
#11878=ORIENTED_EDGE('',*,*,#7776,.F.);
#11879=ORIENTED_EDGE('',*,*,#7779,.F.);
#11880=ORIENTED_EDGE('',*,*,#7782,.F.);
#11881=ORIENTED_EDGE('',*,*,#7785,.F.);
#11882=ORIENTED_EDGE('',*,*,#7788,.F.);
#11883=ORIENTED_EDGE('',*,*,#7791,.F.);
#11884=ORIENTED_EDGE('',*,*,#8618,.F.);
#11885=ORIENTED_EDGE('',*,*,#7796,.F.);
#11886=ORIENTED_EDGE('',*,*,#8619,.F.);
#11887=ORIENTED_EDGE('',*,*,#7853,.T.);
#11888=ORIENTED_EDGE('',*,*,#8615,.T.);
#11889=ORIENTED_EDGE('',*,*,#7851,.T.);
#11890=ORIENTED_EDGE('',*,*,#7848,.T.);
#11891=ORIENTED_EDGE('',*,*,#7845,.T.);
#11892=ORIENTED_EDGE('',*,*,#7842,.T.);
#11893=ORIENTED_EDGE('',*,*,#7839,.T.);
#11894=ORIENTED_EDGE('',*,*,#7836,.T.);
#11895=ORIENTED_EDGE('',*,*,#7833,.T.);
#11896=ORIENTED_EDGE('',*,*,#7830,.T.);
#11897=ORIENTED_EDGE('',*,*,#7827,.T.);
#11898=ORIENTED_EDGE('',*,*,#7824,.T.);
#11899=ORIENTED_EDGE('',*,*,#7821,.T.);
#11900=ORIENTED_EDGE('',*,*,#7818,.T.);
#11901=ORIENTED_EDGE('',*,*,#7815,.T.);
#11902=ORIENTED_EDGE('',*,*,#7812,.T.);
#11903=ORIENTED_EDGE('',*,*,#7809,.T.);
#11904=ORIENTED_EDGE('',*,*,#7806,.T.);
#11905=ORIENTED_EDGE('',*,*,#7803,.T.);
#11906=ORIENTED_EDGE('',*,*,#7800,.T.);
#11907=ORIENTED_EDGE('',*,*,#7793,.T.);
#11908=ORIENTED_EDGE('',*,*,#8618,.T.);
#11909=ORIENTED_EDGE('',*,*,#7790,.F.);
#11910=ORIENTED_EDGE('',*,*,#8617,.T.);
#11911=ORIENTED_EDGE('',*,*,#7622,.F.);
#11912=ORIENTED_EDGE('',*,*,#8620,.T.);
#11913=ORIENTED_EDGE('',*,*,#7681,.T.);
#11914=ORIENTED_EDGE('',*,*,#8621,.T.);
#11915=ORIENTED_EDGE('',*,*,#7625,.F.);
#11916=ORIENTED_EDGE('',*,*,#7734,.T.);
#11917=ORIENTED_EDGE('',*,*,#8622,.T.);
#11918=ORIENTED_EDGE('',*,*,#7731,.F.);
#11919=ORIENTED_EDGE('',*,*,#8623,.F.);
#11920=ORIENTED_EDGE('',*,*,#8621,.F.);
#11921=ORIENTED_EDGE('',*,*,#7680,.F.);
#11922=ORIENTED_EDGE('',*,*,#7684,.F.);
#11923=ORIENTED_EDGE('',*,*,#7687,.F.);
#11924=ORIENTED_EDGE('',*,*,#7690,.F.);
#11925=ORIENTED_EDGE('',*,*,#7693,.F.);
#11926=ORIENTED_EDGE('',*,*,#7696,.F.);
#11927=ORIENTED_EDGE('',*,*,#7699,.F.);
#11928=ORIENTED_EDGE('',*,*,#7702,.F.);
#11929=ORIENTED_EDGE('',*,*,#7705,.F.);
#11930=ORIENTED_EDGE('',*,*,#7708,.F.);
#11931=ORIENTED_EDGE('',*,*,#7711,.F.);
#11932=ORIENTED_EDGE('',*,*,#7714,.F.);
#11933=ORIENTED_EDGE('',*,*,#7717,.F.);
#11934=ORIENTED_EDGE('',*,*,#7720,.F.);
#11935=ORIENTED_EDGE('',*,*,#7723,.F.);
#11936=ORIENTED_EDGE('',*,*,#7726,.F.);
#11937=ORIENTED_EDGE('',*,*,#7729,.F.);
#11938=ORIENTED_EDGE('',*,*,#7732,.F.);
#11939=ORIENTED_EDGE('',*,*,#8622,.F.);
#11940=ORIENTED_EDGE('',*,*,#7737,.F.);
#11941=ORIENTED_EDGE('',*,*,#8624,.F.);
#11942=ORIENTED_EDGE('',*,*,#7676,.F.);
#11943=ORIENTED_EDGE('',*,*,#8625,.F.);
#11944=ORIENTED_EDGE('',*,*,#7674,.F.);
#11945=ORIENTED_EDGE('',*,*,#7671,.F.);
#11946=ORIENTED_EDGE('',*,*,#7668,.F.);
#11947=ORIENTED_EDGE('',*,*,#7665,.F.);
#11948=ORIENTED_EDGE('',*,*,#7662,.F.);
#11949=ORIENTED_EDGE('',*,*,#7659,.F.);
#11950=ORIENTED_EDGE('',*,*,#7656,.F.);
#11951=ORIENTED_EDGE('',*,*,#7653,.F.);
#11952=ORIENTED_EDGE('',*,*,#7650,.F.);
#11953=ORIENTED_EDGE('',*,*,#7647,.F.);
#11954=ORIENTED_EDGE('',*,*,#7644,.F.);
#11955=ORIENTED_EDGE('',*,*,#7641,.F.);
#11956=ORIENTED_EDGE('',*,*,#7638,.F.);
#11957=ORIENTED_EDGE('',*,*,#7635,.F.);
#11958=ORIENTED_EDGE('',*,*,#7632,.F.);
#11959=ORIENTED_EDGE('',*,*,#7629,.F.);
#11960=ORIENTED_EDGE('',*,*,#7626,.F.);
#11961=ORIENTED_EDGE('',*,*,#8620,.F.);
#11962=ORIENTED_EDGE('',*,*,#7621,.F.);
#11963=ORIENTED_EDGE('',*,*,#7628,.F.);
#11964=ORIENTED_EDGE('',*,*,#7631,.F.);
#11965=ORIENTED_EDGE('',*,*,#7634,.F.);
#11966=ORIENTED_EDGE('',*,*,#7637,.F.);
#11967=ORIENTED_EDGE('',*,*,#7640,.F.);
#11968=ORIENTED_EDGE('',*,*,#7643,.F.);
#11969=ORIENTED_EDGE('',*,*,#7646,.F.);
#11970=ORIENTED_EDGE('',*,*,#7649,.F.);
#11971=ORIENTED_EDGE('',*,*,#7652,.F.);
#11972=ORIENTED_EDGE('',*,*,#7655,.F.);
#11973=ORIENTED_EDGE('',*,*,#7658,.F.);
#11974=ORIENTED_EDGE('',*,*,#7661,.F.);
#11975=ORIENTED_EDGE('',*,*,#7664,.F.);
#11976=ORIENTED_EDGE('',*,*,#7667,.F.);
#11977=ORIENTED_EDGE('',*,*,#7670,.F.);
#11978=ORIENTED_EDGE('',*,*,#7673,.F.);
#11979=ORIENTED_EDGE('',*,*,#8626,.F.);
#11980=ORIENTED_EDGE('',*,*,#7678,.F.);
#11981=ORIENTED_EDGE('',*,*,#8627,.F.);
#11982=ORIENTED_EDGE('',*,*,#7735,.T.);
#11983=ORIENTED_EDGE('',*,*,#8623,.T.);
#11984=ORIENTED_EDGE('',*,*,#7733,.T.);
#11985=ORIENTED_EDGE('',*,*,#7730,.T.);
#11986=ORIENTED_EDGE('',*,*,#7727,.T.);
#11987=ORIENTED_EDGE('',*,*,#7724,.T.);
#11988=ORIENTED_EDGE('',*,*,#7721,.T.);
#11989=ORIENTED_EDGE('',*,*,#7718,.T.);
#11990=ORIENTED_EDGE('',*,*,#7715,.T.);
#11991=ORIENTED_EDGE('',*,*,#7712,.T.);
#11992=ORIENTED_EDGE('',*,*,#7709,.T.);
#11993=ORIENTED_EDGE('',*,*,#7706,.T.);
#11994=ORIENTED_EDGE('',*,*,#7703,.T.);
#11995=ORIENTED_EDGE('',*,*,#7700,.T.);
#11996=ORIENTED_EDGE('',*,*,#7697,.T.);
#11997=ORIENTED_EDGE('',*,*,#7694,.T.);
#11998=ORIENTED_EDGE('',*,*,#7691,.T.);
#11999=ORIENTED_EDGE('',*,*,#7688,.T.);
#12000=ORIENTED_EDGE('',*,*,#7685,.T.);
#12001=ORIENTED_EDGE('',*,*,#7682,.T.);
#12002=ORIENTED_EDGE('',*,*,#7675,.T.);
#12003=ORIENTED_EDGE('',*,*,#8626,.T.);
#12004=ORIENTED_EDGE('',*,*,#7672,.F.);
#12005=ORIENTED_EDGE('',*,*,#8625,.T.);
#12006=ORIENTED_EDGE('',*,*,#7624,.F.);
#12007=ORIENTED_EDGE('',*,*,#7978,.F.);
#12008=ORIENTED_EDGE('',*,*,#7860,.F.);
#12009=ORIENTED_EDGE('',*,*,#7742,.F.);
#12010=ORIENTED_EDGE('',*,*,#8628,.F.);
#12011=ORIENTED_EDGE('',*,*,#8629,.F.);
#12012=ORIENTED_EDGE('',*,*,#8630,.T.);
#12013=ORIENTED_EDGE('',*,*,#8631,.F.);
#12014=ORIENTED_EDGE('',*,*,#8632,.F.);
#12015=ORIENTED_EDGE('',*,*,#8633,.T.);
#12016=ORIENTED_EDGE('',*,*,#8634,.F.);
#12017=ORIENTED_EDGE('',*,*,#8630,.F.);
#12018=ORIENTED_EDGE('',*,*,#8635,.F.);
#12019=ORIENTED_EDGE('',*,*,#8636,.F.);
#12020=ORIENTED_EDGE('',*,*,#8633,.F.);
#12021=ORIENTED_EDGE('',*,*,#8637,.F.);
#12022=ORIENTED_EDGE('',*,*,#8631,.T.);
#12023=ORIENTED_EDGE('',*,*,#8634,.T.);
#12024=ORIENTED_EDGE('',*,*,#8636,.T.);
#12025=ORIENTED_EDGE('',*,*,#8638,.F.);
#12026=ORIENTED_EDGE('',*,*,#8603,.T.);
#12027=ORIENTED_EDGE('',*,*,#8031,.T.);
#12028=ORIENTED_EDGE('',*,*,#8600,.T.);
#12029=ORIENTED_EDGE('',*,*,#8090,.T.);
#12030=ORIENTED_EDGE('',*,*,#8611,.T.);
#12031=ORIENTED_EDGE('',*,*,#7913,.T.);
#12032=ORIENTED_EDGE('',*,*,#8608,.T.);
#12033=ORIENTED_EDGE('',*,*,#7972,.T.);
#12034=ORIENTED_EDGE('',*,*,#8619,.T.);
#12035=ORIENTED_EDGE('',*,*,#7795,.T.);
#12036=ORIENTED_EDGE('',*,*,#8616,.T.);
#12037=ORIENTED_EDGE('',*,*,#7854,.T.);
#12038=ORIENTED_EDGE('',*,*,#8627,.T.);
#12039=ORIENTED_EDGE('',*,*,#7677,.T.);
#12040=ORIENTED_EDGE('',*,*,#8624,.T.);
#12041=ORIENTED_EDGE('',*,*,#7736,.T.);
#12042=ORIENTED_EDGE('',*,*,#8639,.F.);
#12043=ORIENTED_EDGE('',*,*,#7616,.T.);
#12044=ORIENTED_EDGE('',*,*,#8640,.T.);
#12045=ORIENTED_EDGE('',*,*,#7613,.F.);
#12046=ORIENTED_EDGE('',*,*,#8641,.F.);
#12047=ORIENTED_EDGE('',*,*,#8642,.F.);
#12048=ORIENTED_EDGE('',*,*,#7598,.F.);
#12049=ORIENTED_EDGE('',*,*,#7602,.F.);
#12050=ORIENTED_EDGE('',*,*,#7605,.F.);
#12051=ORIENTED_EDGE('',*,*,#7608,.F.);
#12052=ORIENTED_EDGE('',*,*,#7611,.F.);
#12053=ORIENTED_EDGE('',*,*,#7614,.F.);
#12054=ORIENTED_EDGE('',*,*,#8640,.F.);
#12055=ORIENTED_EDGE('',*,*,#7619,.F.);
#12056=ORIENTED_EDGE('',*,*,#8643,.F.);
#12057=ORIENTED_EDGE('',*,*,#7594,.F.);
#12058=ORIENTED_EDGE('',*,*,#8644,.F.);
#12059=ORIENTED_EDGE('',*,*,#7592,.F.);
#12060=ORIENTED_EDGE('',*,*,#7589,.F.);
#12061=ORIENTED_EDGE('',*,*,#7586,.F.);
#12062=ORIENTED_EDGE('',*,*,#7583,.F.);
#12063=ORIENTED_EDGE('',*,*,#7580,.F.);
#12064=ORIENTED_EDGE('',*,*,#7576,.F.);
#12065=ORIENTED_EDGE('',*,*,#8645,.F.);
#12066=ORIENTED_EDGE('',*,*,#7578,.F.);
#12067=ORIENTED_EDGE('',*,*,#7582,.F.);
#12068=ORIENTED_EDGE('',*,*,#7585,.F.);
#12069=ORIENTED_EDGE('',*,*,#7588,.F.);
#12070=ORIENTED_EDGE('',*,*,#7591,.F.);
#12071=ORIENTED_EDGE('',*,*,#8646,.F.);
#12072=ORIENTED_EDGE('',*,*,#7596,.F.);
#12073=ORIENTED_EDGE('',*,*,#8647,.F.);
#12074=ORIENTED_EDGE('',*,*,#7617,.T.);
#12075=ORIENTED_EDGE('',*,*,#8641,.T.);
#12076=ORIENTED_EDGE('',*,*,#7615,.T.);
#12077=ORIENTED_EDGE('',*,*,#7612,.T.);
#12078=ORIENTED_EDGE('',*,*,#7609,.T.);
#12079=ORIENTED_EDGE('',*,*,#7606,.T.);
#12080=ORIENTED_EDGE('',*,*,#7603,.T.);
#12081=ORIENTED_EDGE('',*,*,#7600,.T.);
#12082=ORIENTED_EDGE('',*,*,#8648,.F.);
#12083=ORIENTED_EDGE('',*,*,#8649,.T.);
#12084=ORIENTED_EDGE('',*,*,#8650,.T.);
#12085=ORIENTED_EDGE('',*,*,#8651,.T.);
#12086=ORIENTED_EDGE('',*,*,#8643,.T.);
#12087=ORIENTED_EDGE('',*,*,#7618,.T.);
#12088=ORIENTED_EDGE('',*,*,#8647,.T.);
#12089=ORIENTED_EDGE('',*,*,#7595,.T.);
#12090=ORIENTED_EDGE('',*,*,#7593,.T.);
#12091=ORIENTED_EDGE('',*,*,#8646,.T.);
#12092=ORIENTED_EDGE('',*,*,#7590,.F.);
#12093=ORIENTED_EDGE('',*,*,#8644,.T.);
#12094=ORIENTED_EDGE('',*,*,#8652,.F.);
#12095=ORIENTED_EDGE('',*,*,#8653,.T.);
#12096=ORIENTED_EDGE('',*,*,#8654,.T.);
#12097=ORIENTED_EDGE('',*,*,#8649,.F.);
#12098=ORIENTED_EDGE('',*,*,#8655,.F.);
#12099=ORIENTED_EDGE('',*,*,#8651,.F.);
#12100=ORIENTED_EDGE('',*,*,#8656,.F.);
#12101=ORIENTED_EDGE('',*,*,#8657,.T.);
#12102=ORIENTED_EDGE('',*,*,#8658,.T.);
#12103=ORIENTED_EDGE('',*,*,#8656,.T.);
#12104=ORIENTED_EDGE('',*,*,#8650,.F.);
#12105=ORIENTED_EDGE('',*,*,#8654,.F.);
#12106=ORIENTED_EDGE('',*,*,#8659,.F.);
#12107=ORIENTED_EDGE('',*,*,#8657,.F.);
#12108=ORIENTED_EDGE('',*,*,#8658,.F.);
#12109=ORIENTED_EDGE('',*,*,#8653,.F.);
#12110=ORIENTED_EDGE('',*,*,#8642,.T.);
#12111=ORIENTED_EDGE('',*,*,#7575,.T.);
#12112=ORIENTED_EDGE('',*,*,#7579,.T.);
#12113=ORIENTED_EDGE('',*,*,#8645,.T.);
#12114=ORIENTED_EDGE('',*,*,#7599,.T.);
#12115=ORIENTED_EDGE('',*,*,#8660,.F.);
#12116=ORIENTED_EDGE('',*,*,#8661,.T.);
#12117=ORIENTED_EDGE('',*,*,#8662,.F.);
#12118=ORIENTED_EDGE('',*,*,#8663,.F.);
#12119=ORIENTED_EDGE('',*,*,#8661,.F.);
#12120=ORIENTED_EDGE('',*,*,#8664,.T.);
#12121=ORIENTED_EDGE('',*,*,#8663,.T.);
#12122=ORIENTED_EDGE('',*,*,#8664,.F.);
#12123=ORIENTED_EDGE('',*,*,#8662,.T.);
#12124=ORIENTED_EDGE('',*,*,#8665,.T.);
#12125=ORIENTED_EDGE('',*,*,#8666,.T.);
#12126=ORIENTED_EDGE('',*,*,#8665,.F.);
#12127=ORIENTED_EDGE('',*,*,#8666,.F.);
#12128=ORIENTED_EDGE('',*,*,#8667,.T.);
#12129=ORIENTED_EDGE('',*,*,#8668,.F.);
#12130=ORIENTED_EDGE('',*,*,#8669,.F.);
#12131=ORIENTED_EDGE('',*,*,#8667,.F.);
#12132=ORIENTED_EDGE('',*,*,#8670,.T.);
#12133=ORIENTED_EDGE('',*,*,#8669,.T.);
#12134=ORIENTED_EDGE('',*,*,#8670,.F.);
#12135=ORIENTED_EDGE('',*,*,#8668,.T.);
#12136=ORIENTED_EDGE('',*,*,#8671,.T.);
#12137=ORIENTED_EDGE('',*,*,#8639,.T.);
#12138=ORIENTED_EDGE('',*,*,#8671,.F.);
#12139=ORIENTED_EDGE('',*,*,#8672,.F.);
#12140=ORIENTED_EDGE('',*,*,#8673,.T.);
#12141=ORIENTED_EDGE('',*,*,#8660,.T.);
#12142=ORIENTED_EDGE('',*,*,#8673,.F.);
#12143=ORIENTED_EDGE('',*,*,#8628,.T.);
#12144=ORIENTED_EDGE('',*,*,#8638,.T.);
#12145=ORIENTED_EDGE('',*,*,#8635,.T.);
#12146=ORIENTED_EDGE('',*,*,#8674,.F.);
#12147=ORIENTED_EDGE('',*,*,#8652,.T.);
#12148=ORIENTED_EDGE('',*,*,#8648,.T.);
#12149=ORIENTED_EDGE('',*,*,#8655,.T.);
#12150=ORIENTED_EDGE('',*,*,#8659,.T.);
#12151=ORIENTED_EDGE('',*,*,#8629,.T.);
#12152=ORIENTED_EDGE('',*,*,#8674,.T.);
#12153=ORIENTED_EDGE('',*,*,#8637,.T.);
#12154=ORIENTED_EDGE('',*,*,#8632,.T.);
#12155=ORIENTED_EDGE('',*,*,#8571,.T.);
#12156=ORIENTED_EDGE('',*,*,#8503,.T.);
#12157=ORIENTED_EDGE('',*,*,#8568,.T.);
#12158=ORIENTED_EDGE('',*,*,#8562,.T.);
#12159=ORIENTED_EDGE('',*,*,#8579,.T.);
#12160=ORIENTED_EDGE('',*,*,#8385,.T.);
#12161=ORIENTED_EDGE('',*,*,#8576,.T.);
#12162=ORIENTED_EDGE('',*,*,#8444,.T.);
#12163=ORIENTED_EDGE('',*,*,#8587,.T.);
#12164=ORIENTED_EDGE('',*,*,#8267,.T.);
#12165=ORIENTED_EDGE('',*,*,#8584,.T.);
#12166=ORIENTED_EDGE('',*,*,#8326,.T.);
#12167=ORIENTED_EDGE('',*,*,#8595,.T.);
#12168=ORIENTED_EDGE('',*,*,#8149,.T.);
#12169=ORIENTED_EDGE('',*,*,#8592,.T.);
#12170=ORIENTED_EDGE('',*,*,#8208,.T.);
#12171=ORIENTED_EDGE('',*,*,#8672,.T.);
#14524=PLANE('',#16116);
#14525=PLANE('',#16119);
#14526=PLANE('',#16122);
#14527=PLANE('',#16125);
#14528=PLANE('',#16128);
#14529=PLANE('',#16129);
#14530=PLANE('',#16130);
#14531=PLANE('',#16131);
#14532=PLANE('',#16132);
#14533=PLANE('',#16135);
#14534=PLANE('',#16138);
#14535=PLANE('',#16141);
#14536=PLANE('',#16144);
#14537=PLANE('',#16145);
#14538=PLANE('',#16146);
#14539=PLANE('',#16147);
#14540=PLANE('',#16148);
#14541=PLANE('',#16149);
#14542=PLANE('',#16150);
#14543=PLANE('',#16151);
#14544=PLANE('',#16155);
#14545=PLANE('',#16158);
#14546=PLANE('',#16159);
#14547=PLANE('',#16160);
#14548=PLANE('',#16161);
#14549=PLANE('',#16163);
#14550=PLANE('',#16166);
#14551=PLANE('',#16172);
#14552=PLANE('',#16174);
#14553=PLANE('',#16183);
#14665=ADVANCED_FACE('',(#2685),#1726,.F.);
#14666=ADVANCED_FACE('',(#2686),#1727,.F.);
#14667=ADVANCED_FACE('',(#2687),#1728,.F.);
#14668=ADVANCED_FACE('',(#2688),#1729,.F.);
#14669=ADVANCED_FACE('',(#2689),#1730,.F.);
#14670=ADVANCED_FACE('',(#2690),#1731,.F.);
#14671=ADVANCED_FACE('',(#2691),#1732,.F.);
#14672=ADVANCED_FACE('',(#2692),#1733,.F.);
#14673=ADVANCED_FACE('',(#2693),#1734,.F.);
#14674=ADVANCED_FACE('',(#2694),#1735,.F.);
#14675=ADVANCED_FACE('',(#2695),#1736,.F.);
#14676=ADVANCED_FACE('',(#2696),#1737,.F.);
#14677=ADVANCED_FACE('',(#2697),#1738,.F.);
#14678=ADVANCED_FACE('',(#2698),#1739,.F.);
#14679=ADVANCED_FACE('',(#2699),#1740,.F.);
#14680=ADVANCED_FACE('',(#2700),#1741,.F.);
#14681=ADVANCED_FACE('',(#2701),#1742,.F.);
#14682=ADVANCED_FACE('',(#2702),#1743,.F.);
#14683=ADVANCED_FACE('',(#2703),#1744,.F.);
#14684=ADVANCED_FACE('',(#2704),#1745,.F.);
#14685=ADVANCED_FACE('',(#2705),#1746,.F.);
#14686=ADVANCED_FACE('',(#2706),#1747,.F.);
#14687=ADVANCED_FACE('',(#2707),#1748,.F.);
#14688=ADVANCED_FACE('',(#2708),#1749,.F.);
#14689=ADVANCED_FACE('',(#2709),#1750,.F.);
#14690=ADVANCED_FACE('',(#2710),#1751,.F.);
#14691=ADVANCED_FACE('',(#2711),#1752,.F.);
#14692=ADVANCED_FACE('',(#2712),#1753,.F.);
#14693=ADVANCED_FACE('',(#2713),#1754,.F.);
#14694=ADVANCED_FACE('',(#2714),#1755,.F.);
#14695=ADVANCED_FACE('',(#2715),#1756,.F.);
#14696=ADVANCED_FACE('',(#2716),#1757,.F.);
#14697=ADVANCED_FACE('',(#2717),#1758,.F.);
#14698=ADVANCED_FACE('',(#2718),#1759,.F.);
#14699=ADVANCED_FACE('',(#2719),#1760,.F.);
#14700=ADVANCED_FACE('',(#2720),#1761,.F.);
#14701=ADVANCED_FACE('',(#2721),#1762,.F.);
#14702=ADVANCED_FACE('',(#2722),#1763,.F.);
#14703=ADVANCED_FACE('',(#2723),#1764,.F.);
#14704=ADVANCED_FACE('',(#2724),#1765,.F.);
#14705=ADVANCED_FACE('',(#2725),#1766,.F.);
#14706=ADVANCED_FACE('',(#2726),#1767,.F.);
#14707=ADVANCED_FACE('',(#2727),#1768,.F.);
#14708=ADVANCED_FACE('',(#2728),#1769,.F.);
#14709=ADVANCED_FACE('',(#2729),#1770,.F.);
#14710=ADVANCED_FACE('',(#2730),#1771,.F.);
#14711=ADVANCED_FACE('',(#2731),#1772,.F.);
#14712=ADVANCED_FACE('',(#2732),#1773,.F.);
#14713=ADVANCED_FACE('',(#2733),#1774,.F.);
#14714=ADVANCED_FACE('',(#2734),#1775,.F.);
#14715=ADVANCED_FACE('',(#2735),#1776,.F.);
#14716=ADVANCED_FACE('',(#2736),#1777,.F.);
#14717=ADVANCED_FACE('',(#2737),#1778,.F.);
#14718=ADVANCED_FACE('',(#2738),#1779,.F.);
#14719=ADVANCED_FACE('',(#2739),#1780,.F.);
#14720=ADVANCED_FACE('',(#2740),#1781,.F.);
#14721=ADVANCED_FACE('',(#2741),#1782,.F.);
#14722=ADVANCED_FACE('',(#2742),#1783,.F.);
#14723=ADVANCED_FACE('',(#2743),#1784,.F.);
#14724=ADVANCED_FACE('',(#2744),#1785,.F.);
#14725=ADVANCED_FACE('',(#2745),#1786,.F.);
#14726=ADVANCED_FACE('',(#2746),#1787,.F.);
#14727=ADVANCED_FACE('',(#2747),#1788,.F.);
#14728=ADVANCED_FACE('',(#2748),#1789,.F.);
#14729=ADVANCED_FACE('',(#2749),#1790,.F.);
#14730=ADVANCED_FACE('',(#2750),#1791,.F.);
#14731=ADVANCED_FACE('',(#2751),#1792,.F.);
#14732=ADVANCED_FACE('',(#2752),#1793,.F.);
#14733=ADVANCED_FACE('',(#2753),#1794,.F.);
#14734=ADVANCED_FACE('',(#2754),#1795,.F.);
#14735=ADVANCED_FACE('',(#2755),#1796,.F.);
#14736=ADVANCED_FACE('',(#2756),#1797,.F.);
#14737=ADVANCED_FACE('',(#2757),#1798,.F.);
#14738=ADVANCED_FACE('',(#2758),#1799,.F.);
#14739=ADVANCED_FACE('',(#2759),#1800,.F.);
#14740=ADVANCED_FACE('',(#2760),#1801,.F.);
#14741=ADVANCED_FACE('',(#2761),#1802,.F.);
#14742=ADVANCED_FACE('',(#2762),#1803,.F.);
#14743=ADVANCED_FACE('',(#2763),#1804,.F.);
#14744=ADVANCED_FACE('',(#2764),#1805,.F.);
#14745=ADVANCED_FACE('',(#2765),#1806,.F.);
#14746=ADVANCED_FACE('',(#2766),#1807,.F.);
#14747=ADVANCED_FACE('',(#2767),#1808,.F.);
#14748=ADVANCED_FACE('',(#2768),#1809,.F.);
#14749=ADVANCED_FACE('',(#2769),#1810,.F.);
#14750=ADVANCED_FACE('',(#2770),#1811,.F.);
#14751=ADVANCED_FACE('',(#2771),#1812,.F.);
#14752=ADVANCED_FACE('',(#2772),#1813,.F.);
#14753=ADVANCED_FACE('',(#2773),#1814,.F.);
#14754=ADVANCED_FACE('',(#2774),#1815,.F.);
#14755=ADVANCED_FACE('',(#2775),#1816,.F.);
#14756=ADVANCED_FACE('',(#2776),#1817,.F.);
#14757=ADVANCED_FACE('',(#2777),#1818,.F.);
#14758=ADVANCED_FACE('',(#2778),#1819,.F.);
#14759=ADVANCED_FACE('',(#2779),#1820,.F.);
#14760=ADVANCED_FACE('',(#2780),#1821,.F.);
#14761=ADVANCED_FACE('',(#2781),#1822,.F.);
#14762=ADVANCED_FACE('',(#2782),#1823,.F.);
#14763=ADVANCED_FACE('',(#2783),#1824,.F.);
#14764=ADVANCED_FACE('',(#2784),#1825,.F.);
#14765=ADVANCED_FACE('',(#2785),#1826,.F.);
#14766=ADVANCED_FACE('',(#2786),#1827,.F.);
#14767=ADVANCED_FACE('',(#2787),#1828,.F.);
#14768=ADVANCED_FACE('',(#2788),#1829,.F.);
#14769=ADVANCED_FACE('',(#2789),#1830,.F.);
#14770=ADVANCED_FACE('',(#2790),#1831,.F.);
#14771=ADVANCED_FACE('',(#2791),#1832,.F.);
#14772=ADVANCED_FACE('',(#2792),#1833,.F.);
#14773=ADVANCED_FACE('',(#2793),#1834,.F.);
#14774=ADVANCED_FACE('',(#2794),#1835,.F.);
#14775=ADVANCED_FACE('',(#2795),#1836,.F.);
#14776=ADVANCED_FACE('',(#2796),#1837,.F.);
#14777=ADVANCED_FACE('',(#2797),#1838,.F.);
#14778=ADVANCED_FACE('',(#2798),#1839,.F.);
#14779=ADVANCED_FACE('',(#2799),#1840,.F.);
#14780=ADVANCED_FACE('',(#2800),#1841,.F.);
#14781=ADVANCED_FACE('',(#2801),#1842,.F.);
#14782=ADVANCED_FACE('',(#2802),#1843,.F.);
#14783=ADVANCED_FACE('',(#2803),#1844,.F.);
#14784=ADVANCED_FACE('',(#2804),#1845,.F.);
#14785=ADVANCED_FACE('',(#2805),#1846,.F.);
#14786=ADVANCED_FACE('',(#2806),#1847,.F.);
#14787=ADVANCED_FACE('',(#2807),#1848,.F.);
#14788=ADVANCED_FACE('',(#2808),#1849,.F.);
#14789=ADVANCED_FACE('',(#2809),#1850,.F.);
#14790=ADVANCED_FACE('',(#2810),#1851,.F.);
#14791=ADVANCED_FACE('',(#2811),#1852,.F.);
#14792=ADVANCED_FACE('',(#2812),#1853,.F.);
#14793=ADVANCED_FACE('',(#2813),#1854,.F.);
#14794=ADVANCED_FACE('',(#2814),#1855,.F.);
#14795=ADVANCED_FACE('',(#2815),#1856,.F.);
#14796=ADVANCED_FACE('',(#2816),#1857,.F.);
#14797=ADVANCED_FACE('',(#2817),#1858,.F.);
#14798=ADVANCED_FACE('',(#2818),#1859,.F.);
#14799=ADVANCED_FACE('',(#2819),#1860,.F.);
#14800=ADVANCED_FACE('',(#2820),#1861,.F.);
#14801=ADVANCED_FACE('',(#2821),#1862,.F.);
#14802=ADVANCED_FACE('',(#2822),#1863,.F.);
#14803=ADVANCED_FACE('',(#2823),#1864,.F.);
#14804=ADVANCED_FACE('',(#2824),#1865,.F.);
#14805=ADVANCED_FACE('',(#2825),#1866,.F.);
#14806=ADVANCED_FACE('',(#2826),#1867,.F.);
#14807=ADVANCED_FACE('',(#2827),#1868,.F.);
#14808=ADVANCED_FACE('',(#2828),#1869,.F.);
#14809=ADVANCED_FACE('',(#2829),#1870,.F.);
#14810=ADVANCED_FACE('',(#2830),#1871,.F.);
#14811=ADVANCED_FACE('',(#2831),#1872,.F.);
#14812=ADVANCED_FACE('',(#2832),#1873,.F.);
#14813=ADVANCED_FACE('',(#2833),#1874,.F.);
#14814=ADVANCED_FACE('',(#2834),#1875,.F.);
#14815=ADVANCED_FACE('',(#2835),#1876,.F.);
#14816=ADVANCED_FACE('',(#2836),#1877,.F.);
#14817=ADVANCED_FACE('',(#2837),#1878,.F.);
#14818=ADVANCED_FACE('',(#2838),#1879,.F.);
#14819=ADVANCED_FACE('',(#2839),#1880,.F.);
#14820=ADVANCED_FACE('',(#2840),#1881,.F.);
#14821=ADVANCED_FACE('',(#2841),#1882,.F.);
#14822=ADVANCED_FACE('',(#2842),#1883,.F.);
#14823=ADVANCED_FACE('',(#2843),#1884,.F.);
#14824=ADVANCED_FACE('',(#2844),#1885,.F.);
#14825=ADVANCED_FACE('',(#2845),#1886,.F.);
#14826=ADVANCED_FACE('',(#2846),#1887,.F.);
#14827=ADVANCED_FACE('',(#2847),#1888,.F.);
#14828=ADVANCED_FACE('',(#2848),#1889,.F.);
#14829=ADVANCED_FACE('',(#2849),#1890,.F.);
#14830=ADVANCED_FACE('',(#2850),#1891,.F.);
#14831=ADVANCED_FACE('',(#2851),#1892,.F.);
#14832=ADVANCED_FACE('',(#2852),#1893,.F.);
#14833=ADVANCED_FACE('',(#2853),#1894,.F.);
#14834=ADVANCED_FACE('',(#2854),#1895,.F.);
#14835=ADVANCED_FACE('',(#2855),#1896,.F.);
#14836=ADVANCED_FACE('',(#2856),#1897,.F.);
#14837=ADVANCED_FACE('',(#2857),#1898,.F.);
#14838=ADVANCED_FACE('',(#2858),#1899,.F.);
#14839=ADVANCED_FACE('',(#2859),#1900,.F.);
#14840=ADVANCED_FACE('',(#2860),#1901,.F.);
#14841=ADVANCED_FACE('',(#2861),#1902,.F.);
#14842=ADVANCED_FACE('',(#2862),#1903,.F.);
#14843=ADVANCED_FACE('',(#2863),#1904,.F.);
#14844=ADVANCED_FACE('',(#2864),#1905,.F.);
#14845=ADVANCED_FACE('',(#2865),#1906,.F.);
#14846=ADVANCED_FACE('',(#2866),#1907,.F.);
#14847=ADVANCED_FACE('',(#2867),#1908,.F.);
#14848=ADVANCED_FACE('',(#2868),#1909,.F.);
#14849=ADVANCED_FACE('',(#2869),#1910,.F.);
#14850=ADVANCED_FACE('',(#2870),#1911,.F.);
#14851=ADVANCED_FACE('',(#2871),#1912,.F.);
#14852=ADVANCED_FACE('',(#2872),#1913,.F.);
#14853=ADVANCED_FACE('',(#2873),#1914,.F.);
#14854=ADVANCED_FACE('',(#2874),#1915,.F.);
#14855=ADVANCED_FACE('',(#2875),#1916,.F.);
#14856=ADVANCED_FACE('',(#2876),#1917,.F.);
#14857=ADVANCED_FACE('',(#2877),#1918,.F.);
#14858=ADVANCED_FACE('',(#2878),#1919,.F.);
#14859=ADVANCED_FACE('',(#2879),#1920,.F.);
#14860=ADVANCED_FACE('',(#2880),#1921,.F.);
#14861=ADVANCED_FACE('',(#2881),#1922,.F.);
#14862=ADVANCED_FACE('',(#2882),#1923,.F.);
#14863=ADVANCED_FACE('',(#2883),#1924,.F.);
#14864=ADVANCED_FACE('',(#2884),#1925,.F.);
#14865=ADVANCED_FACE('',(#2885),#1926,.F.);
#14866=ADVANCED_FACE('',(#2886),#1927,.F.);
#14867=ADVANCED_FACE('',(#2887),#1928,.F.);
#14868=ADVANCED_FACE('',(#2888),#1929,.F.);
#14869=ADVANCED_FACE('',(#2889),#1930,.F.);
#14870=ADVANCED_FACE('',(#2890),#1931,.F.);
#14871=ADVANCED_FACE('',(#2891),#1932,.F.);
#14872=ADVANCED_FACE('',(#2892),#1933,.F.);
#14873=ADVANCED_FACE('',(#2893),#1934,.F.);
#14874=ADVANCED_FACE('',(#2894),#1935,.F.);
#14875=ADVANCED_FACE('',(#2895),#1936,.F.);
#14876=ADVANCED_FACE('',(#2896),#1937,.F.);
#14877=ADVANCED_FACE('',(#2897),#1938,.F.);
#14878=ADVANCED_FACE('',(#2898),#1939,.F.);
#14879=ADVANCED_FACE('',(#2899),#1940,.F.);
#14880=ADVANCED_FACE('',(#2900),#1941,.F.);
#14881=ADVANCED_FACE('',(#2901),#1942,.F.);
#14882=ADVANCED_FACE('',(#2902),#1943,.F.);
#14883=ADVANCED_FACE('',(#2903),#1944,.F.);
#14884=ADVANCED_FACE('',(#2904),#1945,.F.);
#14885=ADVANCED_FACE('',(#2905),#1946,.F.);
#14886=ADVANCED_FACE('',(#2906),#1947,.F.);
#14887=ADVANCED_FACE('',(#2907),#1948,.F.);
#14888=ADVANCED_FACE('',(#2908),#1949,.F.);
#14889=ADVANCED_FACE('',(#2909),#1950,.F.);
#14890=ADVANCED_FACE('',(#2910),#1951,.F.);
#14891=ADVANCED_FACE('',(#2911),#1952,.F.);
#14892=ADVANCED_FACE('',(#2912),#1953,.F.);
#14893=ADVANCED_FACE('',(#2913),#1954,.F.);
#14894=ADVANCED_FACE('',(#2914),#1955,.F.);
#14895=ADVANCED_FACE('',(#2915),#1956,.F.);
#14896=ADVANCED_FACE('',(#2916),#1957,.F.);
#14897=ADVANCED_FACE('',(#2917),#1958,.F.);
#14898=ADVANCED_FACE('',(#2918),#1959,.F.);
#14899=ADVANCED_FACE('',(#2919),#1960,.F.);
#14900=ADVANCED_FACE('',(#2920),#1961,.F.);
#14901=ADVANCED_FACE('',(#2921),#1962,.F.);
#14902=ADVANCED_FACE('',(#2922),#1963,.F.);
#14903=ADVANCED_FACE('',(#2923),#1964,.F.);
#14904=ADVANCED_FACE('',(#2924),#1965,.F.);
#14905=ADVANCED_FACE('',(#2925),#1966,.F.);
#14906=ADVANCED_FACE('',(#2926),#1967,.F.);
#14907=ADVANCED_FACE('',(#2927),#1968,.F.);
#14908=ADVANCED_FACE('',(#2928),#1969,.F.);
#14909=ADVANCED_FACE('',(#2929),#1970,.F.);
#14910=ADVANCED_FACE('',(#2930),#1971,.F.);
#14911=ADVANCED_FACE('',(#2931),#1972,.F.);
#14912=ADVANCED_FACE('',(#2932),#1973,.F.);
#14913=ADVANCED_FACE('',(#2933),#1974,.F.);
#14914=ADVANCED_FACE('',(#2934),#1975,.F.);
#14915=ADVANCED_FACE('',(#2935),#1976,.F.);
#14916=ADVANCED_FACE('',(#2936),#1977,.F.);
#14917=ADVANCED_FACE('',(#2937),#1978,.F.);
#14918=ADVANCED_FACE('',(#2938),#1979,.F.);
#14919=ADVANCED_FACE('',(#2939),#1980,.F.);
#14920=ADVANCED_FACE('',(#2940),#1981,.F.);
#14921=ADVANCED_FACE('',(#2941),#1982,.F.);
#14922=ADVANCED_FACE('',(#2942),#1983,.F.);
#14923=ADVANCED_FACE('',(#2943),#1984,.F.);
#14924=ADVANCED_FACE('',(#2944),#1985,.F.);
#14925=ADVANCED_FACE('',(#2945),#1986,.F.);
#14926=ADVANCED_FACE('',(#2946),#1987,.F.);
#14927=ADVANCED_FACE('',(#2947),#1988,.F.);
#14928=ADVANCED_FACE('',(#2948),#1989,.F.);
#14929=ADVANCED_FACE('',(#2949),#1990,.F.);
#14930=ADVANCED_FACE('',(#2950),#1991,.F.);
#14931=ADVANCED_FACE('',(#2951),#1992,.F.);
#14932=ADVANCED_FACE('',(#2952),#1993,.F.);
#14933=ADVANCED_FACE('',(#2953),#1994,.F.);
#14934=ADVANCED_FACE('',(#2954),#1995,.F.);
#14935=ADVANCED_FACE('',(#2955),#1996,.F.);
#14936=ADVANCED_FACE('',(#2956),#1997,.F.);
#14937=ADVANCED_FACE('',(#2957),#1998,.F.);
#14938=ADVANCED_FACE('',(#2958),#1999,.F.);
#14939=ADVANCED_FACE('',(#2959),#2000,.F.);
#14940=ADVANCED_FACE('',(#2960),#2001,.F.);
#14941=ADVANCED_FACE('',(#2961),#2002,.F.);
#14942=ADVANCED_FACE('',(#2962),#2003,.F.);
#14943=ADVANCED_FACE('',(#2963),#2004,.F.);
#14944=ADVANCED_FACE('',(#2964),#2005,.F.);
#14945=ADVANCED_FACE('',(#2965),#2006,.F.);
#14946=ADVANCED_FACE('',(#2966),#2007,.F.);
#14947=ADVANCED_FACE('',(#2967),#2008,.F.);
#14948=ADVANCED_FACE('',(#2968),#2009,.F.);
#14949=ADVANCED_FACE('',(#2969),#2010,.F.);
#14950=ADVANCED_FACE('',(#2970),#2011,.F.);
#14951=ADVANCED_FACE('',(#2971),#2012,.F.);
#14952=ADVANCED_FACE('',(#2972),#2013,.F.);
#14953=ADVANCED_FACE('',(#2973),#2014,.F.);
#14954=ADVANCED_FACE('',(#2974),#2015,.F.);
#14955=ADVANCED_FACE('',(#2975),#2016,.F.);
#14956=ADVANCED_FACE('',(#2976),#2017,.F.);
#14957=ADVANCED_FACE('',(#2977),#2018,.F.);
#14958=ADVANCED_FACE('',(#2978),#2019,.F.);
#14959=ADVANCED_FACE('',(#2979),#2020,.F.);
#14960=ADVANCED_FACE('',(#2980),#2021,.F.);
#14961=ADVANCED_FACE('',(#2981),#2022,.F.);
#14962=ADVANCED_FACE('',(#2982),#2023,.F.);
#14963=ADVANCED_FACE('',(#2983),#2024,.F.);
#14964=ADVANCED_FACE('',(#2984),#2025,.F.);
#14965=ADVANCED_FACE('',(#2985),#2026,.F.);
#14966=ADVANCED_FACE('',(#2986),#2027,.F.);
#14967=ADVANCED_FACE('',(#2987),#2028,.F.);
#14968=ADVANCED_FACE('',(#2988),#2029,.F.);
#14969=ADVANCED_FACE('',(#2989),#2030,.F.);
#14970=ADVANCED_FACE('',(#2990),#2031,.F.);
#14971=ADVANCED_FACE('',(#2991),#2032,.F.);
#14972=ADVANCED_FACE('',(#2992),#2033,.F.);
#14973=ADVANCED_FACE('',(#2993),#2034,.F.);
#14974=ADVANCED_FACE('',(#2994),#2035,.F.);
#14975=ADVANCED_FACE('',(#2995),#14524,.T.);
#14976=ADVANCED_FACE('',(#2996),#2036,.F.);
#14977=ADVANCED_FACE('',(#2997),#240,.F.);
#14978=ADVANCED_FACE('',(#2998),#241,.F.);
#14979=ADVANCED_FACE('',(#2999),#2037,.F.);
#14980=ADVANCED_FACE('',(#3000),#14525,.T.);
#14981=ADVANCED_FACE('',(#3001),#2038,.F.);
#14982=ADVANCED_FACE('',(#3002),#242,.F.);
#14983=ADVANCED_FACE('',(#3003),#243,.F.);
#14984=ADVANCED_FACE('',(#3004),#2039,.F.);
#14985=ADVANCED_FACE('',(#3005),#14526,.T.);
#14986=ADVANCED_FACE('',(#3006),#2040,.F.);
#14987=ADVANCED_FACE('',(#3007),#244,.F.);
#14988=ADVANCED_FACE('',(#3008),#245,.F.);
#14989=ADVANCED_FACE('',(#3009),#2041,.F.);
#14990=ADVANCED_FACE('',(#3010),#14527,.T.);
#14991=ADVANCED_FACE('',(#3011),#2042,.F.);
#14992=ADVANCED_FACE('',(#3012),#246,.F.);
#14993=ADVANCED_FACE('',(#3013),#247,.F.);
#14994=ADVANCED_FACE('',(#3014),#2043,.F.);
#14995=ADVANCED_FACE('',(#3015),#14528,.F.);
#14996=ADVANCED_FACE('',(#3016),#14529,.F.);
#14997=ADVANCED_FACE('',(#3017),#14530,.F.);
#14998=ADVANCED_FACE('',(#3018),#14531,.F.);
#14999=ADVANCED_FACE('',(#3019),#14532,.F.);
#15000=ADVANCED_FACE('',(#3020),#2044,.F.);
#15001=ADVANCED_FACE('',(#3021),#248,.F.);
#15002=ADVANCED_FACE('',(#3022),#249,.F.);
#15003=ADVANCED_FACE('',(#3023),#2045,.F.);
#15004=ADVANCED_FACE('',(#3024),#14533,.F.);
#15005=ADVANCED_FACE('',(#3025),#2046,.F.);
#15006=ADVANCED_FACE('',(#3026),#250,.F.);
#15007=ADVANCED_FACE('',(#3027),#251,.F.);
#15008=ADVANCED_FACE('',(#3028),#2047,.F.);
#15009=ADVANCED_FACE('',(#3029),#14534,.F.);
#15010=ADVANCED_FACE('',(#3030),#2048,.F.);
#15011=ADVANCED_FACE('',(#3031),#252,.F.);
#15012=ADVANCED_FACE('',(#3032),#253,.F.);
#15013=ADVANCED_FACE('',(#3033),#2049,.F.);
#15014=ADVANCED_FACE('',(#3034),#14535,.F.);
#15015=ADVANCED_FACE('',(#3035),#2050,.F.);
#15016=ADVANCED_FACE('',(#3036),#254,.F.);
#15017=ADVANCED_FACE('',(#3037),#255,.F.);
#15018=ADVANCED_FACE('',(#3038),#2051,.F.);
#15019=ADVANCED_FACE('',(#3039),#14536,.F.);
#15020=ADVANCED_FACE('',(#3040),#14537,.F.);
#15021=ADVANCED_FACE('',(#3041),#14538,.F.);
#15022=ADVANCED_FACE('',(#3042),#14539,.F.);
#15023=ADVANCED_FACE('',(#3043),#14540,.F.);
#15024=ADVANCED_FACE('',(#3044),#14541,.F.);
#15025=ADVANCED_FACE('',(#3045),#14542,.F.);
#15026=ADVANCED_FACE('',(#3046,#1644,#1645,#1646,#1647,#1648),#14543,.F.);
#15027=ADVANCED_FACE('',(#3047),#2052,.F.);
#15028=ADVANCED_FACE('',(#3048),#256,.F.);
#15029=ADVANCED_FACE('',(#3049),#257,.F.);
#15030=ADVANCED_FACE('',(#3050,#1649),#14544,.T.);
#15031=ADVANCED_FACE('',(#3051),#2053,.F.);
#15032=ADVANCED_FACE('',(#3052),#14545,.T.);
#15033=ADVANCED_FACE('',(#3053),#14546,.T.);
#15034=ADVANCED_FACE('',(#3054),#14547,.T.);
#15035=ADVANCED_FACE('',(#3055,#1650),#14548,.F.);
#15036=ADVANCED_FACE('',(#3056,#1651),#14549,.T.);
#15037=ADVANCED_FACE('',(#3057,#1652),#14550,.F.);
#15038=ADVANCED_FACE('',(#3058),#2054,.F.);
#15039=ADVANCED_FACE('',(#3059),#2055,.F.);
#15040=ADVANCED_FACE('',(#3060,#1653),#14551,.T.);
#15041=ADVANCED_FACE('',(#3061,#1654),#14552,.F.);
#15042=ADVANCED_FACE('',(#3062),#2056,.F.);
#15043=ADVANCED_FACE('',(#3063),#2057,.F.);
#15044=ADVANCED_FACE('',(#3064),#2058,.F.);
#15045=ADVANCED_FACE('',(#3065,#1655),#2059,.T.);
#15046=ADVANCED_FACE('',(#3066,#1656,#1657,#1658,#1659,#1660),#14553,.T.);
#15479=CLOSED_SHELL('',(#14665,#14666,#14667,#14668,#14669,#14670,#14671,
#14672,#14673,#14674,#14675,#14676,#14677,#14678,#14679,#14680,#14681,#14682,
#14683,#14684,#14685,#14686,#14687,#14688,#14689,#14690,#14691,#14692,#14693,
#14694,#14695,#14696,#14697,#14698,#14699,#14700,#14701,#14702,#14703,#14704,
#14705,#14706,#14707,#14708,#14709,#14710,#14711,#14712,#14713,#14714,#14715,
#14716,#14717,#14718,#14719,#14720,#14721,#14722,#14723,#14724,#14725,#14726,
#14727,#14728,#14729,#14730,#14731,#14732,#14733,#14734,#14735,#14736,#14737,
#14738,#14739,#14740,#14741,#14742,#14743,#14744,#14745,#14746,#14747,#14748,
#14749,#14750,#14751,#14752,#14753,#14754,#14755,#14756,#14757,#14758,#14759,
#14760,#14761,#14762,#14763,#14764,#14765,#14766,#14767,#14768,#14769,#14770,
#14771,#14772,#14773,#14774,#14775,#14776,#14777,#14778,#14779,#14780,#14781,
#14782,#14783,#14784,#14785,#14786,#14787,#14788,#14789,#14790,#14791,#14792,
#14793,#14794,#14795,#14796,#14797,#14798,#14799,#14800,#14801,#14802,#14803,
#14804,#14805,#14806,#14807,#14808,#14809,#14810,#14811,#14812,#14813,#14814,
#14815,#14816,#14817,#14818,#14819,#14820,#14821,#14822,#14823,#14824,#14825,
#14826,#14827,#14828,#14829,#14830,#14831,#14832,#14833,#14834,#14835,#14836,
#14837,#14838,#14839,#14840,#14841,#14842,#14843,#14844,#14845,#14846,#14847,
#14848,#14849,#14850,#14851,#14852,#14853,#14854,#14855,#14856,#14857,#14858,
#14859,#14860,#14861,#14862,#14863,#14864,#14865,#14866,#14867,#14868,#14869,
#14870,#14871,#14872,#14873,#14874,#14875,#14876,#14877,#14878,#14879,#14880,
#14881,#14882,#14883,#14884,#14885,#14886,#14887,#14888,#14889,#14890,#14891,
#14892,#14893,#14894,#14895,#14896,#14897,#14898,#14899,#14900,#14901,#14902,
#14903,#14904,#14905,#14906,#14907,#14908,#14909,#14910,#14911,#14912,#14913,
#14914,#14915,#14916,#14917,#14918,#14919,#14920,#14921,#14922,#14923,#14924,
#14925,#14926,#14927,#14928,#14929,#14930,#14931,#14932,#14933,#14934,#14935,
#14936,#14937,#14938,#14939,#14940,#14941,#14942,#14943,#14944,#14945,#14946,
#14947,#14948,#14949,#14950,#14951,#14952,#14953,#14954,#14955,#14956,#14957,
#14958,#14959,#14960,#14961,#14962,#14963,#14964,#14965,#14966,#14967,#14968,
#14969,#14970,#14971,#14972,#14973,#14974,#14975,#14976,#14977,#14978,#14979,
#14980,#14981,#14982,#14983,#14984,#14985,#14986,#14987,#14988,#14989,#14990,
#14991,#14992,#14993,#14994,#14995,#14996,#14997,#14998,#14999,#15000,#15001,
#15002,#15003,#15004,#15005,#15006,#15007,#15008,#15009,#15010,#15011,#15012,
#15013,#15014,#15015,#15016,#15017,#15018,#15019,#15020,#15021,#15022,#15023,
#15024,#15025,#15026,#15027,#15028,#15029,#15030,#15031,#15032,#15033,#15034,
#15035,#15036,#15037,#15038,#15039,#15040,#15041,#15042,#15043,#15044,#15045,
#15046));
#15752=AXIS2_PLACEMENT_3D('',#20082,#17006,#17007);
#15753=AXIS2_PLACEMENT_3D('',#20083,#17008,#17009);
#15754=AXIS2_PLACEMENT_3D('',#20088,#17011,#17012);
#15755=AXIS2_PLACEMENT_3D('',#20102,#17013,#17014);
#15756=AXIS2_PLACEMENT_3D('',#20147,#17016,#17017);
#15757=AXIS2_PLACEMENT_3D('',#20191,#17018,#17019);
#15758=AXIS2_PLACEMENT_3D('',#20278,#17021,#17022);
#15759=AXIS2_PLACEMENT_3D('',#20368,#17024,#17025);
#15760=AXIS2_PLACEMENT_3D('',#20455,#17027,#17028);
#15761=AXIS2_PLACEMENT_3D('',#20545,#17030,#17031);
#15762=AXIS2_PLACEMENT_3D('',#20576,#17033,#17034);
#15763=AXIS2_PLACEMENT_3D('',#20614,#17035,#17036);
#15764=AXIS2_PLACEMENT_3D('',#20631,#17038,#17039);
#15765=AXIS2_PLACEMENT_3D('',#20644,#17040,#17041);
#15766=AXIS2_PLACEMENT_3D('',#20682,#17043,#17044);
#15767=AXIS2_PLACEMENT_3D('',#20719,#17046,#17047);
#15768=AXIS2_PLACEMENT_3D('',#20756,#17049,#17050);
#15769=AXIS2_PLACEMENT_3D('',#20794,#17052,#17053);
#15770=AXIS2_PLACEMENT_3D('',#20832,#17055,#17056);
#15771=AXIS2_PLACEMENT_3D('',#20844,#17058,#17059);
#15772=AXIS2_PLACEMENT_3D('',#20852,#17060,#17061);
#15773=AXIS2_PLACEMENT_3D('',#20874,#17063,#17064);
#15774=AXIS2_PLACEMENT_3D('',#20877,#17066,#17067);
#15775=AXIS2_PLACEMENT_3D('',#20879,#17068,#17069);
#15776=AXIS2_PLACEMENT_3D('',#20902,#17070,#17071);
#15777=AXIS2_PLACEMENT_3D('',#20950,#17073,#17074);
#15778=AXIS2_PLACEMENT_3D('',#20998,#17076,#17077);
#15779=AXIS2_PLACEMENT_3D('',#21049,#17079,#17080);
#15780=AXIS2_PLACEMENT_3D('',#21100,#17082,#17083);
#15781=AXIS2_PLACEMENT_3D('',#21148,#17085,#17086);
#15782=AXIS2_PLACEMENT_3D('',#21199,#17088,#17089);
#15783=AXIS2_PLACEMENT_3D('',#21250,#17091,#17092);
#15784=AXIS2_PLACEMENT_3D('',#21298,#17094,#17095);
#15785=AXIS2_PLACEMENT_3D('',#21346,#17097,#17098);
#15786=AXIS2_PLACEMENT_3D('',#21400,#17100,#17101);
#15787=AXIS2_PLACEMENT_3D('',#21448,#17103,#17104);
#15788=AXIS2_PLACEMENT_3D('',#21496,#17106,#17107);
#15789=AXIS2_PLACEMENT_3D('',#21547,#17109,#17110);
#15790=AXIS2_PLACEMENT_3D('',#21598,#17112,#17113);
#15791=AXIS2_PLACEMENT_3D('',#21646,#17115,#17116);
#15792=AXIS2_PLACEMENT_3D('',#21697,#17118,#17119);
#15793=AXIS2_PLACEMENT_3D('',#21716,#17121,#17122);
#15794=AXIS2_PLACEMENT_3D('',#21736,#17123,#17124);
#15795=AXIS2_PLACEMENT_3D('',#21747,#17126,#17127);
#15796=AXIS2_PLACEMENT_3D('',#21754,#17128,#17129);
#15797=AXIS2_PLACEMENT_3D('',#21779,#17131,#17132);
#15798=AXIS2_PLACEMENT_3D('',#21803,#17134,#17135);
#15799=AXIS2_PLACEMENT_3D('',#21828,#17137,#17138);
#15800=AXIS2_PLACEMENT_3D('',#21852,#17140,#17141);
#15801=AXIS2_PLACEMENT_3D('',#21877,#17143,#17144);
#15802=AXIS2_PLACEMENT_3D('',#21902,#17146,#17147);
#15803=AXIS2_PLACEMENT_3D('',#21926,#17149,#17150);
#15804=AXIS2_PLACEMENT_3D('',#21951,#17152,#17153);
#15805=AXIS2_PLACEMENT_3D('',#21975,#17155,#17156);
#15806=AXIS2_PLACEMENT_3D('',#22000,#17158,#17159);
#15807=AXIS2_PLACEMENT_3D('',#22025,#17161,#17162);
#15808=AXIS2_PLACEMENT_3D('',#22049,#17164,#17165);
#15809=AXIS2_PLACEMENT_3D('',#22074,#17167,#17168);
#15810=AXIS2_PLACEMENT_3D('',#22098,#17170,#17171);
#15811=AXIS2_PLACEMENT_3D('',#22123,#17173,#17174);
#15812=AXIS2_PLACEMENT_3D('',#22148,#17176,#17177);
#15813=AXIS2_PLACEMENT_3D('',#22172,#17179,#17180);
#15814=AXIS2_PLACEMENT_3D('',#22183,#17182,#17183);
#15815=AXIS2_PLACEMENT_3D('',#22189,#17184,#17185);
#15816=AXIS2_PLACEMENT_3D('',#22211,#17187,#17188);
#15817=AXIS2_PLACEMENT_3D('',#22214,#17190,#17191);
#15818=AXIS2_PLACEMENT_3D('',#22216,#17192,#17193);
#15819=AXIS2_PLACEMENT_3D('',#22239,#17194,#17195);
#15820=AXIS2_PLACEMENT_3D('',#22287,#17197,#17198);
#15821=AXIS2_PLACEMENT_3D('',#22335,#17200,#17201);
#15822=AXIS2_PLACEMENT_3D('',#22386,#17203,#17204);
#15823=AXIS2_PLACEMENT_3D('',#22437,#17206,#17207);
#15824=AXIS2_PLACEMENT_3D('',#22485,#17209,#17210);
#15825=AXIS2_PLACEMENT_3D('',#22536,#17212,#17213);
#15826=AXIS2_PLACEMENT_3D('',#22587,#17215,#17216);
#15827=AXIS2_PLACEMENT_3D('',#22635,#17218,#17219);
#15828=AXIS2_PLACEMENT_3D('',#22683,#17221,#17222);
#15829=AXIS2_PLACEMENT_3D('',#22737,#17224,#17225);
#15830=AXIS2_PLACEMENT_3D('',#22785,#17227,#17228);
#15831=AXIS2_PLACEMENT_3D('',#22833,#17230,#17231);
#15832=AXIS2_PLACEMENT_3D('',#22884,#17233,#17234);
#15833=AXIS2_PLACEMENT_3D('',#22935,#17236,#17237);
#15834=AXIS2_PLACEMENT_3D('',#22983,#17239,#17240);
#15835=AXIS2_PLACEMENT_3D('',#23034,#17242,#17243);
#15836=AXIS2_PLACEMENT_3D('',#23053,#17245,#17246);
#15837=AXIS2_PLACEMENT_3D('',#23073,#17247,#17248);
#15838=AXIS2_PLACEMENT_3D('',#23084,#17250,#17251);
#15839=AXIS2_PLACEMENT_3D('',#23091,#17252,#17253);
#15840=AXIS2_PLACEMENT_3D('',#23116,#17255,#17256);
#15841=AXIS2_PLACEMENT_3D('',#23140,#17258,#17259);
#15842=AXIS2_PLACEMENT_3D('',#23165,#17261,#17262);
#15843=AXIS2_PLACEMENT_3D('',#23189,#17264,#17265);
#15844=AXIS2_PLACEMENT_3D('',#23214,#17267,#17268);
#15845=AXIS2_PLACEMENT_3D('',#23239,#17270,#17271);
#15846=AXIS2_PLACEMENT_3D('',#23263,#17273,#17274);
#15847=AXIS2_PLACEMENT_3D('',#23288,#17276,#17277);
#15848=AXIS2_PLACEMENT_3D('',#23312,#17279,#17280);
#15849=AXIS2_PLACEMENT_3D('',#23337,#17282,#17283);
#15850=AXIS2_PLACEMENT_3D('',#23362,#17285,#17286);
#15851=AXIS2_PLACEMENT_3D('',#23386,#17288,#17289);
#15852=AXIS2_PLACEMENT_3D('',#23411,#17291,#17292);
#15853=AXIS2_PLACEMENT_3D('',#23435,#17294,#17295);
#15854=AXIS2_PLACEMENT_3D('',#23460,#17297,#17298);
#15855=AXIS2_PLACEMENT_3D('',#23485,#17300,#17301);
#15856=AXIS2_PLACEMENT_3D('',#23509,#17303,#17304);
#15857=AXIS2_PLACEMENT_3D('',#23520,#17306,#17307);
#15858=AXIS2_PLACEMENT_3D('',#23526,#17308,#17309);
#15859=AXIS2_PLACEMENT_3D('',#23548,#17311,#17312);
#15860=AXIS2_PLACEMENT_3D('',#23551,#17314,#17315);
#15861=AXIS2_PLACEMENT_3D('',#23553,#17316,#17317);
#15862=AXIS2_PLACEMENT_3D('',#23576,#17318,#17319);
#15863=AXIS2_PLACEMENT_3D('',#23624,#17321,#17322);
#15864=AXIS2_PLACEMENT_3D('',#23672,#17324,#17325);
#15865=AXIS2_PLACEMENT_3D('',#23723,#17327,#17328);
#15866=AXIS2_PLACEMENT_3D('',#23774,#17330,#17331);
#15867=AXIS2_PLACEMENT_3D('',#23822,#17333,#17334);
#15868=AXIS2_PLACEMENT_3D('',#23873,#17336,#17337);
#15869=AXIS2_PLACEMENT_3D('',#23924,#17339,#17340);
#15870=AXIS2_PLACEMENT_3D('',#23972,#17342,#17343);
#15871=AXIS2_PLACEMENT_3D('',#24020,#17345,#17346);
#15872=AXIS2_PLACEMENT_3D('',#24074,#17348,#17349);
#15873=AXIS2_PLACEMENT_3D('',#24122,#17351,#17352);
#15874=AXIS2_PLACEMENT_3D('',#24170,#17354,#17355);
#15875=AXIS2_PLACEMENT_3D('',#24221,#17357,#17358);
#15876=AXIS2_PLACEMENT_3D('',#24272,#17360,#17361);
#15877=AXIS2_PLACEMENT_3D('',#24320,#17363,#17364);
#15878=AXIS2_PLACEMENT_3D('',#24371,#17366,#17367);
#15879=AXIS2_PLACEMENT_3D('',#24390,#17369,#17370);
#15880=AXIS2_PLACEMENT_3D('',#24410,#17371,#17372);
#15881=AXIS2_PLACEMENT_3D('',#24421,#17374,#17375);
#15882=AXIS2_PLACEMENT_3D('',#24428,#17376,#17377);
#15883=AXIS2_PLACEMENT_3D('',#24453,#17379,#17380);
#15884=AXIS2_PLACEMENT_3D('',#24477,#17382,#17383);
#15885=AXIS2_PLACEMENT_3D('',#24502,#17385,#17386);
#15886=AXIS2_PLACEMENT_3D('',#24526,#17388,#17389);
#15887=AXIS2_PLACEMENT_3D('',#24551,#17391,#17392);
#15888=AXIS2_PLACEMENT_3D('',#24576,#17394,#17395);
#15889=AXIS2_PLACEMENT_3D('',#24600,#17397,#17398);
#15890=AXIS2_PLACEMENT_3D('',#24625,#17400,#17401);
#15891=AXIS2_PLACEMENT_3D('',#24649,#17403,#17404);
#15892=AXIS2_PLACEMENT_3D('',#24674,#17406,#17407);
#15893=AXIS2_PLACEMENT_3D('',#24699,#17409,#17410);
#15894=AXIS2_PLACEMENT_3D('',#24723,#17412,#17413);
#15895=AXIS2_PLACEMENT_3D('',#24748,#17415,#17416);
#15896=AXIS2_PLACEMENT_3D('',#24772,#17418,#17419);
#15897=AXIS2_PLACEMENT_3D('',#24797,#17421,#17422);
#15898=AXIS2_PLACEMENT_3D('',#24822,#17424,#17425);
#15899=AXIS2_PLACEMENT_3D('',#24846,#17427,#17428);
#15900=AXIS2_PLACEMENT_3D('',#24857,#17430,#17431);
#15901=AXIS2_PLACEMENT_3D('',#24863,#17432,#17433);
#15902=AXIS2_PLACEMENT_3D('',#24885,#17435,#17436);
#15903=AXIS2_PLACEMENT_3D('',#24888,#17438,#17439);
#15904=AXIS2_PLACEMENT_3D('',#24890,#17440,#17441);
#15905=AXIS2_PLACEMENT_3D('',#24913,#17442,#17443);
#15906=AXIS2_PLACEMENT_3D('',#24961,#17445,#17446);
#15907=AXIS2_PLACEMENT_3D('',#25009,#17448,#17449);
#15908=AXIS2_PLACEMENT_3D('',#25060,#17451,#17452);
#15909=AXIS2_PLACEMENT_3D('',#25111,#17454,#17455);
#15910=AXIS2_PLACEMENT_3D('',#25159,#17457,#17458);
#15911=AXIS2_PLACEMENT_3D('',#25210,#17460,#17461);
#15912=AXIS2_PLACEMENT_3D('',#25261,#17463,#17464);
#15913=AXIS2_PLACEMENT_3D('',#25309,#17466,#17467);
#15914=AXIS2_PLACEMENT_3D('',#25357,#17469,#17470);
#15915=AXIS2_PLACEMENT_3D('',#25411,#17472,#17473);
#15916=AXIS2_PLACEMENT_3D('',#25459,#17475,#17476);
#15917=AXIS2_PLACEMENT_3D('',#25507,#17478,#17479);
#15918=AXIS2_PLACEMENT_3D('',#25558,#17481,#17482);
#15919=AXIS2_PLACEMENT_3D('',#25609,#17484,#17485);
#15920=AXIS2_PLACEMENT_3D('',#25657,#17487,#17488);
#15921=AXIS2_PLACEMENT_3D('',#25708,#17490,#17491);
#15922=AXIS2_PLACEMENT_3D('',#25727,#17493,#17494);
#15923=AXIS2_PLACEMENT_3D('',#25747,#17495,#17496);
#15924=AXIS2_PLACEMENT_3D('',#25758,#17498,#17499);
#15925=AXIS2_PLACEMENT_3D('',#25765,#17500,#17501);
#15926=AXIS2_PLACEMENT_3D('',#25790,#17503,#17504);
#15927=AXIS2_PLACEMENT_3D('',#25814,#17506,#17507);
#15928=AXIS2_PLACEMENT_3D('',#25839,#17509,#17510);
#15929=AXIS2_PLACEMENT_3D('',#25863,#17512,#17513);
#15930=AXIS2_PLACEMENT_3D('',#25888,#17515,#17516);
#15931=AXIS2_PLACEMENT_3D('',#25913,#17518,#17519);
#15932=AXIS2_PLACEMENT_3D('',#25937,#17521,#17522);
#15933=AXIS2_PLACEMENT_3D('',#25962,#17524,#17525);
#15934=AXIS2_PLACEMENT_3D('',#25986,#17527,#17528);
#15935=AXIS2_PLACEMENT_3D('',#26011,#17530,#17531);
#15936=AXIS2_PLACEMENT_3D('',#26036,#17533,#17534);
#15937=AXIS2_PLACEMENT_3D('',#26060,#17536,#17537);
#15938=AXIS2_PLACEMENT_3D('',#26085,#17539,#17540);
#15939=AXIS2_PLACEMENT_3D('',#26109,#17542,#17543);
#15940=AXIS2_PLACEMENT_3D('',#26134,#17545,#17546);
#15941=AXIS2_PLACEMENT_3D('',#26159,#17548,#17549);
#15942=AXIS2_PLACEMENT_3D('',#26183,#17551,#17552);
#15943=AXIS2_PLACEMENT_3D('',#26194,#17554,#17555);
#15944=AXIS2_PLACEMENT_3D('',#26200,#17556,#17557);
#15945=AXIS2_PLACEMENT_3D('',#26222,#17559,#17560);
#15946=AXIS2_PLACEMENT_3D('',#26225,#17562,#17563);
#15947=AXIS2_PLACEMENT_3D('',#26227,#17564,#17565);
#15948=AXIS2_PLACEMENT_3D('',#26250,#17566,#17567);
#15949=AXIS2_PLACEMENT_3D('',#26298,#17569,#17570);
#15950=AXIS2_PLACEMENT_3D('',#26346,#17572,#17573);
#15951=AXIS2_PLACEMENT_3D('',#26397,#17575,#17576);
#15952=AXIS2_PLACEMENT_3D('',#26448,#17578,#17579);
#15953=AXIS2_PLACEMENT_3D('',#26496,#17581,#17582);
#15954=AXIS2_PLACEMENT_3D('',#26547,#17584,#17585);
#15955=AXIS2_PLACEMENT_3D('',#26598,#17587,#17588);
#15956=AXIS2_PLACEMENT_3D('',#26646,#17590,#17591);
#15957=AXIS2_PLACEMENT_3D('',#26694,#17593,#17594);
#15958=AXIS2_PLACEMENT_3D('',#26748,#17596,#17597);
#15959=AXIS2_PLACEMENT_3D('',#26796,#17599,#17600);
#15960=AXIS2_PLACEMENT_3D('',#26844,#17602,#17603);
#15961=AXIS2_PLACEMENT_3D('',#26895,#17605,#17606);
#15962=AXIS2_PLACEMENT_3D('',#26946,#17608,#17609);
#15963=AXIS2_PLACEMENT_3D('',#26994,#17611,#17612);
#15964=AXIS2_PLACEMENT_3D('',#27045,#17614,#17615);
#15965=AXIS2_PLACEMENT_3D('',#27064,#17617,#17618);
#15966=AXIS2_PLACEMENT_3D('',#27084,#17619,#17620);
#15967=AXIS2_PLACEMENT_3D('',#27095,#17622,#17623);
#15968=AXIS2_PLACEMENT_3D('',#27102,#17624,#17625);
#15969=AXIS2_PLACEMENT_3D('',#27127,#17627,#17628);
#15970=AXIS2_PLACEMENT_3D('',#27151,#17630,#17631);
#15971=AXIS2_PLACEMENT_3D('',#27176,#17633,#17634);
#15972=AXIS2_PLACEMENT_3D('',#27200,#17636,#17637);
#15973=AXIS2_PLACEMENT_3D('',#27225,#17639,#17640);
#15974=AXIS2_PLACEMENT_3D('',#27250,#17642,#17643);
#15975=AXIS2_PLACEMENT_3D('',#27274,#17645,#17646);
#15976=AXIS2_PLACEMENT_3D('',#27299,#17648,#17649);
#15977=AXIS2_PLACEMENT_3D('',#27323,#17651,#17652);
#15978=AXIS2_PLACEMENT_3D('',#27348,#17654,#17655);
#15979=AXIS2_PLACEMENT_3D('',#27373,#17657,#17658);
#15980=AXIS2_PLACEMENT_3D('',#27397,#17660,#17661);
#15981=AXIS2_PLACEMENT_3D('',#27422,#17663,#17664);
#15982=AXIS2_PLACEMENT_3D('',#27446,#17666,#17667);
#15983=AXIS2_PLACEMENT_3D('',#27471,#17669,#17670);
#15984=AXIS2_PLACEMENT_3D('',#27496,#17672,#17673);
#15985=AXIS2_PLACEMENT_3D('',#27520,#17675,#17676);
#15986=AXIS2_PLACEMENT_3D('',#27531,#17678,#17679);
#15987=AXIS2_PLACEMENT_3D('',#27537,#17680,#17681);
#15988=AXIS2_PLACEMENT_3D('',#27559,#17683,#17684);
#15989=AXIS2_PLACEMENT_3D('',#27562,#17686,#17687);
#15990=AXIS2_PLACEMENT_3D('',#27564,#17688,#17689);
#15991=AXIS2_PLACEMENT_3D('',#27587,#17690,#17691);
#15992=AXIS2_PLACEMENT_3D('',#27635,#17693,#17694);
#15993=AXIS2_PLACEMENT_3D('',#27683,#17696,#17697);
#15994=AXIS2_PLACEMENT_3D('',#27734,#17699,#17700);
#15995=AXIS2_PLACEMENT_3D('',#27785,#17702,#17703);
#15996=AXIS2_PLACEMENT_3D('',#27833,#17705,#17706);
#15997=AXIS2_PLACEMENT_3D('',#27884,#17708,#17709);
#15998=AXIS2_PLACEMENT_3D('',#27935,#17711,#17712);
#15999=AXIS2_PLACEMENT_3D('',#27983,#17714,#17715);
#16000=AXIS2_PLACEMENT_3D('',#28031,#17717,#17718);
#16001=AXIS2_PLACEMENT_3D('',#28085,#17720,#17721);
#16002=AXIS2_PLACEMENT_3D('',#28133,#17723,#17724);
#16003=AXIS2_PLACEMENT_3D('',#28181,#17726,#17727);
#16004=AXIS2_PLACEMENT_3D('',#28232,#17729,#17730);
#16005=AXIS2_PLACEMENT_3D('',#28283,#17732,#17733);
#16006=AXIS2_PLACEMENT_3D('',#28331,#17735,#17736);
#16007=AXIS2_PLACEMENT_3D('',#28382,#17738,#17739);
#16008=AXIS2_PLACEMENT_3D('',#28401,#17741,#17742);
#16009=AXIS2_PLACEMENT_3D('',#28421,#17743,#17744);
#16010=AXIS2_PLACEMENT_3D('',#28432,#17746,#17747);
#16011=AXIS2_PLACEMENT_3D('',#28439,#17748,#17749);
#16012=AXIS2_PLACEMENT_3D('',#28464,#17751,#17752);
#16013=AXIS2_PLACEMENT_3D('',#28488,#17754,#17755);
#16014=AXIS2_PLACEMENT_3D('',#28513,#17757,#17758);
#16015=AXIS2_PLACEMENT_3D('',#28537,#17760,#17761);
#16016=AXIS2_PLACEMENT_3D('',#28562,#17763,#17764);
#16017=AXIS2_PLACEMENT_3D('',#28587,#17766,#17767);
#16018=AXIS2_PLACEMENT_3D('',#28611,#17769,#17770);
#16019=AXIS2_PLACEMENT_3D('',#28636,#17772,#17773);
#16020=AXIS2_PLACEMENT_3D('',#28660,#17775,#17776);
#16021=AXIS2_PLACEMENT_3D('',#28685,#17778,#17779);
#16022=AXIS2_PLACEMENT_3D('',#28710,#17781,#17782);
#16023=AXIS2_PLACEMENT_3D('',#28734,#17784,#17785);
#16024=AXIS2_PLACEMENT_3D('',#28759,#17787,#17788);
#16025=AXIS2_PLACEMENT_3D('',#28783,#17790,#17791);
#16026=AXIS2_PLACEMENT_3D('',#28808,#17793,#17794);
#16027=AXIS2_PLACEMENT_3D('',#28833,#17796,#17797);
#16028=AXIS2_PLACEMENT_3D('',#28857,#17799,#17800);
#16029=AXIS2_PLACEMENT_3D('',#28868,#17802,#17803);
#16030=AXIS2_PLACEMENT_3D('',#28874,#17804,#17805);
#16031=AXIS2_PLACEMENT_3D('',#28896,#17807,#17808);
#16032=AXIS2_PLACEMENT_3D('',#28899,#17810,#17811);
#16033=AXIS2_PLACEMENT_3D('',#28901,#17812,#17813);
#16034=AXIS2_PLACEMENT_3D('',#28924,#17814,#17815);
#16035=AXIS2_PLACEMENT_3D('',#28972,#17817,#17818);
#16036=AXIS2_PLACEMENT_3D('',#29020,#17820,#17821);
#16037=AXIS2_PLACEMENT_3D('',#29071,#17823,#17824);
#16038=AXIS2_PLACEMENT_3D('',#29122,#17826,#17827);
#16039=AXIS2_PLACEMENT_3D('',#29170,#17829,#17830);
#16040=AXIS2_PLACEMENT_3D('',#29221,#17832,#17833);
#16041=AXIS2_PLACEMENT_3D('',#29272,#17835,#17836);
#16042=AXIS2_PLACEMENT_3D('',#29320,#17838,#17839);
#16043=AXIS2_PLACEMENT_3D('',#29368,#17841,#17842);
#16044=AXIS2_PLACEMENT_3D('',#29422,#17844,#17845);
#16045=AXIS2_PLACEMENT_3D('',#29470,#17847,#17848);
#16046=AXIS2_PLACEMENT_3D('',#29518,#17850,#17851);
#16047=AXIS2_PLACEMENT_3D('',#29569,#17853,#17854);
#16048=AXIS2_PLACEMENT_3D('',#29620,#17856,#17857);
#16049=AXIS2_PLACEMENT_3D('',#29668,#17859,#17860);
#16050=AXIS2_PLACEMENT_3D('',#29719,#17862,#17863);
#16051=AXIS2_PLACEMENT_3D('',#29738,#17865,#17866);
#16052=AXIS2_PLACEMENT_3D('',#29758,#17867,#17868);
#16053=AXIS2_PLACEMENT_3D('',#29769,#17870,#17871);
#16054=AXIS2_PLACEMENT_3D('',#29776,#17872,#17873);
#16055=AXIS2_PLACEMENT_3D('',#29801,#17875,#17876);
#16056=AXIS2_PLACEMENT_3D('',#29825,#17878,#17879);
#16057=AXIS2_PLACEMENT_3D('',#29850,#17881,#17882);
#16058=AXIS2_PLACEMENT_3D('',#29874,#17884,#17885);
#16059=AXIS2_PLACEMENT_3D('',#29899,#17887,#17888);
#16060=AXIS2_PLACEMENT_3D('',#29924,#17890,#17891);
#16061=AXIS2_PLACEMENT_3D('',#29948,#17893,#17894);
#16062=AXIS2_PLACEMENT_3D('',#29973,#17896,#17897);
#16063=AXIS2_PLACEMENT_3D('',#29997,#17899,#17900);
#16064=AXIS2_PLACEMENT_3D('',#30022,#17902,#17903);
#16065=AXIS2_PLACEMENT_3D('',#30047,#17905,#17906);
#16066=AXIS2_PLACEMENT_3D('',#30071,#17908,#17909);
#16067=AXIS2_PLACEMENT_3D('',#30096,#17911,#17912);
#16068=AXIS2_PLACEMENT_3D('',#30120,#17914,#17915);
#16069=AXIS2_PLACEMENT_3D('',#30145,#17917,#17918);
#16070=AXIS2_PLACEMENT_3D('',#30170,#17920,#17921);
#16071=AXIS2_PLACEMENT_3D('',#30194,#17923,#17924);
#16072=AXIS2_PLACEMENT_3D('',#30205,#17926,#17927);
#16073=AXIS2_PLACEMENT_3D('',#30211,#17928,#17929);
#16074=AXIS2_PLACEMENT_3D('',#30233,#17931,#17932);
#16075=AXIS2_PLACEMENT_3D('',#30236,#17934,#17935);
#16076=AXIS2_PLACEMENT_3D('',#30238,#17936,#17937);
#16077=AXIS2_PLACEMENT_3D('',#30261,#17938,#17939);
#16078=AXIS2_PLACEMENT_3D('',#30309,#17941,#17942);
#16079=AXIS2_PLACEMENT_3D('',#30357,#17944,#17945);
#16080=AXIS2_PLACEMENT_3D('',#30408,#17947,#17948);
#16081=AXIS2_PLACEMENT_3D('',#30459,#17950,#17951);
#16082=AXIS2_PLACEMENT_3D('',#30507,#17953,#17954);
#16083=AXIS2_PLACEMENT_3D('',#30558,#17956,#17957);
#16084=AXIS2_PLACEMENT_3D('',#30609,#17959,#17960);
#16085=AXIS2_PLACEMENT_3D('',#30657,#17962,#17963);
#16086=AXIS2_PLACEMENT_3D('',#30705,#17965,#17966);
#16087=AXIS2_PLACEMENT_3D('',#30759,#17968,#17969);
#16088=AXIS2_PLACEMENT_3D('',#30807,#17971,#17972);
#16089=AXIS2_PLACEMENT_3D('',#30855,#17974,#17975);
#16090=AXIS2_PLACEMENT_3D('',#30906,#17977,#17978);
#16091=AXIS2_PLACEMENT_3D('',#30957,#17980,#17981);
#16092=AXIS2_PLACEMENT_3D('',#31005,#17983,#17984);
#16093=AXIS2_PLACEMENT_3D('',#31056,#17986,#17987);
#16094=AXIS2_PLACEMENT_3D('',#31075,#17989,#17990);
#16095=AXIS2_PLACEMENT_3D('',#31095,#17991,#17992);
#16096=AXIS2_PLACEMENT_3D('',#31106,#17994,#17995);
#16097=AXIS2_PLACEMENT_3D('',#31113,#17996,#17997);
#16098=AXIS2_PLACEMENT_3D('',#31138,#17999,#18000);
#16099=AXIS2_PLACEMENT_3D('',#31162,#18002,#18003);
#16100=AXIS2_PLACEMENT_3D('',#31187,#18005,#18006);
#16101=AXIS2_PLACEMENT_3D('',#31211,#18008,#18009);
#16102=AXIS2_PLACEMENT_3D('',#31236,#18011,#18012);
#16103=AXIS2_PLACEMENT_3D('',#31261,#18014,#18015);
#16104=AXIS2_PLACEMENT_3D('',#31285,#18017,#18018);
#16105=AXIS2_PLACEMENT_3D('',#31310,#18020,#18021);
#16106=AXIS2_PLACEMENT_3D('',#31334,#18023,#18024);
#16107=AXIS2_PLACEMENT_3D('',#31359,#18026,#18027);
#16108=AXIS2_PLACEMENT_3D('',#31384,#18029,#18030);
#16109=AXIS2_PLACEMENT_3D('',#31408,#18032,#18033);
#16110=AXIS2_PLACEMENT_3D('',#31433,#18035,#18036);
#16111=AXIS2_PLACEMENT_3D('',#31457,#18038,#18039);
#16112=AXIS2_PLACEMENT_3D('',#31482,#18041,#18042);
#16113=AXIS2_PLACEMENT_3D('',#31507,#18044,#18045);
#16114=AXIS2_PLACEMENT_3D('',#31531,#18047,#18048);
#16115=AXIS2_PLACEMENT_3D('',#31542,#18050,#18051);
#16116=AXIS2_PLACEMENT_3D('',#31548,#18052,#18053);
#16117=AXIS2_PLACEMENT_3D('',#31722,#18054,#18055);
#16118=AXIS2_PLACEMENT_3D('',#32934,#18056,#18057);
#16119=AXIS2_PLACEMENT_3D('',#32935,#18058,#18059);
#16120=AXIS2_PLACEMENT_3D('',#33109,#18060,#18061);
#16121=AXIS2_PLACEMENT_3D('',#34321,#18062,#18063);
#16122=AXIS2_PLACEMENT_3D('',#34322,#18064,#18065);
#16123=AXIS2_PLACEMENT_3D('',#34496,#18066,#18067);
#16124=AXIS2_PLACEMENT_3D('',#35708,#18068,#18069);
#16125=AXIS2_PLACEMENT_3D('',#35709,#18070,#18071);
#16126=AXIS2_PLACEMENT_3D('',#35883,#18072,#18073);
#16127=AXIS2_PLACEMENT_3D('',#37095,#18074,#18075);
#16128=AXIS2_PLACEMENT_3D('',#37096,#18076,#18077);
#16129=AXIS2_PLACEMENT_3D('',#37097,#18078,#18079);
#16130=AXIS2_PLACEMENT_3D('',#37098,#18080,#18081);
#16131=AXIS2_PLACEMENT_3D('',#37099,#18082,#18083);
#16132=AXIS2_PLACEMENT_3D('',#37100,#18084,#18085);
#16133=AXIS2_PLACEMENT_3D('',#37274,#18086,#18087);
#16134=AXIS2_PLACEMENT_3D('',#38486,#18088,#18089);
#16135=AXIS2_PLACEMENT_3D('',#38487,#18090,#18091);
#16136=AXIS2_PLACEMENT_3D('',#38661,#18092,#18093);
#16137=AXIS2_PLACEMENT_3D('',#39873,#18094,#18095);
#16138=AXIS2_PLACEMENT_3D('',#39874,#18096,#18097);
#16139=AXIS2_PLACEMENT_3D('',#40048,#18098,#18099);
#16140=AXIS2_PLACEMENT_3D('',#41260,#18100,#18101);
#16141=AXIS2_PLACEMENT_3D('',#41261,#18102,#18103);
#16142=AXIS2_PLACEMENT_3D('',#41435,#18104,#18105);
#16143=AXIS2_PLACEMENT_3D('',#42647,#18106,#18107);
#16144=AXIS2_PLACEMENT_3D('',#42648,#18108,#18109);
#16145=AXIS2_PLACEMENT_3D('',#42649,#18110,#18111);
#16146=AXIS2_PLACEMENT_3D('',#42650,#18112,#18113);
#16147=AXIS2_PLACEMENT_3D('',#42651,#18114,#18115);
#16148=AXIS2_PLACEMENT_3D('',#42652,#18116,#18117);
#16149=AXIS2_PLACEMENT_3D('',#42661,#18122,#18123);
#16150=AXIS2_PLACEMENT_3D('',#42667,#18127,#18128);
#16151=AXIS2_PLACEMENT_3D('',#42673,#18132,#18133);
#16152=AXIS2_PLACEMENT_3D('',#42674,#18134,#18135);
#16153=AXIS2_PLACEMENT_3D('',#42676,#18136,#18137);
#16154=AXIS2_PLACEMENT_3D('',#42677,#18138,#18139);
#16155=AXIS2_PLACEMENT_3D('',#44018,#18140,#18141);
#16156=AXIS2_PLACEMENT_3D('',#44021,#18142,#18143);
#16157=AXIS2_PLACEMENT_3D('',#44027,#18147,#18148);
#16158=AXIS2_PLACEMENT_3D('',#44028,#18149,#18150);
#16159=AXIS2_PLACEMENT_3D('',#44034,#18154,#18155);
#16160=AXIS2_PLACEMENT_3D('',#44040,#18159,#18160);
#16161=AXIS2_PLACEMENT_3D('',#44042,#18162,#18163);
#16162=AXIS2_PLACEMENT_3D('',#44043,#18164,#18165);
#16163=AXIS2_PLACEMENT_3D('',#44044,#18166,#18167);
#16164=AXIS2_PLACEMENT_3D('',#44046,#18168,#18169);
#16165=AXIS2_PLACEMENT_3D('',#44048,#18170,#18171);
#16166=AXIS2_PLACEMENT_3D('',#44049,#18172,#18173);
#16167=AXIS2_PLACEMENT_3D('',#44051,#18174,#18175);
#16168=AXIS2_PLACEMENT_3D('',#44053,#18176,#18177);
#16169=AXIS2_PLACEMENT_3D('',#44054,#18178,#18179);
#16170=AXIS2_PLACEMENT_3D('',#44056,#18181,#18182);
#16171=AXIS2_PLACEMENT_3D('',#44059,#18184,#18185);
#16172=AXIS2_PLACEMENT_3D('',#44060,#18186,#18187);
#16173=AXIS2_PLACEMENT_3D('',#44062,#18188,#18189);
#16174=AXIS2_PLACEMENT_3D('',#44063,#18190,#18191);
#16175=AXIS2_PLACEMENT_3D('',#44065,#18192,#18193);
#16176=AXIS2_PLACEMENT_3D('',#44067,#18194,#18195);
#16177=AXIS2_PLACEMENT_3D('',#44068,#18196,#18197);
#16178=AXIS2_PLACEMENT_3D('',#44070,#18199,#18200);
#16179=AXIS2_PLACEMENT_3D('',#44072,#18202,#18203);
#16180=AXIS2_PLACEMENT_3D('',#44074,#18204,#18205);
#16181=AXIS2_PLACEMENT_3D('',#44076,#18207,#18208);
#16182=AXIS2_PLACEMENT_3D('',#44077,#18209,#18210);
#16183=AXIS2_PLACEMENT_3D('',#44078,#18211,#18212);
#17006=DIRECTION('axis',(0.,0.,1.));
#17007=DIRECTION('refdir',(1.,0.,0.));
#17008=DIRECTION('center_axis',(0.,0.,-1.));
#17009=DIRECTION('ref_axis',(1.,0.,0.));
#17010=DIRECTION('',(0.,0.,-1.));
#17011=DIRECTION('center_axis',(0.,0.,-1.));
#17012=DIRECTION('ref_axis',(1.,0.,0.));
#17013=DIRECTION('center_axis',(0.,0.,-1.));
#17014=DIRECTION('ref_axis',(1.,0.,0.));
#17015=DIRECTION('',(0.,0.,-1.));
#17016=DIRECTION('center_axis',(0.,0.,-1.));
#17017=DIRECTION('ref_axis',(1.,0.,0.));
#17018=DIRECTION('center_axis',(0.,0.,-1.));
#17019=DIRECTION('ref_axis',(1.,0.,0.));
#17020=DIRECTION('',(0.,0.,-1.));
#17021=DIRECTION('center_axis',(0.,0.,-1.));
#17022=DIRECTION('ref_axis',(1.,0.,0.));
#17023=DIRECTION('',(0.,0.,-1.));
#17024=DIRECTION('center_axis',(0.,0.,-1.));
#17025=DIRECTION('ref_axis',(1.,0.,0.));
#17026=DIRECTION('',(0.,0.,-1.));
#17027=DIRECTION('center_axis',(0.,0.,-1.));
#17028=DIRECTION('ref_axis',(1.,0.,0.));
#17029=DIRECTION('',(0.,0.,-1.));
#17030=DIRECTION('center_axis',(0.,0.,-1.));
#17031=DIRECTION('ref_axis',(0.936837928895156,-0.349763770255632,0.));
#17032=DIRECTION('',(0.,0.,-1.));
#17033=DIRECTION('center_axis',(0.,0.,-1.));
#17034=DIRECTION('ref_axis',(1.,0.,0.));
#17035=DIRECTION('center_axis',(0.,0.,-1.));
#17036=DIRECTION('ref_axis',(1.,-3.92491481346641E-15,0.));
#17037=DIRECTION('',(1.22464679914735E-16,-4.95661034150385E-31,-1.));
#17038=DIRECTION('center_axis',(0.,0.,1.));
#17039=DIRECTION('ref_axis',(1.,-3.92491481346641E-15,0.));
#17040=DIRECTION('center_axis',(0.,0.,-1.));
#17041=DIRECTION('ref_axis',(1.,-3.92491481346641E-15,0.));
#17042=DIRECTION('',(1.22464679914735E-16,-4.95661034150385E-31,-1.));
#17043=DIRECTION('center_axis',(0.,0.,-1.));
#17044=DIRECTION('ref_axis',(1.,-3.92491481346641E-15,0.));
#17045=DIRECTION('',(1.22464679914735E-16,-4.95661034150385E-31,-1.));
#17046=DIRECTION('center_axis',(0.,0.,-1.));
#17047=DIRECTION('ref_axis',(1.,-3.92491481346641E-15,0.));
#17048=DIRECTION('',(1.22464679914735E-16,-4.95661034150385E-31,-1.));
#17049=DIRECTION('center_axis',(0.,0.,-1.));
#17050=DIRECTION('ref_axis',(1.,-3.92491481346641E-15,0.));
#17051=DIRECTION('',(1.22464679914735E-16,-4.95661034150385E-31,-1.));
#17052=DIRECTION('center_axis',(0.,0.,-1.));
#17053=DIRECTION('ref_axis',(1.,-3.92491481346641E-15,0.));
#17054=DIRECTION('',(1.22464679914735E-16,-4.95661034150385E-31,-1.));
#17055=DIRECTION('center_axis',(0.,0.,-1.));
#17056=DIRECTION('ref_axis',(-0.608987936736927,-0.793179483414,0.));
#17057=DIRECTION('',(1.22464679914735E-16,-4.95661034150385E-31,-1.));
#17058=DIRECTION('center_axis',(0.,0.,-1.));
#17059=DIRECTION('ref_axis',(1.,-3.92491481346641E-15,0.));
#17060=DIRECTION('center_axis',(0.,0.,1.));
#17061=DIRECTION('ref_axis',(-1.,0.,0.));
#17062=DIRECTION('',(0.,0.,1.));
#17063=DIRECTION('center_axis',(0.,0.,-1.));
#17064=DIRECTION('ref_axis',(-1.,0.,0.));
#17065=DIRECTION('',(0.,0.,1.));
#17066=DIRECTION('center_axis',(0.,0.,-1.));
#17067=DIRECTION('ref_axis',(-1.,0.,0.));
#17068=DIRECTION('center_axis',(0.,0.,-1.));
#17069=DIRECTION('ref_axis',(-1.,0.,0.));
#17070=DIRECTION('center_axis',(0.,0.,1.));
#17071=DIRECTION('ref_axis',(-1.,0.,0.));
#17072=DIRECTION('',(0.,0.,1.));
#17073=DIRECTION('center_axis',(0.,0.,1.));
#17074=DIRECTION('ref_axis',(-1.,0.,0.));
#17075=DIRECTION('',(0.,0.,1.));
#17076=DIRECTION('center_axis',(0.,0.,1.));
#17077=DIRECTION('ref_axis',(-1.,0.,0.));
#17078=DIRECTION('',(0.,0.,1.));
#17079=DIRECTION('center_axis',(0.,0.,1.));
#17080=DIRECTION('ref_axis',(-1.,0.,0.));
#17081=DIRECTION('',(0.,0.,1.));
#17082=DIRECTION('center_axis',(0.,0.,1.));
#17083=DIRECTION('ref_axis',(-1.,0.,0.));
#17084=DIRECTION('',(0.,0.,1.));
#17085=DIRECTION('center_axis',(0.,0.,1.));
#17086=DIRECTION('ref_axis',(-1.,0.,0.));
#17087=DIRECTION('',(0.,0.,1.));
#17088=DIRECTION('center_axis',(0.,0.,1.));
#17089=DIRECTION('ref_axis',(-1.,0.,0.));
#17090=DIRECTION('',(0.,0.,1.));
#17091=DIRECTION('center_axis',(0.,0.,1.));
#17092=DIRECTION('ref_axis',(-1.,0.,0.));
#17093=DIRECTION('',(0.,0.,1.));
#17094=DIRECTION('center_axis',(0.,0.,1.));
#17095=DIRECTION('ref_axis',(-1.,0.,0.));
#17096=DIRECTION('',(0.,0.,1.));
#17097=DIRECTION('center_axis',(0.,0.,1.));
#17098=DIRECTION('ref_axis',(-1.,0.,0.));
#17099=DIRECTION('',(0.,0.,1.));
#17100=DIRECTION('center_axis',(0.,0.,1.));
#17101=DIRECTION('ref_axis',(-1.,0.,0.));
#17102=DIRECTION('',(0.,0.,1.));
#17103=DIRECTION('center_axis',(0.,0.,1.));
#17104=DIRECTION('ref_axis',(-1.,0.,0.));
#17105=DIRECTION('',(0.,0.,1.));
#17106=DIRECTION('center_axis',(0.,0.,1.));
#17107=DIRECTION('ref_axis',(-1.,0.,0.));
#17108=DIRECTION('',(0.,0.,1.));
#17109=DIRECTION('center_axis',(0.,0.,1.));
#17110=DIRECTION('ref_axis',(-1.,0.,0.));
#17111=DIRECTION('',(0.,0.,1.));
#17112=DIRECTION('center_axis',(0.,0.,1.));
#17113=DIRECTION('ref_axis',(-1.,0.,0.));
#17114=DIRECTION('',(0.,0.,1.));
#17115=DIRECTION('center_axis',(0.,0.,1.));
#17116=DIRECTION('ref_axis',(-1.,0.,0.));
#17117=DIRECTION('',(0.,0.,1.));
#17118=DIRECTION('center_axis',(0.,0.,1.));
#17119=DIRECTION('ref_axis',(-0.938438080411676,-0.34544749128232,0.));
#17120=DIRECTION('',(0.,0.,1.));
#17121=DIRECTION('center_axis',(0.,0.,-1.));
#17122=DIRECTION('ref_axis',(-1.,0.,0.));
#17123=DIRECTION('center_axis',(0.,0.,1.));
#17124=DIRECTION('ref_axis',(0.417702001320551,0.908584084217199,0.));
#17125=DIRECTION('',(-1.22464679914735E-16,-1.24549850322111E-29,1.));
#17126=DIRECTION('center_axis',(0.,0.,-1.));
#17127=DIRECTION('ref_axis',(-1.,-1.01580206170838E-13,0.));
#17128=DIRECTION('center_axis',(0.,0.,1.));
#17129=DIRECTION('ref_axis',(-1.,-1.01580206170838E-13,0.));
#17130=DIRECTION('',(-1.22464679914735E-16,-1.24549850322111E-29,1.));
#17131=DIRECTION('center_axis',(0.,0.,1.));
#17132=DIRECTION('ref_axis',(-1.,-1.01580206170838E-13,0.));
#17133=DIRECTION('',(-1.22464679914735E-16,-1.24549850322111E-29,1.));
#17134=DIRECTION('center_axis',(0.,0.,1.));
#17135=DIRECTION('ref_axis',(-1.,-1.01580206170838E-13,0.));
#17136=DIRECTION('',(-1.22464679914735E-16,-1.24549850322111E-29,1.));
#17137=DIRECTION('center_axis',(0.,0.,1.));
#17138=DIRECTION('ref_axis',(-1.,-1.01580206170838E-13,0.));
#17139=DIRECTION('',(-1.22464679914735E-16,-1.24549850322111E-29,1.));
#17140=DIRECTION('center_axis',(0.,0.,1.));
#17141=DIRECTION('ref_axis',(-1.,-1.01580206170838E-13,0.));
#17142=DIRECTION('',(-1.22464679914735E-16,-1.24549850322111E-29,1.));
#17143=DIRECTION('center_axis',(0.,0.,1.));
#17144=DIRECTION('ref_axis',(-1.,-1.01580206170838E-13,0.));
#17145=DIRECTION('',(-1.22464679914735E-16,-1.24549850322111E-29,1.));
#17146=DIRECTION('center_axis',(0.,0.,1.));
#17147=DIRECTION('ref_axis',(-1.,-1.01580206170838E-13,0.));
#17148=DIRECTION('',(-1.22464679914735E-16,-1.24549850322111E-29,1.));
#17149=DIRECTION('center_axis',(0.,0.,1.));
#17150=DIRECTION('ref_axis',(-1.,-1.01580206170838E-13,0.));
#17151=DIRECTION('',(-1.22464679914735E-16,-1.24549850322111E-29,1.));
#17152=DIRECTION('center_axis',(0.,0.,1.));
#17153=DIRECTION('ref_axis',(-1.,-1.01580206170838E-13,0.));
#17154=DIRECTION('',(-1.22464679914735E-16,-1.24549850322111E-29,1.));
#17155=DIRECTION('center_axis',(0.,0.,1.));
#17156=DIRECTION('ref_axis',(-1.,-1.01580206170838E-13,0.));
#17157=DIRECTION('',(-1.22464679914735E-16,-1.24549850322111E-29,1.));
#17158=DIRECTION('center_axis',(0.,0.,1.));
#17159=DIRECTION('ref_axis',(-1.,-1.01580206170838E-13,0.));
#17160=DIRECTION('',(-1.22464679914735E-16,-1.24549850322111E-29,1.));
#17161=DIRECTION('center_axis',(0.,0.,1.));
#17162=DIRECTION('ref_axis',(-1.,-1.01580206170838E-13,0.));
#17163=DIRECTION('',(-1.22464679914735E-16,-1.24549850322111E-29,1.));
#17164=DIRECTION('center_axis',(0.,0.,1.));
#17165=DIRECTION('ref_axis',(-1.,-1.01580206170838E-13,0.));
#17166=DIRECTION('',(-1.22464679914735E-16,-1.24549850322111E-29,1.));
#17167=DIRECTION('center_axis',(0.,0.,1.));
#17168=DIRECTION('ref_axis',(-1.,-1.01580206170838E-13,0.));
#17169=DIRECTION('',(-1.22464679914735E-16,-1.24549850322111E-29,1.));
#17170=DIRECTION('center_axis',(0.,0.,1.));
#17171=DIRECTION('ref_axis',(-1.,-1.01580206170838E-13,0.));
#17172=DIRECTION('',(-1.22464679914735E-16,-1.24549850322111E-29,1.));
#17173=DIRECTION('center_axis',(0.,0.,1.));
#17174=DIRECTION('ref_axis',(-1.,-1.01580206170838E-13,0.));
#17175=DIRECTION('',(-1.22464679914735E-16,-1.24549850322111E-29,1.));
#17176=DIRECTION('center_axis',(0.,0.,1.));
#17177=DIRECTION('ref_axis',(-1.,-1.01580206170838E-13,0.));
#17178=DIRECTION('',(-1.22464679914735E-16,-1.24549850322111E-29,1.));
#17179=DIRECTION('center_axis',(0.,0.,1.));
#17180=DIRECTION('ref_axis',(0.609342743503397,-0.792906943430157,0.));
#17181=DIRECTION('',(-1.22464679914735E-16,-1.24549850322111E-29,1.));
#17182=DIRECTION('center_axis',(0.,0.,1.));
#17183=DIRECTION('ref_axis',(-1.,-1.01580206170838E-13,0.));
#17184=DIRECTION('center_axis',(0.,0.,1.));
#17185=DIRECTION('ref_axis',(-1.,0.,0.));
#17186=DIRECTION('',(0.,0.,1.));
#17187=DIRECTION('center_axis',(0.,0.,-1.));
#17188=DIRECTION('ref_axis',(-1.,0.,0.));
#17189=DIRECTION('',(0.,0.,1.));
#17190=DIRECTION('center_axis',(0.,0.,-1.));
#17191=DIRECTION('ref_axis',(-1.,0.,0.));
#17192=DIRECTION('center_axis',(0.,0.,-1.));
#17193=DIRECTION('ref_axis',(-1.,0.,0.));
#17194=DIRECTION('center_axis',(0.,0.,1.));
#17195=DIRECTION('ref_axis',(-1.,0.,0.));
#17196=DIRECTION('',(0.,0.,1.));
#17197=DIRECTION('center_axis',(0.,0.,1.));
#17198=DIRECTION('ref_axis',(-1.,0.,0.));
#17199=DIRECTION('',(0.,0.,1.));
#17200=DIRECTION('center_axis',(0.,0.,1.));
#17201=DIRECTION('ref_axis',(-1.,0.,0.));
#17202=DIRECTION('',(0.,0.,1.));
#17203=DIRECTION('center_axis',(0.,0.,1.));
#17204=DIRECTION('ref_axis',(-1.,0.,0.));
#17205=DIRECTION('',(0.,0.,1.));
#17206=DIRECTION('center_axis',(0.,0.,1.));
#17207=DIRECTION('ref_axis',(-1.,0.,0.));
#17208=DIRECTION('',(0.,0.,1.));
#17209=DIRECTION('center_axis',(0.,0.,1.));
#17210=DIRECTION('ref_axis',(-1.,0.,0.));
#17211=DIRECTION('',(0.,0.,1.));
#17212=DIRECTION('center_axis',(0.,0.,1.));
#17213=DIRECTION('ref_axis',(-1.,0.,0.));
#17214=DIRECTION('',(0.,0.,1.));
#17215=DIRECTION('center_axis',(0.,0.,1.));
#17216=DIRECTION('ref_axis',(-1.,0.,0.));
#17217=DIRECTION('',(0.,0.,1.));
#17218=DIRECTION('center_axis',(0.,0.,1.));
#17219=DIRECTION('ref_axis',(-1.,0.,0.));
#17220=DIRECTION('',(0.,0.,1.));
#17221=DIRECTION('center_axis',(0.,0.,1.));
#17222=DIRECTION('ref_axis',(-1.,0.,0.));
#17223=DIRECTION('',(0.,0.,1.));
#17224=DIRECTION('center_axis',(0.,0.,1.));
#17225=DIRECTION('ref_axis',(-1.,0.,0.));
#17226=DIRECTION('',(0.,0.,1.));
#17227=DIRECTION('center_axis',(0.,0.,1.));
#17228=DIRECTION('ref_axis',(-1.,0.,0.));
#17229=DIRECTION('',(0.,0.,1.));
#17230=DIRECTION('center_axis',(0.,0.,1.));
#17231=DIRECTION('ref_axis',(-1.,0.,0.));
#17232=DIRECTION('',(0.,0.,1.));
#17233=DIRECTION('center_axis',(0.,0.,1.));
#17234=DIRECTION('ref_axis',(-1.,0.,0.));
#17235=DIRECTION('',(0.,0.,1.));
#17236=DIRECTION('center_axis',(0.,0.,1.));
#17237=DIRECTION('ref_axis',(-1.,0.,0.));
#17238=DIRECTION('',(0.,0.,1.));
#17239=DIRECTION('center_axis',(0.,0.,1.));
#17240=DIRECTION('ref_axis',(-1.,0.,0.));
#17241=DIRECTION('',(0.,0.,1.));
#17242=DIRECTION('center_axis',(0.,0.,1.));
#17243=DIRECTION('ref_axis',(-0.938438085006596,-0.345447478799822,0.));
#17244=DIRECTION('',(0.,0.,1.));
#17245=DIRECTION('center_axis',(0.,0.,-1.));
#17246=DIRECTION('ref_axis',(-1.,0.,0.));
#17247=DIRECTION('center_axis',(0.,0.,1.));
#17248=DIRECTION('ref_axis',(0.417701990298203,0.908584089284487,0.));
#17249=DIRECTION('',(-1.22464679914735E-16,-1.29843461996317E-29,1.));
#17250=DIRECTION('center_axis',(0.,0.,-1.));
#17251=DIRECTION('ref_axis',(-1.,-1.05902768135554E-13,0.));
#17252=DIRECTION('center_axis',(0.,0.,1.));
#17253=DIRECTION('ref_axis',(-1.,-1.05902768135554E-13,0.));
#17254=DIRECTION('',(-1.22464679914735E-16,-1.29843461996317E-29,1.));
#17255=DIRECTION('center_axis',(0.,0.,1.));
#17256=DIRECTION('ref_axis',(-1.,-1.05902768135554E-13,0.));
#17257=DIRECTION('',(-1.22464679914735E-16,-1.29843461996317E-29,1.));
#17258=DIRECTION('center_axis',(0.,0.,1.));
#17259=DIRECTION('ref_axis',(-1.,-1.05902768135554E-13,0.));
#17260=DIRECTION('',(-1.22464679914735E-16,-1.29843461996317E-29,1.));
#17261=DIRECTION('center_axis',(0.,0.,1.));
#17262=DIRECTION('ref_axis',(-1.,-1.05902768135554E-13,0.));
#17263=DIRECTION('',(-1.22464679914735E-16,-1.29843461996317E-29,1.));
#17264=DIRECTION('center_axis',(0.,0.,1.));
#17265=DIRECTION('ref_axis',(-1.,-1.05902768135554E-13,0.));
#17266=DIRECTION('',(-1.22464679914735E-16,-1.29843461996317E-29,1.));
#17267=DIRECTION('center_axis',(0.,0.,1.));
#17268=DIRECTION('ref_axis',(-1.,-1.05902768135554E-13,0.));
#17269=DIRECTION('',(-1.22464679914735E-16,-1.29843461996317E-29,1.));
#17270=DIRECTION('center_axis',(0.,0.,1.));
#17271=DIRECTION('ref_axis',(-1.,-1.05902768135554E-13,0.));
#17272=DIRECTION('',(-1.22464679914735E-16,-1.29843461996317E-29,1.));
#17273=DIRECTION('center_axis',(0.,0.,1.));
#17274=DIRECTION('ref_axis',(-1.,-1.05902768135554E-13,0.));
#17275=DIRECTION('',(-1.22464679914735E-16,-1.29843461996317E-29,1.));
#17276=DIRECTION('center_axis',(0.,0.,1.));
#17277=DIRECTION('ref_axis',(-1.,-1.05902768135554E-13,0.));
#17278=DIRECTION('',(-1.22464679914735E-16,-1.29843461996317E-29,1.));
#17279=DIRECTION('center_axis',(0.,0.,1.));
#17280=DIRECTION('ref_axis',(-1.,-1.05902768135554E-13,0.));
#17281=DIRECTION('',(-1.22464679914735E-16,-1.29843461996317E-29,1.));
#17282=DIRECTION('center_axis',(0.,0.,1.));
#17283=DIRECTION('ref_axis',(-1.,-1.05902768135554E-13,0.));
#17284=DIRECTION('',(-1.22464679914735E-16,-1.29843461996317E-29,1.));
#17285=DIRECTION('center_axis',(0.,0.,1.));
#17286=DIRECTION('ref_axis',(-1.,-1.05902768135554E-13,0.));
#17287=DIRECTION('',(-1.22464679914735E-16,-1.29843461996317E-29,1.));
#17288=DIRECTION('center_axis',(0.,0.,1.));
#17289=DIRECTION('ref_axis',(-1.,-1.05902768135554E-13,0.));
#17290=DIRECTION('',(-1.22464679914735E-16,-1.29843461996317E-29,1.));
#17291=DIRECTION('center_axis',(0.,0.,1.));
#17292=DIRECTION('ref_axis',(-1.,-1.05902768135554E-13,0.));
#17293=DIRECTION('',(-1.22464679914735E-16,-1.29843461996317E-29,1.));
#17294=DIRECTION('center_axis',(0.,0.,1.));
#17295=DIRECTION('ref_axis',(-1.,-1.05902768135554E-13,0.));
#17296=DIRECTION('',(-1.22464679914735E-16,-1.29843461996317E-29,1.));
#17297=DIRECTION('center_axis',(0.,0.,1.));
#17298=DIRECTION('ref_axis',(-1.,-1.05902768135554E-13,0.));
#17299=DIRECTION('',(-1.22464679914735E-16,-1.29843461996317E-29,1.));
#17300=DIRECTION('center_axis',(0.,0.,1.));
#17301=DIRECTION('ref_axis',(-1.,-1.05902768135554E-13,0.));
#17302=DIRECTION('',(-1.22464679914735E-16,-1.29843461996317E-29,1.));
#17303=DIRECTION('center_axis',(0.,0.,1.));
#17304=DIRECTION('ref_axis',(0.609342733687785,-0.792906950973377,0.));
#17305=DIRECTION('',(-1.22464679914735E-16,-1.29843461996317E-29,1.));
#17306=DIRECTION('center_axis',(0.,0.,1.));
#17307=DIRECTION('ref_axis',(-1.,-1.05902768135554E-13,0.));
#17308=DIRECTION('center_axis',(0.,0.,1.));
#17309=DIRECTION('ref_axis',(-1.,0.,0.));
#17310=DIRECTION('',(0.,0.,1.));
#17311=DIRECTION('center_axis',(0.,0.,-1.));
#17312=DIRECTION('ref_axis',(-1.,0.,0.));
#17313=DIRECTION('',(0.,0.,1.));
#17314=DIRECTION('center_axis',(0.,0.,-1.));
#17315=DIRECTION('ref_axis',(-1.,0.,0.));
#17316=DIRECTION('center_axis',(0.,0.,-1.));
#17317=DIRECTION('ref_axis',(-1.,0.,0.));
#17318=DIRECTION('center_axis',(0.,0.,1.));
#17319=DIRECTION('ref_axis',(-1.,0.,0.));
#17320=DIRECTION('',(0.,0.,1.));
#17321=DIRECTION('center_axis',(0.,0.,1.));
#17322=DIRECTION('ref_axis',(-1.,0.,0.));
#17323=DIRECTION('',(0.,0.,1.));
#17324=DIRECTION('center_axis',(0.,0.,1.));
#17325=DIRECTION('ref_axis',(-1.,0.,0.));
#17326=DIRECTION('',(0.,0.,1.));
#17327=DIRECTION('center_axis',(0.,0.,1.));
#17328=DIRECTION('ref_axis',(-1.,0.,0.));
#17329=DIRECTION('',(0.,0.,1.));
#17330=DIRECTION('center_axis',(0.,0.,1.));
#17331=DIRECTION('ref_axis',(-1.,0.,0.));
#17332=DIRECTION('',(0.,0.,1.));
#17333=DIRECTION('center_axis',(0.,0.,1.));
#17334=DIRECTION('ref_axis',(-1.,0.,0.));
#17335=DIRECTION('',(0.,0.,1.));
#17336=DIRECTION('center_axis',(0.,0.,1.));
#17337=DIRECTION('ref_axis',(-1.,0.,0.));
#17338=DIRECTION('',(0.,0.,1.));
#17339=DIRECTION('center_axis',(0.,0.,1.));
#17340=DIRECTION('ref_axis',(-1.,0.,0.));
#17341=DIRECTION('',(0.,0.,1.));
#17342=DIRECTION('center_axis',(0.,0.,1.));
#17343=DIRECTION('ref_axis',(-1.,0.,0.));
#17344=DIRECTION('',(0.,0.,1.));
#17345=DIRECTION('center_axis',(0.,0.,1.));
#17346=DIRECTION('ref_axis',(-1.,0.,0.));
#17347=DIRECTION('',(0.,0.,1.));
#17348=DIRECTION('center_axis',(0.,0.,1.));
#17349=DIRECTION('ref_axis',(-1.,0.,0.));
#17350=DIRECTION('',(0.,0.,1.));
#17351=DIRECTION('center_axis',(0.,0.,1.));
#17352=DIRECTION('ref_axis',(-1.,0.,0.));
#17353=DIRECTION('',(0.,0.,1.));
#17354=DIRECTION('center_axis',(0.,0.,1.));
#17355=DIRECTION('ref_axis',(-1.,0.,0.));
#17356=DIRECTION('',(0.,0.,1.));
#17357=DIRECTION('center_axis',(0.,0.,1.));
#17358=DIRECTION('ref_axis',(-1.,0.,0.));
#17359=DIRECTION('',(0.,0.,1.));
#17360=DIRECTION('center_axis',(0.,0.,1.));
#17361=DIRECTION('ref_axis',(-1.,0.,0.));
#17362=DIRECTION('',(0.,0.,1.));
#17363=DIRECTION('center_axis',(0.,0.,1.));
#17364=DIRECTION('ref_axis',(-1.,0.,0.));
#17365=DIRECTION('',(0.,0.,1.));
#17366=DIRECTION('center_axis',(0.,0.,1.));
#17367=DIRECTION('ref_axis',(-0.938438094004156,-0.345447454357167,0.));
#17368=DIRECTION('',(0.,0.,1.));
#17369=DIRECTION('center_axis',(0.,0.,-1.));
#17370=DIRECTION('ref_axis',(-1.,0.,0.));
#17371=DIRECTION('center_axis',(0.,0.,1.));
#17372=DIRECTION('ref_axis',(0.417701964204128,0.908584101280676,0.));
#17373=DIRECTION('',(-1.22464679914735E-16,-1.29843461996317E-29,1.));
#17374=DIRECTION('center_axis',(0.,0.,-1.));
#17375=DIRECTION('ref_axis',(-1.,-1.05902768135554E-13,0.));
#17376=DIRECTION('center_axis',(0.,0.,1.));
#17377=DIRECTION('ref_axis',(-1.,-1.05902768135554E-13,0.));
#17378=DIRECTION('',(-1.22464679914735E-16,-1.29843461996317E-29,1.));
#17379=DIRECTION('center_axis',(0.,0.,1.));
#17380=DIRECTION('ref_axis',(-1.,-1.05902768135554E-13,0.));
#17381=DIRECTION('',(-1.22464679914735E-16,-1.29843461996317E-29,1.));
#17382=DIRECTION('center_axis',(0.,0.,1.));
#17383=DIRECTION('ref_axis',(-1.,-1.05902768135554E-13,0.));
#17384=DIRECTION('',(-1.22464679914735E-16,-1.29843461996317E-29,1.));
#17385=DIRECTION('center_axis',(0.,0.,1.));
#17386=DIRECTION('ref_axis',(-1.,-1.05902768135554E-13,0.));
#17387=DIRECTION('',(-1.22464679914735E-16,-1.29843461996317E-29,1.));
#17388=DIRECTION('center_axis',(0.,0.,1.));
#17389=DIRECTION('ref_axis',(-1.,-1.05902768135554E-13,0.));
#17390=DIRECTION('',(-1.22464679914735E-16,-1.29843461996317E-29,1.));
#17391=DIRECTION('center_axis',(0.,0.,1.));
#17392=DIRECTION('ref_axis',(-1.,-1.05902768135554E-13,0.));
#17393=DIRECTION('',(-1.22464679914735E-16,-1.29843461996317E-29,1.));
#17394=DIRECTION('center_axis',(0.,0.,1.));
#17395=DIRECTION('ref_axis',(-1.,-1.05902768135554E-13,0.));
#17396=DIRECTION('',(-1.22464679914735E-16,-1.29843461996317E-29,1.));
#17397=DIRECTION('center_axis',(0.,0.,1.));
#17398=DIRECTION('ref_axis',(-1.,-1.05902768135554E-13,0.));
#17399=DIRECTION('',(-1.22464679914735E-16,-1.29843461996317E-29,1.));
#17400=DIRECTION('center_axis',(0.,0.,1.));
#17401=DIRECTION('ref_axis',(-1.,-1.05902768135554E-13,0.));
#17402=DIRECTION('',(-1.22464679914735E-16,-1.29843461996317E-29,1.));
#17403=DIRECTION('center_axis',(0.,0.,1.));
#17404=DIRECTION('ref_axis',(-1.,-1.05902768135554E-13,0.));
#17405=DIRECTION('',(-1.22464679914735E-16,-1.29843461996317E-29,1.));
#17406=DIRECTION('center_axis',(0.,0.,1.));
#17407=DIRECTION('ref_axis',(-1.,-1.05902768135554E-13,0.));
#17408=DIRECTION('',(-1.22464679914735E-16,-1.29843461996317E-29,1.));
#17409=DIRECTION('center_axis',(0.,0.,1.));
#17410=DIRECTION('ref_axis',(-1.,-1.05902768135554E-13,0.));
#17411=DIRECTION('',(-1.22464679914735E-16,-1.29843461996317E-29,1.));
#17412=DIRECTION('center_axis',(0.,0.,1.));
#17413=DIRECTION('ref_axis',(-1.,-1.05902768135554E-13,0.));
#17414=DIRECTION('',(-1.22464679914735E-16,-1.29843461996317E-29,1.));
#17415=DIRECTION('center_axis',(0.,0.,1.));
#17416=DIRECTION('ref_axis',(-1.,-1.05902768135554E-13,0.));
#17417=DIRECTION('',(-1.22464679914735E-16,-1.29843461996317E-29,1.));
#17418=DIRECTION('center_axis',(0.,0.,1.));
#17419=DIRECTION('ref_axis',(-1.,-1.05902768135554E-13,0.));
#17420=DIRECTION('',(-1.22464679914735E-16,-1.29843461996317E-29,1.));
#17421=DIRECTION('center_axis',(0.,0.,1.));
#17422=DIRECTION('ref_axis',(-1.,-1.05902768135554E-13,0.));
#17423=DIRECTION('',(-1.22464679914735E-16,-1.29843461996317E-29,1.));
#17424=DIRECTION('center_axis',(0.,0.,1.));
#17425=DIRECTION('ref_axis',(-1.,-1.05902768135554E-13,0.));
#17426=DIRECTION('',(-1.22464679914735E-16,-1.29843461996317E-29,1.));
#17427=DIRECTION('center_axis',(0.,0.,1.));
#17428=DIRECTION('ref_axis',(0.609342756385647,-0.792906933530248,0.));
#17429=DIRECTION('',(-1.22464679914735E-16,-1.29843461996317E-29,1.));
#17430=DIRECTION('center_axis',(0.,0.,1.));
#17431=DIRECTION('ref_axis',(-1.,-1.05902768135554E-13,0.));
#17432=DIRECTION('center_axis',(0.,0.,1.));
#17433=DIRECTION('ref_axis',(-1.,0.,0.));
#17434=DIRECTION('',(0.,0.,1.));
#17435=DIRECTION('center_axis',(0.,0.,-1.));
#17436=DIRECTION('ref_axis',(-1.,0.,0.));
#17437=DIRECTION('',(0.,0.,1.));
#17438=DIRECTION('center_axis',(0.,0.,-1.));
#17439=DIRECTION('ref_axis',(-1.,0.,0.));
#17440=DIRECTION('center_axis',(0.,0.,-1.));
#17441=DIRECTION('ref_axis',(-1.,0.,0.));
#17442=DIRECTION('center_axis',(0.,0.,1.));
#17443=DIRECTION('ref_axis',(-1.,0.,0.));
#17444=DIRECTION('',(0.,0.,1.));
#17445=DIRECTION('center_axis',(0.,0.,1.));
#17446=DIRECTION('ref_axis',(-1.,0.,0.));
#17447=DIRECTION('',(0.,0.,1.));
#17448=DIRECTION('center_axis',(0.,0.,1.));
#17449=DIRECTION('ref_axis',(-1.,0.,0.));
#17450=DIRECTION('',(0.,0.,1.));
#17451=DIRECTION('center_axis',(0.,0.,1.));
#17452=DIRECTION('ref_axis',(-1.,0.,0.));
#17453=DIRECTION('',(0.,0.,1.));
#17454=DIRECTION('center_axis',(0.,0.,1.));
#17455=DIRECTION('ref_axis',(-1.,0.,0.));
#17456=DIRECTION('',(0.,0.,1.));
#17457=DIRECTION('center_axis',(0.,0.,1.));
#17458=DIRECTION('ref_axis',(-1.,0.,0.));
#17459=DIRECTION('',(0.,0.,1.));
#17460=DIRECTION('center_axis',(0.,0.,1.));
#17461=DIRECTION('ref_axis',(-1.,0.,0.));
#17462=DIRECTION('',(0.,0.,1.));
#17463=DIRECTION('center_axis',(0.,0.,1.));
#17464=DIRECTION('ref_axis',(-1.,0.,0.));
#17465=DIRECTION('',(0.,0.,1.));
#17466=DIRECTION('center_axis',(0.,0.,1.));
#17467=DIRECTION('ref_axis',(-1.,0.,0.));
#17468=DIRECTION('',(0.,0.,1.));
#17469=DIRECTION('center_axis',(0.,0.,1.));
#17470=DIRECTION('ref_axis',(-1.,0.,0.));
#17471=DIRECTION('',(0.,0.,1.));
#17472=DIRECTION('center_axis',(0.,0.,1.));
#17473=DIRECTION('ref_axis',(-1.,0.,0.));
#17474=DIRECTION('',(0.,0.,1.));
#17475=DIRECTION('center_axis',(0.,0.,1.));
#17476=DIRECTION('ref_axis',(-1.,0.,0.));
#17477=DIRECTION('',(0.,0.,1.));
#17478=DIRECTION('center_axis',(0.,0.,1.));
#17479=DIRECTION('ref_axis',(-1.,0.,0.));
#17480=DIRECTION('',(0.,0.,1.));
#17481=DIRECTION('center_axis',(0.,0.,1.));
#17482=DIRECTION('ref_axis',(-1.,0.,0.));
#17483=DIRECTION('',(0.,0.,1.));
#17484=DIRECTION('center_axis',(0.,0.,1.));
#17485=DIRECTION('ref_axis',(-1.,0.,0.));
#17486=DIRECTION('',(0.,0.,1.));
#17487=DIRECTION('center_axis',(0.,0.,1.));
#17488=DIRECTION('ref_axis',(-1.,0.,0.));
#17489=DIRECTION('',(0.,0.,1.));
#17490=DIRECTION('center_axis',(0.,0.,1.));
#17491=DIRECTION('ref_axis',(-0.938438098661675,-0.345447441704612,0.));
#17492=DIRECTION('',(0.,0.,1.));
#17493=DIRECTION('center_axis',(0.,0.,-1.));
#17494=DIRECTION('ref_axis',(-1.,0.,0.));
#17495=DIRECTION('center_axis',(0.,0.,1.));
#17496=DIRECTION('ref_axis',(0.417701952176177,0.908584106810267,0.));
#17497=DIRECTION('',(-1.22464679914735E-16,-1.29843461996317E-29,1.));
#17498=DIRECTION('center_axis',(0.,0.,-1.));
#17499=DIRECTION('ref_axis',(-1.,-1.05902768135554E-13,0.));
#17500=DIRECTION('center_axis',(0.,0.,1.));
#17501=DIRECTION('ref_axis',(-1.,-1.05902768135554E-13,0.));
#17502=DIRECTION('',(-1.22464679914735E-16,-1.29843461996317E-29,1.));
#17503=DIRECTION('center_axis',(0.,0.,1.));
#17504=DIRECTION('ref_axis',(-1.,-1.05902768135554E-13,0.));
#17505=DIRECTION('',(-1.22464679914735E-16,-1.29843461996317E-29,1.));
#17506=DIRECTION('center_axis',(0.,0.,1.));
#17507=DIRECTION('ref_axis',(-1.,-1.05902768135554E-13,0.));
#17508=DIRECTION('',(-1.22464679914735E-16,-1.29843461996317E-29,1.));
#17509=DIRECTION('center_axis',(0.,0.,1.));
#17510=DIRECTION('ref_axis',(-1.,-1.05902768135554E-13,0.));
#17511=DIRECTION('',(-1.22464679914735E-16,-1.29843461996317E-29,1.));
#17512=DIRECTION('center_axis',(0.,0.,1.));
#17513=DIRECTION('ref_axis',(-1.,-1.05902768135554E-13,0.));
#17514=DIRECTION('',(-1.22464679914735E-16,-1.29843461996317E-29,1.));
#17515=DIRECTION('center_axis',(0.,0.,1.));
#17516=DIRECTION('ref_axis',(-1.,-1.05902768135554E-13,0.));
#17517=DIRECTION('',(-1.22464679914735E-16,-1.29843461996317E-29,1.));
#17518=DIRECTION('center_axis',(0.,0.,1.));
#17519=DIRECTION('ref_axis',(-1.,-1.05902768135554E-13,0.));
#17520=DIRECTION('',(-1.22464679914735E-16,-1.29843461996317E-29,1.));
#17521=DIRECTION('center_axis',(0.,0.,1.));
#17522=DIRECTION('ref_axis',(-1.,-1.05902768135554E-13,0.));
#17523=DIRECTION('',(-1.22464679914735E-16,-1.29843461996317E-29,1.));
#17524=DIRECTION('center_axis',(0.,0.,1.));
#17525=DIRECTION('ref_axis',(-1.,-1.05902768135554E-13,0.));
#17526=DIRECTION('',(-1.22464679914735E-16,-1.29843461996317E-29,1.));
#17527=DIRECTION('center_axis',(0.,0.,1.));
#17528=DIRECTION('ref_axis',(-1.,-1.05902768135554E-13,0.));
#17529=DIRECTION('',(-1.22464679914735E-16,-1.29843461996317E-29,1.));
#17530=DIRECTION('center_axis',(0.,0.,1.));
#17531=DIRECTION('ref_axis',(-1.,-1.05902768135554E-13,0.));
#17532=DIRECTION('',(-1.22464679914735E-16,-1.29843461996317E-29,1.));
#17533=DIRECTION('center_axis',(0.,0.,1.));
#17534=DIRECTION('ref_axis',(-1.,-1.05902768135554E-13,0.));
#17535=DIRECTION('',(-1.22464679914735E-16,-1.29843461996317E-29,1.));
#17536=DIRECTION('center_axis',(0.,0.,1.));
#17537=DIRECTION('ref_axis',(-1.,-1.05902768135554E-13,0.));
#17538=DIRECTION('',(-1.22464679914735E-16,-1.29843461996317E-29,1.));
#17539=DIRECTION('center_axis',(0.,0.,1.));
#17540=DIRECTION('ref_axis',(-1.,-1.05902768135554E-13,0.));
#17541=DIRECTION('',(-1.22464679914735E-16,-1.29843461996317E-29,1.));
#17542=DIRECTION('center_axis',(0.,0.,1.));
#17543=DIRECTION('ref_axis',(-1.,-1.05902768135554E-13,0.));
#17544=DIRECTION('',(-1.22464679914735E-16,-1.29843461996317E-29,1.));
#17545=DIRECTION('center_axis',(0.,0.,1.));
#17546=DIRECTION('ref_axis',(-1.,-1.05902768135554E-13,0.));
#17547=DIRECTION('',(-1.22464679914735E-16,-1.29843461996317E-29,1.));
#17548=DIRECTION('center_axis',(0.,0.,1.));
#17549=DIRECTION('ref_axis',(-1.,-1.05902768135554E-13,0.));
#17550=DIRECTION('',(-1.22464679914735E-16,-1.29843461996317E-29,1.));
#17551=DIRECTION('center_axis',(0.,0.,1.));
#17552=DIRECTION('ref_axis',(0.609342754269626,-0.792906935156394,0.));
#17553=DIRECTION('',(-1.22464679914735E-16,-1.29843461996317E-29,1.));
#17554=DIRECTION('center_axis',(0.,0.,1.));
#17555=DIRECTION('ref_axis',(-1.,-1.05902768135554E-13,0.));
#17556=DIRECTION('center_axis',(0.,0.,-1.));
#17557=DIRECTION('ref_axis',(1.,0.,0.));
#17558=DIRECTION('',(0.,0.,-1.));
#17559=DIRECTION('center_axis',(0.,0.,1.));
#17560=DIRECTION('ref_axis',(1.,0.,0.));
#17561=DIRECTION('',(0.,0.,-1.));
#17562=DIRECTION('center_axis',(0.,0.,1.));
#17563=DIRECTION('ref_axis',(1.,0.,0.));
#17564=DIRECTION('center_axis',(0.,0.,1.));
#17565=DIRECTION('ref_axis',(1.,0.,0.));
#17566=DIRECTION('center_axis',(0.,0.,-1.));
#17567=DIRECTION('ref_axis',(1.,0.,0.));
#17568=DIRECTION('',(0.,0.,-1.));
#17569=DIRECTION('center_axis',(0.,0.,-1.));
#17570=DIRECTION('ref_axis',(1.,0.,0.));
#17571=DIRECTION('',(0.,0.,-1.));
#17572=DIRECTION('center_axis',(0.,0.,-1.));
#17573=DIRECTION('ref_axis',(1.,0.,0.));
#17574=DIRECTION('',(0.,0.,-1.));
#17575=DIRECTION('center_axis',(0.,0.,-1.));
#17576=DIRECTION('ref_axis',(1.,0.,0.));
#17577=DIRECTION('',(0.,0.,-1.));
#17578=DIRECTION('center_axis',(0.,0.,-1.));
#17579=DIRECTION('ref_axis',(1.,0.,0.));
#17580=DIRECTION('',(0.,0.,-1.));
#17581=DIRECTION('center_axis',(0.,0.,-1.));
#17582=DIRECTION('ref_axis',(1.,0.,0.));
#17583=DIRECTION('',(0.,0.,-1.));
#17584=DIRECTION('center_axis',(0.,0.,-1.));
#17585=DIRECTION('ref_axis',(1.,0.,0.));
#17586=DIRECTION('',(0.,0.,-1.));
#17587=DIRECTION('center_axis',(0.,0.,-1.));
#17588=DIRECTION('ref_axis',(1.,0.,0.));
#17589=DIRECTION('',(0.,0.,-1.));
#17590=DIRECTION('center_axis',(0.,0.,-1.));
#17591=DIRECTION('ref_axis',(1.,0.,0.));
#17592=DIRECTION('',(0.,0.,-1.));
#17593=DIRECTION('center_axis',(0.,0.,-1.));
#17594=DIRECTION('ref_axis',(1.,0.,0.));
#17595=DIRECTION('',(0.,0.,-1.));
#17596=DIRECTION('center_axis',(0.,0.,-1.));
#17597=DIRECTION('ref_axis',(1.,0.,0.));
#17598=DIRECTION('',(0.,0.,-1.));
#17599=DIRECTION('center_axis',(0.,0.,-1.));
#17600=DIRECTION('ref_axis',(1.,0.,0.));
#17601=DIRECTION('',(0.,0.,-1.));
#17602=DIRECTION('center_axis',(0.,0.,-1.));
#17603=DIRECTION('ref_axis',(1.,0.,0.));
#17604=DIRECTION('',(0.,0.,-1.));
#17605=DIRECTION('center_axis',(0.,0.,-1.));
#17606=DIRECTION('ref_axis',(1.,0.,0.));
#17607=DIRECTION('',(0.,0.,-1.));
#17608=DIRECTION('center_axis',(0.,0.,-1.));
#17609=DIRECTION('ref_axis',(1.,0.,0.));
#17610=DIRECTION('',(0.,0.,-1.));
#17611=DIRECTION('center_axis',(0.,0.,-1.));
#17612=DIRECTION('ref_axis',(1.,0.,0.));
#17613=DIRECTION('',(0.,0.,-1.));
#17614=DIRECTION('center_axis',(0.,0.,-1.));
#17615=DIRECTION('ref_axis',(0.938439812457555,-0.345442785993033,0.));
#17616=DIRECTION('',(0.,0.,-1.));
#17617=DIRECTION('center_axis',(0.,0.,-1.));
#17618=DIRECTION('ref_axis',(1.,0.,0.));
#17619=DIRECTION('center_axis',(0.,0.,-1.));
#17620=DIRECTION('ref_axis',(-0.41770183671358,0.908584159891698,0.));
#17621=DIRECTION('',(1.22464679914735E-16,-1.35137073670524E-29,-1.));
#17622=DIRECTION('center_axis',(0.,0.,1.));
#17623=DIRECTION('ref_axis',(1.,-1.10225330100271E-13,0.));
#17624=DIRECTION('center_axis',(0.,0.,-1.));
#17625=DIRECTION('ref_axis',(1.,-1.10225330100271E-13,0.));
#17626=DIRECTION('',(1.22464679914735E-16,-1.35137073670524E-29,-1.));
#17627=DIRECTION('center_axis',(0.,0.,-1.));
#17628=DIRECTION('ref_axis',(1.,-1.10225330100271E-13,0.));
#17629=DIRECTION('',(1.22464679914735E-16,-1.35137073670524E-29,-1.));
#17630=DIRECTION('center_axis',(0.,0.,-1.));
#17631=DIRECTION('ref_axis',(1.,-1.10225330100271E-13,0.));
#17632=DIRECTION('',(1.22464679914735E-16,-1.35137073670524E-29,-1.));
#17633=DIRECTION('center_axis',(0.,0.,-1.));
#17634=DIRECTION('ref_axis',(1.,-1.10225330100271E-13,0.));
#17635=DIRECTION('',(1.22464679914735E-16,-1.35137073670524E-29,-1.));
#17636=DIRECTION('center_axis',(0.,0.,-1.));
#17637=DIRECTION('ref_axis',(1.,-1.10225330100271E-13,0.));
#17638=DIRECTION('',(1.22464679914735E-16,-1.35137073670524E-29,-1.));
#17639=DIRECTION('center_axis',(0.,0.,-1.));
#17640=DIRECTION('ref_axis',(1.,-1.10225330100271E-13,0.));
#17641=DIRECTION('',(1.22464679914735E-16,-1.35137073670524E-29,-1.));
#17642=DIRECTION('center_axis',(0.,0.,-1.));
#17643=DIRECTION('ref_axis',(1.,-1.10225330100271E-13,0.));
#17644=DIRECTION('',(1.22464679914735E-16,-1.35137073670524E-29,-1.));
#17645=DIRECTION('center_axis',(0.,0.,-1.));
#17646=DIRECTION('ref_axis',(1.,-1.10225330100271E-13,0.));
#17647=DIRECTION('',(1.22464679914735E-16,-1.35137073670524E-29,-1.));
#17648=DIRECTION('center_axis',(0.,0.,-1.));
#17649=DIRECTION('ref_axis',(1.,-1.10225330100271E-13,0.));
#17650=DIRECTION('',(1.22464679914735E-16,-1.35137073670524E-29,-1.));
#17651=DIRECTION('center_axis',(0.,0.,-1.));
#17652=DIRECTION('ref_axis',(1.,-1.10225330100271E-13,0.));
#17653=DIRECTION('',(1.22464679914735E-16,-1.35137073670524E-29,-1.));
#17654=DIRECTION('center_axis',(0.,0.,-1.));
#17655=DIRECTION('ref_axis',(1.,-1.10225330100271E-13,0.));
#17656=DIRECTION('',(1.22464679914735E-16,-1.35137073670524E-29,-1.));
#17657=DIRECTION('center_axis',(0.,0.,-1.));
#17658=DIRECTION('ref_axis',(1.,-1.10225330100271E-13,0.));
#17659=DIRECTION('',(1.22464679914735E-16,-1.35137073670524E-29,-1.));
#17660=DIRECTION('center_axis',(0.,0.,-1.));
#17661=DIRECTION('ref_axis',(1.,-1.10225330100271E-13,0.));
#17662=DIRECTION('',(1.22464679914735E-16,-1.35137073670524E-29,-1.));
#17663=DIRECTION('center_axis',(0.,0.,-1.));
#17664=DIRECTION('ref_axis',(1.,-1.10225330100271E-13,0.));
#17665=DIRECTION('',(1.22464679914735E-16,-1.35137073670524E-29,-1.));
#17666=DIRECTION('center_axis',(0.,0.,-1.));
#17667=DIRECTION('ref_axis',(1.,-1.10225330100271E-13,0.));
#17668=DIRECTION('',(1.22464679914735E-16,-1.35137073670524E-29,-1.));
#17669=DIRECTION('center_axis',(0.,0.,-1.));
#17670=DIRECTION('ref_axis',(1.,-1.10225330100271E-13,0.));
#17671=DIRECTION('',(1.22464679914735E-16,-1.35137073670524E-29,-1.));
#17672=DIRECTION('center_axis',(0.,0.,-1.));
#17673=DIRECTION('ref_axis',(1.,-1.10225330100271E-13,0.));
#17674=DIRECTION('',(1.22464679914735E-16,-1.35137073670524E-29,-1.));
#17675=DIRECTION('center_axis',(0.,0.,-1.));
#17676=DIRECTION('ref_axis',(-0.609338757688317,-0.792910006481731,0.));
#17677=DIRECTION('',(1.22464679914735E-16,-1.35137073670524E-29,-1.));
#17678=DIRECTION('center_axis',(0.,0.,-1.));
#17679=DIRECTION('ref_axis',(1.,-1.10225330100271E-13,0.));
#17680=DIRECTION('center_axis',(0.,0.,-1.));
#17681=DIRECTION('ref_axis',(1.,0.,0.));
#17682=DIRECTION('',(0.,0.,-1.));
#17683=DIRECTION('center_axis',(0.,0.,1.));
#17684=DIRECTION('ref_axis',(1.,0.,0.));
#17685=DIRECTION('',(0.,0.,-1.));
#17686=DIRECTION('center_axis',(0.,0.,1.));
#17687=DIRECTION('ref_axis',(1.,0.,0.));
#17688=DIRECTION('center_axis',(0.,0.,1.));
#17689=DIRECTION('ref_axis',(1.,0.,0.));
#17690=DIRECTION('center_axis',(0.,0.,-1.));
#17691=DIRECTION('ref_axis',(1.,0.,0.));
#17692=DIRECTION('',(0.,0.,-1.));
#17693=DIRECTION('center_axis',(0.,0.,-1.));
#17694=DIRECTION('ref_axis',(1.,0.,0.));
#17695=DIRECTION('',(0.,0.,-1.));
#17696=DIRECTION('center_axis',(0.,0.,-1.));
#17697=DIRECTION('ref_axis',(1.,0.,0.));
#17698=DIRECTION('',(0.,0.,-1.));
#17699=DIRECTION('center_axis',(0.,0.,-1.));
#17700=DIRECTION('ref_axis',(1.,0.,0.));
#17701=DIRECTION('',(0.,0.,-1.));
#17702=DIRECTION('center_axis',(0.,0.,-1.));
#17703=DIRECTION('ref_axis',(1.,0.,0.));
#17704=DIRECTION('',(0.,0.,-1.));
#17705=DIRECTION('center_axis',(0.,0.,-1.));
#17706=DIRECTION('ref_axis',(1.,0.,0.));
#17707=DIRECTION('',(0.,0.,-1.));
#17708=DIRECTION('center_axis',(0.,0.,-1.));
#17709=DIRECTION('ref_axis',(1.,0.,0.));
#17710=DIRECTION('',(0.,0.,-1.));
#17711=DIRECTION('center_axis',(0.,0.,-1.));
#17712=DIRECTION('ref_axis',(1.,0.,0.));
#17713=DIRECTION('',(0.,0.,-1.));
#17714=DIRECTION('center_axis',(0.,0.,-1.));
#17715=DIRECTION('ref_axis',(1.,0.,0.));
#17716=DIRECTION('',(0.,0.,-1.));
#17717=DIRECTION('center_axis',(0.,0.,-1.));
#17718=DIRECTION('ref_axis',(1.,0.,0.));
#17719=DIRECTION('',(0.,0.,-1.));
#17720=DIRECTION('center_axis',(0.,0.,-1.));
#17721=DIRECTION('ref_axis',(1.,0.,0.));
#17722=DIRECTION('',(0.,0.,-1.));
#17723=DIRECTION('center_axis',(0.,0.,-1.));
#17724=DIRECTION('ref_axis',(1.,0.,0.));
#17725=DIRECTION('',(0.,0.,-1.));
#17726=DIRECTION('center_axis',(0.,0.,-1.));
#17727=DIRECTION('ref_axis',(1.,0.,0.));
#17728=DIRECTION('',(0.,0.,-1.));
#17729=DIRECTION('center_axis',(0.,0.,-1.));
#17730=DIRECTION('ref_axis',(1.,0.,0.));
#17731=DIRECTION('',(0.,0.,-1.));
#17732=DIRECTION('center_axis',(0.,0.,-1.));
#17733=DIRECTION('ref_axis',(1.,0.,0.));
#17734=DIRECTION('',(0.,0.,-1.));
#17735=DIRECTION('center_axis',(0.,0.,-1.));
#17736=DIRECTION('ref_axis',(1.,0.,0.));
#17737=DIRECTION('',(0.,0.,-1.));
#17738=DIRECTION('center_axis',(0.,0.,-1.));
#17739=DIRECTION('ref_axis',(0.938439817930616,-0.345442771124758,0.));
#17740=DIRECTION('',(0.,0.,-1.));
#17741=DIRECTION('center_axis',(0.,0.,-1.));
#17742=DIRECTION('ref_axis',(1.,0.,0.));
#17743=DIRECTION('center_axis',(0.,0.,-1.));
#17744=DIRECTION('ref_axis',(-0.417701801892756,0.908584175899815,0.));
#17745=DIRECTION('',(1.22464679914735E-16,-1.37783879507626E-29,-1.));
#17746=DIRECTION('center_axis',(0.,0.,1.));
#17747=DIRECTION('ref_axis',(1.,-1.12386611082629E-13,0.));
#17748=DIRECTION('center_axis',(0.,0.,-1.));
#17749=DIRECTION('ref_axis',(1.,-1.12386611082629E-13,0.));
#17750=DIRECTION('',(1.22464679914735E-16,-1.37783879507626E-29,-1.));
#17751=DIRECTION('center_axis',(0.,0.,-1.));
#17752=DIRECTION('ref_axis',(1.,-1.12386611082629E-13,0.));
#17753=DIRECTION('',(1.22464679914735E-16,-1.37783879507626E-29,-1.));
#17754=DIRECTION('center_axis',(0.,0.,-1.));
#17755=DIRECTION('ref_axis',(1.,-1.12386611082629E-13,0.));
#17756=DIRECTION('',(1.22464679914735E-16,-1.37783879507626E-29,-1.));
#17757=DIRECTION('center_axis',(0.,0.,-1.));
#17758=DIRECTION('ref_axis',(1.,-1.12386611082629E-13,0.));
#17759=DIRECTION('',(1.22464679914735E-16,-1.37783879507626E-29,-1.));
#17760=DIRECTION('center_axis',(0.,0.,-1.));
#17761=DIRECTION('ref_axis',(1.,-1.12386611082629E-13,0.));
#17762=DIRECTION('',(1.22464679914735E-16,-1.37783879507626E-29,-1.));
#17763=DIRECTION('center_axis',(0.,0.,-1.));
#17764=DIRECTION('ref_axis',(1.,-1.12386611082629E-13,0.));
#17765=DIRECTION('',(1.22464679914735E-16,-1.37783879507626E-29,-1.));
#17766=DIRECTION('center_axis',(0.,0.,-1.));
#17767=DIRECTION('ref_axis',(1.,-1.12386611082629E-13,0.));
#17768=DIRECTION('',(1.22464679914735E-16,-1.37783879507626E-29,-1.));
#17769=DIRECTION('center_axis',(0.,0.,-1.));
#17770=DIRECTION('ref_axis',(1.,-1.12386611082629E-13,0.));
#17771=DIRECTION('',(1.22464679914735E-16,-1.37783879507626E-29,-1.));
#17772=DIRECTION('center_axis',(0.,0.,-1.));
#17773=DIRECTION('ref_axis',(1.,-1.12386611082629E-13,0.));
#17774=DIRECTION('',(1.22464679914735E-16,-1.37783879507626E-29,-1.));
#17775=DIRECTION('center_axis',(0.,0.,-1.));
#17776=DIRECTION('ref_axis',(1.,-1.12386611082629E-13,0.));
#17777=DIRECTION('',(1.22464679914735E-16,-1.37783879507626E-29,-1.));
#17778=DIRECTION('center_axis',(0.,0.,-1.));
#17779=DIRECTION('ref_axis',(1.,-1.12386611082629E-13,0.));
#17780=DIRECTION('',(1.22464679914735E-16,-1.37783879507626E-29,-1.));
#17781=DIRECTION('center_axis',(0.,0.,-1.));
#17782=DIRECTION('ref_axis',(1.,-1.12386611082629E-13,0.));
#17783=DIRECTION('',(1.22464679914735E-16,-1.37783879507626E-29,-1.));
#17784=DIRECTION('center_axis',(0.,0.,-1.));
#17785=DIRECTION('ref_axis',(1.,-1.12386611082629E-13,0.));
#17786=DIRECTION('',(1.22464679914735E-16,-1.37783879507626E-29,-1.));
#17787=DIRECTION('center_axis',(0.,0.,-1.));
#17788=DIRECTION('ref_axis',(1.,-1.12386611082629E-13,0.));
#17789=DIRECTION('',(1.22464679914735E-16,-1.37783879507626E-29,-1.));
#17790=DIRECTION('center_axis',(0.,0.,-1.));
#17791=DIRECTION('ref_axis',(1.,-1.12386611082629E-13,0.));
#17792=DIRECTION('',(1.22464679914735E-16,-1.37783879507626E-29,-1.));
#17793=DIRECTION('center_axis',(0.,0.,-1.));
#17794=DIRECTION('ref_axis',(1.,-1.12386611082629E-13,0.));
#17795=DIRECTION('',(1.22464679914735E-16,-1.37783879507626E-29,-1.));
#17796=DIRECTION('center_axis',(0.,0.,-1.));
#17797=DIRECTION('ref_axis',(1.,-1.12386611082629E-13,0.));
#17798=DIRECTION('',(1.22464679914735E-16,-1.37783879507626E-29,-1.));
#17799=DIRECTION('center_axis',(0.,0.,-1.));
#17800=DIRECTION('ref_axis',(-0.609338761677812,-0.792910003415867,0.));
#17801=DIRECTION('',(1.22464679914735E-16,-1.37783879507626E-29,-1.));
#17802=DIRECTION('center_axis',(0.,0.,-1.));
#17803=DIRECTION('ref_axis',(1.,-1.12386611082629E-13,0.));
#17804=DIRECTION('center_axis',(0.,0.,-1.));
#17805=DIRECTION('ref_axis',(1.,0.,0.));
#17806=DIRECTION('',(0.,0.,-1.));
#17807=DIRECTION('center_axis',(0.,0.,1.));
#17808=DIRECTION('ref_axis',(1.,0.,0.));
#17809=DIRECTION('',(0.,0.,-1.));
#17810=DIRECTION('center_axis',(0.,0.,1.));
#17811=DIRECTION('ref_axis',(1.,0.,0.));
#17812=DIRECTION('center_axis',(0.,0.,1.));
#17813=DIRECTION('ref_axis',(1.,0.,0.));
#17814=DIRECTION('center_axis',(0.,0.,-1.));
#17815=DIRECTION('ref_axis',(1.,0.,0.));
#17816=DIRECTION('',(0.,0.,-1.));
#17817=DIRECTION('center_axis',(0.,0.,-1.));
#17818=DIRECTION('ref_axis',(1.,0.,0.));
#17819=DIRECTION('',(0.,0.,-1.));
#17820=DIRECTION('center_axis',(0.,0.,-1.));
#17821=DIRECTION('ref_axis',(1.,0.,0.));
#17822=DIRECTION('',(0.,0.,-1.));
#17823=DIRECTION('center_axis',(0.,0.,-1.));
#17824=DIRECTION('ref_axis',(1.,0.,0.));
#17825=DIRECTION('',(0.,0.,-1.));
#17826=DIRECTION('center_axis',(0.,0.,-1.));
#17827=DIRECTION('ref_axis',(1.,0.,0.));
#17828=DIRECTION('',(0.,0.,-1.));
#17829=DIRECTION('center_axis',(0.,0.,-1.));
#17830=DIRECTION('ref_axis',(1.,0.,0.));
#17831=DIRECTION('',(0.,0.,-1.));
#17832=DIRECTION('center_axis',(0.,0.,-1.));
#17833=DIRECTION('ref_axis',(1.,0.,0.));
#17834=DIRECTION('',(0.,0.,-1.));
#17835=DIRECTION('center_axis',(0.,0.,-1.));
#17836=DIRECTION('ref_axis',(1.,0.,0.));
#17837=DIRECTION('',(0.,0.,-1.));
#17838=DIRECTION('center_axis',(0.,0.,-1.));
#17839=DIRECTION('ref_axis',(1.,0.,0.));
#17840=DIRECTION('',(0.,0.,-1.));
#17841=DIRECTION('center_axis',(0.,0.,-1.));
#17842=DIRECTION('ref_axis',(1.,0.,0.));
#17843=DIRECTION('',(0.,0.,-1.));
#17844=DIRECTION('center_axis',(0.,0.,-1.));
#17845=DIRECTION('ref_axis',(1.,0.,0.));
#17846=DIRECTION('',(0.,0.,-1.));
#17847=DIRECTION('center_axis',(0.,0.,-1.));
#17848=DIRECTION('ref_axis',(1.,0.,0.));
#17849=DIRECTION('',(0.,0.,-1.));
#17850=DIRECTION('center_axis',(0.,0.,-1.));
#17851=DIRECTION('ref_axis',(1.,0.,0.));
#17852=DIRECTION('',(0.,0.,-1.));
#17853=DIRECTION('center_axis',(0.,0.,-1.));
#17854=DIRECTION('ref_axis',(1.,0.,0.));
#17855=DIRECTION('',(0.,0.,-1.));
#17856=DIRECTION('center_axis',(0.,0.,-1.));
#17857=DIRECTION('ref_axis',(1.,0.,0.));
#17858=DIRECTION('',(0.,0.,-1.));
#17859=DIRECTION('center_axis',(0.,0.,-1.));
#17860=DIRECTION('ref_axis',(1.,0.,0.));
#17861=DIRECTION('',(0.,0.,-1.));
#17862=DIRECTION('center_axis',(0.,0.,-1.));
#17863=DIRECTION('ref_axis',(0.938439818752348,-0.345442768892418,0.));
#17864=DIRECTION('',(0.,0.,-1.));
#17865=DIRECTION('center_axis',(0.,0.,-1.));
#17866=DIRECTION('ref_axis',(1.,0.,0.));
#17867=DIRECTION('center_axis',(0.,0.,-1.));
#17868=DIRECTION('ref_axis',(-0.4177018103935,0.908584171991783,0.));
#17869=DIRECTION('',(1.22464679914735E-16,-1.32490267833421E-29,-1.));
#17870=DIRECTION('center_axis',(0.,0.,1.));
#17871=DIRECTION('ref_axis',(1.,-1.08064049117913E-13,0.));
#17872=DIRECTION('center_axis',(0.,0.,-1.));
#17873=DIRECTION('ref_axis',(1.,-1.08064049117913E-13,0.));
#17874=DIRECTION('',(1.22464679914735E-16,-1.32490267833421E-29,-1.));
#17875=DIRECTION('center_axis',(0.,0.,-1.));
#17876=DIRECTION('ref_axis',(1.,-1.08064049117913E-13,0.));
#17877=DIRECTION('',(1.22464679914735E-16,-1.32490267833421E-29,-1.));
#17878=DIRECTION('center_axis',(0.,0.,-1.));
#17879=DIRECTION('ref_axis',(1.,-1.08064049117913E-13,0.));
#17880=DIRECTION('',(1.22464679914735E-16,-1.32490267833421E-29,-1.));
#17881=DIRECTION('center_axis',(0.,0.,-1.));
#17882=DIRECTION('ref_axis',(1.,-1.08064049117913E-13,0.));
#17883=DIRECTION('',(1.22464679914735E-16,-1.32490267833421E-29,-1.));
#17884=DIRECTION('center_axis',(0.,0.,-1.));
#17885=DIRECTION('ref_axis',(1.,-1.08064049117913E-13,0.));
#17886=DIRECTION('',(1.22464679914735E-16,-1.32490267833421E-29,-1.));
#17887=DIRECTION('center_axis',(0.,0.,-1.));
#17888=DIRECTION('ref_axis',(1.,-1.08064049117913E-13,0.));
#17889=DIRECTION('',(1.22464679914735E-16,-1.32490267833421E-29,-1.));
#17890=DIRECTION('center_axis',(0.,0.,-1.));
#17891=DIRECTION('ref_axis',(1.,-1.08064049117913E-13,0.));
#17892=DIRECTION('',(1.22464679914735E-16,-1.32490267833421E-29,-1.));
#17893=DIRECTION('center_axis',(0.,0.,-1.));
#17894=DIRECTION('ref_axis',(1.,-1.08064049117913E-13,0.));
#17895=DIRECTION('',(1.22464679914735E-16,-1.32490267833421E-29,-1.));
#17896=DIRECTION('center_axis',(0.,0.,-1.));
#17897=DIRECTION('ref_axis',(1.,-1.08064049117913E-13,0.));
#17898=DIRECTION('',(1.22464679914735E-16,-1.32490267833421E-29,-1.));
#17899=DIRECTION('center_axis',(0.,0.,-1.));
#17900=DIRECTION('ref_axis',(1.,-1.08064049117913E-13,0.));
#17901=DIRECTION('',(1.22464679914735E-16,-1.32490267833421E-29,-1.));
#17902=DIRECTION('center_axis',(0.,0.,-1.));
#17903=DIRECTION('ref_axis',(1.,-1.08064049117913E-13,0.));
#17904=DIRECTION('',(1.22464679914735E-16,-1.32490267833421E-29,-1.));
#17905=DIRECTION('center_axis',(0.,0.,-1.));
#17906=DIRECTION('ref_axis',(1.,-1.08064049117913E-13,0.));
#17907=DIRECTION('',(1.22464679914735E-16,-1.32490267833421E-29,-1.));
#17908=DIRECTION('center_axis',(0.,0.,-1.));
#17909=DIRECTION('ref_axis',(1.,-1.08064049117913E-13,0.));
#17910=DIRECTION('',(1.22464679914735E-16,-1.32490267833421E-29,-1.));
#17911=DIRECTION('center_axis',(0.,0.,-1.));
#17912=DIRECTION('ref_axis',(1.,-1.08064049117913E-13,0.));
#17913=DIRECTION('',(1.22464679914735E-16,-1.32490267833421E-29,-1.));
#17914=DIRECTION('center_axis',(0.,0.,-1.));
#17915=DIRECTION('ref_axis',(1.,-1.08064049117913E-13,0.));
#17916=DIRECTION('',(1.22464679914735E-16,-1.32490267833421E-29,-1.));
#17917=DIRECTION('center_axis',(0.,0.,-1.));
#17918=DIRECTION('ref_axis',(1.,-1.08064049117913E-13,0.));
#17919=DIRECTION('',(1.22464679914735E-16,-1.32490267833421E-29,-1.));
#17920=DIRECTION('center_axis',(0.,0.,-1.));
#17921=DIRECTION('ref_axis',(1.,-1.08064049117913E-13,0.));
#17922=DIRECTION('',(1.22464679914735E-16,-1.32490267833421E-29,-1.));
#17923=DIRECTION('center_axis',(0.,0.,-1.));
#17924=DIRECTION('ref_axis',(-0.609338759590107,-0.792910005020235,0.));
#17925=DIRECTION('',(1.22464679914735E-16,-1.32490267833421E-29,-1.));
#17926=DIRECTION('center_axis',(0.,0.,-1.));
#17927=DIRECTION('ref_axis',(1.,-1.08064049117913E-13,0.));
#17928=DIRECTION('center_axis',(0.,0.,-1.));
#17929=DIRECTION('ref_axis',(1.,0.,0.));
#17930=DIRECTION('',(0.,0.,-1.));
#17931=DIRECTION('center_axis',(0.,0.,1.));
#17932=DIRECTION('ref_axis',(1.,0.,0.));
#17933=DIRECTION('',(0.,0.,-1.));
#17934=DIRECTION('center_axis',(0.,0.,1.));
#17935=DIRECTION('ref_axis',(1.,0.,0.));
#17936=DIRECTION('center_axis',(0.,0.,1.));
#17937=DIRECTION('ref_axis',(1.,0.,0.));
#17938=DIRECTION('center_axis',(0.,0.,-1.));
#17939=DIRECTION('ref_axis',(1.,0.,0.));
#17940=DIRECTION('',(0.,0.,-1.));
#17941=DIRECTION('center_axis',(0.,0.,-1.));
#17942=DIRECTION('ref_axis',(1.,0.,0.));
#17943=DIRECTION('',(0.,0.,-1.));
#17944=DIRECTION('center_axis',(0.,0.,-1.));
#17945=DIRECTION('ref_axis',(1.,0.,0.));
#17946=DIRECTION('',(0.,0.,-1.));
#17947=DIRECTION('center_axis',(0.,0.,-1.));
#17948=DIRECTION('ref_axis',(1.,0.,0.));
#17949=DIRECTION('',(0.,0.,-1.));
#17950=DIRECTION('center_axis',(0.,0.,-1.));
#17951=DIRECTION('ref_axis',(1.,0.,0.));
#17952=DIRECTION('',(0.,0.,-1.));
#17953=DIRECTION('center_axis',(0.,0.,-1.));
#17954=DIRECTION('ref_axis',(1.,0.,0.));
#17955=DIRECTION('',(0.,0.,-1.));
#17956=DIRECTION('center_axis',(0.,0.,-1.));
#17957=DIRECTION('ref_axis',(1.,0.,0.));
#17958=DIRECTION('',(0.,0.,-1.));
#17959=DIRECTION('center_axis',(0.,0.,-1.));
#17960=DIRECTION('ref_axis',(1.,0.,0.));
#17961=DIRECTION('',(0.,0.,-1.));
#17962=DIRECTION('center_axis',(0.,0.,-1.));
#17963=DIRECTION('ref_axis',(1.,0.,0.));
#17964=DIRECTION('',(0.,0.,-1.));
#17965=DIRECTION('center_axis',(0.,0.,-1.));
#17966=DIRECTION('ref_axis',(1.,0.,0.));
#17967=DIRECTION('',(0.,0.,-1.));
#17968=DIRECTION('center_axis',(0.,0.,-1.));
#17969=DIRECTION('ref_axis',(1.,0.,0.));
#17970=DIRECTION('',(0.,0.,-1.));
#17971=DIRECTION('center_axis',(0.,0.,-1.));
#17972=DIRECTION('ref_axis',(1.,0.,0.));
#17973=DIRECTION('',(0.,0.,-1.));
#17974=DIRECTION('center_axis',(0.,0.,-1.));
#17975=DIRECTION('ref_axis',(1.,0.,0.));
#17976=DIRECTION('',(0.,0.,-1.));
#17977=DIRECTION('center_axis',(0.,0.,-1.));
#17978=DIRECTION('ref_axis',(1.,0.,0.));
#17979=DIRECTION('',(0.,0.,-1.));
#17980=DIRECTION('center_axis',(0.,0.,-1.));
#17981=DIRECTION('ref_axis',(1.,0.,0.));
#17982=DIRECTION('',(0.,0.,-1.));
#17983=DIRECTION('center_axis',(0.,0.,-1.));
#17984=DIRECTION('ref_axis',(1.,0.,0.));
#17985=DIRECTION('',(0.,0.,-1.));
#17986=DIRECTION('center_axis',(0.,0.,-1.));
#17987=DIRECTION('ref_axis',(0.93843981373604,-0.345442782519866,0.));
#17988=DIRECTION('',(0.,0.,-1.));
#17989=DIRECTION('center_axis',(0.,0.,-1.));
#17990=DIRECTION('ref_axis',(1.,0.,0.));
#17991=DIRECTION('center_axis',(0.,0.,-1.));
#17992=DIRECTION('ref_axis',(-0.417701842212249,0.908584157363804,0.));
#17993=DIRECTION('',(1.22464679914735E-16,-1.40430685344729E-29,-1.));
#17994=DIRECTION('center_axis',(0.,0.,1.));
#17995=DIRECTION('ref_axis',(1.,-1.14547892064987E-13,0.));
#17996=DIRECTION('center_axis',(0.,0.,-1.));
#17997=DIRECTION('ref_axis',(1.,-1.14547892064987E-13,0.));
#17998=DIRECTION('',(1.22464679914735E-16,-1.40430685344729E-29,-1.));
#17999=DIRECTION('center_axis',(0.,0.,-1.));
#18000=DIRECTION('ref_axis',(1.,-1.14547892064987E-13,0.));
#18001=DIRECTION('',(1.22464679914735E-16,-1.40430685344729E-29,-1.));
#18002=DIRECTION('center_axis',(0.,0.,-1.));
#18003=DIRECTION('ref_axis',(1.,-1.14547892064987E-13,0.));
#18004=DIRECTION('',(1.22464679914735E-16,-1.40430685344729E-29,-1.));
#18005=DIRECTION('center_axis',(0.,0.,-1.));
#18006=DIRECTION('ref_axis',(1.,-1.14547892064987E-13,0.));
#18007=DIRECTION('',(1.22464679914735E-16,-1.40430685344729E-29,-1.));
#18008=DIRECTION('center_axis',(0.,0.,-1.));
#18009=DIRECTION('ref_axis',(1.,-1.14547892064987E-13,0.));
#18010=DIRECTION('',(1.22464679914735E-16,-1.40430685344729E-29,-1.));
#18011=DIRECTION('center_axis',(0.,0.,-1.));
#18012=DIRECTION('ref_axis',(1.,-1.14547892064987E-13,0.));
#18013=DIRECTION('',(1.22464679914735E-16,-1.40430685344729E-29,-1.));
#18014=DIRECTION('center_axis',(0.,0.,-1.));
#18015=DIRECTION('ref_axis',(1.,-1.14547892064987E-13,0.));
#18016=DIRECTION('',(1.22464679914735E-16,-1.40430685344729E-29,-1.));
#18017=DIRECTION('center_axis',(0.,0.,-1.));
#18018=DIRECTION('ref_axis',(1.,-1.14547892064987E-13,0.));
#18019=DIRECTION('',(1.22464679914735E-16,-1.40430685344729E-29,-1.));
#18020=DIRECTION('center_axis',(0.,0.,-1.));
#18021=DIRECTION('ref_axis',(1.,-1.14547892064987E-13,0.));
#18022=DIRECTION('',(1.22464679914735E-16,-1.40430685344729E-29,-1.));
#18023=DIRECTION('center_axis',(0.,0.,-1.));
#18024=DIRECTION('ref_axis',(1.,-1.14547892064987E-13,0.));
#18025=DIRECTION('',(1.22464679914735E-16,-1.40430685344729E-29,-1.));
#18026=DIRECTION('center_axis',(0.,0.,-1.));
#18027=DIRECTION('ref_axis',(1.,-1.14547892064987E-13,0.));
#18028=DIRECTION('',(1.22464679914735E-16,-1.40430685344729E-29,-1.));
#18029=DIRECTION('center_axis',(0.,0.,-1.));
#18030=DIRECTION('ref_axis',(1.,-1.14547892064987E-13,0.));
#18031=DIRECTION('',(1.22464679914735E-16,-1.40430685344729E-29,-1.));
#18032=DIRECTION('center_axis',(0.,0.,-1.));
#18033=DIRECTION('ref_axis',(1.,-1.14547892064987E-13,0.));
#18034=DIRECTION('',(1.22464679914735E-16,-1.40430685344729E-29,-1.));
#18035=DIRECTION('center_axis',(0.,0.,-1.));
#18036=DIRECTION('ref_axis',(1.,-1.14547892064987E-13,0.));
#18037=DIRECTION('',(1.22464679914735E-16,-1.40430685344729E-29,-1.));
#18038=DIRECTION('center_axis',(0.,0.,-1.));
#18039=DIRECTION('ref_axis',(1.,-1.14547892064987E-13,0.));
#18040=DIRECTION('',(1.22464679914735E-16,-1.40430685344729E-29,-1.));
#18041=DIRECTION('center_axis',(0.,0.,-1.));
#18042=DIRECTION('ref_axis',(1.,-1.14547892064987E-13,0.));
#18043=DIRECTION('',(1.22464679914735E-16,-1.40430685344729E-29,-1.));
#18044=DIRECTION('center_axis',(0.,0.,-1.));
#18045=DIRECTION('ref_axis',(1.,-1.14547892064987E-13,0.));
#18046=DIRECTION('',(1.22464679914735E-16,-1.40430685344729E-29,-1.));
#18047=DIRECTION('center_axis',(0.,0.,-1.));
#18048=DIRECTION('ref_axis',(-0.609338755970259,-0.792910007802031,0.));
#18049=DIRECTION('',(1.22464679914735E-16,-1.40430685344729E-29,-1.));
#18050=DIRECTION('center_axis',(0.,0.,-1.));
#18051=DIRECTION('ref_axis',(1.,-1.14547892064987E-13,0.));
#18052=DIRECTION('center_axis',(0.,0.,1.));
#18053=DIRECTION('ref_axis',(1.,0.,0.));
#18054=DIRECTION('center_axis',(0.,0.,-1.));
#18055=DIRECTION('ref_axis',(1.,-1.14547892064987E-13,0.));
#18056=DIRECTION('center_axis',(0.,0.,-1.));
#18057=DIRECTION('ref_axis',(1.,0.,0.));
#18058=DIRECTION('center_axis',(0.,0.,1.));
#18059=DIRECTION('ref_axis',(1.,0.,0.));
#18060=DIRECTION('center_axis',(0.,0.,-1.));
#18061=DIRECTION('ref_axis',(1.,-1.08064049117913E-13,0.));
#18062=DIRECTION('center_axis',(0.,0.,-1.));
#18063=DIRECTION('ref_axis',(1.,0.,0.));
#18064=DIRECTION('center_axis',(0.,0.,1.));
#18065=DIRECTION('ref_axis',(1.,0.,0.));
#18066=DIRECTION('center_axis',(0.,0.,-1.));
#18067=DIRECTION('ref_axis',(1.,-1.12386611082629E-13,0.));
#18068=DIRECTION('center_axis',(0.,0.,-1.));
#18069=DIRECTION('ref_axis',(1.,0.,0.));
#18070=DIRECTION('center_axis',(0.,0.,1.));
#18071=DIRECTION('ref_axis',(1.,0.,0.));
#18072=DIRECTION('center_axis',(0.,0.,-1.));
#18073=DIRECTION('ref_axis',(1.,-1.10225330100271E-13,0.));
#18074=DIRECTION('center_axis',(0.,0.,-1.));
#18075=DIRECTION('ref_axis',(1.,0.,0.));
#18076=DIRECTION('center_axis',(0.,0.,-1.));
#18077=DIRECTION('ref_axis',(1.,0.,0.));
#18078=DIRECTION('center_axis',(0.,0.,-1.));
#18079=DIRECTION('ref_axis',(1.,0.,0.));
#18080=DIRECTION('center_axis',(0.,0.,-1.));
#18081=DIRECTION('ref_axis',(1.,0.,0.));
#18082=DIRECTION('center_axis',(0.,0.,-1.));
#18083=DIRECTION('ref_axis',(1.,0.,0.));
#18084=DIRECTION('center_axis',(0.,0.,1.));
#18085=DIRECTION('ref_axis',(1.,0.,0.));
#18086=DIRECTION('center_axis',(0.,0.,1.));
#18087=DIRECTION('ref_axis',(-1.,-1.05902768135554E-13,0.));
#18088=DIRECTION('center_axis',(0.,0.,1.));
#18089=DIRECTION('ref_axis',(-1.,0.,0.));
#18090=DIRECTION('center_axis',(0.,0.,1.));
#18091=DIRECTION('ref_axis',(1.,0.,0.));
#18092=DIRECTION('center_axis',(0.,0.,1.));
#18093=DIRECTION('ref_axis',(-1.,-1.05902768135554E-13,0.));
#18094=DIRECTION('center_axis',(0.,0.,1.));
#18095=DIRECTION('ref_axis',(-1.,0.,0.));
#18096=DIRECTION('center_axis',(0.,0.,1.));
#18097=DIRECTION('ref_axis',(1.,0.,0.));
#18098=DIRECTION('center_axis',(0.,0.,1.));
#18099=DIRECTION('ref_axis',(-1.,-1.05902768135554E-13,0.));
#18100=DIRECTION('center_axis',(0.,0.,1.));
#18101=DIRECTION('ref_axis',(-1.,0.,0.));
#18102=DIRECTION('center_axis',(0.,0.,1.));
#18103=DIRECTION('ref_axis',(1.,0.,0.));
#18104=DIRECTION('center_axis',(0.,0.,1.));
#18105=DIRECTION('ref_axis',(-1.,-1.01580206170838E-13,0.));
#18106=DIRECTION('center_axis',(0.,0.,1.));
#18107=DIRECTION('ref_axis',(-1.,0.,0.));
#18108=DIRECTION('center_axis',(0.,0.,1.));
#18109=DIRECTION('ref_axis',(-1.,0.,0.));
#18110=DIRECTION('center_axis',(0.,0.,1.));
#18111=DIRECTION('ref_axis',(-1.,0.,0.));
#18112=DIRECTION('center_axis',(0.,0.,1.));
#18113=DIRECTION('ref_axis',(-1.,0.,0.));
#18114=DIRECTION('center_axis',(0.,0.,1.));
#18115=DIRECTION('ref_axis',(-1.,0.,0.));
#18116=DIRECTION('center_axis',(0.,-1.,0.));
#18117=DIRECTION('ref_axis',(-1.,0.,0.));
#18118=DIRECTION('',(0.,0.,-1.));
#18119=DIRECTION('',(-1.,0.,0.));
#18120=DIRECTION('',(0.,0.,-1.));
#18121=DIRECTION('',(1.,0.,0.));
#18122=DIRECTION('center_axis',(1.,0.,0.));
#18123=DIRECTION('ref_axis',(0.,-1.,0.));
#18124=DIRECTION('',(0.,-1.,0.));
#18125=DIRECTION('',(0.,0.,-1.));
#18126=DIRECTION('',(0.,1.,0.));
#18127=DIRECTION('center_axis',(0.,1.,0.));
#18128=DIRECTION('ref_axis',(1.,0.,0.));
#18129=DIRECTION('',(0.,0.,1.));
#18130=DIRECTION('',(-1.,0.,0.));
#18131=DIRECTION('',(1.,0.,0.));
#18132=DIRECTION('center_axis',(0.,0.,1.));
#18133=DIRECTION('ref_axis',(1.,0.,0.));
#18134=DIRECTION('center_axis',(0.,0.,1.));
#18135=DIRECTION('ref_axis',(1.,0.,0.));
#18136=DIRECTION('center_axis',(0.,0.,-1.));
#18137=DIRECTION('ref_axis',(1.,0.,0.));
#18138=DIRECTION('center_axis',(0.,0.,-1.));
#18139=DIRECTION('ref_axis',(1.,-3.92491481346641E-15,0.));
#18140=DIRECTION('center_axis',(0.,0.,1.));
#18141=DIRECTION('ref_axis',(1.,0.,0.));
#18142=DIRECTION('center_axis',(0.,0.,1.));
#18143=DIRECTION('ref_axis',(1.,0.,0.));
#18144=DIRECTION('',(1.,0.,0.));
#18145=DIRECTION('',(0.,1.,0.));
#18146=DIRECTION('',(-1.,0.,0.));
#18147=DIRECTION('center_axis',(0.,0.,-1.));
#18148=DIRECTION('ref_axis',(1.,0.,0.));
#18149=DIRECTION('center_axis',(0.,-1.,0.));
#18150=DIRECTION('ref_axis',(1.,0.,0.));
#18151=DIRECTION('',(0.,0.,1.));
#18152=DIRECTION('',(1.,0.,0.));
#18153=DIRECTION('',(0.,0.,1.));
#18154=DIRECTION('center_axis',(0.,1.,0.));
#18155=DIRECTION('ref_axis',(-1.,0.,0.));
#18156=DIRECTION('',(0.,0.,-1.));
#18157=DIRECTION('',(0.,0.,1.));
#18158=DIRECTION('',(-1.,0.,0.));
#18159=DIRECTION('center_axis',(1.,0.,0.));
#18160=DIRECTION('ref_axis',(0.,1.,0.));
#18161=DIRECTION('',(0.,1.,0.));
#18162=DIRECTION('center_axis',(0.,0.,1.));
#18163=DIRECTION('ref_axis',(1.,0.,0.));
#18164=DIRECTION('center_axis',(0.,0.,-1.));
#18165=DIRECTION('ref_axis',(1.,0.,0.));
#18166=DIRECTION('center_axis',(0.,0.,1.));
#18167=DIRECTION('ref_axis',(1.,0.,0.));
#18168=DIRECTION('center_axis',(0.,0.,-1.));
#18169=DIRECTION('ref_axis',(1.,0.,0.));
#18170=DIRECTION('center_axis',(0.,0.,-1.));
#18171=DIRECTION('ref_axis',(1.,0.,0.));
#18172=DIRECTION('center_axis',(0.,0.,1.));
#18173=DIRECTION('ref_axis',(1.,0.,0.));
#18174=DIRECTION('center_axis',(0.,0.,1.));
#18175=DIRECTION('ref_axis',(1.,0.,0.));
#18176=DIRECTION('center_axis',(0.,0.,-1.));
#18177=DIRECTION('ref_axis',(1.,0.,0.));
#18178=DIRECTION('center_axis',(0.,0.,1.));
#18179=DIRECTION('ref_axis',(1.,0.,0.));
#18180=DIRECTION('',(0.,0.,-1.));
#18181=DIRECTION('center_axis',(0.,0.,1.));
#18182=DIRECTION('ref_axis',(1.,0.,0.));
#18183=DIRECTION('',(0.,0.,-1.));
#18184=DIRECTION('center_axis',(0.,0.,-1.));
#18185=DIRECTION('ref_axis',(1.,0.,0.));
#18186=DIRECTION('center_axis',(0.,0.,1.));
#18187=DIRECTION('ref_axis',(1.,0.,0.));
#18188=DIRECTION('center_axis',(0.,0.,-1.));
#18189=DIRECTION('ref_axis',(1.,0.,0.));
#18190=DIRECTION('center_axis',(0.,0.,1.));
#18191=DIRECTION('ref_axis',(1.,0.,0.));
#18192=DIRECTION('center_axis',(0.,0.,1.));
#18193=DIRECTION('ref_axis',(1.,0.,0.));
#18194=DIRECTION('center_axis',(0.,0.,-1.));
#18195=DIRECTION('ref_axis',(1.,0.,0.));
#18196=DIRECTION('center_axis',(0.,0.,1.));
#18197=DIRECTION('ref_axis',(1.,0.,0.));
#18198=DIRECTION('',(0.,0.,-1.));
#18199=DIRECTION('center_axis',(0.,0.,1.));
#18200=DIRECTION('ref_axis',(1.,0.,0.));
#18201=DIRECTION('',(0.,0.,-1.));
#18202=DIRECTION('center_axis',(0.,0.,1.));
#18203=DIRECTION('ref_axis',(1.,0.,0.));
#18204=DIRECTION('center_axis',(0.,0.,-1.));
#18205=DIRECTION('ref_axis',(1.,0.,0.));
#18206=DIRECTION('',(0.,0.,-1.));
#18207=DIRECTION('center_axis',(0.,0.,1.));
#18208=DIRECTION('ref_axis',(1.,0.,0.));
#18209=DIRECTION('center_axis',(0.,0.,1.));
#18210=DIRECTION('ref_axis',(1.,0.,0.));
#18211=DIRECTION('center_axis',(0.,0.,1.));
#18212=DIRECTION('ref_axis',(1.,0.,0.));
#20082=CARTESIAN_POINT('',(0.,0.,0.));
#20083=CARTESIAN_POINT('Origin',(80.,0.,48.));
#20084=CARTESIAN_POINT('',(74.8632856275073,0.000121616040080763,42.4259584946969));
#20085=CARTESIAN_POINT('',(74.86325,6.29070444552017E-16,42.));
#20086=CARTESIAN_POINT('',(74.86325,6.29070444552017E-16,48.));
#20087=CARTESIAN_POINT('',(79.7872015765661,5.13234034271734,42.));
#20088=CARTESIAN_POINT('Origin',(80.,0.,42.));
#20089=CARTESIAN_POINT('Ctrl Pts',(79.7872818445161,5.13260507264869,42.));
#20090=CARTESIAN_POINT('Ctrl Pts',(79.0562851507116,5.10168006756045,42.0396772434995));
#20091=CARTESIAN_POINT('Ctrl Pts',(78.3315536646317,4.91345033611241,42.079354486999));
#20092=CARTESIAN_POINT('Ctrl Pts',(77.6789039388635,4.58290131773057,42.1190317304985));
#20093=CARTESIAN_POINT('Ctrl Pts',(76.9301312492104,4.20366867917444,42.1645526817226));
#20094=CARTESIAN_POINT('Ctrl Pts',(76.2762364578729,3.6371077237785,42.2100736329468));
#20095=CARTESIAN_POINT('Ctrl Pts',(75.7942602890204,2.94995818481276,42.2555945841709));
#20096=CARTESIAN_POINT('Ctrl Pts',(75.3122841201679,2.26280864584703,42.3011155353951));
#20097=CARTESIAN_POINT('Ctrl Pts',(75.0022265738003,1.45507052331149,42.3466364866192));
#20098=CARTESIAN_POINT('Ctrl Pts',(74.9006161199858,0.621912016979159,42.3921574378433));
#20099=CARTESIAN_POINT('Ctrl Pts',(74.8754662301444,0.415694606583752,42.4034244567945));
#20100=CARTESIAN_POINT('Ctrl Pts',(74.8630863502092,0.207919877499314,42.4146914757457));
#20101=CARTESIAN_POINT('Ctrl Pts',(74.8632856275073,0.000121616040080763,
42.4259584946969));
#20102=CARTESIAN_POINT('Origin',(80.,0.,48.));
#20103=CARTESIAN_POINT('',(74.8628762025111,4.99008593407568E-5,44.1759584946969));
#20104=CARTESIAN_POINT('',(74.8636304222849,4.19133500426576E-5,43.6990415053031));
#20105=CARTESIAN_POINT('',(74.86325,6.29070444552017E-16,48.));
#20106=CARTESIAN_POINT('',(74.9489860411411,-0.934590043769125,42.));
#20107=CARTESIAN_POINT('Ctrl Pts',(74.8636304222849,4.19133500426576E-5,
43.6990415053031));
#20108=CARTESIAN_POINT('Ctrl Pts',(74.8635208617496,0.370740519310411,43.6789457515585));
#20109=CARTESIAN_POINT('Ctrl Pts',(74.9031296129329,0.741416057941528,43.6588499978138));
#20110=CARTESIAN_POINT('Ctrl Pts',(74.9827083545788,1.10330220113088,43.6387542440692));
#20111=CARTESIAN_POINT('Ctrl Pts',(75.1629703175275,1.92304759023842,43.593233292845));
#20112=CARTESIAN_POINT('Ctrl Pts',(75.5483239883248,2.69769334081098,43.5477123416209));
#20113=CARTESIAN_POINT('Ctrl Pts',(76.0933689928018,3.3359744761171,43.5021913903967));
#20114=CARTESIAN_POINT('Ctrl Pts',(76.6384139972788,3.97425561142324,43.4566704391726));
#20115=CARTESIAN_POINT('Ctrl Pts',(77.3431503354356,4.47617213146291,43.4111494879485));
#20116=CARTESIAN_POINT('Ctrl Pts',(78.1245493196722,4.78259088641757,43.3656285367243));
#20117=CARTESIAN_POINT('Ctrl Pts',(78.9059483039088,5.08900964137223,43.3201075855002));
#20118=CARTESIAN_POINT('Ctrl Pts',(79.7640099342254,5.19993063124186,43.274586634276));
#20119=CARTESIAN_POINT('Ctrl Pts',(80.5976420089561,5.10228536737467,43.2290656830519));
#20120=CARTESIAN_POINT('Ctrl Pts',(81.4312740836868,5.00464010350749,43.1835447318277));
#20121=CARTESIAN_POINT('Ctrl Pts',(82.2404766028315,4.69842858590349,43.1380237806036));
#20122=CARTESIAN_POINT('Ctrl Pts',(82.9299126180493,4.2197278344979,43.0925028293795));
#20123=CARTESIAN_POINT('Ctrl Pts',(83.619348633267,3.74102708309231,43.0469818781553));
#20124=CARTESIAN_POINT('Ctrl Pts',(84.1890181445578,3.08983709788513,43.0014609269312));
#20125=CARTESIAN_POINT('Ctrl Pts',(84.5718071021192,2.34287633816629,42.955939975707));
#20126=CARTESIAN_POINT('Ctrl Pts',(84.9545960596807,1.59591557844745,42.9104190244829));
#20127=CARTESIAN_POINT('Ctrl Pts',(85.1505044635128,0.753184044216937,42.8648980732587));
#20128=CARTESIAN_POINT('Ctrl Pts',(85.1364480089129,-0.0860286291164032,
42.8193771220346));
#20129=CARTESIAN_POINT('Ctrl Pts',(85.1223915543129,-0.925241302449768,
42.7738561708104));
#20130=CARTESIAN_POINT('Ctrl Pts',(84.8983702412809,-1.76093511488598,42.7283352195863));
#20131=CARTESIAN_POINT('Ctrl Pts',(84.4907843336716,-2.4946596112628,42.6828142683622));
#20132=CARTESIAN_POINT('Ctrl Pts',(84.0831984260624,-3.22838410763962,42.637293317138));
#20133=CARTESIAN_POINT('Ctrl Pts',(83.4920479238758,-3.86013928795704,42.5917723659139));
#20134=CARTESIAN_POINT('Ctrl Pts',(82.786964128127,-4.31548031249223,42.5462514146897));
#20135=CARTESIAN_POINT('Ctrl Pts',(82.0818803323782,-4.77082133702742,42.5007304634656));
#20136=CARTESIAN_POINT('Ctrl Pts',(81.2628632430673,-5.04974820578038,42.4552095122414));
#20137=CARTESIAN_POINT('Ctrl Pts',(80.4264389659417,-5.11943010927012,42.4096885610173));
#20138=CARTESIAN_POINT('Ctrl Pts',(79.5900146888162,-5.18911201275987,42.3641676097932));
#20139=CARTESIAN_POINT('Ctrl Pts',(78.7361832238761,-5.04954895098638,42.318646658569));
#20140=CARTESIAN_POINT('Ctrl Pts',(77.96547438976,-4.7171163339107,42.2731257073449));
#20141=CARTESIAN_POINT('Ctrl Pts',(77.1947655556439,-4.38468371683501,42.2276047561207));
#20142=CARTESIAN_POINT('Ctrl Pts',(76.5071793523518,-3.85938154445711,42.1820838048966));
#20143=CARTESIAN_POINT('Ctrl Pts',(75.9839213652191,-3.20324008292404,42.1365628536724));
#20144=CARTESIAN_POINT('Ctrl Pts',(75.4606633780864,-2.54709862139098,42.0910419024483));
#20145=CARTESIAN_POINT('Ctrl Pts',(75.1017336071131,-1.76011787070275,42.0455209512241));
#20146=CARTESIAN_POINT('Ctrl Pts',(74.9489860411411,-0.934590043769161,
42.));
#20147=CARTESIAN_POINT('Origin',(80.,0.,42.));
#20148=CARTESIAN_POINT('Ctrl Pts',(74.8632856275073,0.000121616040080763,
42.4259584946969));
#20149=CARTESIAN_POINT('Ctrl Pts',(74.86389146931,-0.631625575059074,42.4602124269698));
#20150=CARTESIAN_POINT('Ctrl Pts',(74.9807637485846,-1.26359027082345,42.4944663592428));
#20151=CARTESIAN_POINT('Ctrl Pts',(75.2085395310293,-1.85267328325476,42.5287202915158));
#20152=CARTESIAN_POINT('Ctrl Pts',(75.5112367571486,-2.63552118702721,42.5742412427399));
#20153=CARTESIAN_POINT('Ctrl Pts',(76.0097945706485,-3.34263810444295,42.6197621939641));
#20154=CARTESIAN_POINT('Ctrl Pts',(76.6454751600456,-3.89071404950825,42.6652831451882));
#20155=CARTESIAN_POINT('Ctrl Pts',(77.2811557494428,-4.43878999457355,42.7108040964123));
#20156=CARTESIAN_POINT('Ctrl Pts',(78.0539591147372,-4.82782496728842,42.7563250476365));
#20157=CARTESIAN_POINT('Ctrl Pts',(78.8728375123135,-5.01198527001719,42.8018459988606));
#20158=CARTESIAN_POINT('Ctrl Pts',(79.6917159098899,-5.19614557274597,42.8473669500848));
#20159=CARTESIAN_POINT('Ctrl Pts',(80.5566693397482,-5.1754312054887,42.8928879013089));
#20160=CARTESIAN_POINT('Ctrl Pts',(81.3657932499147,-4.95228241379094,42.9384088525331));
#20161=CARTESIAN_POINT('Ctrl Pts',(82.1749171600812,-4.72913362209319,42.9839298037572));
#20162=CARTESIAN_POINT('Ctrl Pts',(82.9282115505558,-4.30355040595498,43.0294507549814));
#20163=CARTESIAN_POINT('Ctrl Pts',(83.5369270500077,-3.72567296245263,43.0749717062055));
#20164=CARTESIAN_POINT('Ctrl Pts',(84.1456425494596,-3.14779551895029,43.1204926574296));
#20165=CARTESIAN_POINT('Ctrl Pts',(84.6097791578887,-2.41762384808381,43.1660136086538));
#20166=CARTESIAN_POINT('Ctrl Pts',(84.8746546014611,-1.62118309157148,43.2115345598779));
#20167=CARTESIAN_POINT('Ctrl Pts',(85.1395300450336,-0.824742335059147,
43.2570555111021));
#20168=CARTESIAN_POINT('Ctrl Pts',(85.2051443237493,0.0379675070990354,
43.3025764623262));
#20169=CARTESIAN_POINT('Ctrl Pts',(85.0637670949036,0.865306235619404,43.3480974135504));
#20170=CARTESIAN_POINT('Ctrl Pts',(84.9223898660578,1.69264496413977,43.3936183647745));
#20171=CARTESIAN_POINT('Ctrl Pts',(84.5740211296506,2.48461257902233,43.4391393159986));
#20172=CARTESIAN_POINT('Ctrl Pts',(84.0597039528812,3.14790341083024,43.4846602672228));
#20173=CARTESIAN_POINT('Ctrl Pts',(83.5453867761118,3.81119424263815,43.5301812184469));
#20174=CARTESIAN_POINT('Ctrl Pts',(82.8651211589803,4.34580829137141,43.5757021696711));
#20175=CARTESIAN_POINT('Ctrl Pts',(82.0990526094627,4.68875998754711,43.6212231208952));
#20176=CARTESIAN_POINT('Ctrl Pts',(81.332984059945,5.03171168372281,43.6667440721194));
#20177=CARTESIAN_POINT('Ctrl Pts',(80.4811125780413,5.18300102734094,43.7122650233435));
#20178=CARTESIAN_POINT('Ctrl Pts',(79.64380141847,5.12480386375012,43.7577859745677));
#20179=CARTESIAN_POINT('Ctrl Pts',(78.8064902588986,5.06660670015931,43.8033069257918));
#20180=CARTESIAN_POINT('Ctrl Pts',(77.9837394216597,4.79892302935956,43.8488278770159));
#20181=CARTESIAN_POINT('Ctrl Pts',(77.2724813128825,4.35329000715137,43.8943488282401));
#20182=CARTESIAN_POINT('Ctrl Pts',(76.5612232041052,3.90765698494317,43.9398697794642));
#20183=CARTESIAN_POINT('Ctrl Pts',(75.9614578237895,3.28407461132652,43.9853907306884));
#20184=CARTESIAN_POINT('Ctrl Pts',(75.5438465417775,2.556010256289,44.0309116819125));
#20185=CARTESIAN_POINT('Ctrl Pts',(75.1262352597655,1.82794590125149,44.0764326331367));
#20186=CARTESIAN_POINT('Ctrl Pts',(74.8907780760572,0.995399564793116,44.1219535843608));
#20187=CARTESIAN_POINT('Ctrl Pts',(74.8652153833832,0.156457709503931,44.1674745355849));
#20188=CARTESIAN_POINT('Ctrl Pts',(74.8636273026306,0.10433849694978,44.1703025219556));
#20189=CARTESIAN_POINT('Ctrl Pts',(74.862849311385,0.0521946008383264,44.1731305083262));
#20190=CARTESIAN_POINT('Ctrl Pts',(74.8628762025111,4.99008593407568E-5,
44.1759584946969));
#20191=CARTESIAN_POINT('Origin',(80.,0.,48.));
#20192=CARTESIAN_POINT('',(74.8629839453475,-8.98047708566482E-5,45.9259584946969));
#20193=CARTESIAN_POINT('',(74.8633066453123,0.000121786292464538,45.4490415053031));
#20194=CARTESIAN_POINT('',(74.86325,6.29070444552017E-16,48.));
#20195=CARTESIAN_POINT('Ctrl Pts',(74.8633066453123,0.000121786292464538,
45.4490415053031));
#20196=CARTESIAN_POINT('Ctrl Pts',(74.8631028564357,0.215109900456405,45.437384784139));
#20197=CARTESIAN_POINT('Ctrl Pts',(74.8763564073468,0.430073059765048,45.4257280629749));
#20198=CARTESIAN_POINT('Ctrl Pts',(74.9032715236375,0.643311848838259,45.4140713418108));
#20199=CARTESIAN_POINT('Ctrl Pts',(75.0083784124968,1.47603593821421,45.3685503905866));
#20200=CARTESIAN_POINT('Ctrl Pts',(75.3218241722691,2.28246338164187,45.3230294393625));
#20201=CARTESIAN_POINT('Ctrl Pts',(75.8066801846642,2.96758491418775,45.2775084881384));
#20202=CARTESIAN_POINT('Ctrl Pts',(76.2915361970593,3.65270644673361,45.2319875369142));
#20203=CARTESIAN_POINT('Ctrl Pts',(76.9478024620773,4.21652206839771,45.1864665856901));
#20204=CARTESIAN_POINT('Ctrl Pts',(77.6981609569454,4.59260583073588,45.1409456344659));
#20205=CARTESIAN_POINT('Ctrl Pts',(78.4485194518134,4.96868959307406,45.0954246832418));
#20206=CARTESIAN_POINT('Ctrl Pts',(79.2929701765315,5.1570414960863,45.0499037320176));
#20207=CARTESIAN_POINT('Ctrl Pts',(80.132024152519,5.13547085667211,45.0043827807935));
#20208=CARTESIAN_POINT('Ctrl Pts',(80.9710781285065,5.11390021725791,44.9588618295693));
#20209=CARTESIAN_POINT('Ctrl Pts',(81.8047353557635,4.88240703541727,44.9133408783452));
#20210=CARTESIAN_POINT('Ctrl Pts',(82.5347784918799,4.46826468483543,44.8678199271211));
#20211=CARTESIAN_POINT('Ctrl Pts',(83.2648216279964,4.0541223342536,44.8222989758969));
#20212=CARTESIAN_POINT('Ctrl Pts',(83.8912506729723,3.45733081493057,44.7767780246728));
#20213=CARTESIAN_POINT('Ctrl Pts',(84.3402628766027,2.74820113140603,44.7312570734486));
#20214=CARTESIAN_POINT('Ctrl Pts',(84.7892750802332,2.0390714478815,44.6857361222245));
#20215=CARTESIAN_POINT('Ctrl Pts',(85.0608704425183,1.21760360015545,44.6402151710004));
#20216=CARTESIAN_POINT('Ctrl Pts',(85.1230509507437,0.38057883852083,44.5946942197762));
#20217=CARTESIAN_POINT('Ctrl Pts',(85.1852314589692,-0.456445923113787,
44.5491732685521));
#20218=CARTESIAN_POINT('Ctrl Pts',(85.037997113135,-1.30902759865697,44.5036523173279));
#20219=CARTESIAN_POINT('Ctrl Pts',(84.6986943301815,-2.07671926105541,44.4581313661038));
#20220=CARTESIAN_POINT('Ctrl Pts',(84.359391547228,-2.84441092345386,44.4126104148796));
#20221=CARTESIAN_POINT('Ctrl Pts',(83.8280203271551,-3.52721257270756,44.3670894636555));
#20222=CARTESIAN_POINT('Ctrl Pts',(83.167184181402,-4.04467991999574,44.3215685124314));
#20223=CARTESIAN_POINT('Ctrl Pts',(82.506348035649,-4.56214726728393,44.2760475612072));
#20224=CARTESIAN_POINT('Ctrl Pts',(81.7160469642156,-4.91428031260659,44.2305266099831));
#20225=CARTESIAN_POINT('Ctrl Pts',(80.8893903014861,-5.05959249273419,44.1850056587589));
#20226=CARTESIAN_POINT('Ctrl Pts',(80.0627336387566,-5.2049046728618,44.1394847075348));
#20227=CARTESIAN_POINT('Ctrl Pts',(79.1997213847309,-5.14339598779434,44.0939637563106));
#20228=CARTESIAN_POINT('Ctrl Pts',(78.4020293485828,-4.88231308796566,44.0484428050865));
#20229=CARTESIAN_POINT('Ctrl Pts',(77.6043373124346,-4.62123018813698,44.0029218538623));
#20230=CARTESIAN_POINT('Ctrl Pts',(76.871965494164,-4.16057307354708,43.9574009026382));
#20231=CARTESIAN_POINT('Ctrl Pts',(76.2911982859515,-3.55461406363621,43.911879951414));
#20232=CARTESIAN_POINT('Ctrl Pts',(75.710431077739,-2.94865505372537,43.8663590001899));
#20233=CARTESIAN_POINT('Ctrl Pts',(75.2812684795846,-2.19739414849357,43.8208380489657));
#20234=CARTESIAN_POINT('Ctrl Pts',(75.0542723080574,-1.38934118205641,43.7753170977416));
#20235=CARTESIAN_POINT('Ctrl Pts',(74.9274862385012,-0.93801260273047,43.7498919002621));
#20236=CARTESIAN_POINT('Ctrl Pts',(74.8637690385459,-0.46896688232286,43.7244667027826));
#20237=CARTESIAN_POINT('Ctrl Pts',(74.8636304222849,4.19133500426576E-5,
43.6990415053031));
#20238=CARTESIAN_POINT('Ctrl Pts',(74.8628762025111,4.99008593407568E-5,
44.1759584946969));
#20239=CARTESIAN_POINT('Ctrl Pts',(74.8632821669507,-0.787157515205568,
44.2186514595504));
#20240=CARTESIAN_POINT('Ctrl Pts',(75.047126602999,-1.57454813845282,44.2613444244039));
#20241=CARTESIAN_POINT('Ctrl Pts',(75.3964937240302,-2.27996097356572,44.3040373892574));
#20242=CARTESIAN_POINT('Ctrl Pts',(75.7690029589908,-3.03210042722621,44.3495583404815));
#20243=CARTESIAN_POINT('Ctrl Pts',(76.3296896305517,-3.69104196042718,44.3950792917057));
#20244=CARTESIAN_POINT('Ctrl Pts',(77.0124964276053,-4.17915236366638,44.4406002429298));
#20245=CARTESIAN_POINT('Ctrl Pts',(77.695303224659,-4.66726276690558,44.4861211941539));
#20246=CARTESIAN_POINT('Ctrl Pts',(78.5002301472054,-4.98454204018302,44.5316421453781));
#20247=CARTESIAN_POINT('Ctrl Pts',(79.3324447141988,-5.09360991972006,44.5771630966022));
#20248=CARTESIAN_POINT('Ctrl Pts',(80.1646592811922,-5.20267779925709,44.6226840478264));
#20249=CARTESIAN_POINT('Ctrl Pts',(81.0241614926327,-5.10353428505372,44.6682049990505));
#20250=CARTESIAN_POINT('Ctrl Pts',(81.8096890787593,-4.80785997217622,44.7137259502747));
#20251=CARTESIAN_POINT('Ctrl Pts',(82.5952166648858,-4.51218565929872,44.7592469014988));
#20252=CARTESIAN_POINT('Ctrl Pts',(83.3067696256985,-4.01998054774709,44.804767852723));
#20253=CARTESIAN_POINT('Ctrl Pts',(83.8605163352739,-3.38923379230978,44.8502888039471));
#20254=CARTESIAN_POINT('Ctrl Pts',(84.4142630448494,-2.75848703687247,44.8958097551712));
#20255=CARTESIAN_POINT('Ctrl Pts',(84.8102035031877,-1.98919863754947,44.9413307063954));
#20256=CARTESIAN_POINT('Ctrl Pts',(85.0016899774868,-1.17200232207685,44.9868516576195));
#20257=CARTESIAN_POINT('Ctrl Pts',(85.1931764517859,-0.354806006604231,
45.0323726088437));
#20258=CARTESIAN_POINT('Ctrl Pts',(85.1802089420458,0.510298225017999,45.0778935600678));
#20259=CARTESIAN_POINT('Ctrl Pts',(84.9643152156786,1.32138810091097,45.123414511292));
#20260=CARTESIAN_POINT('Ctrl Pts',(84.7484214893113,2.13247797680394,45.1689354625161));
#20261=CARTESIAN_POINT('Ctrl Pts',(84.329601546317,2.88955349696764,45.2144564137403));
#20262=CARTESIAN_POINT('Ctrl Pts',(83.757198666428,3.50341979426373,45.2599773649644));
#20263=CARTESIAN_POINT('Ctrl Pts',(83.1847957865391,4.11728609155982,45.3054983161885));
#20264=CARTESIAN_POINT('Ctrl Pts',(82.4588099697556,4.5879431659883,45.3510192674127));
#20265=CARTESIAN_POINT('Ctrl Pts',(81.6647732492066,4.85994054516851,45.3965402186368));
#20266=CARTESIAN_POINT('Ctrl Pts',(80.8707365286577,5.13193792434872,45.442061169861));
#20267=CARTESIAN_POINT('Ctrl Pts',(80.0086489043433,5.20527560828067,45.4875821210851));
#20268=CARTESIAN_POINT('Ctrl Pts',(79.1800772464949,5.07131331630493,45.5331030723093));
#20269=CARTESIAN_POINT('Ctrl Pts',(78.3515055886465,4.93735102432919,45.5786240235334));
#20270=CARTESIAN_POINT('Ctrl Pts',(77.556449897264,4.59608875644576,45.6241449747576));
#20271=CARTESIAN_POINT('Ctrl Pts',(76.8885796740965,4.087732333385,45.6696659259817));
#20272=CARTESIAN_POINT('Ctrl Pts',(76.2207094509289,3.57937591032425,45.7151868772058));
#20273=CARTESIAN_POINT('Ctrl Pts',(75.6800246959761,2.90392533208616,45.76070782843));
#20274=CARTESIAN_POINT('Ctrl Pts',(75.3302261941625,2.14095882168743,45.8062287796541));
#20275=CARTESIAN_POINT('Ctrl Pts',(75.0235448835553,1.47203780531562,45.8461386846684));
#20276=CARTESIAN_POINT('Ctrl Pts',(74.8635917035264,0.73584610333616,45.8860485896826));
#20277=CARTESIAN_POINT('Ctrl Pts',(74.8629839453475,-8.98047708566482E-5,
45.9259584946969));
#20278=CARTESIAN_POINT('Origin',(80.,0.,48.));
#20279=CARTESIAN_POINT('',(74.8634284288361,-0.000111732590146046,47.6759584946969));
#20280=CARTESIAN_POINT('',(74.8628882136866,5.62082028603397E-5,47.1990415053031));
#20281=CARTESIAN_POINT('',(74.86325,6.29070444552017E-16,48.));
#20282=CARTESIAN_POINT('Ctrl Pts',(74.8628882136866,5.62082028603397E-5,
47.1990415053031));
#20283=CARTESIAN_POINT('Ctrl Pts',(74.8628543749168,0.0593869527591274,
47.1958238167195));
#20284=CARTESIAN_POINT('Ctrl Pts',(74.863861606955,0.118716546768157,47.192606128136));
#20285=CARTESIAN_POINT('Ctrl Pts',(74.8659174321507,0.178009783776934,47.1893884395524));
#20286=CARTESIAN_POINT('Ctrl Pts',(74.895001389788,1.016836935532,47.1438674883282));
#20287=CARTESIAN_POINT('Ctrl Pts',(75.133951140809,1.8483875848139,47.0983465371041));
#20288=CARTESIAN_POINT('Ctrl Pts',(75.554614815648,2.5746925756988,47.05282558588));
#20289=CARTESIAN_POINT('Ctrl Pts',(75.975278490487,3.30099756658369,47.0073046346558));
#20290=CARTESIAN_POINT('Ctrl Pts',(76.577656089144,3.92205689907159,46.9617836834317));
#20291=CARTESIAN_POINT('Ctrl Pts',(77.2907784831134,4.36470045582208,46.9162627322075));
#20292=CARTESIAN_POINT('Ctrl Pts',(78.0039008770828,4.80734401257257,46.8707417809834));
#20293=CARTESIAN_POINT('Ctrl Pts',(78.8277680663645,5.07157179358564,46.8252208297592));
#20294=CARTESIAN_POINT('Ctrl Pts',(79.6653161220242,5.12625379770042,46.7796998785351));
#20295=CARTESIAN_POINT('Ctrl Pts',(80.5028641776839,5.18093580181521,46.734178927311));
#20296=CARTESIAN_POINT('Ctrl Pts',(81.3540930997216,5.02607202903169,46.6886579760868));
#20297=CARTESIAN_POINT('Ctrl Pts',(82.1187153361258,4.67990775775341,46.6431370248627));
#20298=CARTESIAN_POINT('Ctrl Pts',(82.8833375725299,4.33374348647512,46.5976160736385));
#20299=CARTESIAN_POINT('Ctrl Pts',(83.5613531233007,3.79627871670206,46.5520951224144));
#20300=CARTESIAN_POINT('Ctrl Pts',(84.0728815731323,3.13083487074198,46.5065741711902));
#20301=CARTESIAN_POINT('Ctrl Pts',(84.584410022964,2.4653910247819,46.4610532199661));
#20302=CARTESIAN_POINT('Ctrl Pts',(84.9294513718567,1.67196810263481,46.4155322687419));
#20303=CARTESIAN_POINT('Ctrl Pts',(85.0673545665774,0.844043241310327,46.3700113175178));
#20304=CARTESIAN_POINT('Ctrl Pts',(85.2052577612982,0.0161183799858468,
46.3244903662937));
#20305=CARTESIAN_POINT('Ctrl Pts',(85.136022801847,-0.846308420516015,46.2789694150695));
#20306=CARTESIAN_POINT('Ctrl Pts',(84.8678066063186,-1.64163032991474,46.2334484638454));
#20307=CARTESIAN_POINT('Ctrl Pts',(84.5995904107902,-2.43695223931347,46.1879275126212));
#20308=CARTESIAN_POINT('Ctrl Pts',(84.1323929791847,-3.16516925760907,46.1424065613971));
#20309=CARTESIAN_POINT('Ctrl Pts',(83.5212571859964,-3.74048648262277,46.0968856101729));
#20310=CARTESIAN_POINT('Ctrl Pts',(82.9101213928081,-4.31580370763648,46.0513646589488));
#20311=CARTESIAN_POINT('Ctrl Pts',(82.1550472380371,-4.73822113936829,46.0058437077247));
#20312=CARTESIAN_POINT('Ctrl Pts',(81.3449937979184,-4.95797165988025,45.9603227565005));
#20313=CARTESIAN_POINT('Ctrl Pts',(80.5349403577998,-5.17772218039221,45.9148018052764));
#20314=CARTESIAN_POINT('Ctrl Pts',(79.6699076323335,-5.1948057896843,45.8692808540522));
#20315=CARTESIAN_POINT('Ctrl Pts',(78.8518094689004,-5.00720978199521,45.8237599028281));
#20316=CARTESIAN_POINT('Ctrl Pts',(78.0337113054673,-4.81961377430612,45.7782389516039));
#20317=CARTESIAN_POINT('Ctrl Pts',(77.2625477040674,-4.42733814963586,45.7327180003798));
#20318=CARTESIAN_POINT('Ctrl Pts',(76.6291733194038,-3.87659886833748,45.6871970491556));
#20319=CARTESIAN_POINT('Ctrl Pts',(75.9957989347401,-3.32585958703911,45.6416760979315));
#20320=CARTESIAN_POINT('Ctrl Pts',(75.5002137668128,-2.61665664911263,45.5961551467074));
#20321=CARTESIAN_POINT('Ctrl Pts',(75.2008051918223,-1.83254481248728,45.5506341954832));
#20322=CARTESIAN_POINT('Ctrl Pts',(74.9780672965728,-1.24922344256412,45.5167699654232));
#20323=CARTESIAN_POINT('Ctrl Pts',(74.8638986774373,-0.624445521762548,
45.4829057353631));
#20324=CARTESIAN_POINT('Ctrl Pts',(74.8633066453123,0.000121786292464538,
45.4490415053031));
#20325=CARTESIAN_POINT('Ctrl Pts',(74.8629839453475,-8.98047708566482E-5,
45.9259584946969));
#20326=CARTESIAN_POINT('Ctrl Pts',(74.8628984989094,-0.103557111606977,
45.9315695409068));
#20327=CARTESIAN_POINT('Ctrl Pts',(74.8659627285546,-0.207019362333967,
45.9371805871167));
#20328=CARTESIAN_POINT('Ctrl Pts',(74.8722116978087,-0.310288900473523,
45.9427916333266));
#20329=CARTESIAN_POINT('Ctrl Pts',(74.9229079519428,-1.14808766967639,45.9883125845507));
#20330=CARTESIAN_POINT('Ctrl Pts',(75.1832127088856,-1.97320276552273,46.0338335357748));
#20331=CARTESIAN_POINT('Ctrl Pts',(75.6224581586331,-2.68842323694194,46.079354486999));
#20332=CARTESIAN_POINT('Ctrl Pts',(76.0617036083807,-3.40364370836115,46.1248754382231));
#20333=CARTESIAN_POINT('Ctrl Pts',(76.6798897509331,-4.00896955535324,46.1703963894473));
#20334=CARTESIAN_POINT('Ctrl Pts',(77.4041849738781,-4.43308430147757,46.2159173406714));
#20335=CARTESIAN_POINT('Ctrl Pts',(78.1284801968231,-4.8571990476019,46.2614382918956));
#20336=CARTESIAN_POINT('Ctrl Pts',(78.9588845001607,-5.10010269285848,46.3069592431197));
#20337=CARTESIAN_POINT('Ctrl Pts',(79.7975637847368,-5.13317753955548,46.3524801943439));
#20338=CARTESIAN_POINT('Ctrl Pts',(80.6362430693128,-5.16625238625248,46.398001145568));
#20339=CARTESIAN_POINT('Ctrl Pts',(81.4831973351274,-4.98949843438988,46.4435220967922));
#20340=CARTESIAN_POINT('Ctrl Pts',(82.2386426488751,-4.62373995424531,46.4890430480163));
#20341=CARTESIAN_POINT('Ctrl Pts',(82.9940879626228,-4.25798147410075,46.5345639992405));
#20342=CARTESIAN_POINT('Ctrl Pts',(83.6580243243037,-3.70321846567422,46.5800849504646));
#20343=CARTESIAN_POINT('Ctrl Pts',(84.1522300585487,-3.02481034359698,46.6256059016887));
#20344=CARTESIAN_POINT('Ctrl Pts',(84.6464357927938,-2.34640222151975,46.6711268529128));
#20345=CARTESIAN_POINT('Ctrl Pts',(84.970910899603,-1.54434898579181,46.716647804137));
#20346=CARTESIAN_POINT('Ctrl Pts',(85.0874273379546,-0.713144553985232,
46.7621687553611));
#20347=CARTESIAN_POINT('Ctrl Pts',(85.2039437763063,0.118059877821356,46.8076897065853));
#20348=CARTESIAN_POINT('Ctrl Pts',(85.1125015462003,0.97841550570658,46.8532106578094));
#20349=CARTESIAN_POINT('Ctrl Pts',(84.8238739157559,1.76655951463203,46.8987316090336));
#20350=CARTESIAN_POINT('Ctrl Pts',(84.5352462853114,2.55470352355748,46.9442525602577));
#20351=CARTESIAN_POINT('Ctrl Pts',(84.0494332545284,3.27063591352315,46.9897735114819));
#20352=CARTESIAN_POINT('Ctrl Pts',(83.4236708950806,3.83000909607603,47.035294462706));
#20353=CARTESIAN_POINT('Ctrl Pts',(82.7979085356327,4.3893822786289,47.0808154139302));
#20354=CARTESIAN_POINT('Ctrl Pts',(82.0321968475201,4.79219625376898,47.1263363651543));
#20355=CARTESIAN_POINT('Ctrl Pts',(81.2167481681753,4.99099348517798,47.1718573163784));
#20356=CARTESIAN_POINT('Ctrl Pts',(80.4012994888305,5.18979071658698,47.2173782676026));
#20357=CARTESIAN_POINT('Ctrl Pts',(79.5361138182536,5.18457120426489,47.2628992188267));
#20358=CARTESIAN_POINT('Ctrl Pts',(78.7231230230567,4.9759498851575,47.3084201700509));
#20359=CARTESIAN_POINT('Ctrl Pts',(77.9101322278597,4.76732856605011,47.353941121275));
#20360=CARTESIAN_POINT('Ctrl Pts',(77.1493363080427,4.35530544015742,47.3994620724991));
#20361=CARTESIAN_POINT('Ctrl Pts',(76.5303684497011,3.7884230200728,47.4449830237233));
#20362=CARTESIAN_POINT('Ctrl Pts',(75.9114005913594,3.22154059998819,47.4905039749474));
#20363=CARTESIAN_POINT('Ctrl Pts',(75.4342607944931,2.49979888571167,47.5360249261716));
#20364=CARTESIAN_POINT('Ctrl Pts',(75.1551632935531,1.70822989135296,47.5815458773957));
#20365=CARTESIAN_POINT('Ctrl Pts',(74.9622094643284,1.16097931389284,47.6130167498295));
#20366=CARTESIAN_POINT('Ctrl Pts',(74.8639126621751,0.580353831793524,47.6444876222632));
#20367=CARTESIAN_POINT('Ctrl Pts',(74.8634284288361,-0.000111732590146046,
47.6759584946969));
#20368=CARTESIAN_POINT('Origin',(80.,0.,48.));
#20369=CARTESIAN_POINT('',(74.8636526568313,-4.35339233453846E-6,49.4259584946969));
#20370=CARTESIAN_POINT('',(74.8629661957176,-8.50189945436741E-5,48.9490415053031));
#20371=CARTESIAN_POINT('',(74.86325,6.29070444552017E-16,48.));
#20372=CARTESIAN_POINT('Ctrl Pts',(74.8629661957176,-8.50189945436741E-5,
48.9490415053031));
#20373=CARTESIAN_POINT('Ctrl Pts',(74.8635556721698,0.743029487008711,48.9087418980759));
#20374=CARTESIAN_POINT('Ctrl Pts',(75.0267457376609,1.48639459196899,48.8684422908488));
#20375=CARTESIAN_POINT('Ctrl Pts',(75.3392541588398,2.1605414832218,48.8281426836216));
#20376=CARTESIAN_POINT('Ctrl Pts',(75.6922521550092,2.92203296827837,48.7826217323974));
#20377=CARTESIAN_POINT('Ctrl Pts',(76.2357673683812,3.59520804109921,48.7371007811733));
#20378=CARTESIAN_POINT('Ctrl Pts',(76.9057655435175,4.10075656738261,48.6915798299491));
#20379=CARTESIAN_POINT('Ctrl Pts',(77.5757637186539,4.60630509366602,48.646058878725));
#20380=CARTESIAN_POINT('Ctrl Pts',(78.3722448555547,4.94422707341198,48.6005379275009));
#20381=CARTESIAN_POINT('Ctrl Pts',(79.2013715135795,5.0747102220021,48.5550169762767));
#20382=CARTESIAN_POINT('Ctrl Pts',(80.0304981716043,5.20519337059221,48.5094960250526));
#20383=CARTESIAN_POINT('Ctrl Pts',(80.8922703507531,5.12823768802648,48.4639750738284));
#20384=CARTESIAN_POINT('Ctrl Pts',(81.6851583449729,4.85290970954365,48.4184541226043));
#20385=CARTESIAN_POINT('Ctrl Pts',(82.4780463391927,4.57758173106082,48.3729331713801));
#20386=CARTESIAN_POINT('Ctrl Pts',(83.2020501484835,4.1038814566609,48.327412220156));
#20387=CARTESIAN_POINT('Ctrl Pts',(83.7718712499674,3.48761789338864,48.2818912689318));
#20388=CARTESIAN_POINT('Ctrl Pts',(84.3416923514512,2.87135433011637,48.2363703177077));
#20389=CARTESIAN_POINT('Ctrl Pts',(84.7573307451282,2.11252747797175,48.1908493664835));
#20390=CARTESIAN_POINT('Ctrl Pts',(84.9698179855606,1.30053853730398,48.1453284152594));
#20391=CARTESIAN_POINT('Ctrl Pts',(85.182305225993,0.488549596636203,48.0998074640352));
#20392=CARTESIAN_POINT('Ctrl Pts',(85.1916413131808,-0.376601432554719,
48.0542865128111));
#20393=CARTESIAN_POINT('Ctrl Pts',(84.9967263158304,-1.19298676493227,48.008765561587));
#20394=CARTESIAN_POINT('Ctrl Pts',(84.8018113184798,-2.00937209730982,47.9632446103628));
#20395=CARTESIAN_POINT('Ctrl Pts',(84.4026452365911,-2.77699173287399,47.9177236591387));
#20396=CARTESIAN_POINT('Ctrl Pts',(83.8462558298679,-3.40540854932594,47.8722027079145));
#20397=CARTESIAN_POINT('Ctrl Pts',(83.2898664231448,-4.03382536577789,47.8266817566904));
#20398=CARTESIAN_POINT('Ctrl Pts',(82.5762536915873,-4.52303936311763,47.7811608054663));
#20399=CARTESIAN_POINT('Ctrl Pts',(81.7894919330479,-4.8154137847304,47.7356398542421));
#20400=CARTESIAN_POINT('Ctrl Pts',(81.0027301745085,-5.10778820634318,47.690118903018));
#20401=CARTESIAN_POINT('Ctrl Pts',(80.1428193889873,-5.20332305222899,47.6445979517938));
#20402=CARTESIAN_POINT('Ctrl Pts',(79.3110699824109,-5.09076288266106,47.5990770005697));
#20403=CARTESIAN_POINT('Ctrl Pts',(78.4793205758345,-4.97820271309314,47.5535560493455));
#20404=CARTESIAN_POINT('Ctrl Pts',(77.6757325482029,-4.65754752807148,47.5080350981214));
#20405=CARTESIAN_POINT('Ctrl Pts',(76.9949806386261,-4.1665753244581,47.4625141468972));
#20406=CARTESIAN_POINT('Ctrl Pts',(76.3142287290494,-3.67560312084472,47.4169931956731));
#20407=CARTESIAN_POINT('Ctrl Pts',(75.7563129375275,-3.01431389863962,47.371472244449));
#20408=CARTESIAN_POINT('Ctrl Pts',(75.3869641238935,-2.26061746042296,47.3259512932248));
#20409=CARTESIAN_POINT('Ctrl Pts',(75.043723056891,-1.56019671964928,47.2836480305843));
#20410=CARTESIAN_POINT('Ctrl Pts',(74.8633330952622,-0.779970821893516,
47.2413447679437));
#20411=CARTESIAN_POINT('Ctrl Pts',(74.8628882136866,5.62082028603397E-5,
47.1990415053031));
#20412=CARTESIAN_POINT('Ctrl Pts',(74.8634284288361,-0.000111732590146046,
47.6759584946969));
#20413=CARTESIAN_POINT('Ctrl Pts',(74.8632122442806,-0.259258883083046,
47.6900085734873));
#20414=CARTESIAN_POINT('Ctrl Pts',(74.8824915705452,-0.518374159578633,
47.7040586522777));
#20415=CARTESIAN_POINT('Ctrl Pts',(74.9215471990678,-0.774473513137255,
47.7181087310682));
#20416=CARTESIAN_POINT('Ctrl Pts',(75.0480838105362,-1.60421164882776,47.7636296822923));
#20417=CARTESIAN_POINT('Ctrl Pts',(75.3822122384867,-2.40229164576784,47.8091506335165));
#20418=CARTESIAN_POINT('Ctrl Pts',(75.8845671356794,-3.07468769359052,47.8546715847406));
#20419=CARTESIAN_POINT('Ctrl Pts',(76.3869220328721,-3.74708374141319,47.9001925359648));
#20420=CARTESIAN_POINT('Ctrl Pts',(77.0575033993071,-4.29379584011847,47.9457134871889));
#20421=CARTESIAN_POINT('Ctrl Pts',(77.8173066782509,-4.65041309316053,47.991234438413));
#20422=CARTESIAN_POINT('Ctrl Pts',(78.5771099571947,-5.00703034620259,48.0367553896372));
#20423=CARTESIAN_POINT('Ctrl Pts',(79.4261351486474,-5.17355275358143,48.0822763408613));
#20424=CARTESIAN_POINT('Ctrl Pts',(80.2643543331593,-5.13036147463186,48.1277972920855));
#20425=CARTESIAN_POINT('Ctrl Pts',(81.1025735176711,-5.0871701956823,48.1733182433096));
#20426=CARTESIAN_POINT('Ctrl Pts',(81.9299866952422,-4.8342652304043,48.2188391945338));
#20427=CARTESIAN_POINT('Ctrl Pts',(82.6491121662587,-4.40144258220266,48.2643601457579));
#20428=CARTESIAN_POINT('Ctrl Pts',(83.3682376372753,-3.96861993400101,48.309881096982));
#20429=CARTESIAN_POINT('Ctrl Pts',(83.9790754017373,-3.35587960287571,48.3554020482062));
#20430=CARTESIAN_POINT('Ctrl Pts',(84.4096595965402,-2.63541160285976,48.4009229994303));
#20431=CARTESIAN_POINT('Ctrl Pts',(84.8402437913431,-1.91494360284381,48.4464439506545));
#20432=CARTESIAN_POINT('Ctrl Pts',(85.090574416487,-1.08674793393721,48.4919649018786));
#20433=CARTESIAN_POINT('Ctrl Pts',(85.1311587644999,-0.248398484985625,
48.5374858531028));
#20434=CARTESIAN_POINT('Ctrl Pts',(85.1717431125128,0.589950963965957,48.5830068043269));
#20435=CARTESIAN_POINT('Ctrl Pts',(85.0025811833949,1.43845419296252,48.628527755551));
#20436=CARTESIAN_POINT('Ctrl Pts',(84.6436027931163,2.19714477757134,48.6740487067752));
#20437=CARTESIAN_POINT('Ctrl Pts',(84.2846244028378,2.95583536218017,48.7195696579993));
#20438=CARTESIAN_POINT('Ctrl Pts',(83.7358295513987,3.62471330240126,48.7650906092235));
#20439=CARTESIAN_POINT('Ctrl Pts',(83.0618745148986,4.12497473069372,48.8106115604476));
#20440=CARTESIAN_POINT('Ctrl Pts',(82.3879194783985,4.62523615898618,48.8561325116718));
#20441=CARTESIAN_POINT('Ctrl Pts',(81.5888042568375,4.95688107535002,48.9016534628959));
#20442=CARTESIAN_POINT('Ctrl Pts',(80.7586766255913,5.08083672751136,48.9471744141201));
#20443=CARTESIAN_POINT('Ctrl Pts',(79.9285489943452,5.20479237967269,48.9926953653442));
#20444=CARTESIAN_POINT('Ctrl Pts',(79.067408953414,5.12105876763151,49.0382163165683));
#20445=CARTESIAN_POINT('Ctrl Pts',(78.2767117334743,4.83950096851957,49.0837372677925));
#20446=CARTESIAN_POINT('Ctrl Pts',(77.4860145135347,4.55794316940763,49.1292582190166));
#20447=CARTESIAN_POINT('Ctrl Pts',(76.7657601145866,4.07856118322493,49.1747791702408));
#20448=CARTESIAN_POINT('Ctrl Pts',(76.2008053226555,3.45783340800046,49.2203001214649));
#20449=CARTESIAN_POINT('Ctrl Pts',(75.6358505307244,2.83710563277598,49.2658210726891));
#20450=CARTESIAN_POINT('Ctrl Pts',(75.2261953458102,2.07503206850973,49.3113420239132));
#20451=CARTESIAN_POINT('Ctrl Pts',(75.0201033014939,1.26139642700268,49.3568629751374));
#20452=CARTESIAN_POINT('Ctrl Pts',(74.9158287019511,0.849728276621614,49.3798948149905));
#20453=CARTESIAN_POINT('Ctrl Pts',(74.8636656234315,0.424860397329693,49.4029266548437));
#20454=CARTESIAN_POINT('Ctrl Pts',(74.8636526568313,-4.35339233453846E-6,
49.4259584946969));
#20455=CARTESIAN_POINT('Origin',(80.,0.,48.));
#20456=CARTESIAN_POINT('',(74.8634535980369,0.000107814451578703,51.1759584946969));
#20457=CARTESIAN_POINT('',(74.863409785596,-0.000114188402419197,50.6990415053031));
#20458=CARTESIAN_POINT('',(74.86325,6.29070444552017E-16,48.));
#20459=CARTESIAN_POINT('Ctrl Pts',(74.863409785596,-0.000114188402419197,
50.6990415053031));
#20460=CARTESIAN_POINT('Ctrl Pts',(74.8639137889733,0.587533088950244,50.6671809306565));
#20461=CARTESIAN_POINT('Ctrl Pts',(74.9647094137452,1.17534890055812,50.6353203560098));
#20462=CARTESIAN_POINT('Ctrl Pts',(75.1623764068138,1.72855120469804,50.6034597813632));
#20463=CARTESIAN_POINT('Ctrl Pts',(75.4447940860268,2.51894169147106,50.557938830139));
#20464=CARTESIAN_POINT('Ctrl Pts',(75.9249592108754,3.23867422423114,50.5124178789149));
#20465=CARTESIAN_POINT('Ctrl Pts',(76.5463011178337,3.80295350062791,50.4668969276907));
#20466=CARTESIAN_POINT('Ctrl Pts',(77.1676430247919,4.36723277702467,50.4213759764666));
#20467=CARTESIAN_POINT('Ctrl Pts',(77.9301617138597,4.77605879705811,50.3758550252424));
#20468=CARTESIAN_POINT('Ctrl Pts',(78.744021030849,4.98126571522392,50.3303340740183));
#20469=CARTESIAN_POINT('Ctrl Pts',(79.5578803478383,5.18647263338972,50.2848131227942));
#20470=CARTESIAN_POINT('Ctrl Pts',(80.4230802927489,5.18806044968789,50.23929217157));
#20471=CARTESIAN_POINT('Ctrl Pts',(81.2376873172381,4.98584209551033,50.1937712203459));
#20472=CARTESIAN_POINT('Ctrl Pts',(82.0522943417272,4.78362374133277,50.1482502691217));
#20473=CARTESIAN_POINT('Ctrl Pts',(82.8163084457949,4.37759921667948,50.1027293178976));
#20474=CARTESIAN_POINT('Ctrl Pts',(83.4397172929055,3.81560430882212,50.0572083666734));
#20475=CARTESIAN_POINT('Ctrl Pts',(84.0631261400161,3.25360940096478,50.0116874154493));
#20476=CARTESIAN_POINT('Ctrl Pts',(84.5459297301697,2.53564410990337,49.9661664642252));
#20477=CARTESIAN_POINT('Ctrl Pts',(84.8312465489989,1.74629553037307,49.920645513001));
#20478=CARTESIAN_POINT('Ctrl Pts',(85.1165633678282,0.956946950842764,49.8751245617768));
#20479=CARTESIAN_POINT('Ctrl Pts',(85.204393415333,0.0962150828435583,49.8296036105527));
#20480=CARTESIAN_POINT('Ctrl Pts',(85.0843889927579,-0.734492931849786,
49.7840826593286));
#20481=CARTESIAN_POINT('Ctrl Pts',(84.9643845701827,-1.56520094654313,49.7385617081044));
#20482=CARTESIAN_POINT('Ctrl Pts',(84.6365456775277,-2.36588510793061,49.6930407568803));
#20483=CARTESIAN_POINT('Ctrl Pts',(84.1394966603092,-3.04221279596022,49.6475198056562));
#20484=CARTESIAN_POINT('Ctrl Pts',(83.6424476430907,-3.71854048398984,49.601998854432));
#20485=CARTESIAN_POINT('Ctrl Pts',(82.9761885013088,-4.27051169866158,49.5564779032079));
#20486=CARTESIAN_POINT('Ctrl Pts',(82.2192145687153,-4.63309594057973,49.5109569519837));
#20487=CARTESIAN_POINT('Ctrl Pts',(81.4622406361219,-4.99568018249788,49.4654360007596));
#20488=CARTESIAN_POINT('Ctrl Pts',(80.6145519127169,-5.16887745166244,49.4199150495354));
#20489=CARTESIAN_POINT('Ctrl Pts',(79.7760188619409,-5.13228250843703,49.3743940983113));
#20490=CARTESIAN_POINT('Ctrl Pts',(78.9374858111649,-5.09568756521162,49.3288731470871));
#20491=CARTESIAN_POINT('Ctrl Pts',(78.108108433018,-4.84930040959626,49.283352195863));
#20492=CARTESIAN_POINT('Ctrl Pts',(77.3855998394428,-4.42214914912349,49.2378312446389));
#20493=CARTESIAN_POINT('Ctrl Pts',(76.6630912458677,-3.99499788865072,49.1923102934147));
#20494=CARTESIAN_POINT('Ctrl Pts',(76.0474514368645,-3.38708252332054,49.1467893421906));
#20495=CARTESIAN_POINT('Ctrl Pts',(75.6112120285087,-2.67002461372696,49.1012683909664));
#20496=CARTESIAN_POINT('Ctrl Pts',(75.1749726201528,-1.95296670413337,49.0557474397423));
#20497=CARTESIAN_POINT('Ctrl Pts',(74.9181336124445,-1.12676625027638,49.0102264885181));
#20498=CARTESIAN_POINT('Ctrl Pts',(74.8709544980738,-0.288762074701733,
48.964705537294));
#20499=CARTESIAN_POINT('Ctrl Pts',(74.8655429594531,-0.192641322522879,
48.959484193297));
#20500=CARTESIAN_POINT('Ctrl Pts',(74.8628898212925,-0.0963652741121222,
48.9542628493001));
#20501=CARTESIAN_POINT('Ctrl Pts',(74.8629661957176,-8.50189945436741E-5,
48.9490415053031));
#20502=CARTESIAN_POINT('Ctrl Pts',(74.8636526568313,-4.35339233453846E-6,
49.4259584946969));
#20503=CARTESIAN_POINT('Ctrl Pts',(74.8636399957796,-0.414857476611885,
49.4484476060679));
#20504=CARTESIAN_POINT('Ctrl Pts',(74.9133486457029,-0.829707616969254,
49.4709367174388));
#20505=CARTESIAN_POINT('Ctrl Pts',(75.0128145331795,-1.23226344317328,49.4934258288098));
#20506=CARTESIAN_POINT('Ctrl Pts',(75.2141467128998,-2.04708995309434,49.5389467800339));
#20507=CARTESIAN_POINT('Ctrl Pts',(75.6193399760587,-2.81154525418862,49.5844677312581));
#20508=CARTESIAN_POINT('Ctrl Pts',(76.1806564704738,-3.43556503028439,49.6299886824822));
#20509=CARTESIAN_POINT('Ctrl Pts',(76.7419729648888,-4.05958480638017,49.6755096337063));
#20510=CARTESIAN_POINT('Ctrl Pts',(77.45941269056,-4.54316905747744,49.7210305849305));
#20511=CARTESIAN_POINT('Ctrl Pts',(78.2484504722489,-4.82934429562459,49.7665515361546));
#20512=CARTESIAN_POINT('Ctrl Pts',(79.0374882539378,-5.11551953377174,49.8120724873788));
#20513=CARTESIAN_POINT('Ctrl Pts',(79.8981240916443,-5.20428575896875,49.8575934386029));
#20514=CARTESIAN_POINT('Ctrl Pts',(80.7289621574045,-5.08518497666695,49.9031143898271));
#20515=CARTESIAN_POINT('Ctrl Pts',(81.5598002231647,-4.96608419436515,49.9486353410512));
#20516=CARTESIAN_POINT('Ctrl Pts',(82.3608405169786,-4.63911640456454,49.9941562922754));
#20517=CARTESIAN_POINT('Ctrl Pts',(83.0377084610454,-4.1428033237821,50.0396772434995));
#20518=CARTESIAN_POINT('Ctrl Pts',(83.7145764051122,-3.64649024299964,50.0851981947237));
#20519=CARTESIAN_POINT('Ctrl Pts',(84.267271999432,-2.98083187123535,50.1307191459478));
#20520=CARTESIAN_POINT('Ctrl Pts',(84.6306794018067,-2.22425276250945,50.1762400971719));
#20521=CARTESIAN_POINT('Ctrl Pts',(84.9940868041813,-1.46767365378356,50.2217610483961));
#20522=CARTESIAN_POINT('Ctrl Pts',(85.1682060146108,-0.620173808096055,
50.2672819996202));
#20523=CARTESIAN_POINT('Ctrl Pts',(85.1325231749308,0.218398563743828,50.3128029508444));
#20524=CARTESIAN_POINT('Ctrl Pts',(85.0968403352507,1.05697093558372,50.3583239020685));
#20525=CARTESIAN_POINT('Ctrl Pts',(84.8513554454613,1.88661583357599,50.4038448532927));
#20526=CARTESIAN_POINT('Ctrl Pts',(84.4249903126289,2.60958862792328,50.4493658045168));
#20527=CARTESIAN_POINT('Ctrl Pts',(83.9986251797964,3.33256142227058,50.494886755741));
#20528=CARTESIAN_POINT('Ctrl Pts',(83.3913798039212,3.94886211297289,50.5404077069651));
#20529=CARTESIAN_POINT('Ctrl Pts',(82.6747968107765,4.38588122216179,50.5859286581892));
#20530=CARTESIAN_POINT('Ctrl Pts',(81.9582138176319,4.82290033135069,50.6314496094134));
#20531=CARTESIAN_POINT('Ctrl Pts',(81.1322932072179,5.08063785902618,50.6769705606375));
#20532=CARTESIAN_POINT('Ctrl Pts',(80.2943408323192,5.12872845335609,50.7224915118616));
#20533=CARTESIAN_POINT('Ctrl Pts',(79.4563884574205,5.17681904768601,50.7680124630858));
#20534=CARTESIAN_POINT('Ctrl Pts',(78.606404318037,5.01526270867036,50.8135334143099));
#20535=CARTESIAN_POINT('Ctrl Pts',(77.8445293120887,4.66309319952182,50.8590543655341));
#20536=CARTESIAN_POINT('Ctrl Pts',(77.0826543061403,4.31092369037328,50.9045753167582));
#20537=CARTESIAN_POINT('Ctrl Pts',(76.408888433627,3.76814101109185,50.9500962679824));
#20538=CARTESIAN_POINT('Ctrl Pts',(75.9026114339255,3.09869311362241,50.9956172192065));
#20539=CARTESIAN_POINT('Ctrl Pts',(75.396334434224,2.42924521615298,51.0411381704307));
#20540=CARTESIAN_POINT('Ctrl Pts',(75.0575463073343,1.63313210049556,51.0866591216548));
#20541=CARTESIAN_POINT('Ctrl Pts',(74.9261613830222,0.804147848807305,51.1321800728789));
#20542=CARTESIAN_POINT('Ctrl Pts',(74.8840428677571,0.538397527435993,51.1467728801516));
#20543=CARTESIAN_POINT('Ctrl Pts',(74.8632386240357,0.269269127468966,51.1613656874243));
#20544=CARTESIAN_POINT('Ctrl Pts',(74.8634535980369,0.000107814451578703,
51.1759584946969));
#20545=CARTESIAN_POINT('Origin',(80.,0.,48.));
#20546=CARTESIAN_POINT('',(74.8630099039127,9.58920879684522E-5,52.9259584946969));
#20547=CARTESIAN_POINT('',(74.8636515713633,-1.05953972605244E-5,52.4490415053031));
#20548=CARTESIAN_POINT('',(74.86325,6.29070444552017E-16,48.));
#20549=CARTESIAN_POINT('',(83.8799476118145,3.36633437021263,54.));
#20550=CARTESIAN_POINT('Ctrl Pts',(74.8630099039127,9.58920879684522E-5,
52.9259584946969));
#20551=CARTESIAN_POINT('Ctrl Pts',(74.8636382796423,-0.725842401654488,
52.9653256712289));
#20552=CARTESIAN_POINT('Ctrl Pts',(75.0191418658014,-1.45204116294986,53.0046928477609));
#20553=CARTESIAN_POINT('Ctrl Pts',(75.3177903450041,-2.11362325386402,53.044060024293));
#20554=CARTESIAN_POINT('Ctrl Pts',(75.6631227780752,-2.878622137306,53.0895809755171));
#20555=CARTESIAN_POINT('Ctrl Pts',(76.1998499432974,-3.55722401379127,53.1351019267413));
#20556=CARTESIAN_POINT('Ctrl Pts',(76.8647368947113,-4.06947479034707,53.1806228779654));
#20557=CARTESIAN_POINT('Ctrl Pts',(77.5296238461253,-4.58172556690286,53.2261438291896));
#20558=CARTESIAN_POINT('Ctrl Pts',(78.3226705837311,-4.92762524352918,53.2716647804137));
#20559=CARTESIAN_POINT('Ctrl Pts',(79.1504451677981,-5.06643148578586,53.3171857316378));
#20560=CARTESIAN_POINT('Ctrl Pts',(79.9782197518651,-5.20523772804254,53.362706682862));
#20561=CARTESIAN_POINT('Ctrl Pts',(80.8407221823932,-5.13695053592958,53.4082276340861));
#20562=CARTESIAN_POINT('Ctrl Pts',(81.6363346794966,-4.86959432823606,53.4537485853103));
#20563=CARTESIAN_POINT('Ctrl Pts',(82.4319471766,-4.60223812054255,53.4992695365344));
#20564=CARTESIAN_POINT('Ctrl Pts',(83.1606697402787,-4.13581289726848,53.5447904877586));
#20565=CARTESIAN_POINT('Ctrl Pts',(83.7366512624658,-3.52531601118724,53.5903114389827));
#20566=CARTESIAN_POINT('Ctrl Pts',(84.312632784653,-2.914819125106,53.6358323902068));
#20567=CARTESIAN_POINT('Ctrl Pts',(84.7358732653486,-2.16025057621758,53.681353341431));
#20568=CARTESIAN_POINT('Ctrl Pts',(84.9564959299256,-1.35041792168183,53.7268742926551));
#20569=CARTESIAN_POINT('Ctrl Pts',(85.1771185945027,-0.540585267146073,
53.7723952438793));
#20570=CARTESIAN_POINT('Ctrl Pts',(85.1951234429612,0.324511493037019,53.8179161951034));
#20571=CARTESIAN_POINT('Ctrl Pts',(85.0083774710662,1.14270864307895,53.8634371463276));
#20572=CARTESIAN_POINT('Ctrl Pts',(84.821631499171,1.96090579312088,53.9089580975517));
#20573=CARTESIAN_POINT('Ctrl Pts',(84.4301347069223,2.73220333302164,53.9544790487759));
#20574=CARTESIAN_POINT('Ctrl Pts',(83.8799476118145,3.36633437021264,54.));
#20575=CARTESIAN_POINT('',(76.1197954215944,3.36643663068927,54.));
#20576=CARTESIAN_POINT('Origin',(80.,0.,54.));
#20577=CARTESIAN_POINT('Ctrl Pts',(76.1197954215944,3.36643663068927,54.));
#20578=CARTESIAN_POINT('Ctrl Pts',(76.5997425438788,3.91867143724511,53.9603227565005));
#20579=CARTESIAN_POINT('Ctrl Pts',(77.198769156323,4.36792997703869,53.920645513001));
#20580=CARTESIAN_POINT('Ctrl Pts',(77.8641232237026,4.67209812654765,53.8809682695015));
#20581=CARTESIAN_POINT('Ctrl Pts',(78.6274713642647,5.02106449307235,53.8354473182774));
#20582=CARTESIAN_POINT('Ctrl Pts',(79.478123276234,5.17905506715725,53.7899263670532));
#20583=CARTESIAN_POINT('Ctrl Pts',(80.315865632671,5.12744848588364,53.7444054158291));
#20584=CARTESIAN_POINT('Ctrl Pts',(81.1536079891079,5.07584190461002,53.6988844646049));
#20585=CARTESIAN_POINT('Ctrl Pts',(81.9784407900124,4.81463816797789,53.6533635133808));
#20586=CARTESIAN_POINT('Ctrl Pts',(82.693183411522,4.37461459180461,53.6078425621567));
#20587=CARTESIAN_POINT('Ctrl Pts',(83.4079260330316,3.93459101563133,53.5623216109325));
#20588=CARTESIAN_POINT('Ctrl Pts',(84.0125784751463,3.31574759991691,53.5168006597084));
#20589=CARTESIAN_POINT('Ctrl Pts',(84.4359049723902,2.59099170638668,53.4712797084842));
#20590=CARTESIAN_POINT('Ctrl Pts',(84.8592314696341,1.86623581285645,53.4257587572601));
#20591=CARTESIAN_POINT('Ctrl Pts',(85.1012320220073,1.03556744151041,53.3802378060359));
#20592=CARTESIAN_POINT('Ctrl Pts',(85.1333946855385,0.196852593275327,53.3347168548118));
#20593=CARTESIAN_POINT('Ctrl Pts',(85.1655573490699,-0.641862254959766,
53.2891959035876));
#20594=CARTESIAN_POINT('Ctrl Pts',(84.9878821237593,-1.48862358008391,53.2436749523635));
#20595=CARTESIAN_POINT('Ctrl Pts',(84.6213021217404,-2.24367055085715,53.1981540011394));
#20596=CARTESIAN_POINT('Ctrl Pts',(84.2547221197216,-2.9987175216304,53.1526330499152));
#20597=CARTESIAN_POINT('Ctrl Pts',(83.6992373409944,-3.66205013805274,53.1071120986911));
#20598=CARTESIAN_POINT('Ctrl Pts',(83.0202920939743,-4.15551768120208,53.0615911474669));
#20599=CARTESIAN_POINT('Ctrl Pts',(82.3413468469542,-4.6489852243514,53.0160701962428));
#20600=CARTESIAN_POINT('Ctrl Pts',(81.5389411316412,-4.97258769422772,52.9705492450186));
#20601=CARTESIAN_POINT('Ctrl Pts',(80.7076104593837,-5.08819994104047,52.9250282937945));
#20602=CARTESIAN_POINT('Ctrl Pts',(79.8762797871261,-5.20381218785322,52.8795073425703));
#20603=CARTESIAN_POINT('Ctrl Pts',(79.0160241579242,-5.1114342116024,52.8339863913462));
#20604=CARTESIAN_POINT('Ctrl Pts',(78.2281945743439,-4.82194948714952,52.7884654401221));
#20605=CARTESIAN_POINT('Ctrl Pts',(77.4403649907635,-4.53246476269664,52.7429444888979));
#20606=CARTESIAN_POINT('Ctrl Pts',(76.7249614528048,-4.04587329004171,52.6974235376738));
#20607=CARTESIAN_POINT('Ctrl Pts',(76.1662692568043,-3.41950287091639,52.6519025864496));
#20608=CARTESIAN_POINT('Ctrl Pts',(75.6075770608038,-2.79313245179107,52.6063816352255));
#20609=CARTESIAN_POINT('Ctrl Pts',(75.2055962067615,-2.02698308619534,52.5608606840013));
#20610=CARTESIAN_POINT('Ctrl Pts',(75.0076860699755,-1.21131866814437,52.5153397327772));
#20611=CARTESIAN_POINT('Ctrl Pts',(74.9116051012844,-0.815331738490969,
52.4932403236192));
#20612=CARTESIAN_POINT('Ctrl Pts',(74.8636212843626,-0.407674672990421,
52.4711409144611));
#20613=CARTESIAN_POINT('Ctrl Pts',(74.8636515713633,-1.05953972605244E-5,
52.4490415053031));
#20614=CARTESIAN_POINT('Origin',(80.,0.,57.8647410325605));
#20615=CARTESIAN_POINT('',(73.8872027408445,4.9881108922234E-5,43.1352589674395));
#20616=CARTESIAN_POINT('',(73.8867924003229,0.000144735339684834,42.9897410325605));
#20617=CARTESIAN_POINT('',(73.88675,2.47426426879123E-14,57.8647410325605));
#20618=CARTESIAN_POINT('',(85.6017891526601,-2.44781205398602,42.));
#20619=CARTESIAN_POINT('Ctrl Pts',(73.8867924003229,0.00014473533968537,
42.9897410325605));
#20620=CARTESIAN_POINT('Ctrl Pts',(73.8865552402621,0.247445601036081,42.9784740136094));
#20621=CARTESIAN_POINT('Ctrl Pts',(73.9608139639282,1.49374897980165,42.9216860434341));
#20622=CARTESIAN_POINT('Ctrl Pts',(74.7901455575896,3.65425999548639,42.8193771220346));
#20623=CARTESIAN_POINT('Ctrl Pts',(77.1247475918389,5.6770538401786,42.6828142683621));
#20624=CARTESIAN_POINT('Ctrl Pts',(80.1368351706977,6.36221026869802,42.5462514146897));
#20625=CARTESIAN_POINT('Ctrl Pts',(83.1167004331651,5.54813947205128,42.4096885610173));
#20626=CARTESIAN_POINT('Ctrl Pts',(85.3621237298141,3.42697795347734,42.2731257073449));
#20627=CARTESIAN_POINT('Ctrl Pts',(86.3441251020869,0.497881335996617,42.1365628536724));
#20628=CARTESIAN_POINT('Ctrl Pts',(86.0018547597101,-1.53226660829892,42.0455209512241));
#20629=CARTESIAN_POINT('Ctrl Pts',(85.6017891526601,-2.4478120539861,42.));
#20630=CARTESIAN_POINT('',(83.6329556492824,-4.91665117868322,42.));
#20631=CARTESIAN_POINT('Origin',(80.,0.,42.));
#20632=CARTESIAN_POINT('Ctrl Pts',(73.8872027408445,4.98811089222687E-5,
43.1352589674395));
#20633=CARTESIAN_POINT('Ctrl Pts',(73.8870723527698,0.441218568097294,43.1151632136948));
#20634=CARTESIAN_POINT('Ctrl Pts',(74.0409887873294,1.88163402125046,43.049546508726));
#20635=CARTESIAN_POINT('Ctrl Pts',(75.1606667541984,4.13243333827823,42.9384088525331));
#20636=CARTESIAN_POINT('Ctrl Pts',(77.6767884766317,5.92442701100857,42.8018459988606));
#20637=CARTESIAN_POINT('Ctrl Pts',(80.7403278321772,6.32044846892683,42.6652831451882));
#20638=CARTESIAN_POINT('Ctrl Pts',(83.6294253939595,5.22718080357853,42.5287202915158));
#20639=CARTESIAN_POINT('Ctrl Pts',(85.6633177227071,2.90223574469819,42.3921574378434));
#20640=CARTESIAN_POINT('Ctrl Pts',(86.3627699345494,-0.106570534545254,
42.2555945841709));
#20641=CARTESIAN_POINT('Ctrl Pts',(85.5971716734128,-2.96257437178865,42.1248754382231));
#20642=CARTESIAN_POINT('Ctrl Pts',(84.3329182412889,-4.39891812993667,42.0396772434995));
#20643=CARTESIAN_POINT('Ctrl Pts',(83.6330530644635,-4.91696557452334,42.));
#20644=CARTESIAN_POINT('Origin',(80.,0.,57.8647410325605));
#20645=CARTESIAN_POINT('',(73.8868174136284,0.000144937957391733,44.8852589674395));
#20646=CARTESIAN_POINT('',(73.8863051433301,5.93870499029922E-5,44.7397410325605));
#20647=CARTESIAN_POINT('',(73.88675,2.47426426879123E-14,57.8647410325605));
#20648=CARTESIAN_POINT('Ctrl Pts',(73.8863051433301,5.93870499033134E-5,
44.7397410325605));
#20649=CARTESIAN_POINT('Ctrl Pts',(73.8862731401809,0.0621168333236095,
44.7369130461899));
#20650=CARTESIAN_POINT('Ctrl Pts',(73.9021026716431,1.12307150188376,44.6885641085951));
#20651=CARTESIAN_POINT('Ctrl Pts',(74.4799467231356,3.16625379319216,44.5946942197762));
#20652=CARTESIAN_POINT('Ctrl Pts',(76.621290400294,5.39263133473806,44.4581313661038));
#20653=CARTESIAN_POINT('Ctrl Pts',(79.5587595524336,6.34834294257372,44.3215685124313));
#20654=CARTESIAN_POINT('Ctrl Pts',(82.6001982072725,5.80819426108823,44.1850056587589));
#20655=CARTESIAN_POINT('Ctrl Pts',(85.0289520597644,3.89946052862007,44.0484428050865));
#20656=CARTESIAN_POINT('Ctrl Pts',(86.272733737581,1.07189678402622,43.911879951414));
#20657=CARTESIAN_POINT('Ctrl Pts',(86.0384709317063,-2.00823809264104,43.7753170977416));
#20658=CARTESIAN_POINT('Ctrl Pts',(84.3813629617958,-4.61517164026814,43.6387542440692));
#20659=CARTESIAN_POINT('Ctrl Pts',(81.6918743166977,-6.13463234755794,43.5021913903967));
#20660=CARTESIAN_POINT('Ctrl Pts',(78.6037291538527,-6.20858889925048,43.3656285367243));
#20661=CARTESIAN_POINT('Ctrl Pts',(75.8445875723747,-4.81961646710041,43.2290656830519));
#20662=CARTESIAN_POINT('Ctrl Pts',(74.211443274136,-2.50328738630905,43.1037698483306));
#20663=CARTESIAN_POINT('Ctrl Pts',(73.8875134131035,-0.75169806720796,43.0239949648335));
#20664=CARTESIAN_POINT('Ctrl Pts',(73.8867924003229,0.00014473533968537,
42.9897410325605));
#20665=CARTESIAN_POINT('Ctrl Pts',(73.8868174136284,0.000144937957391837,
44.8852589674395));
#20666=CARTESIAN_POINT('Ctrl Pts',(73.8865748843346,0.256002452711397,44.8736022462753));
#20667=CARTESIAN_POINT('Ctrl Pts',(73.96394371651,1.51086982432855,44.8164245738871));
#20668=CARTESIAN_POINT('Ctrl Pts',(74.8055314959948,3.67609127100912,44.7137259502747));
#20669=CARTESIAN_POINT('Ctrl Pts',(77.1486004080237,5.68908344454576,44.5771630966022));
#20670=CARTESIAN_POINT('Ctrl Pts',(80.1635447169054,6.36155666463022,44.4406002429298));
#20671=CARTESIAN_POINT('Ctrl Pts',(83.1399529776901,5.53505604037131,44.3040373892574));
#20672=CARTESIAN_POINT('Ctrl Pts',(85.3764939963492,3.4043299457581,44.167474535585));
#20673=CARTESIAN_POINT('Ctrl Pts',(86.3461715250332,0.471441453942473,44.0309116819125));
#20674=CARTESIAN_POINT('Ctrl Pts',(85.8205004111942,-2.57253280683391,43.8943488282401));
#20675=CARTESIAN_POINT('Ctrl Pts',(83.9233445571365,-5.0103410604769,43.7577859745677));
#20676=CARTESIAN_POINT('Ctrl Pts',(81.1017308763422,-6.26756245882339,43.6212231208953));
#20677=CARTESIAN_POINT('Ctrl Pts',(78.020516297909,-6.04795786312262,43.4846602672228));
#20678=CARTESIAN_POINT('Ctrl Pts',(75.40572755909,-4.40327273783911,43.3480974135504));
#20679=CARTESIAN_POINT('Ctrl Pts',(74.0989624637806,-2.11574457800119,43.2316303136226));
#20680=CARTESIAN_POINT('Ctrl Pts',(73.88736770816,-0.558117835861341,43.160684164919));
#20681=CARTESIAN_POINT('Ctrl Pts',(73.8872027408445,4.98811089222687E-5,
43.1352589674395));
#20682=CARTESIAN_POINT('Origin',(80.,0.,57.8647410325605));
#20683=CARTESIAN_POINT('',(73.886319437839,6.68934239483887E-5,46.6352589674395));
#20684=CARTESIAN_POINT('',(73.8864333681599,-0.000106876724841452,46.4897410325605));
#20685=CARTESIAN_POINT('',(73.88675,2.47426426879123E-14,57.8647410325605));
#20686=CARTESIAN_POINT('Ctrl Pts',(73.88643336816,-0.000106876724841626,
46.4897410325606));
#20687=CARTESIAN_POINT('Ctrl Pts',(73.8871566616212,0.875730995516464,46.4498311275463));
#20688=CARTESIAN_POINT('Ctrl Pts',(74.2946407647659,2.7511948992005,46.364400271308));
#20689=CARTESIAN_POINT('Ctrl Pts',(76.1457328328429,5.06367217232759,46.2334484638453));
#20690=CARTESIAN_POINT('Ctrl Pts',(78.9843219438627,6.2820816096985,46.0968856101729));
#20691=CARTESIAN_POINT('Ctrl Pts',(82.0622353147722,6.02024391292702,45.9603227565005));
#20692=CARTESIAN_POINT('Ctrl Pts',(84.6542240982161,4.33985590869289,45.8237599028281));
#20693=CARTESIAN_POINT('Ctrl Pts',(86.149537876292,1.63686748781935,45.6871970491556));
#20694=CARTESIAN_POINT('Ctrl Pts',(86.1958358052853,-1.45181608290028,45.5506341954832));
#20695=CARTESIAN_POINT('Ctrl Pts',(84.7822087023876,-4.19840817351866,45.4140713418108));
#20696=CARTESIAN_POINT('Ctrl Pts',(82.2417495768579,-5.95572918282979,45.2775084881383));
#20697=CARTESIAN_POINT('Ctrl Pts',(79.1730669113078,-6.30970149306707,45.140945634466));
#20698=CARTESIAN_POINT('Ctrl Pts',(76.2992345216118,-5.17691859491353,45.0043827807935));
#20699=CARTESIAN_POINT('Ctrl Pts',(74.3388679796599,-2.87301696801453,44.8706479134917));
#20700=CARTESIAN_POINT('Ctrl Pts',(73.886788281912,-0.936796744990568,44.782433997414));
#20701=CARTESIAN_POINT('Ctrl Pts',(73.8863051433301,5.93870499033134E-5,
44.7397410325605));
#20702=CARTESIAN_POINT('Ctrl Pts',(73.886319437839,6.68934239489178E-5,
46.6352589674394));
#20703=CARTESIAN_POINT('Ctrl Pts',(73.8862791662938,0.0706764567001249,
46.6320412788559));
#20704=CARTESIAN_POINT('Ctrl Pts',(73.9044361060887,1.14018559218357,46.5833026390481));
#20705=CARTESIAN_POINT('Ctrl Pts',(74.4932859058703,3.18939648797121,46.4890430480163));
#20706=CARTESIAN_POINT('Ctrl Pts',(76.6439559920085,5.40676601013892,46.3524801943438));
#20707=CARTESIAN_POINT('Ctrl Pts',(79.5854108583403,6.35013904694908,46.2159173406715));
#20708=CARTESIAN_POINT('Ctrl Pts',(82.624555380254,5.79722857302948,46.079354486999));
#20709=CARTESIAN_POINT('Ctrl Pts',(85.0452758157915,3.87831690486471,45.9427916333266));
#20710=CARTESIAN_POINT('Ctrl Pts',(86.2771777145318,1.04555727349326,45.8062287796541));
#20711=CARTESIAN_POINT('Ctrl Pts',(86.0299879841389,-2.03356705891616,45.6696659259817));
#20712=CARTESIAN_POINT('Ctrl Pts',(84.3619519504042,-4.63352190610293,45.5331030723093));
#20713=CARTESIAN_POINT('Ctrl Pts',(81.6661090088627,-6.14167980625449,45.3965402186368));
#20714=CARTESIAN_POINT('Ctrl Pts',(78.5776807367317,-6.20267345467319,45.2599773649644));
#20715=CARTESIAN_POINT('Ctrl Pts',(75.8243936079491,-4.80213091560737,45.123414511292));
#20716=CARTESIAN_POINT('Ctrl Pts',(74.2060361265203,-2.48619421143874,44.9985083787837));
#20717=CARTESIAN_POINT('Ctrl Pts',(73.8875219915012,-0.743153080433105,
44.9191231974995));
#20718=CARTESIAN_POINT('Ctrl Pts',(73.8868174136284,0.000144937957391837,
44.8852589674395));
#20719=CARTESIAN_POINT('Origin',(80.,0.,57.8647410325605));
#20720=CARTESIAN_POINT('',(73.8864122443122,-0.000101181168932138,48.3852589674395));
#20721=CARTESIAN_POINT('',(73.8869623482907,-0.000132973038949946,48.2397410325606));
#20722=CARTESIAN_POINT('',(73.88675,2.47426426879123E-14,57.8647410325605));
#20723=CARTESIAN_POINT('Ctrl Pts',(73.8869623482907,-0.000132973038949845,
48.2397410325606));
#20724=CARTESIAN_POINT('Ctrl Pts',(73.887538634748,0.690679527368656,48.2082701601268));
#20725=CARTESIAN_POINT('Ctrl Pts',(74.1737315907217,2.38118134833958,48.131278336469));
#20726=CARTESIAN_POINT('Ctrl Pts',(75.701999226811,4.69290321850953,48.008765561587));
#20727=CARTESIAN_POINT('Ctrl Pts',(78.4182705988775,6.16395030530382,47.8722027079146));
#20728=CARTESIAN_POINT('Ctrl Pts',(81.507244931279,6.18258554180725,47.7356398542421));
#20729=CARTESIAN_POINT('Ctrl Pts',(84.2410670818731,4.74441790651735,47.5990770005697));
#20730=CARTESIAN_POINT('Ctrl Pts',(85.9755664309368,2.18832289529958,47.4625141468972));
#20731=CARTESIAN_POINT('Ctrl Pts',(86.3020428293569,-0.88340672488984,47.3259512932248));
#20732=CARTESIAN_POINT('Ctrl Pts',(85.1435686306702,-3.74697918411825,47.1893884395524));
#20733=CARTESIAN_POINT('Ctrl Pts',(82.7731151553917,-5.72765079239012,47.05282558588));
#20734=CARTESIAN_POINT('Ctrl Pts',(79.7492324481405,-6.35871582157629,46.9162627322075));
#20735=CARTESIAN_POINT('Ctrl Pts',(76.7844381088919,-5.49147639429357,46.7796998785351));
#20736=CARTESIAN_POINT('Ctrl Pts',(74.5773267431693,-3.33028017053867,46.6431370248627));
#20737=CARTESIAN_POINT('Ctrl Pts',(73.9195634847512,-1.24529947180603,46.5464840762045));
#20738=CARTESIAN_POINT('Ctrl Pts',(73.8863316782904,-0.123243395635752,
46.4953520787704));
#20739=CARTESIAN_POINT('Ctrl Pts',(73.88643336816,-0.000106876724841626,
46.4897410325606));
#20740=CARTESIAN_POINT('Ctrl Pts',(73.8864122443122,-0.000101181168932155,
48.3852589674395));
#20741=CARTESIAN_POINT('Ctrl Pts',(73.8871137806768,0.88427994577413,48.3449593602123));
#20742=CARTESIAN_POINT('Ctrl Pts',(74.3007018159247,2.76826051963491,48.259138801761));
#20743=CARTESIAN_POINT('Ctrl Pts',(76.1670218022879,5.07980592226054,48.1277972920855));
#20744=CARTESIAN_POINT('Ctrl Pts',(79.0107001846261,6.28628952143238,47.991234438413));
#20745=CARTESIAN_POINT('Ctrl Pts',(82.0874873209564,6.01153447605647,47.8546715847406));
#20746=CARTESIAN_POINT('Ctrl Pts',(84.6723997386214,4.32028132816605,47.7181087310682));
#20747=CARTESIAN_POINT('Ctrl Pts',(86.1563544240622,1.61104012280873,47.5815458773957));
#20748=CARTESIAN_POINT('Ctrl Pts',(86.1896870770046,-1.47781052937492,47.4449830237233));
#20749=CARTESIAN_POINT('Ctrl Pts',(84.7645435231389,-4.21844462901729,47.3084201700509));
#20750=CARTESIAN_POINT('Ctrl Pts',(82.2167303935176,-5.96508645657586,47.1718573163784));
#20751=CARTESIAN_POINT('Ctrl Pts',(79.1465889950142,-6.30617473025753,47.035294462706));
#20752=CARTESIAN_POINT('Ctrl Pts',(76.2775368648236,-5.1613388068622,46.8987316090336));
#20753=CARTESIAN_POINT('Ctrl Pts',(74.3325425970884,-2.85596626489593,46.7653864439447));
#20754=CARTESIAN_POINT('Ctrl Pts',(73.8868488917334,-0.928243855928552,
46.67756223008));
#20755=CARTESIAN_POINT('Ctrl Pts',(73.886319437839,6.68934239489178E-5,
46.6352589674394));
#20756=CARTESIAN_POINT('Origin',(80.,0.,57.8647410325605));
#20757=CARTESIAN_POINT('',(73.8869401609568,-0.000135895702726013,50.1352589674395));
#20758=CARTESIAN_POINT('',(73.8872292021947,-5.18097543697425E-6,49.9897410325606));
#20759=CARTESIAN_POINT('',(73.88675,2.47426426879123E-14,57.8647410325605));
#20760=CARTESIAN_POINT('Ctrl Pts',(73.8872292021947,-5.18097543696777E-6,
49.9897410325605));
#20761=CARTESIAN_POINT('Ctrl Pts',(73.8872446337552,0.505626675227688,49.9667091927074));
#20762=CARTESIAN_POINT('Ctrl Pts',(74.0720197357253,2.0106184806943,49.8981564016301));
#20763=CARTESIAN_POINT('Ctrl Pts',(75.2937534075295,4.28338584247207,49.7840826593286));
#20764=CARTESIAN_POINT('Ctrl Pts',(77.8652792970721,5.99492441863291,49.6475198056562));
#20765=CARTESIAN_POINT('Ctrl Pts',(80.939809508912,6.2938787207563,49.5109569519837));
#20766=CARTESIAN_POINT('Ctrl Pts',(83.792892369597,5.10980613499994,49.3743940983113));
#20767=CARTESIAN_POINT('Ctrl Pts',(85.7522558536446,2.72170973082036,49.2378312446388));
#20768=CARTESIAN_POINT('Ctrl Pts',(86.3562150670656,-0.307703243139823,
49.1012683909664));
#20769=CARTESIAN_POINT('Ctrl Pts',(85.4624590769004,-3.26461208994559,48.964705537294));
#20770=CARTESIAN_POINT('Ctrl Pts',(83.2815836418895,-5.45228026296463,48.8281426836216));
#20771=CARTESIAN_POINT('Ctrl Pts',(80.3274685256469,-6.35522742546172,48.6915798299491));
#20772=CARTESIAN_POINT('Ctrl Pts',(77.2961919879637,-5.76069210240215,48.5550169762767));
#20773=CARTESIAN_POINT('Ctrl Pts',(74.9020138373674,-3.80876467509304,48.4184541226043));
#20774=CARTESIAN_POINT('Ctrl Pts',(73.9839869412179,-1.61601829022539,48.3133621413656));
#20775=CARTESIAN_POINT('Ctrl Pts',(73.8867050668903,-0.308544189810323,
48.253791111351));
#20776=CARTESIAN_POINT('Ctrl Pts',(73.8869623482907,-0.000132973038949845,
48.2397410325606));
#20777=CARTESIAN_POINT('Ctrl Pts',(73.8869401609568,-0.000135895702726048,
50.1352589674395));
#20778=CARTESIAN_POINT('Ctrl Pts',(73.8875399757514,0.699223566656964,50.1033983927928));
#20779=CARTESIAN_POINT('Ctrl Pts',(74.1788859977704,2.39828340957575,50.026016866922));
#20780=CARTESIAN_POINT('Ctrl Pts',(75.7217357950776,4.71090282906051,49.9031143898271));
#20781=CARTESIAN_POINT('Ctrl Pts',(78.4441579740491,6.17053528166351,49.7665515361547));
#20782=CARTESIAN_POINT('Ctrl Pts',(81.5331832701364,6.17620426573987,49.6299886824822));
#20783=CARTESIAN_POINT('Ctrl Pts',(84.2609445326221,4.72657399835094,49.4934258288098));
#20784=CARTESIAN_POINT('Ctrl Pts',(85.9846992690839,2.16322091580975,49.3568629751373));
#20785=CARTESIAN_POINT('Ctrl Pts',(86.2982790838942,-0.909851995299122,
49.2203001214649));
#20786=CARTESIAN_POINT('Ctrl Pts',(85.1277951530875,-3.76853644535141,49.0837372677925));
#20787=CARTESIAN_POINT('Ctrl Pts',(82.7490486508255,-5.73924050614397,48.94717441412));
#20788=CARTESIAN_POINT('Ctrl Pts',(79.7225437079984,-6.35760710314802,48.8106115604476));
#20789=CARTESIAN_POINT('Ctrl Pts',(76.7614158020519,-5.47793049104956,48.6740487067752));
#20790=CARTESIAN_POINT('Ctrl Pts',(74.563395616688,-3.3074889041874,48.5374858531028));
#20791=CARTESIAN_POINT('Ctrl Pts',(73.9170067231604,-1.22818326457397,48.4412226066575));
#20792=CARTESIAN_POINT('Ctrl Pts',(73.886321351052,-0.114684384477866,48.3904803114364));
#20793=CARTESIAN_POINT('Ctrl Pts',(73.8864122443122,-0.000101181168932155,
48.3852589674395));
#20794=CARTESIAN_POINT('Origin',(80.,0.,57.8647410325605));
#20795=CARTESIAN_POINT('',(73.8872279103786,-1.26095903427159E-5,51.8852589674395));
#20796=CARTESIAN_POINT('',(73.8869923021753,0.000128310058932331,51.7397410325606));
#20797=CARTESIAN_POINT('',(73.88675,2.47426426879123E-14,57.8647410325605));
#20798=CARTESIAN_POINT('Ctrl Pts',(73.8869923021753,0.000128310058932178,
51.7397410325606));
#20799=CARTESIAN_POINT('Ctrl Pts',(73.8867364614564,0.320457389107717,51.7251482252879));
#20800=CARTESIAN_POINT('Ctrl Pts',(73.9887295387364,1.63986289423491,51.6650344667911));
#20801=CARTESIAN_POINT('Ctrl Pts',(74.9243661842076,3.83850135239988,51.5593997570702));
#20802=CARTESIAN_POINT('Ctrl Pts',(77.3299139839692,5.77639956476208,51.4228369033978));
#20803=CARTESIAN_POINT('Ctrl Pts',(80.3646142555919,6.35320452285083,51.2862740497253));
#20804=CARTESIAN_POINT('Ctrl Pts',(83.3134004559793,5.43300365203046,51.1497111960529));
#20805=CARTESIAN_POINT('Ctrl Pts',(85.481449977994,3.23262391926018,51.0131483423805));
#20806=CARTESIAN_POINT('Ctrl Pts',(86.3579052283988,0.270540886612342,50.8765854887081));
#20807=CARTESIAN_POINT('Ctrl Pts',(85.736247022437,-2.75528970567801,50.7400226350356));
#20808=CARTESIAN_POINT('Ctrl Pts',(83.7629567073689,-5.13189127740411,50.6034597813632));
#20809=CARTESIAN_POINT('Ctrl Pts',(80.903000756919,-6.2992651077435,50.4668969276907));
#20810=CARTESIAN_POINT('Ctrl Pts',(77.8302707029787,-5.98234285562748,50.3303340740183));
#20811=CARTESIAN_POINT('Ctrl Pts',(75.2687940477242,-4.25580092365468,50.1937712203459));
#20812=CARTESIAN_POINT('Ctrl Pts',(74.0661167021499,-1.98677733436168,50.0802402065266));
#20813=CARTESIAN_POINT('Ctrl Pts',(73.8872141342676,-0.493722191832877,
50.0122301439315));
#20814=CARTESIAN_POINT('Ctrl Pts',(73.8872292021947,-5.18097543696777E-6,
49.9897410325605));
#20815=CARTESIAN_POINT('Ctrl Pts',(73.8872279103786,-1.26095903429935E-5,
51.8852589674395));
#20816=CARTESIAN_POINT('Ctrl Pts',(73.8872661113861,0.514174273776074,51.8618374253733));
#20817=CARTESIAN_POINT('Ctrl Pts',(74.076305415408,2.02773695413552,51.7928949320831));
#20818=CARTESIAN_POINT('Ctrl Pts',(75.3117746142583,4.30310269326682,51.6784314875687));
#20819=CARTESIAN_POINT('Ctrl Pts',(77.8904620590793,6.00383208915477,51.5418686338962));
#20820=CARTESIAN_POINT('Ctrl Pts',(80.9662200126132,6.28987829428071,51.4053057802239));
#20821=CARTESIAN_POINT('Ctrl Pts',(83.8143075062239,5.09384023309799,51.2687429265514));
#20822=CARTESIAN_POINT('Ctrl Pts',(85.7636295740737,2.6975403991448,51.132180072879));
#20823=CARTESIAN_POINT('Ctrl Pts',(86.354867380944,-0.334380983822473,50.9956172192065));
#20824=CARTESIAN_POINT('Ctrl Pts',(85.4487075396391,-3.28751216265552,50.8590543655341));
#20825=CARTESIAN_POINT('Ctrl Pts',(83.258668528712,-5.46600672263342,50.7224915118617));
#20826=CARTESIAN_POINT('Ctrl Pts',(80.3007893255799,-6.35654590588445,50.5859286581892));
#20827=CARTESIAN_POINT('Ctrl Pts',(77.2720351219492,-5.74929192997566,50.4493658045168));
#20828=CARTESIAN_POINT('Ctrl Pts',(74.8860713886881,-3.78733207289439,50.3128029508444));
#20829=CARTESIAN_POINT('Ctrl Pts',(73.9806267980956,-1.59889694717195,50.2081006718186));
#20830=CARTESIAN_POINT('Ctrl Pts',(73.8866829874418,-0.299989671876453,
50.148919344017));
#20831=CARTESIAN_POINT('Ctrl Pts',(73.8869401609568,-0.000135895702726048,
50.1352589674395));
#20832=CARTESIAN_POINT('Origin',(80.,0.,57.8647410325605));
#20833=CARTESIAN_POINT('',(73.8870077577991,0.000138281717805,53.6352589674395));
#20834=CARTESIAN_POINT('',(73.8864642614677,0.000114121245111251,53.4897410325605));
#20835=CARTESIAN_POINT('',(73.88675,2.47426426879123E-14,57.8647410325605));
#20836=CARTESIAN_POINT('',(78.4211181181246,-5.90584097022478,54.));
#20837=CARTESIAN_POINT('Ctrl Pts',(78.4211181181246,-5.90584097022479,54.));
#20838=CARTESIAN_POINT('Ctrl Pts',(77.455879038986,-5.647791608345,53.9544790487759));
#20839=CARTESIAN_POINT('Ctrl Pts',(75.6552430725963,-4.64961437394933,53.8634371463276));
#20840=CARTESIAN_POINT('Ctrl Pts',(74.161524344143,-2.34018528006132,53.7418568021407));
#20841=CARTESIAN_POINT('Ctrl Pts',(73.8875141280071,-0.670206627459226,
53.665797409178));
#20842=CARTESIAN_POINT('Ctrl Pts',(73.8870077577991,0.000138281717805347,
53.6352589674395));
#20843=CARTESIAN_POINT('',(81.5790669755174,-5.90611323035058,54.));
#20844=CARTESIAN_POINT('Origin',(80.,0.,54.));
#20845=CARTESIAN_POINT('Ctrl Pts',(81.5790669755174,-5.90611323035057,54.));
#20846=CARTESIAN_POINT('Ctrl Pts',(80.7376823715278,-6.13029255477271,53.9603227565005));
#20847=CARTESIAN_POINT('Ctrl Pts',(78.8264544132615,-6.2231800657142,53.8751245617769));
#20848=CARTESIAN_POINT('Ctrl Pts',(76.1161979867926,-5.04105954615917,53.7444054158291));
#20849=CARTESIAN_POINT('Ctrl Pts',(74.2862708285712,-2.72742222003944,53.6139963368488));
#20850=CARTESIAN_POINT('Ctrl Pts',(73.8872120918914,-0.863825582696248,
53.5291082090926));
#20851=CARTESIAN_POINT('Ctrl Pts',(73.8864642614677,0.000114121245111225,
53.4897410325605));
#20852=CARTESIAN_POINT('Origin',(32.,-32.,48.));
#20853=CARTESIAN_POINT('',(33.6684805778295,-31.9993859124995,53.3285196366098));
#20854=CARTESIAN_POINT('',(33.6648118344815,-31.9985150168184,53.5214803633902));
#20855=CARTESIAN_POINT('',(33.666,-32.,48.));
#20856=CARTESIAN_POINT('',(31.3249228143251,-33.5230977622534,54.));
#20857=CARTESIAN_POINT('Ctrl Pts',(33.6648118344815,-31.9985150168184,53.5214803633902));
#20858=CARTESIAN_POINT('Ctrl Pts',(33.6661629666675,-31.8287715688263,53.5328138566339));
#20859=CARTESIAN_POINT('Ctrl Pts',(33.6422867594775,-31.659410867237,53.5441473498775));
#20860=CARTESIAN_POINT('Ctrl Pts',(33.5916050633703,-31.4985170507268,53.5554808431211));
#20861=CARTESIAN_POINT('Ctrl Pts',(33.4259531005074,-30.9726392967347,53.5925241061943));
#20862=CARTESIAN_POINT('Ctrl Pts',(32.973939640304,-30.537212789371,53.6295673692676));
#20863=CARTESIAN_POINT('Ctrl Pts',(32.442142359202,-30.3909996812704,53.6666106323408));
#20864=CARTESIAN_POINT('Ctrl Pts',(31.9103450780999,-30.2447865731697,53.703653895414));
#20865=CARTESIAN_POINT('Ctrl Pts',(31.2987639760992,-30.387786864332,53.7406971584873));
#20866=CARTESIAN_POINT('Ctrl Pts',(30.8877751462098,-30.7555547378681,53.7777404215606));
#20867=CARTESIAN_POINT('Ctrl Pts',(30.4767863163205,-31.1233226114042,53.8147836846338));
#20868=CARTESIAN_POINT('Ctrl Pts',(30.2663897585425,-31.7158580673142,53.851826947707));
#20869=CARTESIAN_POINT('Ctrl Pts',(30.351816552213,-32.2596861396068,53.8888702107803));
#20870=CARTESIAN_POINT('Ctrl Pts',(30.4372433458836,-32.8035142118994,53.9259134738535));
#20871=CARTESIAN_POINT('Ctrl Pts',(30.8184934910026,-33.2986349005747,53.9629567369268));
#20872=CARTESIAN_POINT('Ctrl Pts',(31.3249228143251,-33.5230977622534,54.));
#20873=CARTESIAN_POINT('',(33.666,-32.,54.));
#20874=CARTESIAN_POINT('Origin',(32.,-32.,54.));
#20875=CARTESIAN_POINT('',(33.666,-32.,55.));
#20876=CARTESIAN_POINT('',(33.666,-32.,48.));
#20877=CARTESIAN_POINT('Origin',(32.,-32.,55.));
#20878=CARTESIAN_POINT('',(33.6146716598692,-32.4224676707571,54.));
#20879=CARTESIAN_POINT('Origin',(32.,-32.,54.));
#20880=CARTESIAN_POINT('Ctrl Pts',(33.6146732908669,-32.4224680167337,54.));
#20881=CARTESIAN_POINT('Ctrl Pts',(33.4771404824827,-32.9453622991658,53.9636851831628));
#20882=CARTESIAN_POINT('Ctrl Pts',(33.0618476186246,-33.3962238432118,53.9273703663255));
#20883=CARTESIAN_POINT('Ctrl Pts',(32.5515251931148,-33.574862517777,53.8910555494883));
#20884=CARTESIAN_POINT('Ctrl Pts',(32.0309661071345,-33.7570845415485,53.854012286415));
#20885=CARTESIAN_POINT('Ctrl Pts',(31.4115267880172,-33.6560530141969,53.8169690233418));
#20886=CARTESIAN_POINT('Ctrl Pts',(30.9761676664273,-33.3177477807437,53.7799257602686));
#20887=CARTESIAN_POINT('Ctrl Pts',(30.5408085448373,-32.9794425472904,53.7428824971953));
#20888=CARTESIAN_POINT('Ctrl Pts',(30.2895296207747,-32.4038636077355,53.7058392341221));
#20889=CARTESIAN_POINT('Ctrl Pts',(30.3375623733908,-31.8545189866324,53.6687959710489));
#20890=CARTESIAN_POINT('Ctrl Pts',(30.3855951260069,-31.3051743655294,53.6317527079756));
#20891=CARTESIAN_POINT('Ctrl Pts',(30.7329395553015,-30.7820640628781,53.5947094449023));
#20892=CARTESIAN_POINT('Ctrl Pts',(31.2205277178506,-30.5244968291776,53.5576661818291));
#20893=CARTESIAN_POINT('Ctrl Pts',(31.7081158803996,-30.2669295954771,53.5206229187558));
#20894=CARTESIAN_POINT('Ctrl Pts',(32.335947776203,-30.2749054307274,53.4835796556826));
#20895=CARTESIAN_POINT('Ctrl Pts',(32.8167940806439,-30.5448068015671,53.4465363926094));
#20896=CARTESIAN_POINT('Ctrl Pts',(33.2976403850846,-30.8147081724067,53.4094931295362));
#20897=CARTESIAN_POINT('Ctrl Pts',(33.6315010981628,-31.3465350788358,53.3724498664629));
#20898=CARTESIAN_POINT('Ctrl Pts',(33.6655714697797,-31.8969101642465,53.3354066033897));
#20899=CARTESIAN_POINT('Ctrl Pts',(33.6676828885014,-31.9310181649572,53.3331109477964));
#20900=CARTESIAN_POINT('Ctrl Pts',(33.6686429432612,-31.9651974011345,53.3308152922031));
#20901=CARTESIAN_POINT('Ctrl Pts',(33.6684805778295,-31.9993859124995,53.3285196366098));
#20902=CARTESIAN_POINT('Origin',(32.,-32.,48.));
#20903=CARTESIAN_POINT('',(33.6641301080328,-31.9988695643883,52.6285196366098));
#20904=CARTESIAN_POINT('',(33.6637769838569,-32.0008964513587,52.8214803633902));
#20905=CARTESIAN_POINT('',(33.666,-32.,48.));
#20906=CARTESIAN_POINT('Ctrl Pts',(33.6637769838569,-32.0008964513587,52.8214803633902));
#20907=CARTESIAN_POINT('Ctrl Pts',(33.6621335736406,-31.664768877266,52.8438876115277));
#20908=CARTESIAN_POINT('Ctrl Pts',(33.563356481064,-31.3277533767314,52.8662948596652));
#20909=CARTESIAN_POINT('Ctrl Pts',(33.374088211561,-31.0530981103508,52.8887021078028));
#20910=CARTESIAN_POINT('Ctrl Pts',(33.0611932832952,-30.599042921398,52.925745370876));
#20911=CARTESIAN_POINT('Ctrl Pts',(32.50098494745,-30.3154189560176,52.9627886339492));
#20912=CARTESIAN_POINT('Ctrl Pts',(31.9498071641372,-30.3320029614108,52.9998318970225));
#20913=CARTESIAN_POINT('Ctrl Pts',(31.3986293808243,-30.348586966804,53.0368751600957));
#20914=CARTESIAN_POINT('Ctrl Pts',(30.8564821500439,-30.6653789429709,53.073918423169));
#20915=CARTESIAN_POINT('Ctrl Pts',(30.5714576898881,-31.1374325180527,53.1109616862422));
#20916=CARTESIAN_POINT('Ctrl Pts',(30.2864332297323,-31.6094860931344,53.1480049493154));
#20917=CARTESIAN_POINT('Ctrl Pts',(30.2585315402012,-32.2368012671311,53.1850482123886));
#20918=CARTESIAN_POINT('Ctrl Pts',(30.5005032885542,-32.7322905055208,53.2220914754619));
#20919=CARTESIAN_POINT('Ctrl Pts',(30.7424750369073,-33.2277797439105,53.2591347385351));
#20920=CARTESIAN_POINT('Ctrl Pts',(31.2543202231446,-33.5914430466933,53.2961780016084));
#20921=CARTESIAN_POINT('Ctrl Pts',(31.8018549075792,-33.656932440832,53.3332212646817));
#20922=CARTESIAN_POINT('Ctrl Pts',(32.3493895920138,-33.7224218349707,53.3702645277549));
#20923=CARTESIAN_POINT('Ctrl Pts',(32.9326137746457,-33.4897373204654,53.4073077908281));
#20924=CARTESIAN_POINT('Ctrl Pts',(33.2845806332005,-33.0652305629025,53.4443510539014));
#20925=CARTESIAN_POINT('Ctrl Pts',(33.5288622156088,-32.7706028729368,53.470060823731));
#20926=CARTESIAN_POINT('Ctrl Pts',(33.6617468220652,-32.3835741406163,53.4957705935606));
#20927=CARTESIAN_POINT('Ctrl Pts',(33.6648118344815,-31.9985150168184,53.5214803633902));
#20928=CARTESIAN_POINT('Ctrl Pts',(33.6684805778295,-31.9993859124995,53.3285196366098));
#20929=CARTESIAN_POINT('Ctrl Pts',(33.6660229747349,-32.5168716262576,53.2937720291298));
#20930=CARTESIAN_POINT('Ctrl Pts',(33.406412239859,-33.0364823406136,53.2590244216499));
#20931=CARTESIAN_POINT('Ctrl Pts',(32.9900196909147,-33.3433519640963,53.2242768141699));
#20932=CARTESIAN_POINT('Ctrl Pts',(32.5461175102774,-33.6704954141429,53.1872335510967));
#20933=CARTESIAN_POINT('Ctrl Pts',(31.9240331188471,-33.7558590498438,53.1501902880235));
#20934=CARTESIAN_POINT('Ctrl Pts',(31.408420821415,-33.5603767883024,53.1131470249502));
#20935=CARTESIAN_POINT('Ctrl Pts',(30.8928085239829,-33.364894526761,53.076103761877));
#20936=CARTESIAN_POINT('Ctrl Pts',(30.483668320549,-32.8885663679775,53.0390604988037));
#20937=CARTESIAN_POINT('Ctrl Pts',(30.3682246614595,-32.3493595890129,53.0020172357305));
#20938=CARTESIAN_POINT('Ctrl Pts',(30.2527810023701,-31.8101528100483,52.9649739726572));
#20939=CARTESIAN_POINT('Ctrl Pts',(30.4310338876251,-31.2080674109028,52.927930709584));
#20940=CARTESIAN_POINT('Ctrl Pts',(30.8214136864304,-30.8186133475755,52.8908874465107));
#20941=CARTESIAN_POINT('Ctrl Pts',(31.2117934852357,-30.4291592842482,52.8538441834375));
#20942=CARTESIAN_POINT('Ctrl Pts',(31.8143001975914,-30.2523365567391,52.8168009203643));
#20943=CARTESIAN_POINT('Ctrl Pts',(32.3532310680952,-30.3690588208124,52.779757657291));
#20944=CARTESIAN_POINT('Ctrl Pts',(32.892161938599,-30.4857810848857,52.7427143942178));
#20945=CARTESIAN_POINT('Ctrl Pts',(33.3675169672511,-30.8960483405412,52.7056711311445));
#20946=CARTESIAN_POINT('Ctrl Pts',(33.5617757404346,-31.4121242462018,52.6686278680713));
#20947=CARTESIAN_POINT('Ctrl Pts',(33.6318863371789,-31.5983829624405,52.6552584575841));
#20948=CARTESIAN_POINT('Ctrl Pts',(33.6653817597626,-31.7984241538003,52.641889047097));
#20949=CARTESIAN_POINT('Ctrl Pts',(33.6641301080328,-31.9988695643883,52.6285196366098));
#20950=CARTESIAN_POINT('Origin',(32.,-32.,48.));
#20951=CARTESIAN_POINT('',(33.6643835906196,-32.0012498155686,51.9285196366098));
#20952=CARTESIAN_POINT('',(33.6681251706529,-32.0009136526364,52.1214803633902));
#20953=CARTESIAN_POINT('',(33.666,-32.,48.));
#20954=CARTESIAN_POINT('Ctrl Pts',(33.6681251706529,-32.0009136526364,52.1214803633902));
#20955=CARTESIAN_POINT('Ctrl Pts',(33.6648306539093,-31.5020153412742,52.1549613664216));
#20956=CARTESIAN_POINT('Ctrl Pts',(33.4261511460292,-31.0003826202633,52.188442369453));
#20957=CARTESIAN_POINT('Ctrl Pts',(33.0352551049814,-30.6911883151967,52.2219233724844));
#20958=CARTESIAN_POINT('Ctrl Pts',(32.6027691107821,-30.3490968320775,52.2589666355576));
#20959=CARTESIAN_POINT('Ctrl Pts',(31.9839528618204,-30.2425717379885,52.2960098986308));
#20960=CARTESIAN_POINT('Ctrl Pts',(31.461973246163,-30.4203582047467,52.3330531617041));
#20961=CARTESIAN_POINT('Ctrl Pts',(30.9399936305057,-30.598144671505,52.3700964247773));
#20962=CARTESIAN_POINT('Ctrl Pts',(30.5148506481528,-31.0602426991104,52.4071396878506));
#20963=CARTESIAN_POINT('Ctrl Pts',(30.3810875652485,-31.5951990002834,52.4441829509239));
#20964=CARTESIAN_POINT('Ctrl Pts',(30.2473244823442,-32.1301553014564,52.4812262139971));
#20965=CARTESIAN_POINT('Ctrl Pts',(30.4049412988885,-32.7379698761969,52.5182694770703));
#20966=CARTESIAN_POINT('Ctrl Pts',(30.7818131318635,-33.1405095471833,52.5553127401435));
#20967=CARTESIAN_POINT('Ctrl Pts',(31.1586849648385,-33.5430492181697,52.5923560032168));
#20968=CARTESIAN_POINT('Ctrl Pts',(31.7548118142443,-33.740313985402,52.62939926629));
#20969=CARTESIAN_POINT('Ctrl Pts',(32.2974098252054,-33.6420375976381,52.6664425293633));
#20970=CARTESIAN_POINT('Ctrl Pts',(32.8400078361665,-33.5437612098741,52.7034857924365));
#20971=CARTESIAN_POINT('Ctrl Pts',(33.329077008683,-33.1499436671139,52.7405290555098));
#20972=CARTESIAN_POINT('Ctrl Pts',(33.540820834598,-32.6407916894713,52.777572318583));
#20973=CARTESIAN_POINT('Ctrl Pts',(33.6244820874556,-32.439622695946,52.7922083335187));
#20974=CARTESIAN_POINT('Ctrl Pts',(33.6648504301063,-32.2204489892046,52.8068443484545));
#20975=CARTESIAN_POINT('Ctrl Pts',(33.6637769838569,-32.0008964513587,52.8214803633902));
#20976=CARTESIAN_POINT('Ctrl Pts',(33.6641301080328,-31.9988695643883,52.6285196366098));
#20977=CARTESIAN_POINT('Ctrl Pts',(33.6619137486376,-32.3538078098979,52.6048457840237));
#20978=CARTESIAN_POINT('Ctrl Pts',(33.5507462927464,-32.7100135039337,52.5811719314377));
#20979=CARTESIAN_POINT('Ctrl Pts',(33.3409999223511,-32.9932070489303,52.5574980788516));
#20980=CARTESIAN_POINT('Ctrl Pts',(33.0128028133694,-33.4363293903327,52.5204548157783));
#20981=CARTESIAN_POINT('Ctrl Pts',(32.443246077691,-33.7006895174718,52.4834115527051));
#20982=CARTESIAN_POINT('Ctrl Pts',(31.8929556540234,-33.6653176007117,52.4463682896318));
#20983=CARTESIAN_POINT('Ctrl Pts',(31.3426652303558,-33.6299456839516,52.4093250265586));
#20984=CARTESIAN_POINT('Ctrl Pts',(30.8116411186989,-33.2948417232924,52.3722817634854));
#20985=CARTESIAN_POINT('Ctrl Pts',(30.5428771415083,-32.8133475089059,52.3352385004122));
#20986=CARTESIAN_POINT('Ctrl Pts',(30.2741131643176,-32.3318532945195,52.2981952373389));
#20987=CARTESIAN_POINT('Ctrl Pts',(30.2676093215931,-31.7039688264058,52.2611519742656));
#20988=CARTESIAN_POINT('Ctrl Pts',(30.5263417019884,-31.2170106150328,52.2241087111924));
#20989=CARTESIAN_POINT('Ctrl Pts',(30.7850740823836,-30.7300524036599,52.1870654481191));
#20990=CARTESIAN_POINT('Ctrl Pts',(31.3090426858984,-30.3840204490277,52.1500221850459));
#20991=CARTESIAN_POINT('Ctrl Pts',(31.8584823380995,-30.3372571061758,52.1129789219727));
#20992=CARTESIAN_POINT('Ctrl Pts',(32.4079219903006,-30.2904937633239,52.0759356588994));
#20993=CARTESIAN_POINT('Ctrl Pts',(32.982832691188,-30.5429990322524,52.0388923958262));
#20994=CARTESIAN_POINT('Ctrl Pts',(33.3201384125524,-30.9792278665667,52.0018491327529));
#20995=CARTESIAN_POINT('Ctrl Pts',(33.5427111247615,-31.2670754441422,51.9774059673719));
#20996=CARTESIAN_POINT('Ctrl Pts',(33.6618287241732,-31.6349177348701,51.9529628019908));
#20997=CARTESIAN_POINT('Ctrl Pts',(33.6643835906196,-32.0012498155686,51.9285196366098));
#20998=CARTESIAN_POINT('Origin',(32.,-32.,48.));
#20999=CARTESIAN_POINT('',(33.6686262364557,-32.0004179151258,51.2285196366098));
#21000=CARTESIAN_POINT('',(33.6665286247185,-31.9985210141682,51.4214803633902));
#21001=CARTESIAN_POINT('',(33.666,-32.,48.));
#21002=CARTESIAN_POINT('Ctrl Pts',(33.6665286247185,-31.9985210141682,51.4214803633902));
#21003=CARTESIAN_POINT('Ctrl Pts',(33.6675618774755,-31.8863136434922,51.4289918582422));
#21004=CARTESIAN_POINT('Ctrl Pts',(33.6571969459659,-31.774296080394,51.4365033530943));
#21005=CARTESIAN_POINT('Ctrl Pts',(33.634733907746,-31.6647595174629,51.4440148479463));
#21006=CARTESIAN_POINT('Ctrl Pts',(33.5239564592356,-31.1245752003957,51.4810581110195));
#21007=CARTESIAN_POINT('Ctrl Pts',(33.1189515966928,-30.6447291065599,51.5181013740928));
#21008=CARTESIAN_POINT('Ctrl Pts',(32.6050473497745,-30.4447962077593,51.555144637166));
#21009=CARTESIAN_POINT('Ctrl Pts',(32.0911431028562,-30.2448633089587,51.5921879002393));
#21010=CARTESIAN_POINT('Ctrl Pts',(31.4683394715624,-30.3248436051933,51.6292311633125));
#21011=CARTESIAN_POINT('Ctrl Pts',(31.0216280193636,-30.6481385443608,51.6662744263857));
#21012=CARTESIAN_POINT('Ctrl Pts',(30.5749165671649,-30.9714334835282,51.703317689459));
#21013=CARTESIAN_POINT('Ctrl Pts',(30.3042972940611,-31.5380430656285,51.7403609525322));
#21014=CARTESIAN_POINT('Ctrl Pts',(30.3336041144233,-32.0886898226008,51.7774042156055));
#21015=CARTESIAN_POINT('Ctrl Pts',(30.3629109347855,-32.6393365795731,51.8144474786787));
#21016=CARTESIAN_POINT('Ctrl Pts',(30.6921438486138,-33.1740205114175,51.8514907417519));
#21017=CARTESIAN_POINT('Ctrl Pts',(31.1706476550385,-33.448073141423,51.8885340048252));
#21018=CARTESIAN_POINT('Ctrl Pts',(31.6491514614632,-33.7221257714285,51.9255772678984));
#21019=CARTESIAN_POINT('Ctrl Pts',(32.2769261604843,-33.735547099595,51.9626205309717));
#21020=CARTESIAN_POINT('Ctrl Pts',(32.7667054630863,-33.4821956161538,51.9996637940449));
#21021=CARTESIAN_POINT('Ctrl Pts',(33.2564847656884,-33.2288441327127,52.0367070571182));
#21022=CARTESIAN_POINT('Ctrl Pts',(33.6082686718714,-32.7087198376638,52.0737503201914));
#21023=CARTESIAN_POINT('Ctrl Pts',(33.6610827552445,-32.1598287540646,52.1107935832646));
#21024=CARTESIAN_POINT('Ctrl Pts',(33.6661616139421,-32.1070447223078,52.1143558433065));
#21025=CARTESIAN_POINT('Ctrl Pts',(33.6684756955563,-32.053994664512,52.1179181033483));
#21026=CARTESIAN_POINT('Ctrl Pts',(33.6681251706529,-32.0009136526364,52.1214803633902));
#21027=CARTESIAN_POINT('Ctrl Pts',(33.6643835906196,-32.0012498155686,51.9285196366098));
#21028=CARTESIAN_POINT('Ctrl Pts',(33.6657005872652,-32.1900886968112,51.9159195389176));
#21029=CARTESIAN_POINT('Ctrl Pts',(33.6360439148516,-32.3785262770164,51.9033194412254));
#21030=CARTESIAN_POINT('Ctrl Pts',(33.5736181236639,-32.5553982113817,51.8907193435332));
#21031=CARTESIAN_POINT('Ctrl Pts',(33.3900913715693,-33.0753873221826,51.85367608046));
#21032=CARTESIAN_POINT('Ctrl Pts',(32.9233371255385,-33.4954131440844,51.8166328173867));
#21033=CARTESIAN_POINT('Ctrl Pts',(32.3869395954384,-33.6232741373353,51.7795895543135));
#21034=CARTESIAN_POINT('Ctrl Pts',(31.8505420653383,-33.7511351305863,51.7425462912403));
#21035=CARTESIAN_POINT('Ctrl Pts',(31.244501251169,-33.5868312951865,51.705503028167));
#21036=CARTESIAN_POINT('Ctrl Pts',(30.8461381445101,-33.2055471758926,51.6684597650938));
#21037=CARTESIAN_POINT('Ctrl Pts',(30.4477750378511,-32.8242630565987,51.6314165020205));
#21038=CARTESIAN_POINT('Ctrl Pts',(30.2570896387025,-32.2259986534107,51.5943732389472));
#21039=CARTESIAN_POINT('Ctrl Pts',(30.3613385511927,-31.6845165129817,51.557329975874));
#21040=CARTESIAN_POINT('Ctrl Pts',(30.4655874636828,-31.1430343725527,51.5202867128007));
#21041=CARTESIAN_POINT('Ctrl Pts',(30.8647706878118,-30.6583344948828,51.4832434497275));
#21042=CARTESIAN_POINT('Ctrl Pts',(31.3762241449887,-30.4522129159655,51.4462001866543));
#21043=CARTESIAN_POINT('Ctrl Pts',(31.8876776021656,-30.2460913370482,51.4091569235811));
#21044=CARTESIAN_POINT('Ctrl Pts',(32.5114012923905,-30.3185480568836,51.3721136605078));
#21045=CARTESIAN_POINT('Ctrl Pts',(32.9619826368709,-30.6364272732807,51.3350703974346));
#21046=CARTESIAN_POINT('Ctrl Pts',(33.3939980793994,-30.9412084898682,51.2995534771596));
#21047=CARTESIAN_POINT('Ctrl Pts',(33.6668456440257,-31.4716039419519,51.2640365568847));
#21048=CARTESIAN_POINT('Ctrl Pts',(33.6686262364557,-32.0004179151258,51.2285196366098));
#21049=CARTESIAN_POINT('Origin',(32.,-32.,48.));
#21050=CARTESIAN_POINT('',(33.6656097964572,-31.9984850050081,50.5285196366098));
#21051=CARTESIAN_POINT('',(33.6632910498763,-32.0000156711391,50.7214803633902));
#21052=CARTESIAN_POINT('',(33.666,-32.,48.));
#21053=CARTESIAN_POINT('Ctrl Pts',(33.6632910498763,-32.0000156711391,50.7214803633902));
#21054=CARTESIAN_POINT('Ctrl Pts',(33.663267639484,-31.7210181193327,50.7400656131361));
#21055=CARTESIAN_POINT('Ctrl Pts',(33.5968497698977,-31.4420100931612,50.758650862882));
#21056=CARTESIAN_POINT('Ctrl Pts',(33.4640996060852,-31.1992794035667,50.7772361126279));
#21057=CARTESIAN_POINT('Ctrl Pts',(33.1995080989302,-30.7154797821718,50.8142793757012));
#21058=CARTESIAN_POINT('Ctrl Pts',(32.6714007751648,-30.3757977747389,50.8513226387744));
#21059=CARTESIAN_POINT('Ctrl Pts',(32.1214366826114,-30.3356700260391,50.8883659018477));
#21060=CARTESIAN_POINT('Ctrl Pts',(31.571472590058,-30.2955422773393,50.9254091649209));
#21061=CARTESIAN_POINT('Ctrl Pts',(30.9996517287167,-30.5549687873725,50.9624524279942));
#21062=CARTESIAN_POINT('Ctrl Pts',(30.6676362241477,-30.9952373917923,50.9994956910674));
#21063=CARTESIAN_POINT('Ctrl Pts',(30.3356207195788,-31.4355059962121,51.0365389541406));
#21064=CARTESIAN_POINT('Ctrl Pts',(30.2434105717823,-32.0566166950185,51.0735822172139));
#21065=CARTESIAN_POINT('Ctrl Pts',(30.4332006444406,-32.5743526003433,51.1106254802871));
#21066=CARTESIAN_POINT('Ctrl Pts',(30.6229907170988,-33.0920885056681,51.1476687433603));
#21067=CARTESIAN_POINT('Ctrl Pts',(31.0947810102119,-33.5064496175111,51.1847120064336));
#21068=CARTESIAN_POINT('Ctrl Pts',(31.6326828437495,-33.6278265377282,51.2217552695068));
#21069=CARTESIAN_POINT('Ctrl Pts',(32.1705846772872,-33.7492034579452,51.2587985325801));
#21070=CARTESIAN_POINT('Ctrl Pts',(32.7745980512495,-33.5775961865362,51.2958417956533));
#21071=CARTESIAN_POINT('Ctrl Pts',(33.1683297209918,-33.1915312806824,51.3328850587266));
#21072=CARTESIAN_POINT('Ctrl Pts',(33.4822219499024,-32.8837511778476,51.3624168269478));
#21073=CARTESIAN_POINT('Ctrl Pts',(33.6624663466319,-32.4396691649416,51.391948595169));
#21074=CARTESIAN_POINT('Ctrl Pts',(33.6665286247185,-31.9985210141682,51.4214803633902));
#21075=CARTESIAN_POINT('Ctrl Pts',(33.6686262364557,-32.0004179151258,51.2285196366098));
#21076=CARTESIAN_POINT('Ctrl Pts',(33.6687027575733,-32.023143742516,51.2269932938115));
#21077=CARTESIAN_POINT('Ctrl Pts',(33.6682786564179,-32.0458666491388,51.2254669510132));
#21078=CARTESIAN_POINT('Ctrl Pts',(33.6673450516818,-32.0685686027211,51.2239406082148));
#21079=CARTESIAN_POINT('Ctrl Pts',(33.6446871232761,-32.6195290028056,51.1868973451416));
#21080=CARTESIAN_POINT('Ctrl Pts',(33.3219322677286,-33.1581480900158,51.1498540820684));
#21081=CARTESIAN_POINT('Ctrl Pts',(32.8467713568352,-33.4379566905658,51.1128108189952));
#21082=CARTESIAN_POINT('Ctrl Pts',(32.3716104459418,-33.7177652911157,51.0757675559219));
#21083=CARTESIAN_POINT('Ctrl Pts',(31.7440434797025,-33.7387634050054,51.0387242928486));
#21084=CARTESIAN_POINT('Ctrl Pts',(31.251241699047,-33.491342409186,51.0016810297754));
#21085=CARTESIAN_POINT('Ctrl Pts',(30.7584399183916,-33.2439214133666,50.9646377667021));
#21086=CARTESIAN_POINT('Ctrl Pts',(30.4004033233201,-32.7280813078381,50.9275945036289));
#21087=CARTESIAN_POINT('Ctrl Pts',(30.340967518355,-32.179867727859,50.8905512405557));
#21088=CARTESIAN_POINT('Ctrl Pts',(30.2815317133899,-31.6316541478799,50.8535079774824));
#21089=CARTESIAN_POINT('Ctrl Pts',(30.5206966985314,-31.0510670934503,50.8164647144092));
#21090=CARTESIAN_POINT('Ctrl Pts',(30.9490218734015,-30.7037800525773,50.7794214513359));
#21091=CARTESIAN_POINT('Ctrl Pts',(31.3773470482717,-30.3564930117043,50.7423781882627));
#21092=CARTESIAN_POINT('Ctrl Pts',(31.9948324128706,-30.242505984388,50.7053349251895));
#21093=CARTESIAN_POINT('Ctrl Pts',(32.5189200125302,-30.4139788162581,50.6682916621163));
#21094=CARTESIAN_POINT('Ctrl Pts',(33.0430076121899,-30.5854516481282,50.631248399043));
#21095=CARTESIAN_POINT('Ctrl Pts',(33.4736974469104,-31.0423843391848,50.5942051359697));
#21096=CARTESIAN_POINT('Ctrl Pts',(33.6139081836433,-31.5756869676153,50.5571618728965));
#21097=CARTESIAN_POINT('Ctrl Pts',(33.6500456502904,-31.7131386806355,50.5476144608009));
#21098=CARTESIAN_POINT('Ctrl Pts',(33.6668870964128,-31.8556635155748,50.5380670487053));
#21099=CARTESIAN_POINT('Ctrl Pts',(33.6656097964572,-31.9984850050081,50.5285196366098));
#21100=CARTESIAN_POINT('Origin',(32.,-32.,48.));
#21101=CARTESIAN_POINT('',(33.6634354342081,-32.000507607353,49.8285196366098));
#21102=CARTESIAN_POINT('',(33.6665861374632,-32.0014707565485,50.0214803633902));
#21103=CARTESIAN_POINT('',(33.666,-32.,48.));
#21104=CARTESIAN_POINT('Ctrl Pts',(33.6665861374632,-32.0014707565485,50.0214803633902));
#21105=CARTESIAN_POINT('Ctrl Pts',(33.6625139716522,-31.5584612743337,50.05113936803));
#21106=CARTESIAN_POINT('Ctrl Pts',(33.4805422623644,-31.1124970258842,50.0807983726698));
#21107=CARTESIAN_POINT('Ctrl Pts',(33.1642404300765,-30.8044727727622,50.1104573773096));
#21108=CARTESIAN_POINT('Ctrl Pts',(32.7691883328704,-30.4197591392497,50.1475006403828));
#21109=CARTESIAN_POINT('Ctrl Pts',(32.164590541927,-30.2502223504349,50.1845439034561));
#21110=CARTESIAN_POINT('Ctrl Pts',(31.6271077280869,-30.3734415216048,50.2215871665293));
#21111=CARTESIAN_POINT('Ctrl Pts',(31.0896249142469,-30.4966606927747,50.2586304296025));
#21112=CARTESIAN_POINT('Ctrl Pts',(30.6192570775103,-30.9126358239292,50.2956736926758));
#21113=CARTESIAN_POINT('Ctrl Pts',(30.4312419895041,-31.4310189505827,50.332716955749));
#21114=CARTESIAN_POINT('Ctrl Pts',(30.2432269014979,-31.9494020772363,50.3697602188223));
#21115=CARTESIAN_POINT('Ctrl Pts',(30.3375645622221,-32.5701931993888,50.4068034818955));
#21116=CARTESIAN_POINT('Ctrl Pts',(30.6710865696546,-33.0093216656442,50.4438467449688));
#21117=CARTESIAN_POINT('Ctrl Pts',(31.0046085770871,-33.4484501318996,50.480890008042));
#21118=CARTESIAN_POINT('Ctrl Pts',(31.5773149312279,-33.7059159422579,50.5179332711152));
#21119=CARTESIAN_POINT('Ctrl Pts',(32.1271383097918,-33.663904137947,50.5549765341885));
#21120=CARTESIAN_POINT('Ctrl Pts',(32.6769616883557,-33.621892333636,50.5920197972617));
#21121=CARTESIAN_POINT('Ctrl Pts',(33.2039020913427,-33.2804029146558,50.629063060335));
#21122=CARTESIAN_POINT('Ctrl Pts',(33.4668344475638,-32.7956995874872,50.6661063234082));
#21123=CARTESIAN_POINT('Ctrl Pts',(33.5978490648701,-32.554180354827,50.6845643367355));
#21124=CARTESIAN_POINT('Ctrl Pts',(33.6633142999988,-32.2771031787025,50.7030223500629));
#21125=CARTESIAN_POINT('Ctrl Pts',(33.6632910498763,-32.0000156711391,50.7214803633902));
#21126=CARTESIAN_POINT('Ctrl Pts',(33.6656097964572,-31.9984850050081,50.5285196366098));
#21127=CARTESIAN_POINT('Ctrl Pts',(33.6619312656801,-32.4098004851152,50.5010237856321));
#21128=CARTESIAN_POINT('Ctrl Pts',(33.5079762138442,-32.8235764117193,50.4735279346545));
#21129=CARTESIAN_POINT('Ctrl Pts',(33.231865087192,-33.1257218047281,50.4460320836768));
#21130=CARTESIAN_POINT('Ctrl Pts',(32.8598796152629,-33.5327814476059,50.4089888206036));
#21131=CARTESIAN_POINT('Ctrl Pts',(32.2661770326593,-33.737228167557,50.3719455575303));
#21132=CARTESIAN_POINT('Ctrl Pts',(31.722432421963,-33.6455082540982,50.334902294457));
#21133=CARTESIAN_POINT('Ctrl Pts',(31.1786878112666,-33.5537883406393,50.2978590313838));
#21134=CARTESIAN_POINT('Ctrl Pts',(30.6849011724773,-33.1659017937705,50.2608157683106));
#21135=CARTESIAN_POINT('Ctrl Pts',(30.4670265940585,-32.6593433941116,50.2237725052373));
#21136=CARTESIAN_POINT('Ctrl Pts',(30.2491520156396,-32.1527849944527,50.1867292421641));
#21137=CARTESIAN_POINT('Ctrl Pts',(30.3071894975912,-31.5275547420038,50.1496859790908));
#21138=CARTESIAN_POINT('Ctrl Pts',(30.6145814028672,-31.0697546101155,50.1126427160176));
#21139=CARTESIAN_POINT('Ctrl Pts',(30.9219733081434,-30.6119544782272,50.0755994529443));
#21140=CARTESIAN_POINT('Ctrl Pts',(31.4787196367441,-30.3215844668996,50.0385561898711));
#21141=CARTESIAN_POINT('Ctrl Pts',(32.0300562875329,-30.3315163188504,50.0015129267979));
#21142=CARTESIAN_POINT('Ctrl Pts',(32.5813929383217,-30.3414481708013,49.9644696637246));
#21143=CARTESIAN_POINT('Ctrl Pts',(33.1273199112987,-30.6516818860305,49.9274264006514));
#21144=CARTESIAN_POINT('Ctrl Pts',(33.4180239837953,-31.1202561986215,49.8903831375781));
#21145=CARTESIAN_POINT('Ctrl Pts',(33.5798525249692,-31.3811011767704,49.8697619705887));
#21146=CARTESIAN_POINT('Ctrl Pts',(33.6625899605592,-31.6910143728597,49.8491408035992));
#21147=CARTESIAN_POINT('Ctrl Pts',(33.6634354342081,-32.000507607353,49.8285196366098));
#21148=CARTESIAN_POINT('Origin',(32.,-32.,48.));
#21149=CARTESIAN_POINT('',(33.6674693081957,-32.0012453487566,49.1285196366098));
#21150=CARTESIAN_POINT('',(33.6680839806342,-31.999059079215,49.3214803633902));
#21151=CARTESIAN_POINT('',(33.666,-32.,48.));
#21152=CARTESIAN_POINT('Ctrl Pts',(33.6680839806342,-31.999059079215,49.3214803633902));
#21153=CARTESIAN_POINT('Ctrl Pts',(33.6684556670003,-31.9440785511347,49.3251698598506));
#21154=CARTESIAN_POINT('Ctrl Pts',(33.6659729369783,-31.8891320008961,49.328859356311));
#21155=CARTESIAN_POINT('Ctrl Pts',(33.6605253939354,-31.8344809793795,49.3325488527715));
#21156=CARTESIAN_POINT('Ctrl Pts',(33.6058310007557,-31.2857740788653,49.3695921158447));
#21157=CARTESIAN_POINT('Ctrl Pts',(33.2522671158011,-30.7668581022072,49.4066353789179));
#21158=CARTESIAN_POINT('Ctrl Pts',(32.7616226557065,-30.5151861866193,49.4436786419912));
#21159=CARTESIAN_POINT('Ctrl Pts',(32.2709781956119,-30.2635142710314,49.4807219050645));
#21160=CARTESIAN_POINT('Ctrl Pts',(31.6432531603773,-30.2790864165136,49.5177651681377));
#21161=CARTESIAN_POINT('Ctrl Pts',(31.1656911224287,-30.5547768937298,49.5548084312109));
#21162=CARTESIAN_POINT('Ctrl Pts',(30.6881290844802,-30.830467370946,49.5918516942842));
#21163=CARTESIAN_POINT('Ctrl Pts',(30.3607300438178,-31.3662761798961,49.6288949573574));
#21164=CARTESIAN_POINT('Ctrl Pts',(30.3333100262012,-31.9170201149068,49.6659382204307));
#21165=CARTESIAN_POINT('Ctrl Pts',(30.3058900085846,-32.4677640499176,49.7029814835039));
#21166=CARTESIAN_POINT('Ctrl Pts',(30.5784490140139,-33.033443110989,49.7400247465772));
#21167=CARTESIAN_POINT('Ctrl Pts',(31.0262655194942,-33.3552056270417,49.7770680096504));
#21168=CARTESIAN_POINT('Ctrl Pts',(31.4740820249745,-33.6769681430945,49.8141112727237));
#21169=CARTESIAN_POINT('Ctrl Pts',(32.097156030506,-33.7548141141286,49.8511545357969));
#21170=CARTESIAN_POINT('Ctrl Pts',(32.6103722496354,-33.5531216459011,49.8881977988701));
#21171=CARTESIAN_POINT('Ctrl Pts',(33.1235884687648,-33.3514291776736,49.9252410619434));
#21172=CARTESIAN_POINT('Ctrl Pts',(33.5269469014922,-32.8701982701844,49.9622843250166));
#21173=CARTESIAN_POINT('Ctrl Pts',(33.6358729161216,-32.3296375773346,49.9993275880899));
#21174=CARTESIAN_POINT('Ctrl Pts',(33.6575863877605,-32.2218814153821,50.0067118465233));
#21175=CARTESIAN_POINT('Ctrl Pts',(33.6675999922806,-32.1117676645154,50.0140961049568));
#21176=CARTESIAN_POINT('Ctrl Pts',(33.6665861374632,-32.0014707565485,50.0214803633902));
#21177=CARTESIAN_POINT('Ctrl Pts',(33.6634354342081,-32.000507607353,49.8285196366098));
#21178=CARTESIAN_POINT('Ctrl Pts',(33.6641087447684,-32.2469789945802,49.812097540526));
#21179=CARTESIAN_POINT('Ctrl Pts',(33.6128456395138,-32.493184039427,49.7956754444422));
#21180=CARTESIAN_POINT('Ctrl Pts',(33.508231507918,-32.7141280649899,49.7792533483584));
#21181=CARTESIAN_POINT('Ctrl Pts',(33.2722537875278,-33.2125107088145,49.7422100852852));
#21182=CARTESIAN_POINT('Ctrl Pts',(32.7648171747314,-33.5823610865111,49.7051668222119));
#21183=CARTESIAN_POINT('Ctrl Pts',(32.2181219120838,-33.6544376706759,49.6681235591386));
#21184=CARTESIAN_POINT('Ctrl Pts',(31.6714266494361,-33.7265142548407,49.6310802960654));
#21185=CARTESIAN_POINT('Ctrl Pts',(31.0854727369374,-33.5008170454736,49.5940370329922));
#21186=CARTESIAN_POINT('Ctrl Pts',(30.7283895077441,-33.0806238617888,49.556993769919));
#21187=CARTESIAN_POINT('Ctrl Pts',(30.3713062785509,-32.6604306781041,49.5199505068457));
#21188=CARTESIAN_POINT('Ctrl Pts',(30.2430937326631,-32.0457415201017,49.4829072437725));
#21189=CARTESIAN_POINT('Ctrl Pts',(30.4024212358755,-31.5178348134704,49.4458639806992));
#21190=CARTESIAN_POINT('Ctrl Pts',(30.5617487390879,-30.9899281068391,49.408820717626));
#21191=CARTESIAN_POINT('Ctrl Pts',(31.0086162914005,-30.5488038515789,49.3717774545528));
#21192=CARTESIAN_POINT('Ctrl Pts',(31.5385397239134,-30.3963181150002,49.3347341914795));
#21193=CARTESIAN_POINT('Ctrl Pts',(32.0684631564263,-30.2438323784214,49.2976909284063));
#21194=CARTESIAN_POINT('Ctrl Pts',(32.6814424691395,-30.3799851605242,49.260647665333));
#21195=CARTESIAN_POINT('Ctrl Pts',(33.0969816522974,-30.7424736864759,49.2236044022598));
#21196=CARTESIAN_POINT('Ctrl Pts',(33.4525248970599,-31.0526257778542,49.1919094803764));
#21197=CARTESIAN_POINT('Ctrl Pts',(33.6635253872144,-31.5284746399745,49.1602145584931));
#21198=CARTESIAN_POINT('Ctrl Pts',(33.6674693081957,-32.0012453487566,49.1285196366098));
#21199=CARTESIAN_POINT('Origin',(32.,-32.,48.));
#21200=CARTESIAN_POINT('',(33.6673134814248,-31.9986999266192,48.4285196366098));
#21201=CARTESIAN_POINT('',(33.6637466903966,-31.9991286486337,48.6214803633902));
#21202=CARTESIAN_POINT('',(33.666,-32.,48.));
#21203=CARTESIAN_POINT('Ctrl Pts',(33.6637466903966,-31.9991286486337,48.6214803633902));
#21204=CARTESIAN_POINT('Ctrl Pts',(33.6647970901213,-31.7776577039004,48.6362436147445));
#21205=CARTESIAN_POINT('Ctrl Pts',(33.6236994106997,-31.5565607626247,48.6510068660988));
#21206=CARTESIAN_POINT('Ctrl Pts',(33.5386159953374,-31.353933479444,48.6657701174531));
#21207=CARTESIAN_POINT('Ctrl Pts',(33.3251286501182,-30.8455105327269,48.7028133805264));
#21208=CARTESIAN_POINT('Ctrl Pts',(32.8347136636581,-30.4533698020822,48.7398566435996));
#21209=CARTESIAN_POINT('Ctrl Pts',(32.2917822745966,-30.3569527595584,48.7768999066729));
#21210=CARTESIAN_POINT('Ctrl Pts',(31.7488508855352,-30.2605357170346,48.8139431697461));
#21211=CARTESIAN_POINT('Ctrl Pts',(31.1534030938725,-30.4598423626317,48.8509864328193));
#21212=CARTESIAN_POINT('Ctrl Pts',(30.7779125803921,-30.8636710560197,48.8880296958926));
#21213=CARTESIAN_POINT('Ctrl Pts',(30.4024220669116,-31.2674997494077,48.9250729589658));
#21214=CARTESIAN_POINT('Ctrl Pts',(30.2468888316136,-31.8758504905866,48.962116222039));
#21215=CARTESIAN_POINT('Ctrl Pts',(30.3824840396265,-32.4103452790375,48.9991594851123));
#21216=CARTESIAN_POINT('Ctrl Pts',(30.5180792476393,-32.9448400674884,49.0362027481855));
#21217=CARTESIAN_POINT('Ctrl Pts',(30.9448028989631,-33.4054789032113,49.0732460112588));
#21218=CARTESIAN_POINT('Ctrl Pts',(31.4673885645646,-33.5814759526894,49.110289274332));
#21219=CARTESIAN_POINT('Ctrl Pts',(31.9899742301661,-33.7574730021676,49.1473325374053));
#21220=CARTESIAN_POINT('Ctrl Pts',(32.6084219100455,-33.648828265401,49.1843758004785));
#21221=CARTESIAN_POINT('Ctrl Pts',(33.0397332992827,-33.3052569848326,49.2214190635518));
#21222=CARTESIAN_POINT('Ctrl Pts',(33.4280862201802,-32.9959052874864,49.2547728301646));
#21223=CARTESIAN_POINT('Ctrl Pts',(33.6647238634908,-32.4960937617278,49.2881265967774));
#21224=CARTESIAN_POINT('Ctrl Pts',(33.6680839806342,-31.999059079215,49.3214803633902));
#21225=CARTESIAN_POINT('Ctrl Pts',(33.6674693081957,-32.0012453487566,49.1285196366098));
#21226=CARTESIAN_POINT('Ctrl Pts',(33.6681348228517,-32.0810227675013,49.1231712954199));
#21227=CARTESIAN_POINT('Ctrl Pts',(33.6629044681521,-32.1607125368175,49.11782295423));
#21228=CARTESIAN_POINT('Ctrl Pts',(33.6514778687695,-32.2395037027839,49.11247461304));
#21229=CARTESIAN_POINT('Ctrl Pts',(33.5723358484811,-32.7852209233395,49.0754313499668));
#21230=CARTESIAN_POINT('Ctrl Pts',(33.1959527543017,-33.2878310946498,49.0383880868936));
#21231=CARTESIAN_POINT('Ctrl Pts',(32.6945594492755,-33.5173425276136,49.0013448238203));
#21232=CARTESIAN_POINT('Ctrl Pts',(32.1931661442492,-33.7468539605773,48.9643015607471));
#21233=CARTESIAN_POINT('Ctrl Pts',(31.5667626283762,-33.7032666551944,48.9272582976738));
#21234=CARTESIAN_POINT('Ctrl Pts',(31.1019877539881,-33.4065259260658,48.8902150346006));
#21235=CARTESIAN_POINT('Ctrl Pts',(30.6372128796001,-33.1097851969372,48.8531717715273));
#21236=CARTESIAN_POINT('Ctrl Pts',(30.3340666466971,-32.5598910440628,48.8161285084541));
#21237=CARTESIAN_POINT('Ctrl Pts',(30.3312671277136,-32.0084720501211,48.7790852453809));
#21238=CARTESIAN_POINT('Ctrl Pts',(30.32846760873,-31.4570530561794,48.7420419823076));
#21239=CARTESIAN_POINT('Ctrl Pts',(30.6260148036659,-30.9041092211704,48.7049987192344));
#21240=CARTESIAN_POINT('Ctrl Pts',(31.0877527295011,-30.6026646457811,48.6679554561611));
#21241=CARTESIAN_POINT('Ctrl Pts',(31.5494906553363,-30.3012200703919,48.6309121930879));
#21242=CARTESIAN_POINT('Ctrl Pts',(32.1754193120707,-30.2512747546223,48.5938689300147));
#21243=CARTESIAN_POINT('Ctrl Pts',(32.6791171403395,-30.4756834041513,48.5568256669414));
#21244=CARTESIAN_POINT('Ctrl Pts',(33.1828149686084,-30.7000920536804,48.5197824038682));
#21245=CARTESIAN_POINT('Ctrl Pts',(33.5642819684116,-31.1988546685082,48.4827391407949));
#21246=CARTESIAN_POINT('Ctrl Pts',(33.6489609090579,-31.7437401805171,48.4456958777217));
#21247=CARTESIAN_POINT('Ctrl Pts',(33.6620489020421,-31.8279577876803,48.4399704640177));
#21248=CARTESIAN_POINT('Ctrl Pts',(33.6680469690924,-31.9132772178947,48.4342450503137));
#21249=CARTESIAN_POINT('Ctrl Pts',(33.6673134814248,-31.9986999266192,48.4285196366098));
#21250=CARTESIAN_POINT('Origin',(32.,-32.,48.));
#21251=CARTESIAN_POINT('',(33.6633884171911,-31.9995809948869,47.7285196366098));
#21252=CARTESIAN_POINT('',(33.6649068066772,-32.0014151417835,47.9214803633902));
#21253=CARTESIAN_POINT('',(33.666,-32.,48.));
#21254=CARTESIAN_POINT('Ctrl Pts',(33.6649068066772,-32.0014151417835,47.9214803633902));
#21255=CARTESIAN_POINT('Ctrl Pts',(33.6617820842682,-31.6145003896715,47.9473173696384));
#21256=CARTESIAN_POINT('Ctrl Pts',(33.5274209283347,-31.2256285879447,47.9731543758866));
#21257=CARTESIAN_POINT('Ctrl Pts',(33.2809047305485,-30.9304093300005,47.9989913821348));
#21258=CARTESIAN_POINT('Ctrl Pts',(32.927467328448,-30.5071449420422,48.036034645208));
#21259=CARTESIAN_POINT('Ctrl Pts',(32.3434864205215,-30.2763907205152,48.0730779082812));
#21260=CARTESIAN_POINT('Ctrl Pts',(31.7961885037315,-30.3437385459776,48.1101211713545));
#21261=CARTESIAN_POINT('Ctrl Pts',(31.2488905869415,-30.41108637144,48.1471644344277));
#21262=CARTESIAN_POINT('Ctrl Pts',(30.7382756612879,-30.7765362438918,48.184207697501));
#21263=CARTESIAN_POINT('Ctrl Pts',(30.4979983480558,-31.2728602832685,48.2212509605742));
#21264=CARTESIAN_POINT('Ctrl Pts',(30.2577210348237,-31.7691843226452,48.2582942236475));
#21265=CARTESIAN_POINT('Ctrl Pts',(30.2877813340129,-32.3963825289467,48.2953374867207));
#21266=CARTESIAN_POINT('Ctrl Pts',(30.5744238157098,-32.8674524038101,48.3323807497939));
#21267=CARTESIAN_POINT('Ctrl Pts',(30.8610662974067,-33.3385222786736,48.3694240128672));
#21268=CARTESIAN_POINT('Ctrl Pts',(31.4042909616111,-33.6534638220991,48.4064672759405));
#21269=CARTESIAN_POINT('Ctrl Pts',(31.9555211474962,-33.6681614915144,48.4435105390137));
#21270=CARTESIAN_POINT('Ctrl Pts',(32.5067513333814,-33.6828591609297,48.4805538020869));
#21271=CARTESIAN_POINT('Ctrl Pts',(33.0659870409472,-33.3973129563348,48.5175970651601));
#21272=CARTESIAN_POINT('Ctrl Pts',(33.377325042741,-32.9421872726427,48.5546403282334));
#21273=CARTESIAN_POINT('Ctrl Pts',(33.5645821511335,-32.6684477387846,48.5769203399523));
#21274=CARTESIAN_POINT('Ctrl Pts',(33.662161476028,-32.3333622890182,48.5992003516713));
#21275=CARTESIAN_POINT('Ctrl Pts',(33.6637466903966,-31.9991286486337,48.6214803633902));
#21276=CARTESIAN_POINT('Ctrl Pts',(33.6673134814248,-31.9986999266192,48.4285196366098));
#21277=CARTESIAN_POINT('Ctrl Pts',(33.6633013248413,-32.4659597025715,48.3972017872405));
#21278=CARTESIAN_POINT('Ctrl Pts',(33.4578770968944,-32.9363096322133,48.3658839378713));
#21279=CARTESIAN_POINT('Ctrl Pts',(33.1096935360429,-33.2463231646516,48.334566088502));
#21280=CARTESIAN_POINT('Ctrl Pts',(32.6978563408921,-33.6130122275871,48.2975228254288));
#21281=CARTESIAN_POINT('Ctrl Pts',(32.0862910691011,-33.755381944268,48.2604795623554));
#21282=CARTESIAN_POINT('Ctrl Pts',(31.5548466729667,-33.6082847043089,48.2234362992822));
#21283=CARTESIAN_POINT('Ctrl Pts',(31.0234022768324,-33.4611874643497,48.1863930362089));
#21284=CARTESIAN_POINT('Ctrl Pts',(30.5720787563548,-33.0246232677504,48.1493497731358));
#21285=CARTESIAN_POINT('Ctrl Pts',(30.4073993073046,-32.498361523704,48.1123065100625));
#21286=CARTESIAN_POINT('Ctrl Pts',(30.2427198582543,-31.9720997796577,48.0752632469893));
#21287=CARTESIAN_POINT('Ctrl Pts',(30.3646844806315,-31.3561404881642,48.038219983916));
#21288=CARTESIAN_POINT('Ctrl Pts',(30.7174828245619,-30.9323432811109,48.0011767208428));
#21289=CARTESIAN_POINT('Ctrl Pts',(31.0702811684923,-30.5085460740576,47.9641334577695));
#21290=CARTESIAN_POINT('Ctrl Pts',(31.653913233976,-30.2769109514445,47.9270901946963));
#21291=CARTESIAN_POINT('Ctrl Pts',(32.2013121524606,-30.3434328893901,47.8900469316231));
#21292=CARTESIAN_POINT('Ctrl Pts',(32.7487110709453,-30.4099548273358,47.8530036685498));
#21293=CARTESIAN_POINT('Ctrl Pts',(33.2598768424309,-30.7746338258402,47.8159604054765));
#21294=CARTESIAN_POINT('Ctrl Pts',(33.5009027815667,-31.2705947525773,47.7789171424033));
#21295=CARTESIAN_POINT('Ctrl Pts',(33.610208362449,-31.4955136861422,47.7621179738054));
#21296=CARTESIAN_POINT('Ctrl Pts',(33.6639560548541,-31.747432513297,47.7453188052076));
#21297=CARTESIAN_POINT('Ctrl Pts',(33.6633884171911,-31.9995809948869,47.7285196366098));
#21298=CARTESIAN_POINT('Origin',(32.,-32.,48.));
#21299=CARTESIAN_POINT('',(33.6657775986594,-32.0015218249574,47.0285196366098));
#21300=CARTESIAN_POINT('',(33.6687537257198,-32.0000368502801,47.2214803633902));
#21301=CARTESIAN_POINT('',(33.666,-32.,48.));
#21302=CARTESIAN_POINT('Ctrl Pts',(33.6687533332126,-32.0000368450276,47.2214803633902));
#21303=CARTESIAN_POINT('Ctrl Pts',(33.6685745432646,-31.4505822546247,47.2583911245323));
#21304=CARTESIAN_POINT('Ctrl Pts',(33.3706768056139,-30.9009615283162,47.2953018856743));
#21305=CARTESIAN_POINT('Ctrl Pts',(32.9101378018718,-30.6012897685026,47.3322126468164));
#21306=CARTESIAN_POINT('Ctrl Pts',(32.4479455591964,-30.300542249597,47.3692559098897));
#21307=CARTESIAN_POINT('Ctrl Pts',(31.8219422581151,-30.2515414474562,47.4062991729629));
#21308=CARTESIAN_POINT('Ctrl Pts',(31.318583614841,-30.4767098634442,47.4433424360361));
#21309=CARTESIAN_POINT('Ctrl Pts',(30.815224971567,-30.7018782794321,47.4803856991094));
#21310=CARTESIAN_POINT('Ctrl Pts',(30.4345109861002,-31.2012159135488,47.5174289621826));
#21311=CARTESIAN_POINT('Ctrl Pts',(30.3506543138547,-31.7462285719679,47.5544722252559));
#21312=CARTESIAN_POINT('Ctrl Pts',(30.2667976416092,-32.2912412303871,47.5915154883291));
#21313=CARTESIAN_POINT('Ctrl Pts',(30.479798282585,-32.8819289131088,47.6285587514023));
#21314=CARTESIAN_POINT('Ctrl Pts',(30.8921882984194,-33.2479961393901,47.6656020144756));
#21315=CARTESIAN_POINT('Ctrl Pts',(31.3045783142539,-33.6140633656714,47.7026452775488));
#21316=CARTESIAN_POINT('Ctrl Pts',(31.9163577049469,-33.7555101355125,47.7396885406221));
#21317=CARTESIAN_POINT('Ctrl Pts',(32.4475795385531,-33.6076111739971,47.7767318036953));
#21318=CARTESIAN_POINT('Ctrl Pts',(32.9788013721592,-33.4597122124816,47.8137750667686));
#21319=CARTESIAN_POINT('Ctrl Pts',(33.4294656486784,-33.0224675196098,47.8508183298418));
#21320=CARTESIAN_POINT('Ctrl Pts',(33.5933508388009,-32.4959578959791,47.887861592915));
#21321=CARTESIAN_POINT('Ctrl Pts',(33.6429290718713,-32.3366792154913,47.8990678497401));
#21322=CARTESIAN_POINT('Ctrl Pts',(33.6662620891541,-32.1692312594838,47.9102741065651));
#21323=CARTESIAN_POINT('Ctrl Pts',(33.6649068066772,-32.0014151417835,47.9214803633902));
#21324=CARTESIAN_POINT('Ctrl Pts',(33.6633884171911,-31.9995809948869,47.7285196366098));
#21325=CARTESIAN_POINT('Ctrl Pts',(33.6627043767632,-32.3034363704314,47.7082755421344));
#21326=CARTESIAN_POINT('Ctrl Pts',(33.5831445764217,-32.6076252460772,47.688031447659));
#21327=CARTESIAN_POINT('Ctrl Pts',(33.4268834615959,-32.8653003881351,47.6677873531836));
#21328=CARTESIAN_POINT('Ctrl Pts',(33.1409520957033,-33.3368022419862,47.6307440901104));
#21329=CARTESIAN_POINT('Ctrl Pts',(32.598203257132,-33.6525630947185,47.5937008270371));
#21330=CARTESIAN_POINT('Ctrl Pts',(32.0469958714793,-33.6680924922637,47.5566575639639));
#21331=CARTESIAN_POINT('Ctrl Pts',(31.4957884858266,-33.6836218898089,47.5196143008906));
#21332=CARTESIAN_POINT('Ctrl Pts',(30.9361225530924,-33.398919832167,47.4825710378174));
#21333=CARTESIAN_POINT('Ctrl Pts',(30.6240981694338,-32.9442644371823,47.4455277747442));
#21334=CARTESIAN_POINT('Ctrl Pts',(30.3120737857752,-32.4896090421976,47.4084845116709));
#21335=CARTESIAN_POINT('Ctrl Pts',(30.2476909511922,-31.8650003098702,47.3714412485976));
#21336=CARTESIAN_POINT('Ctrl Pts',(30.4604109016885,-31.3562558093131,47.3343979855244));
#21337=CARTESIAN_POINT('Ctrl Pts',(30.6731308521849,-30.8475113087561,47.2973547224512));
#21338=CARTESIAN_POINT('Ctrl Pts',(31.1629535877605,-30.4546310399694,47.260311459378));
#21339=CARTESIAN_POINT('Ctrl Pts',(31.7057388805693,-30.3573948836455,47.2232681963047));
#21340=CARTESIAN_POINT('Ctrl Pts',(32.2485241733781,-30.2601587273215,47.1862249332315));
#21341=CARTESIAN_POINT('Ctrl Pts',(32.8442720234201,-30.4585666834602,47.1491816701582));
#21342=CARTESIAN_POINT('Ctrl Pts',(33.2203714448242,-30.8618283471548,47.112138407085));
#21343=CARTESIAN_POINT('Ctrl Pts',(33.503364613578,-31.165259539949,47.0842654835932));
#21344=CARTESIAN_POINT('Ctrl Pts',(33.6619995116097,-31.584672681627,47.0563925601015));
#21345=CARTESIAN_POINT('Ctrl Pts',(33.6657775986594,-32.0015218249574,47.0285196366098));
#21346=CARTESIAN_POINT('Origin',(32.,-32.,48.));
#21347=CARTESIAN_POINT('',(33.6685587644994,-31.9994832045425,46.3285196366098));
#21348=CARTESIAN_POINT('',(33.6650141741342,-31.9985615245759,46.5214803633902));
#21349=CARTESIAN_POINT('',(33.666,-32.,48.));
#21350=CARTESIAN_POINT('Ctrl Pts',(33.6650141741342,-31.9985615245759,46.5214803633902));
#21351=CARTESIAN_POINT('Ctrl Pts',(33.6663655706979,-31.8347406294782,46.5324216163529));
#21352=CARTESIAN_POINT('Ctrl Pts',(33.6441442554494,-31.6712783426402,46.5433628693156));
#21353=CARTESIAN_POINT('Ctrl Pts',(33.5968493993272,-31.5154247984472,46.5543041222783));
#21354=CARTESIAN_POINT('Ctrl Pts',(33.436725526557,-30.9877591043886,46.5913473853516));
#21355=CARTESIAN_POINT('Ctrl Pts',(32.9891928793346,-30.5473096280065,46.6283906484248));
#21356=CARTESIAN_POINT('Ctrl Pts',(32.4590399703841,-30.3956236614555,46.665433911498));
#21357=CARTESIAN_POINT('Ctrl Pts',(31.9288870614335,-30.2439376949046,46.7024771745713));
#21358=CARTESIAN_POINT('Ctrl Pts',(31.3161138907549,-30.3810152381847,46.7395204376445));
#21359=CARTESIAN_POINT('Ctrl Pts',(30.9011221386267,-30.7441303507629,46.7765637007178));
#21360=CARTESIAN_POINT('Ctrl Pts',(30.4861303864983,-31.1072454633411,46.813606963791));
#21361=CARTESIAN_POINT('Ctrl Pts',(30.2689200529203,-31.6963981452175,46.8506502268642));
#21362=CARTESIAN_POINT('Ctrl Pts',(30.3488854087639,-32.2419953237128,46.8876934899375));
#21363=CARTESIAN_POINT('Ctrl Pts',(30.4288507646075,-32.7875925022081,46.9247367530107));
#21364=CARTESIAN_POINT('Ctrl Pts',(30.8059918098727,-33.2896341773223,46.961780016084));
#21365=CARTESIAN_POINT('Ctrl Pts',(31.3077308472083,-33.5183888007308,46.9988232791572));
#21366=CARTESIAN_POINT('Ctrl Pts',(31.809469884544,-33.7471434241392,47.0358665422305));
#21367=CARTESIAN_POINT('Ctrl Pts',(32.43580691395,-33.702610995842,47.0729098053037));
#21368=CARTESIAN_POINT('Ctrl Pts',(32.9001335069413,-33.4051693135608,47.109953068377));
#21369=CARTESIAN_POINT('Ctrl Pts',(33.3644600999327,-33.1077276312796,47.1469963314502));
#21370=CARTESIAN_POINT('Ctrl Pts',(33.6667762565094,-32.5573766950145,47.1840395945234));
#21371=CARTESIAN_POINT('Ctrl Pts',(33.668743742663,-32.0059541090467,47.2210828575967));
#21372=CARTESIAN_POINT('Ctrl Pts',(33.6687507802643,-32.0039816975615,47.2212153595278));
#21373=CARTESIAN_POINT('Ctrl Pts',(33.6687539750312,-32.002009272365,47.221347861459));
#21374=CARTESIAN_POINT('Ctrl Pts',(33.6687533332126,-32.0000368450276,47.2214803633902));
#21375=CARTESIAN_POINT('Ctrl Pts',(33.6657775986594,-32.0015218249574,47.0285196366098));
#21376=CARTESIAN_POINT('Ctrl Pts',(33.6670206093262,-32.1386674028061,47.0193492970283));
#21377=CARTESIAN_POINT('Ctrl Pts',(33.6515012237676,-32.2755354419662,47.0101789574468));
#21378=CARTESIAN_POINT('Ctrl Pts',(33.6181332971531,-32.4079041643904,47.0010086178652));
#21379=CARTESIAN_POINT('Ctrl Pts',(33.4833447353118,-32.9426029466809,46.963965354792));
#21380=CARTESIAN_POINT('Ctrl Pts',(33.057316618863,-33.4038851400114,46.9269220917187));
#21381=CARTESIAN_POINT('Ctrl Pts',(32.5349971038525,-33.5806705139124,46.8898788286455));
#21382=CARTESIAN_POINT('Ctrl Pts',(32.0126775888419,-33.7574558878134,46.8528355655722));
#21383=CARTESIAN_POINT('Ctrl Pts',(31.3940666752695,-33.6497444422849,46.815792302499));
#21384=CARTESIAN_POINT('Ctrl Pts',(30.962237362908,-33.3068243507597,46.7787490394258));
#21385=CARTESIAN_POINT('Ctrl Pts',(30.5304080505466,-32.9639042592346,46.7417057763525));
#21386=CARTESIAN_POINT('Ctrl Pts',(30.285360339396,-32.3857755217127,46.7046625132793));
#21387=CARTESIAN_POINT('Ctrl Pts',(30.339226733363,-31.8369867137117,46.6676192502061));
#21388=CARTESIAN_POINT('Ctrl Pts',(30.39309312733,-31.2881979057106,46.6305759871328));
#21389=CARTESIAN_POINT('Ctrl Pts',(30.7458736264145,-30.7687490272304,46.5935327240596));
#21390=CARTESIAN_POINT('Ctrl Pts',(31.236137787108,-30.5163370684692,46.5564894609863));
#21391=CARTESIAN_POINT('Ctrl Pts',(31.7264019478016,-30.2639251097081,46.5194461979131));
#21392=CARTESIAN_POINT('Ctrl Pts',(32.3541497701043,-30.278550070666,46.4824029348399));
#21393=CARTESIAN_POINT('Ctrl Pts',(32.8321272543511,-30.5535196485092,46.4453596717666));
#21394=CARTESIAN_POINT('Ctrl Pts',(33.3101047385979,-30.8284892263525,46.4083164086934));
#21395=CARTESIAN_POINT('Ctrl Pts',(33.6383118847889,-31.363803421081,46.3712731456201));
#21396=CARTESIAN_POINT('Ctrl Pts',(33.6665628824563,-31.9145053598074,46.3342298825469));
#21397=CARTESIAN_POINT('Ctrl Pts',(33.6680145197335,-31.942802394565,46.3323264672345));
#21398=CARTESIAN_POINT('Ctrl Pts',(33.6686741912351,-31.97114005715,46.3304230519221));
#21399=CARTESIAN_POINT('Ctrl Pts',(33.6685587644994,-31.9994832045425,46.3285196366098));
#21400=CARTESIAN_POINT('Origin',(32.,-32.,48.));
#21401=CARTESIAN_POINT('',(33.6642558539866,-31.9988063630671,45.6285196366098));
#21402=CARTESIAN_POINT('',(33.6636859258726,-32.0008167215673,45.8214803633902));
#21403=CARTESIAN_POINT('',(33.666,-32.,48.));
#21404=CARTESIAN_POINT('Ctrl Pts',(33.6636859258726,-32.0008167215673,45.8214803633902));
#21405=CARTESIAN_POINT('Ctrl Pts',(33.6622209390427,-31.6705283459497,45.8434953712468));
#21406=CARTESIAN_POINT('Ctrl Pts',(33.5671083318336,-31.3394623203548,45.8655103791033));
#21407=CARTESIAN_POINT('Ctrl Pts',(33.3840133726138,-31.0676652347372,45.8875253869599));
#21408=CARTESIAN_POINT('Ctrl Pts',(33.0759310505021,-30.6103294476841,45.9245686500332));
#21409=CARTESIAN_POINT('Ctrl Pts',(32.5187472242561,-30.3207998372036,45.9616119131065));
#21410=CARTESIAN_POINT('Ctrl Pts',(31.9674261915623,-30.3315635831428,45.9986551761797));
#21411=CARTESIAN_POINT('Ctrl Pts',(31.4161051588685,-30.3423273290819,46.035698439253));
#21412=CARTESIAN_POINT('Ctrl Pts',(30.8706469197269,-30.6533844314407,46.0727417023262));
#21413=CARTESIAN_POINT('Ctrl Pts',(30.5806502067447,-31.1223968468165,46.1097849653994));
#21414=CARTESIAN_POINT('Ctrl Pts',(30.2906534937624,-31.5914092621924,46.1468282284726));
#21415=CARTESIAN_POINT('Ctrl Pts',(30.2561183069395,-32.2183769905854,46.1838714915459));
#21416=CARTESIAN_POINT('Ctrl Pts',(30.4928477605068,-32.7164029990739,46.2209147546191));
#21417=CARTESIAN_POINT('Ctrl Pts',(30.7295772140741,-33.2144290075624,46.2579580176924));
#21418=CARTESIAN_POINT('Ctrl Pts',(31.2375713080316,-33.5835132961463,46.2950012807656));
#21419=CARTESIAN_POINT('Ctrl Pts',(31.7843746994676,-33.6547648956458,46.3320445438389));
#21420=CARTESIAN_POINT('Ctrl Pts',(32.3311780909037,-33.7260164951454,46.3690878069121));
#21421=CARTESIAN_POINT('Ctrl Pts',(32.9167907798183,-33.4994354055607,46.4061310699853));
#21422=CARTESIAN_POINT('Ctrl Pts',(33.2732395751167,-33.0787039049007,46.4431743330586));
#21423=CARTESIAN_POINT('Ctrl Pts',(33.5244061648518,-32.7822414182582,46.4692763431691));
#21424=CARTESIAN_POINT('Ctrl Pts',(33.6617902136893,-32.3893809923948,46.4953783532797));
#21425=CARTESIAN_POINT('Ctrl Pts',(33.6650141741342,-31.9985615245759,46.5214803633902));
#21426=CARTESIAN_POINT('Ctrl Pts',(33.6685587644994,-31.9994832045425,46.3285196366098));
#21427=CARTESIAN_POINT('Ctrl Pts',(33.6664278170942,-32.5227394156102,46.2933797888489));
#21428=CARTESIAN_POINT('Ctrl Pts',(33.4001232888826,-33.0478649913129,46.258239941088));
#21429=CARTESIAN_POINT('Ctrl Pts',(32.9757782336594,-33.353734838659,46.2231000933271));
#21430=CARTESIAN_POINT('Ctrl Pts',(32.5284477380514,-33.67617269606,46.1860568302539));
#21431=CARTESIAN_POINT('Ctrl Pts',(31.9054918976918,-33.7549587281378,46.1490135671807));
#21432=CARTESIAN_POINT('Ctrl Pts',(31.3919719272917,-33.5540408738129,46.1119703041074));
#21433=CARTESIAN_POINT('Ctrl Pts',(30.8784519568916,-33.3531230194881,46.0749270410342));
#21434=CARTESIAN_POINT('Ctrl Pts',(30.4743678564511,-32.8725012787608,46.037883777961));
#21435=CARTESIAN_POINT('Ctrl Pts',(30.3646263192768,-32.3321055541248,46.0008405148877));
#21436=CARTESIAN_POINT('Ctrl Pts',(30.2548847821026,-31.7917098294888,45.9637972518145));
#21437=CARTESIAN_POINT('Ctrl Pts',(30.4394858081946,-31.1915401209442,45.9267539887412));
#21438=CARTESIAN_POINT('Ctrl Pts',(30.8339569689707,-30.8062308328363,45.889710725668));
#21439=CARTESIAN_POINT('Ctrl Pts',(31.2284281297467,-30.4209215447285,45.8526674625947));
#21440=CARTESIAN_POINT('Ctrl Pts',(31.8327694252067,-30.2504726770573,45.8156241995215));
#21441=CARTESIAN_POINT('Ctrl Pts',(32.3704375554525,-30.3728807074486,45.7785809364483));
#21442=CARTESIAN_POINT('Ctrl Pts',(32.9081056856982,-30.4952887378399,45.741537673375));
#21443=CARTESIAN_POINT('Ctrl Pts',(33.3791006507296,-30.9105536662937,45.7044944103018));
#21444=CARTESIAN_POINT('Ctrl Pts',(33.5678977084122,-31.4286525132299,45.6674511472285));
#21445=CARTESIAN_POINT('Ctrl Pts',(33.6340379819389,-31.6101553389139,45.6544739770223));
#21446=CARTESIAN_POINT('Ctrl Pts',(33.6655448403235,-31.8042787039313,45.641496806816));
#21447=CARTESIAN_POINT('Ctrl Pts',(33.6642558539866,-31.9988063630671,45.6285196366098));
#21448=CARTESIAN_POINT('Origin',(32.,-32.,48.));
#21449=CARTESIAN_POINT('',(33.6642508521176,-32.0011912824064,44.9285196366098));
#21450=CARTESIAN_POINT('',(33.6679951137542,-32.0009960538572,45.1214803633902));
#21451=CARTESIAN_POINT('',(33.666,-32.,48.));
#21452=CARTESIAN_POINT('Ctrl Pts',(33.6679951137542,-32.0009960538572,45.1214803633902));
#21453=CARTESIAN_POINT('Ctrl Pts',(33.6645083963353,-31.507841323258,45.1545691261407));
#21454=CARTESIAN_POINT('Ctrl Pts',(33.432088645058,-31.0118309857062,45.1876578888911));
#21455=CARTESIAN_POINT('Ctrl Pts',(33.0490210707781,-30.702195730029,45.2207466516416));
#21456=CARTESIAN_POINT('Ctrl Pts',(32.6201723696075,-30.3555553820867,45.2577899147148));
#21457=CARTESIAN_POINT('Ctrl Pts',(32.0025157192002,-30.2425002018306,45.2948331777881));
#21458=CARTESIAN_POINT('Ctrl Pts',(31.4786874536787,-30.4147636267296,45.3318764408613));
#21459=CARTESIAN_POINT('Ctrl Pts',(30.9548591881572,-30.5870270516286,45.3689197039346));
#21460=CARTESIAN_POINT('Ctrl Pts',(30.5248593075215,-31.0446090816829,45.4059629670078));
#21461=CARTESIAN_POINT('Ctrl Pts',(30.3854534255734,-31.5781226610747,45.443006230081));
#21462=CARTESIAN_POINT('Ctrl Pts',(30.2460475436252,-32.1116362404665,45.4800494931543));
#21463=CARTESIAN_POINT('Ctrl Pts',(30.3972356603645,-32.7210813691959,45.5170927562276));
#21464=CARTESIAN_POINT('Ctrl Pts',(30.7698349133548,-33.127579260935,45.5541360193008));
#21465=CARTESIAN_POINT('Ctrl Pts',(31.1424341663451,-33.534077152674,45.591179282374));
#21466=CARTESIAN_POINT('Ctrl Pts',(31.7364445555863,-33.7376278074227,45.6282225454472));
#21467=CARTESIAN_POINT('Ctrl Pts',(32.280050147849,-33.6450875492755,45.6652658085205));
#21468=CARTESIAN_POINT('Ctrl Pts',(32.8236557401117,-33.5525472911282,45.7023090715937));
#21469=CARTESIAN_POINT('Ctrl Pts',(33.3168565353959,-33.1639161200851,45.739352334667));
#21470=CARTESIAN_POINT('Ctrl Pts',(33.5339665240493,-32.6570295527506,45.7763955977403));
#21471=CARTESIAN_POINT('Ctrl Pts',(33.6220468941052,-32.4513883627525,45.7914238529569));
#21472=CARTESIAN_POINT('Ctrl Pts',(33.6646859798409,-32.2262837319,45.8064521081736));
#21473=CARTESIAN_POINT('Ctrl Pts',(33.6636859258726,-32.0008167215673,45.8214803633902));
#21474=CARTESIAN_POINT('Ctrl Pts',(33.6642558539866,-31.9988063630671,45.6285196366098));
#21475=CARTESIAN_POINT('Ctrl Pts',(33.6618654357062,-32.3595568684207,45.6044535437428));
#21476=CARTESIAN_POINT('Ctrl Pts',(33.5466851733263,-32.7216978020734,45.5803874508758));
#21477=CARTESIAN_POINT('Ctrl Pts',(33.3304348817757,-33.0073153428977,45.5563213580088));
#21478=CARTESIAN_POINT('Ctrl Pts',(32.9975758471228,-33.4469465602108,45.5192780949355));
#21479=CARTESIAN_POINT('Ctrl Pts',(32.4252586274834,-33.7052762294185,45.4822348318623));
#21480=CARTESIAN_POINT('Ctrl Pts',(31.8753724793036,-33.6640940946256,45.4451915687891));
#21481=CARTESIAN_POINT('Ctrl Pts',(31.3254863311237,-33.6229119598326,45.4081483057158));
#21482=CARTESIAN_POINT('Ctrl Pts',(30.7980312544034,-33.2822180210392,45.3711050426426));
#21483=CARTESIAN_POINT('Ctrl Pts',(30.5343678322437,-32.7979119773011,45.3340617795693));
#21484=CARTESIAN_POINT('Ctrl Pts',(30.270704410084,-32.313605933563,45.2970185164961));
#21485=CARTESIAN_POINT('Ctrl Pts',(30.270832642485,-31.6856877848803,45.2599752534229));
#21486=CARTESIAN_POINT('Ctrl Pts',(30.5346938509953,-31.2014894713457,45.2229319903496));
#21487=CARTESIAN_POINT('Ctrl Pts',(30.7985550595056,-30.7172911578112,45.1858887272764));
#21488=CARTESIAN_POINT('Ctrl Pts',(31.3261492441253,-30.3768126794248,45.1488454642031));
#21489=CARTESIAN_POINT('Ctrl Pts',(31.8760521667326,-30.3358551417286,45.1118022011299));
#21490=CARTESIAN_POINT('Ctrl Pts',(32.4259550893399,-30.2948976040324,45.0747589380566));
#21491=CARTESIAN_POINT('Ctrl Pts',(32.9981667499349,-30.5534610070264,45.0377156749834));
#21492=CARTESIAN_POINT('Ctrl Pts',(33.3308461953179,-30.9932281395021,45.0006724119102));
#21493=CARTESIAN_POINT('Ctrl Pts',(33.5468435929401,-31.2787539136153,44.97662148681));
#21494=CARTESIAN_POINT('Ctrl Pts',(33.6618671138013,-31.6406654174441,44.9525705617099));
#21495=CARTESIAN_POINT('Ctrl Pts',(33.6642508521176,-32.0011912824064,44.9285196366098));
#21496=CARTESIAN_POINT('Origin',(32.,-32.,48.));
#21497=CARTESIAN_POINT('',(33.6685557839381,-32.0005207187555,44.2285196366098));
#21498=CARTESIAN_POINT('',(33.666705446585,-31.9985486374404,44.4214803633902));
#21499=CARTESIAN_POINT('',(33.666,-32.,48.));
#21500=CARTESIAN_POINT('Ctrl Pts',(33.666705446585,-31.9985486374404,44.4214803633902));
#21501=CARTESIAN_POINT('Ctrl Pts',(33.6676776984237,-31.8922296343042,44.4285996179613));
#21502=CARTESIAN_POINT('Ctrl Pts',(33.6583758869896,-31.7860801019361,44.4357188725324));
#21503=CARTESIAN_POINT('Ctrl Pts',(33.638183541047,-31.6820443176578,44.4428381271035));
#21504=CARTESIAN_POINT('Ctrl Pts',(33.5331177121255,-31.1407200978874,44.4798813901768));
#21505=CARTESIAN_POINT('Ctrl Pts',(33.1332035875173,-30.6566230988116,44.51692465325));
#21506=CARTESIAN_POINT('Ctrl Pts',(32.6214397021988,-30.4512734823014,44.5539679163232));
#21507=CARTESIAN_POINT('Ctrl Pts',(32.1096758168802,-30.2459238657912,44.5910111793965));
#21508=CARTESIAN_POINT('Ctrl Pts',(31.4860621708514,-30.3193216318466,44.6280544424697));
#21509=CARTESIAN_POINT('Ctrl Pts',(31.035960987131,-30.6378803607033,44.665097705543));
#21510=CARTESIAN_POINT('Ctrl Pts',(30.5858598034106,-30.9564390895599,44.7021409686162));
#21511=CARTESIAN_POINT('Ctrl Pts',(30.3092710819986,-31.5201587812177,44.7391842316894));
#21512=CARTESIAN_POINT('Ctrl Pts',(30.3327603220732,-32.071084361417,44.7762274947627));
#21513=CARTESIAN_POINT('Ctrl Pts',(30.3562495621479,-32.6220099416162,44.8132707578359));
#21514=CARTESIAN_POINT('Ctrl Pts',(30.6798167637091,-33.160141410357,44.8503140209092));
#21515=CARTESIAN_POINT('Ctrl Pts',(31.1553993297926,-33.4392327254398,44.8873572839824));
#21516=CARTESIAN_POINT('Ctrl Pts',(31.6309818958761,-33.7183240405225,44.9244005470557));
#21517=CARTESIAN_POINT('Ctrl Pts',(32.258579826482,-33.7383752019473,44.9614438101289));
#21518=CARTESIAN_POINT('Ctrl Pts',(32.7510077115729,-33.490210906969,44.9984870732021));
#21519=CARTESIAN_POINT('Ctrl Pts',(33.2434355966639,-33.2420466119907,45.0355303362754));
#21520=CARTESIAN_POINT('Ctrl Pts',(33.60069343624,-32.7256668606095,45.0725735993487));
#21521=CARTESIAN_POINT('Ctrl Pts',(33.6593019800612,-32.1773642271046,45.1096168624219));
#21522=CARTESIAN_POINT('Ctrl Pts',(33.6655586509436,-32.1188309673081,45.1135713627447));
#21523=CARTESIAN_POINT('Ctrl Pts',(33.6684118179163,-32.0599339040282,45.1175258630675));
#21524=CARTESIAN_POINT('Ctrl Pts',(33.6679951137542,-32.0009960538572,45.1214803633902));
#21525=CARTESIAN_POINT('Ctrl Pts',(33.6642508521176,-32.0011912824064,44.9285196366098));
#21526=CARTESIAN_POINT('Ctrl Pts',(33.6655385503544,-32.1959477778902,44.9155272986366));
#21527=CARTESIAN_POINT('Ctrl Pts',(33.6339560104401,-32.3902999199697,44.9025349606635));
#21528=CARTESIAN_POINT('Ctrl Pts',(33.5676642183743,-32.5719878260169,44.8895426226904));
#21529=CARTESIAN_POINT('Ctrl Pts',(33.3786555658768,-33.0900095180987,44.8524993596172));
#21530=CARTESIAN_POINT('Ctrl Pts',(32.9074910307108,-33.505082040305,44.815456096544));
#21531=CARTESIAN_POINT('Ctrl Pts',(32.3697729493851,-33.6272704571109,44.7784128334707));
#21532=CARTESIAN_POINT('Ctrl Pts',(31.8320548680593,-33.7494588739168,44.7413695703975));
#21533=CARTESIAN_POINT('Ctrl Pts',(31.2277832405737,-33.5787631853222,44.7043263073242));
#21534=CARTESIAN_POINT('Ctrl Pts',(30.8334694871393,-33.1932928128699,44.667283044251));
#21535=CARTESIAN_POINT('Ctrl Pts',(30.4391557337048,-32.8078224404177,44.6302397811777));
#21536=CARTESIAN_POINT('Ctrl Pts',(30.2547998543215,-32.2075773841077,44.5931965181045));
#21537=CARTESIAN_POINT('Ctrl Pts',(30.364762099767,-31.6672265270128,44.5561532550313));
#21538=CARTESIAN_POINT('Ctrl Pts',(30.4747243452125,-31.1268756699178,44.519109991958));
#21539=CARTESIAN_POINT('Ctrl Pts',(30.8790047154868,-30.646419012038,44.4820667288848));
#21540=CARTESIAN_POINT('Ctrl Pts',(31.3926067052714,-30.4457109148541,44.4450234658115));
#21541=CARTESIAN_POINT('Ctrl Pts',(31.906208695056,-30.2450028176701,44.4079802027383));
#21542=CARTESIAN_POINT('Ctrl Pts',(32.5291323043508,-30.324043281182,44.370936939665));
#21543=CARTESIAN_POINT('Ctrl Pts',(32.9763310672053,-30.6466638178604,44.3338936765918));
#21544=CARTESIAN_POINT('Ctrl Pts',(33.4003680481787,-30.9525748572825,44.2987689965978));
#21545=CARTESIAN_POINT('Ctrl Pts',(33.6664114443341,-31.4774878746799,44.2636443166038));
#21546=CARTESIAN_POINT('Ctrl Pts',(33.6685557839381,-32.0005207187555,44.2285196366098));
#21547=CARTESIAN_POINT('Origin',(32.,-32.,48.));
#21548=CARTESIAN_POINT('',(33.6657843894837,-31.9984780271603,43.5285196366098));
#21549=CARTESIAN_POINT('',(33.6632944811816,-31.9999190856909,43.7214803633902));
#21550=CARTESIAN_POINT('',(33.666,-32.,48.));
#21551=CARTESIAN_POINT('Ctrl Pts',(33.6632944811816,-31.9999190856909,43.7214803633902));
#21552=CARTESIAN_POINT('Ctrl Pts',(33.6634128178791,-31.7268111612894,43.7396733728552));
#21553=CARTESIAN_POINT('Ctrl Pts',(33.5999067829313,-31.4537550667933,43.7578663823202));
#21554=CARTESIAN_POINT('Ctrl Pts',(33.4724751700925,-31.2147879244965,43.7760593917851));
#21555=CARTESIAN_POINT('Ctrl Pts',(33.2130083255708,-30.7282206671663,43.8131026548584));
#21556=CARTESIAN_POINT('Ctrl Pts',(32.6885181894386,-30.3829797242392,43.8501459179316));
#21557=CARTESIAN_POINT('Ctrl Pts',(32.1390086040352,-30.3370454792411,43.8871891810049));
#21558=CARTESIAN_POINT('Ctrl Pts',(31.5894990186317,-30.291111234243,43.9242324440781));
#21559=CARTESIAN_POINT('Ctrl Pts',(31.0149699839572,-30.5444836871738,43.9612757071514));
#21560=CARTESIAN_POINT('Ctrl Pts',(30.6783228710374,-30.9812209774104,43.9983189702246));
#21561=CARTESIAN_POINT('Ctrl Pts',(30.3416757581177,-31.417958267647,44.0353622332978));
#21562=CARTESIAN_POINT('Ctrl Pts',(30.2429105669527,-32.0380603951895,44.0724054963711));
#21563=CARTESIAN_POINT('Ctrl Pts',(30.4272217134811,-32.5577719888467,44.1094487594443));
#21564=CARTESIAN_POINT('Ctrl Pts',(30.6115328600096,-33.0774835825039,44.1464920225176));
#21565=CARTESIAN_POINT('Ctrl Pts',(31.0789203442315,-33.4968046422757,44.1835352855908));
#21566=CARTESIAN_POINT('Ctrl Pts',(31.6155101876733,-33.6238561248802,44.2205785486641));
#21567=CARTESIAN_POINT('Ctrl Pts',(32.1521000311151,-33.7509076074846,44.2576218117373));
#21568=CARTESIAN_POINT('Ctrl Pts',(32.7578922337768,-33.5856895129216,44.2946650748105));
#21569=CARTESIAN_POINT('Ctrl Pts',(33.1556795684902,-33.2038047454075,44.3317083378838));
#21570=CARTESIAN_POINT('Ctrl Pts',(33.4770171235125,-32.8953134818994,44.3616323463859));
#21571=CARTESIAN_POINT('Ctrl Pts',(33.6626188288084,-32.4454340131511,44.3915563548881));
#21572=CARTESIAN_POINT('Ctrl Pts',(33.666705446585,-31.9985486374404,44.4214803633902));
#21573=CARTESIAN_POINT('Ctrl Pts',(33.6685557839381,-32.0005207187555,44.2285196366098));
#21574=CARTESIAN_POINT('Ctrl Pts',(33.6686729122274,-32.0290898605868,44.2266010535306));
#21575=CARTESIAN_POINT('Ctrl Pts',(33.6680026787812,-32.0576533927864,44.2246824704513));
#21576=CARTESIAN_POINT('Ctrl Pts',(33.6665278243027,-32.0861753184357,44.2227638873721));
#21577=CARTESIAN_POINT('Ctrl Pts',(33.6380519021311,-32.6368656724877,44.1857206242988));
#21578=CARTESIAN_POINT('Ctrl Pts',(33.3096261413737,-33.1720457707468,44.1486773612256));
#21579=CARTESIAN_POINT('Ctrl Pts',(32.8315363893394,-33.4468201021218,44.1116340981523));
#21580=CARTESIAN_POINT('Ctrl Pts',(32.3534466373052,-33.7215944334968,44.0745908350791));
#21581=CARTESIAN_POINT('Ctrl Pts',(31.725692893994,-33.7359629979876,44.0375475720059));
#21582=CARTESIAN_POINT('Ctrl Pts',(31.2355318684904,-33.4833508184354,44.0005043089326));
#21583=CARTESIAN_POINT('Ctrl Pts',(30.7453708429867,-33.2307386388832,43.9634610458594));
#21584=CARTESIAN_POINT('Ctrl Pts',(30.3928025352905,-32.711145715288,43.9264177827861));
#21585=CARTESIAN_POINT('Ctrl Pts',(30.3391602912853,-32.1623349520288,43.8893745197129));
#21586=CARTESIAN_POINT('Ctrl Pts',(30.2855180472801,-31.6135241887696,43.8523312566396));
#21587=CARTESIAN_POINT('Ctrl Pts',(30.5308018669659,-31.0354955858464,43.8152879935664));
#21588=CARTESIAN_POINT('Ctrl Pts',(30.9627712044431,-30.6927518978913,43.7782447304932));
#21589=CARTESIAN_POINT('Ctrl Pts',(31.3947405419203,-30.3500082099362,43.7412014674199));
#21590=CARTESIAN_POINT('Ctrl Pts',(32.0133953971889,-30.2425494369492,43.7041582043467));
#21591=CARTESIAN_POINT('Ctrl Pts',(32.5356426630091,-30.4195481304534,43.6671149412734));
#21592=CARTESIAN_POINT('Ctrl Pts',(33.0578899288294,-30.5965468239577,43.6300716782002));
#21593=CARTESIAN_POINT('Ctrl Pts',(33.4837296052012,-31.0580029839533,43.593028415127));
#21594=CARTESIAN_POINT('Ctrl Pts',(33.618299765207,-31.5927567744109,43.5559851520537));
#21595=CARTESIAN_POINT('Ctrl Pts',(33.651558523582,-31.7249201537679,43.5468299802391));
#21596=CARTESIAN_POINT('Ctrl Pts',(33.667025905015,-31.861560712161,43.5376748084244));
#21597=CARTESIAN_POINT('Ctrl Pts',(33.6657843894837,-31.9984780271603,43.5285196366098));
#21598=CARTESIAN_POINT('Origin',(32.,-32.,48.));
#21599=CARTESIAN_POINT('',(33.6633867149896,-32.0004154269497,42.8285196366098));
#21600=CARTESIAN_POINT('',(33.6664085055627,-32.0014938638813,43.0214803633902));
#21601=CARTESIAN_POINT('',(33.666,-32.,48.));
#21602=CARTESIAN_POINT('Ctrl Pts',(33.6664085055627,-32.0014938638813,43.0214803633902));
#21603=CARTESIAN_POINT('Ctrl Pts',(33.6623727377844,-31.5642233612903,43.050747127749));
#21604=CARTESIAN_POINT('Ctrl Pts',(33.4856936746432,-31.1240664805265,43.0800138921079));
#21605=CARTESIAN_POINT('Ctrl Pts',(33.1768026773126,-30.816836196291,43.1092806564668));
#21606=CARTESIAN_POINT('Ctrl Pts',(32.7858359706835,-30.4279714723517,43.1463239195401));
#21607=CARTESIAN_POINT('Ctrl Pts',(32.183062556742,-30.2520583620278,43.1833671826133));
#21608=CARTESIAN_POINT('Ctrl Pts',(31.6443082797766,-30.3695937527617,43.2204104456865));
#21609=CARTESIAN_POINT('Ctrl Pts',(31.1055540028112,-30.4871291434957,43.2574537087597));
#21610=CARTESIAN_POINT('Ctrl Pts',(30.6308188628218,-30.8981130352873,43.294496971833));
#21611=CARTESIAN_POINT('Ctrl Pts',(30.4373390864957,-31.4144814267063,43.3315402349062));
#21612=CARTESIAN_POINT('Ctrl Pts',(30.2438593101695,-31.9308498181252,43.3685834979795));
#21613=CARTESIAN_POINT('Ctrl Pts',(30.3316348975066,-32.5526027091714,43.4056267610527));
#21614=CARTESIAN_POINT('Ctrl Pts',(30.6605002152946,-32.995229348729,43.442670024126));
#21615=CARTESIAN_POINT('Ctrl Pts',(30.9893655330827,-33.4378559882867,43.4797132871992));
#21616=CARTESIAN_POINT('Ctrl Pts',(31.5593205813218,-33.7013563763557,43.5167565502724));
#21617=CARTESIAN_POINT('Ctrl Pts',(32.1095570205873,-33.6651541638684,43.5537998133457));
#21618=CARTESIAN_POINT('Ctrl Pts',(32.6597934598528,-33.628951951381,43.5908430764189));
#21619=CARTESIAN_POINT('Ctrl Pts',(33.1903112901447,-33.2930471383373,43.6278863394922));
#21620=CARTESIAN_POINT('Ctrl Pts',(33.4583484288351,-32.8111479459487,43.6649296025654));
#21621=CARTESIAN_POINT('Ctrl Pts',(33.5947448372928,-32.5659232752123,43.6837798561737));
#21622=CARTESIAN_POINT('Ctrl Pts',(33.6631718694299,-32.2828933592601,43.7026301097819));
#21623=CARTESIAN_POINT('Ctrl Pts',(33.6632944811816,-31.9999190856909,43.7214803633902));
#21624=CARTESIAN_POINT('Ctrl Pts',(33.6657843894837,-31.9984780271603,43.5285196366098));
#21625=CARTESIAN_POINT('Ctrl Pts',(33.6620025381831,-32.4155496728804,43.5006315453512));
#21626=CARTESIAN_POINT('Ctrl Pts',(33.503177614974,-32.8351893633072,43.4727434540926));
#21627=CARTESIAN_POINT('Ctrl Pts',(33.2199064719879,-33.1386700027057,43.444855362834));
#21628=CARTESIAN_POINT('Ctrl Pts',(32.8436423751234,-33.5417780196234,43.4078120997608));
#21629=CARTESIAN_POINT('Ctrl Pts',(32.2478135377548,-33.7399426325393,43.3707688366875));
#21630=CARTESIAN_POINT('Ctrl Pts',(31.7050680049991,-33.6424847916052,43.3337255736143));
#21631=CARTESIAN_POINT('Ctrl Pts',(31.1623224722433,-33.545026950671,43.296682310541));
#21632=CARTESIAN_POINT('Ctrl Pts',(30.6726602441004,-33.1519466558869,43.2596390474678));
#21633=CARTESIAN_POINT('Ctrl Pts',(30.4601481013144,-32.6431153137696,43.2225957843945));
#21634=CARTESIAN_POINT('Ctrl Pts',(30.2476359585285,-32.1342839716523,43.1855525213213));
#21635=CARTESIAN_POINT('Ctrl Pts',(30.3122739010995,-31.5097015822019,43.1485092582481));
#21636=CARTESIAN_POINT('Ctrl Pts',(30.6244839565387,-31.0551736700466,43.1114659951748));
#21637=CARTESIAN_POINT('Ctrl Pts',(30.9366940119779,-30.6006457578913,43.0744227321016));
#21638=CARTESIAN_POINT('Ctrl Pts',(31.4964761802852,-30.3161723230313,43.0373794690283));
#21639=CARTESIAN_POINT('Ctrl Pts',(32.0476771774324,-30.331926847221,43.0003362059551));
#21640=CARTESIAN_POINT('Ctrl Pts',(32.5988781745796,-30.3476813714108,42.9632929428818));
#21641=CARTESIAN_POINT('Ctrl Pts',(33.1414980005666,-30.6636638546505,42.9262496798086));
#21642=CARTESIAN_POINT('Ctrl Pts',(33.4272367634802,-31.1352824646434,42.8892064167354));
#21643=CARTESIAN_POINT('Ctrl Pts',(33.583275622188,-31.3928283044107,42.8689774900268));
#21644=CARTESIAN_POINT('Ctrl Pts',(33.6627090958471,-31.696786928658,42.8487485633183));
#21645=CARTESIAN_POINT('Ctrl Pts',(33.6633867149896,-32.0004154269497,42.8285196366098));
#21646=CARTESIAN_POINT('Origin',(32.,-32.,48.));
#21647=CARTESIAN_POINT('',(33.6673070425528,-32.0013037875835,42.1285196366098));
#21648=CARTESIAN_POINT('',(33.6682077276635,-31.9991447210259,42.3214803633902));
#21649=CARTESIAN_POINT('',(33.666,-32.,48.));
#21650=CARTESIAN_POINT('Ctrl Pts',(33.6682077276635,-31.9991447210259,42.3214803633902));
#21651=CARTESIAN_POINT('Ctrl Pts',(33.6685152776142,-31.9500189184328,42.3247776195697));
#21652=CARTESIAN_POINT('Ctrl Pts',(33.6665333026985,-31.9009182818708,42.3280748757492));
#21653=CARTESIAN_POINT('Ctrl Pts',(33.662181037674,-31.8520286556063,42.3313721319287));
#21654=CARTESIAN_POINT('Ctrl Pts',(33.6132852014122,-31.3027746126452,42.3684153950019));
#21655=CARTESIAN_POINT('Ctrl Pts',(33.2652217397612,-30.7801533642977,42.4054586580752));
#21656=CARTESIAN_POINT('Ctrl Pts',(32.7772627875611,-30.5233133209011,42.4425019211484));
#21657=CARTESIAN_POINT('Ctrl Pts',(32.2893038353611,-30.2664732775045,42.4795451842217));
#21658=CARTESIAN_POINT('Ctrl Pts',(31.6614493926119,-30.2754144390588,42.5165884472949));
#21659=CARTESIAN_POINT('Ctrl Pts',(31.1810021559353,-30.5460454993071,42.5536317103682));
#21660=CARTESIAN_POINT('Ctrl Pts',(30.7005549192587,-30.8166765595554,42.5906749734414));
#21661=CARTESIAN_POINT('Ctrl Pts',(30.3675148886547,-31.3489975184977,42.6277182365146));
#21662=CARTESIAN_POINT('Ctrl Pts',(30.3342794227585,-31.8994211306946,42.6647614995879));
#21663=CARTESIAN_POINT('Ctrl Pts',(30.3010439568623,-32.4498447428914,42.7018047626611));
#21664=CARTESIAN_POINT('Ctrl Pts',(30.5676130556739,-33.018371008343,42.7388480257344));
#21665=CARTESIAN_POINT('Ctrl Pts',(31.0120061215156,-33.3448454215074,42.7758912888076));
#21666=CARTESIAN_POINT('Ctrl Pts',(31.4563991873573,-33.6713198346718,42.8129345518809));
#21667=CARTESIAN_POINT('Ctrl Pts',(32.078616220229,-33.7557423955491,42.8499778149541));
#21668=CARTESIAN_POINT('Ctrl Pts',(32.5939340915773,-33.5594817824733,42.8870210780274));
#21669=CARTESIAN_POINT('Ctrl Pts',(33.1092519629256,-33.3632211693975,42.9240643411006));
#21670=CARTESIAN_POINT('Ctrl Pts',(33.5176706727504,-32.8862773823686,42.9611076041738));
#21671=CARTESIAN_POINT('Ctrl Pts',(33.6323000280045,-32.3468973200768,42.998150867247));
#21672=CARTESIAN_POINT('Ctrl Pts',(33.656364188659,-32.2336651689923,43.0059273659614));
#21673=CARTESIAN_POINT('Ctrl Pts',(33.6674808531087,-32.1176814088911,43.0137038646758));
#21674=CARTESIAN_POINT('Ctrl Pts',(33.6664085055627,-32.0014938638813,43.0214803633902));
#21675=CARTESIAN_POINT('Ctrl Pts',(33.6633867149896,-32.0004154269497,42.8285196366098));
#21676=CARTESIAN_POINT('Ctrl Pts',(33.6639499537789,-32.2527922225036,42.8117053002451));
#21677=CARTESIAN_POINT('Ctrl Pts',(33.6101009496347,-32.5049409347766,42.7948909638803));
#21678=CARTESIAN_POINT('Ctrl Pts',(33.500604739542,-32.7300182319024,42.7780766275156));
#21679=CARTESIAN_POINT('Ctrl Pts',(33.2593762528503,-33.2258806524225,42.7410333644424));
#21680=CARTESIAN_POINT('Ctrl Pts',(32.7480615796269,-33.5903507567164,42.7039901013691));
#21681=CARTESIAN_POINT('Ctrl Pts',(32.2006355348935,-33.6566491529375,42.6669468382959));
#21682=CARTESIAN_POINT('Ctrl Pts',(31.6532094901602,-33.7229475491586,42.6299035752227));
#21683=CARTESIAN_POINT('Ctrl Pts',(31.069672073917,-33.4910742373069,42.5928603121494));
#21684=CARTESIAN_POINT('Ctrl Pts',(30.7170468575088,-33.0671328874538,42.5558170490762));
#21685=CARTESIAN_POINT('Ctrl Pts',(30.3644216411006,-32.6431915376008,42.5187737860029));
#21686=CARTESIAN_POINT('Ctrl Pts',(30.2427086245275,-32.0271821497465,42.4817305229297));
#21687=CARTESIAN_POINT('Ctrl Pts',(30.4076029969488,-31.5009878737835,42.4446872598565));
#21688=CARTESIAN_POINT('Ctrl Pts',(30.5724973693701,-30.9747935978205,42.4076439967832));
#21689=CARTESIAN_POINT('Ctrl Pts',(31.0239991307858,-30.5384144337488,42.3706007337099));
#21690=CARTESIAN_POINT('Ctrl Pts',(31.5555035773089,-30.3915339446307,42.3335574706367));
#21691=CARTESIAN_POINT('Ctrl Pts',(32.087008023832,-30.2446534555125,42.2965142075635));
#21692=CARTESIAN_POINT('Ctrl Pts',(32.6985151554626,-30.3872716413479,42.2594709444902));
#21693=CARTESIAN_POINT('Ctrl Pts',(33.1102025176852,-30.7541295221294,42.222427681417));
#21694=CARTESIAN_POINT('Ctrl Pts',(33.4580908339469,-31.0641355659471,42.1911249998146));
#21695=CARTESIAN_POINT('Ctrl Pts',(33.6632925897301,-31.5342658601802,42.1598223182122));
#21696=CARTESIAN_POINT('Ctrl Pts',(33.6673070425528,-32.0013037875835,42.1285196366098));
#21697=CARTESIAN_POINT('Origin',(32.,-32.,48.));
#21698=CARTESIAN_POINT('',(33.6674738845699,-31.9987897819954,41.4285196366098));
#21699=CARTESIAN_POINT('',(33.6638410100825,-31.9990545799874,41.6214803633902));
#21700=CARTESIAN_POINT('',(33.666,-32.,48.));
#21701=CARTESIAN_POINT('',(30.7309291201476,-30.9206413469515,41.));
#21702=CARTESIAN_POINT('Ctrl Pts',(33.6674738845699,-31.9987897819954,41.4285196366098));
#21703=CARTESIAN_POINT('Ctrl Pts',(33.6635381632177,-32.4716720161883,41.3968095469596));
#21704=CARTESIAN_POINT('Ctrl Pts',(33.452320926774,-32.9475347722184,41.3650994573094));
#21705=CARTESIAN_POINT('Ctrl Pts',(33.0964755924645,-33.2578208392569,41.3333893676592));
#21706=CARTESIAN_POINT('Ctrl Pts',(32.6807822759957,-33.6202924858546,41.296346104586));
#21707=CARTESIAN_POINT('Ctrl Pts',(32.0677212020934,-33.7568087318644,41.2593028415127));
#21708=CARTESIAN_POINT('Ctrl Pts',(31.5378645772582,-33.6037827123866,41.2222595784395));
#21709=CARTESIAN_POINT('Ctrl Pts',(31.008007952423,-33.4507566929088,41.1852163153662));
#21710=CARTESIAN_POINT('Ctrl Pts',(30.5613557766549,-33.0081884079434,41.148173052293));
#21711=CARTESIAN_POINT('Ctrl Pts',(30.402364501489,-32.4811509461478,41.1111297892197));
#21712=CARTESIAN_POINT('Ctrl Pts',(30.2433732263231,-31.9541134843521,41.0740865261465));
#21713=CARTESIAN_POINT('Ctrl Pts',(30.3720428517593,-31.3426068457262,41.0370432630732));
#21714=CARTESIAN_POINT('Ctrl Pts',(30.7309291201476,-30.9206413469515,41.));
#21715=CARTESIAN_POINT('',(33.2714670322121,-30.9187899875149,41.));
#21716=CARTESIAN_POINT('Origin',(32.,-32.,41.));
#21717=CARTESIAN_POINT('Ctrl Pts',(33.2714683511891,-30.9187889684226,41.));
#21718=CARTESIAN_POINT('Ctrl Pts',(32.9206802420719,-30.5073507297867,41.0363148168373));
#21719=CARTESIAN_POINT('Ctrl Pts',(32.3508928184604,-30.2813273881367,41.0726296336745));
#21720=CARTESIAN_POINT('Ctrl Pts',(31.8135997916615,-30.3418001164503,41.1089444505117));
#21721=CARTESIAN_POINT('Ctrl Pts',(31.2655290956605,-30.4034858794192,41.1459877135849));
#21722=CARTESIAN_POINT('Ctrl Pts',(30.751269494614,-30.7632767551392,41.1830309766582));
#21723=CARTESIAN_POINT('Ctrl Pts',(30.5058096205078,-31.2569744715082,41.2200742397314));
#21724=CARTESIAN_POINT('Ctrl Pts',(30.2603497464016,-31.7506721878771,41.2571175028047));
#21725=CARTESIAN_POINT('Ctrl Pts',(30.2836895992358,-32.3782767448949,41.2941607658779));
#21726=CARTESIAN_POINT('Ctrl Pts',(30.5653173100033,-32.852378515895,41.3312040289512));
#21727=CARTESIAN_POINT('Ctrl Pts',(30.8469450207708,-33.326480286895,41.3682472920244));
#21728=CARTESIAN_POINT('Ctrl Pts',(31.3868605894716,-33.6470792718774,41.4052905550977));
#21729=CARTESIAN_POINT('Ctrl Pts',(31.9379165745124,-33.6675827533924,41.4423338181709));
#21730=CARTESIAN_POINT('Ctrl Pts',(32.4889725595533,-33.6880862349073,41.4793770812441));
#21731=CARTESIAN_POINT('Ctrl Pts',(33.0511689609341,-33.4084942129547,41.5164203443174));
#21732=CARTESIAN_POINT('Ctrl Pts',(33.3672906927666,-32.9566900927607,41.5534636073906));
#21733=CARTESIAN_POINT('Ctrl Pts',(33.5607723402275,-32.6801643221405,41.5761358593905));
#21734=CARTESIAN_POINT('Ctrl Pts',(33.6620737637366,-32.3391274427084,41.5988081113903));
#21735=CARTESIAN_POINT('Ctrl Pts',(33.6638410100825,-31.9990545799874,41.6214803633902));
#21736=CARTESIAN_POINT('Origin',(32.,-32.,39.4540747194623));
#21737=CARTESIAN_POINT('',(34.0532845839741,-31.9981685058867,53.7459252805377));
#21738=CARTESIAN_POINT('',(34.0546388766263,-32.0018310485179,53.8040747194623));
#21739=CARTESIAN_POINT('',(34.05475,-31.9999999999998,39.4540747194623));
#21740=CARTESIAN_POINT('',(31.6163320011532,-29.9813874990081,54.));
#21741=CARTESIAN_POINT('Ctrl Pts',(34.0546388766263,-32.0018310485179,53.8040747194623));
#21742=CARTESIAN_POINT('Ctrl Pts',(34.0493720989589,-31.4803615643801,53.832339883235));
#21743=CARTESIAN_POINT('Ctrl Pts',(33.5817165233639,-30.267781276506,53.8976483100809));
#21744=CARTESIAN_POINT('Ctrl Pts',(32.2875197530249,-29.8538180613451,53.9629567369268));
#21745=CARTESIAN_POINT('Ctrl Pts',(31.6163320011532,-29.9813874990081,54.));
#21746=CARTESIAN_POINT('',(30.6584342820381,-30.4387365847154,54.));
#21747=CARTESIAN_POINT('Origin',(32.,-32.,54.));
#21748=CARTESIAN_POINT('Ctrl Pts',(34.0532845839741,-31.9981685058867,53.7459252805377));
#21749=CARTESIAN_POINT('Ctrl Pts',(34.0549509938535,-31.7888165552494,53.7572587737813));
#21750=CARTESIAN_POINT('Ctrl Pts',(33.9292547539713,-30.8972175167488,53.8056355300982));
#21751=CARTESIAN_POINT('Ctrl Pts',(32.6546770307308,-29.6694113223394,53.8903271032523));
#21752=CARTESIAN_POINT('Ctrl Pts',(31.1647629871531,-30.0047891265576,53.9636851831628));
#21753=CARTESIAN_POINT('Ctrl Pts',(30.6584328706692,-30.4387350900138,54.));
#21754=CARTESIAN_POINT('Origin',(32.,-32.,39.4540747194623));
#21755=CARTESIAN_POINT('',(34.0520082578512,-32.0011056323104,53.0459252805377));
#21756=CARTESIAN_POINT('',(34.0578094041387,-31.9992426192728,53.1040747194623));
#21757=CARTESIAN_POINT('',(34.05475,-31.9999999999998,39.4540747194623));
#21758=CARTESIAN_POINT('Ctrl Pts',(34.0578094041387,-31.9992426192728,53.1040747194623));
#21759=CARTESIAN_POINT('Ctrl Pts',(34.0580096564622,-31.9570764465673,53.1063703750556));
#21760=CARTESIAN_POINT('Ctrl Pts',(34.0377190194437,-31.2347025738574,53.1457092937222));
#21761=CARTESIAN_POINT('Ctrl Pts',(33.188671237128,-29.8822030499806,53.2220914754619));
#21762=CARTESIAN_POINT('Ctrl Pts',(30.8656743801615,-29.8526922201837,53.3332212646816));
#21763=CARTESIAN_POINT('Ctrl Pts',(29.5804895672685,-31.7882160395824,53.4443510539014));
#21764=CARTESIAN_POINT('Ctrl Pts',(30.5102291276843,-33.9178753902133,53.5554808431211));
#21765=CARTESIAN_POINT('Ctrl Pts',(32.8021731990342,-34.291695073573,53.6666106323408));
#21766=CARTESIAN_POINT('Ctrl Pts',(33.9655643323599,-33.007470946703,53.7494752577879));
#21767=CARTESIAN_POINT('Ctrl Pts',(34.0562745401495,-32.1637799036814,53.7952966201617));
#21768=CARTESIAN_POINT('Ctrl Pts',(34.0546388766263,-32.0018310485179,53.8040747194623));
#21769=CARTESIAN_POINT('Ctrl Pts',(34.0520082578512,-32.0011056323104,53.0459252805377));
#21770=CARTESIAN_POINT('Ctrl Pts',(34.0499813688103,-31.5865449283087,53.0683325286752));
#21771=CARTESIAN_POINT('Ctrl Pts',(33.726754614814,-30.48373431258,53.127783039886));
#21772=CARTESIAN_POINT('Ctrl Pts',(31.9269572285084,-29.572527465193,53.2242768141699));
#21773=CARTESIAN_POINT('Ctrl Pts',(29.9209962036954,-30.7446672845728,53.3354066033898));
#21774=CARTESIAN_POINT('Ctrl Pts',(29.8177591150446,-33.0657522553465,53.4465363926093));
#21775=CARTESIAN_POINT('Ctrl Pts',(31.7116016656226,-34.4113173899075,53.5576661818292));
#21776=CARTESIAN_POINT('Ctrl Pts',(33.6494719430299,-33.6381800302083,53.6574624778052));
#21777=CARTESIAN_POINT('Ctrl Pts',(34.0495043713317,-32.473078610703,53.7202155107081));
#21778=CARTESIAN_POINT('Ctrl Pts',(34.0532845839741,-31.9981685058867,53.7459252805377));
#21779=CARTESIAN_POINT('Origin',(32.,-32.,39.4540747194623));
#21780=CARTESIAN_POINT('',(34.0573710650655,-32.0011268473916,52.3459252805377));
#21781=CARTESIAN_POINT('',(34.0524437812007,-31.99860578477,52.4040747194623));
#21782=CARTESIAN_POINT('',(34.05475,-31.9999999999998,39.4540747194623));
#21783=CARTESIAN_POINT('Ctrl Pts',(34.0524437812007,-31.99860578477,52.4040747194623));
#21784=CARTESIAN_POINT('Ctrl Pts',(34.0539874975223,-31.751387773122,52.4174441299495));
#21785=CARTESIAN_POINT('Ctrl Pts',(33.8982127967441,-30.8210709022261,52.4678568035099));
#21786=CARTESIAN_POINT('Ctrl Pts',(32.5140660253384,-29.6264478034877,52.5553127401435));
#21787=CARTESIAN_POINT('Ctrl Pts',(30.284773107188,-30.2806972020757,52.6664425293633));
#21788=CARTESIAN_POINT('Ctrl Pts',(29.6252320820182,-32.5084312487041,52.777572318583));
#21789=CARTESIAN_POINT('Ctrl Pts',(31.1390631138414,-34.2708597317664,52.8887021078028));
#21790=CARTESIAN_POINT('Ctrl Pts',(33.3932461919552,-33.9615363252737,52.9975362414291));
#21791=CARTESIAN_POINT('Ctrl Pts',(34.0547783357362,-32.6374801765024,53.0693271119824));
#21792=CARTESIAN_POINT('Ctrl Pts',(34.0578094041387,-31.9992426192728,53.1040747194623));
#21793=CARTESIAN_POINT('Ctrl Pts',(34.0573710650655,-32.0011268473916,52.3459252805377));
#21794=CARTESIAN_POINT('Ctrl Pts',(34.05330779479,-31.3858139390653,52.3794062835691));
#21795=CARTESIAN_POINT('Ctrl Pts',(33.4332399063797,-30.0826172598142,52.4499305496737));
#21796=CARTESIAN_POINT('Ctrl Pts',(31.2169954713513,-29.7011055471504,52.5574980788516));
#21797=CARTESIAN_POINT('Ctrl Pts',(29.6439536772523,-31.4108821177788,52.6686278680713));
#21798=CARTESIAN_POINT('Ctrl Pts',(30.2271406288629,-33.6598142860527,52.779757657291));
#21799=CARTESIAN_POINT('Ctrl Pts',(32.432827862626,-34.3896998451232,52.8908874465108));
#21800=CARTESIAN_POINT('Ctrl Pts',(33.8775323335813,-33.2263675462608,52.979609987593));
#21801=CARTESIAN_POINT('Ctrl Pts',(34.0533321856309,-32.2718892920576,53.031289265602));
#21802=CARTESIAN_POINT('Ctrl Pts',(34.0520082578512,-32.0011056323104,53.0459252805377));
#21803=CARTESIAN_POINT('Origin',(32.,-32.,39.4540747194623));
#21804=CARTESIAN_POINT('',(34.0554019757745,-31.9981759026781,51.6459252805377));
#21805=CARTESIAN_POINT('',(34.0527564122603,-32.0015414517042,51.7040747194623));
#21806=CARTESIAN_POINT('',(34.05475,-31.9999999999998,39.4540747194623));
#21807=CARTESIAN_POINT('Ctrl Pts',(34.0527564122603,-32.0015414517042,51.7040747194623));
#21808=CARTESIAN_POINT('Ctrl Pts',(34.0496053847508,-31.5497282207227,51.7285178848434));
#21809=CARTESIAN_POINT('Ctrl Pts',(33.680048118902,-30.4085132206192,51.7900043132977));
#21810=CARTESIAN_POINT('Ctrl Pts',(31.7940455863876,-29.5801661817881,51.8885340048252));
#21811=CARTESIAN_POINT('Ctrl Pts',(29.8553460280345,-30.8604947990401,51.9996637940449));
#21812=CARTESIAN_POINT('Ctrl Pts',(29.8794104413083,-33.1836861751323,52.1107935832647));
#21813=CARTESIAN_POINT('Ctrl Pts',(31.844215591537,-34.4235808867133,52.2219233724843));
#21814=CARTESIAN_POINT('Ctrl Pts',(33.6980657303603,-33.5631151460834,52.3196837512169));
#21815=CARTESIAN_POINT('Ctrl Pts',(34.0497102491075,-32.4363665050346,52.3804008668763));
#21816=CARTESIAN_POINT('Ctrl Pts',(34.0524437812007,-31.99860578477,52.4040747194623));
#21817=CARTESIAN_POINT('Ctrl Pts',(34.0554019757745,-31.9981759026781,51.6459252805377));
#21818=CARTESIAN_POINT('Ctrl Pts',(34.0566763311782,-31.859785689655,51.6534367753897));
#21819=CARTESIAN_POINT('Ctrl Pts',(33.9808503317639,-31.0403066930034,51.6979915333149));
#21820=CARTESIAN_POINT('Ctrl Pts',(32.8805414477757,-29.736670690513,51.7795895543136));
#21821=CARTESIAN_POINT('Ctrl Pts',(30.5761493204034,-30.0326001869503,51.8907193435332));
#21822=CARTESIAN_POINT('Ctrl Pts',(29.5748498880924,-32.1290726458106,52.001849132753));
#21823=CARTESIAN_POINT('Ctrl Pts',(30.7930215501968,-34.1074192405717,52.1129789219727));
#21824=CARTESIAN_POINT('Ctrl Pts',(33.1158067773521,-34.1570785575888,52.2241087111924));
#21825=CARTESIAN_POINT('Ctrl Pts',(34.0252705293619,-32.8124059202895,52.3017574973807));
#21826=CARTESIAN_POINT('Ctrl Pts',(34.0578033826196,-32.0665939597273,52.3423630204958));
#21827=CARTESIAN_POINT('Ctrl Pts',(34.0573710650655,-32.0011268473916,52.3459252805377));
#21828=CARTESIAN_POINT('Origin',(32.,-32.,39.4540747194623));
#21829=CARTESIAN_POINT('',(34.0514089344138,-32.0000193278948,50.9459252805377));
#21830=CARTESIAN_POINT('',(34.0579890512349,-32.0005154328357,51.0040747194623));
#21831=CARTESIAN_POINT('',(34.05475,-31.9999999999998,39.4540747194623));
#21832=CARTESIAN_POINT('Ctrl Pts',(34.057989051235,-32.0005154328357,51.0040747194623));
#21833=CARTESIAN_POINT('Ctrl Pts',(34.0557929694248,-31.3483062423322,51.0395916397373));
#21834=CARTESIAN_POINT('Ctrl Pts',(33.3683017673568,-30.0118742773859,51.1121518230855));
#21835=CARTESIAN_POINT('Ctrl Pts',(31.0922024613207,-29.7474644236002,51.2217552695068));
#21836=CARTESIAN_POINT('Ctrl Pts',(29.6152125517546,-31.5408685177941,51.3328850587265));
#21837=CARTESIAN_POINT('Ctrl Pts',(30.3207542514557,-33.7544647647039,51.4440148479463));
#21838=CARTESIAN_POINT('Ctrl Pts',(32.563123452382,-34.3623938867708,51.555144637166));
#21839=CARTESIAN_POINT('Ctrl Pts',(33.9102708685271,-33.1501141796208,51.6418312610047));
#21840=CARTESIAN_POINT('Ctrl Pts',(34.0543807212984,-32.2344446277146,51.6914746217701));
#21841=CARTESIAN_POINT('Ctrl Pts',(34.0527564122603,-32.0015414517042,51.7040747194623));
#21842=CARTESIAN_POINT('Ctrl Pts',(34.0514089344138,-32.0000193278948,50.9459252805377));
#21843=CARTESIAN_POINT('Ctrl Pts',(34.0513800613624,-31.6559195562416,50.9645105302836));
#21844=CARTESIAN_POINT('Ctrl Pts',(33.8061927556769,-30.6259373145995,51.0201390431027));
#21845=CARTESIAN_POINT('Ctrl Pts',(32.1767300235671,-29.5778564663098,51.1128108189952));
#21846=CARTESIAN_POINT('Ctrl Pts',(30.0609756751137,-30.5377423393424,51.2239406082148));
#21847=CARTESIAN_POINT('Ctrl Pts',(29.7197953608552,-32.8358705657033,51.3350703974346));
#21848=CARTESIAN_POINT('Ctrl Pts',(31.465433604746,-34.3690191153306,51.4462001866543));
#21849=CARTESIAN_POINT('Ctrl Pts',(33.5492418405736,-33.7769847980368,51.5498184810221));
#21850=CARTESIAN_POINT('Ctrl Pts',(34.0503917921621,-32.5422630352122,51.6163935123165));
#21851=CARTESIAN_POINT('Ctrl Pts',(34.0554019757745,-31.9981759026781,51.6459252805377));
#21852=CARTESIAN_POINT('Origin',(32.,-32.,39.4540747194623));
#21853=CARTESIAN_POINT('',(34.055472908735,-32.0018139477898,50.2459252805377));
#21854=CARTESIAN_POINT('',(34.0542687450602,-31.9981314910207,50.3040747194623));
#21855=CARTESIAN_POINT('',(34.05475,-31.9999999999998,39.4540747194623));
#21856=CARTESIAN_POINT('Ctrl Pts',(34.0542687450602,-31.9981314910207,50.3040747194623));
#21857=CARTESIAN_POINT('Ctrl Pts',(34.0558440944503,-31.8219835585998,50.3136221315579));
#21858=CARTESIAN_POINT('Ctrl Pts',(33.9544817357664,-30.9641799391559,50.3602128067267));
#21859=CARTESIAN_POINT('Ctrl Pts',(32.7551980511737,-29.6918213247557,50.4438467449688));
#21860=CARTESIAN_POINT('Ctrl Pts',(30.470483670184,-30.1135767468053,50.5549765341884));
#21861=CARTESIAN_POINT('Ctrl Pts',(29.5855660473401,-32.2617662727765,50.6661063234083));
#21862=CARTESIAN_POINT('Ctrl Pts',(30.9103121945009,-34.1703901446276,50.7772361126279));
#21863=CARTESIAN_POINT('Ctrl Pts',(33.2323288041292,-34.0926964930404,50.8883659018477));
#21864=CARTESIAN_POINT('Ctrl Pts',(34.0448660118093,-32.7367198389241,50.9639787707924));
#21865=CARTESIAN_POINT('Ctrl Pts',(34.0580834280455,-32.0285441806329,51.002548376664));
#21866=CARTESIAN_POINT('Ctrl Pts',(34.057989051235,-32.0005154328357,51.0040747194623));
#21867=CARTESIAN_POINT('Ctrl Pts',(34.055472908735,-32.0018139477898,50.2459252805377));
#21868=CARTESIAN_POINT('Ctrl Pts',(34.0504505301634,-31.4554311545241,50.2755842851775));
#21869=CARTESIAN_POINT('Ctrl Pts',(33.5457056833664,-30.2184358152945,50.3422865528905));
#21870=CARTESIAN_POINT('Ctrl Pts',(31.4573199910465,-29.6328263251734,50.4460320836768));
#21871=CARTESIAN_POINT('Ctrl Pts',(29.7169448784392,-31.1719467946929,50.5571618728964));
#21872=CARTESIAN_POINT('Ctrl Pts',(30.0659970543811,-33.4688925778434,50.6682916621163));
#21873=CARTESIAN_POINT('Ctrl Pts',(32.1850277527679,-34.4215238032342,50.7794214513359));
#21874=CARTESIAN_POINT('Ctrl Pts',(33.8086577032695,-33.3693128790145,50.8719659908098));
#21875=CARTESIAN_POINT('Ctrl Pts',(34.0514376097974,-32.3417633592069,50.9274672672104));
#21876=CARTESIAN_POINT('Ctrl Pts',(34.0514089344138,-32.0000193278948,50.9459252805377));
#21877=CARTESIAN_POINT('Origin',(32.,-32.,39.4540747194623));
#21878=CARTESIAN_POINT('',(34.0573202636303,-31.9988395216185,49.5459252805377));
#21879=CARTESIAN_POINT('',(34.0515870098674,-32.0006260541466,49.6040747194623));
#21880=CARTESIAN_POINT('',(34.05475,-31.9999999999998,39.4540747194623));
#21881=CARTESIAN_POINT('Ctrl Pts',(34.0515870098674,-32.0006260541466,49.6040747194623));
#21882=CARTESIAN_POINT('Ctrl Pts',(34.0505442505756,-31.6189146354342,49.6246958864518));
#21883=CARTESIAN_POINT('Ctrl Pts',(33.7651923215172,-30.5500595553348,49.6823603165144));
#21884=CARTESIAN_POINT('Ctrl Pts',(32.0437417120601,-29.5718114661385,49.7770680096504));
#21885=CARTESIAN_POINT('Ctrl Pts',(29.9837635871641,-30.6461892226366,49.8881977988701));
#21886=CARTESIAN_POINT('Ctrl Pts',(29.7690231621222,-32.9595599211113,49.9993275880899));
#21887=CARTESIAN_POINT('Ctrl Pts',(31.5960485451694,-34.3947517857787,50.1104573773095));
#21888=CARTESIAN_POINT('Ctrl Pts',(33.6040409500067,-33.7032818934708,50.2120397544338));
#21889=CARTESIAN_POINT('Ctrl Pts',(34.0497318536352,-32.5054246979535,50.2765788684846));
#21890=CARTESIAN_POINT('Ctrl Pts',(34.0542687450602,-31.9981314910207,50.3040747194623));
#21891=CARTESIAN_POINT('Ctrl Pts',(34.0573202636303,-31.9988395216185,49.5459252805377));
#21892=CARTESIAN_POINT('Ctrl Pts',(34.0577786805335,-31.9310296536276,49.5496147769981));
#21893=CARTESIAN_POINT('Ctrl Pts',(34.0239729579483,-31.1828581577522,49.5903475365317));
#21894=CARTESIAN_POINT('Ctrl Pts',(33.1084096420059,-29.8391110939209,49.6681235591387));
#21895=CARTESIAN_POINT('Ctrl Pts',(30.785808172351,-29.8967284995564,49.7792533483584));
#21896=CARTESIAN_POINT('Ctrl Pts',(29.5744218959985,-31.8792371733684,49.8903831375781));
#21897=CARTESIAN_POINT('Ctrl Pts',(30.5828983961289,-33.9722666764952,50.0015129267979));
#21898=CARTESIAN_POINT('Ctrl Pts',(32.8882909162952,-34.2602991056352,50.1126427160176));
#21899=CARTESIAN_POINT('Ctrl Pts',(33.9824180683095,-32.9549395059557,50.1941135005975));
#21900=CARTESIAN_POINT('Ctrl Pts',(34.0567233398191,-32.1378479043595,50.2385410221042));
#21901=CARTESIAN_POINT('Ctrl Pts',(34.055472908735,-32.0018139477898,50.2459252805377));
#21902=CARTESIAN_POINT('Origin',(32.,-32.,39.4540747194623));
#21903=CARTESIAN_POINT('',(34.0519708956138,-31.9989253245976,48.8459252805377));
#21904=CARTESIAN_POINT('',(34.0565621614737,-32.0015359425915,48.9040747194623));
#21905=CARTESIAN_POINT('',(34.05475,-31.9999999999998,39.4540747194623));
#21906=CARTESIAN_POINT('Ctrl Pts',(34.0565621614737,-32.0015359425915,48.9040747194623));
#21907=CARTESIAN_POINT('Ctrl Pts',(34.0516979528083,-31.418447338828,48.9357696413457));
#21908=CARTESIAN_POINT('Ctrl Pts',(33.4873124744596,-30.1456437189272,49.0045078263022));
#21909=CARTESIAN_POINT('Ctrl Pts',(31.3284246265722,-29.6661192380166,49.1102892743321));
#21910=CARTESIAN_POINT('Ctrl Pts',(29.6750012716246,-31.2982922215028,49.2214190635517));
#21911=CARTESIAN_POINT('Ctrl Pts',(30.1493915393249,-33.5726605541655,49.3325488527715));
#21912=CARTESIAN_POINT('Ctrl Pts',(32.317438601222,-34.4077470024496,49.4436786419912));
#21913=CARTESIAN_POINT('Ctrl Pts',(33.8465759975202,-33.2932195337787,49.5341872642215));
#21914=CARTESIAN_POINT('Ctrl Pts',(34.0524174329609,-32.3046098974271,49.5876526233785));
#21915=CARTESIAN_POINT('Ctrl Pts',(34.0515870098674,-32.0006260541466,49.6040747194623));
#21916=CARTESIAN_POINT('Ctrl Pts',(34.0519708956138,-31.9989253245976,48.8459252805377));
#21917=CARTESIAN_POINT('Ctrl Pts',(34.0532663991156,-31.7257756104976,48.860688531892));
#21918=CARTESIAN_POINT('Ctrl Pts',(33.8753960113233,-30.7688700324249,48.9124950463195));
#21919=CARTESIAN_POINT('Ctrl Pts',(32.4246384795753,-29.6088297926389,49.0013448238203));
#21920=CARTESIAN_POINT('Ctrl Pts',(30.2214637798412,-30.34627036294,49.1124746130401));
#21921=CARTESIAN_POINT('Ctrl Pts',(29.6459861413742,-32.5971863631273,49.2236044022597));
#21922=CARTESIAN_POINT('Ctrl Pts',(31.2248764581043,-34.3015638799969,49.3347341914795));
#21923=CARTESIAN_POINT('Ctrl Pts',(33.4371809635416,-33.9129210756653,49.4421744842388));
#21924=CARTESIAN_POINT('Ctrl Pts',(34.0531760855389,-32.6118539357201,49.5125715139249));
#21925=CARTESIAN_POINT('Ctrl Pts',(34.0573202636303,-31.9988395216185,49.5459252805377));
#21926=CARTESIAN_POINT('Origin',(32.,-32.,39.4540747194623));
#21927=CARTESIAN_POINT('',(34.0534017172989,-32.0017453556898,48.1459252805377));
#21928=CARTESIAN_POINT('',(34.056369973564,-31.9983965631577,48.2040747194623));
#21929=CARTESIAN_POINT('',(34.05475,-31.9999999999998,39.4540747194623));
#21930=CARTESIAN_POINT('Ctrl Pts',(34.056369973564,-31.9983965631577,48.2040747194623));
#21931=CARTESIAN_POINT('Ctrl Pts',(34.0572746156918,-31.8930410344953,48.2098001331663));
#21932=CARTESIAN_POINT('Ctrl Pts',(34.0020141870959,-31.106989754687,48.2525688099435));
#21933=CARTESIAN_POINT('Ctrl Pts',(32.9883371782127,-29.7816216473485,48.3323807497939));
#21934=CARTESIAN_POINT('Ctrl Pts',(30.6723823629214,-29.966420814655,48.4435105390137));
#21935=CARTESIAN_POINT('Ctrl Pts',(29.5714488116707,-32.0123295991414,48.5546403282333));
#21936=CARTESIAN_POINT('Ctrl Pts',(30.693098971438,-34.0469544682025,48.6657701174531));
#21937=CARTESIAN_POINT('Ctrl Pts',(33.0108107797937,-34.2082288062616,48.7768999066728));
#21938=CARTESIAN_POINT('Ctrl Pts',(34.0062529590955,-32.8789465616399,48.8563347740093));
#21939=CARTESIAN_POINT('Ctrl Pts',(34.0573829695406,-32.09992889047,48.8987263782724));
#21940=CARTESIAN_POINT('Ctrl Pts',(34.0565621614737,-32.0015359425915,48.9040747194623));
#21941=CARTESIAN_POINT('Ctrl Pts',(34.0534017172989,-32.0017453556898,48.1459252805377));
#21942=CARTESIAN_POINT('Ctrl Pts',(34.0495478617348,-31.524546624056,48.1717622867859));
#21943=CARTESIAN_POINT('Ctrl Pts',(33.6462462789142,-30.3572999443065,48.2346425561073));
#21944=CARTESIAN_POINT('Ctrl Pts',(31.7033877262933,-29.5895987972966,48.334566088502));
#21945=CARTESIAN_POINT('Ctrl Pts',(29.8140971767976,-30.9417742932515,48.4456958777216));
#21946=CARTESIAN_POINT('Ctrl Pts',(29.9253211859677,-33.2624264800428,48.5568256669414));
#21947=CARTESIAN_POINT('Ctrl Pts',(31.9352687467854,-34.427719642744,48.6679554561611));
#21948=CARTESIAN_POINT('Ctrl Pts',(33.7295722549086,-33.5115468202576,48.7643219940266));
#21949=CARTESIAN_POINT('Ctrl Pts',(34.050015782034,-32.4111501580791,48.8236452688187));
#21950=CARTESIAN_POINT('Ctrl Pts',(34.0519708956138,-31.9989253245976,48.8459252805377));
#21951=CARTESIAN_POINT('Origin',(32.,-32.,39.4540747194623));
#21952=CARTESIAN_POINT('',(34.0581462892693,-32.0000454490473,47.4459252805377));
#21953=CARTESIAN_POINT('',(34.0515290217428,-31.9994832228354,47.5040747194623));
#21954=CARTESIAN_POINT('',(34.05475,-31.9999999999998,39.4540747194623));
#21955=CARTESIAN_POINT('Ctrl Pts',(34.0515290217428,-31.9994832228354,47.5040747194623));
#21956=CARTESIAN_POINT('Ctrl Pts',(34.0522291138724,-31.6884975730474,47.5208738880602));
#21957=CARTESIAN_POINT('Ctrl Pts',(33.8397673943927,-30.6926760820841,47.5747163197312));
#21958=CARTESIAN_POINT('Ctrl Pts',(32.2929749124037,-29.5891539671616,47.6656020144756));
#21959=CARTESIAN_POINT('Ctrl Pts',(30.1335187541459,-30.4462108726646,47.7767318036953));
#21960=CARTESIAN_POINT('Ctrl Pts',(29.6822459909475,-32.7252787373636,47.8878615929151));
#21961=CARTESIAN_POINT('Ctrl Pts',(31.3521565618384,-34.3405793669477,47.9989913821348));
#21962=CARTESIAN_POINT('Ctrl Pts',(33.4983863159947,-33.8409464804423,48.1043957576506));
#21963=CARTESIAN_POINT('Ctrl Pts',(34.0514216069734,-32.5746882946331,48.172756870093));
#21964=CARTESIAN_POINT('Ctrl Pts',(34.056369973564,-31.9983965631577,48.2040747194623));
#21965=CARTESIAN_POINT('Ctrl Pts',(34.0581458051732,-32.0000454425691,47.4459252805377));
#21966=CARTESIAN_POINT('Ctrl Pts',(34.057925295782,-31.3223792843277,47.4828360416798));
#21967=CARTESIAN_POINT('Ctrl Pts',(33.321785989982,-29.9642037469477,47.556790065895));
#21968=CARTESIAN_POINT('Ctrl Pts',(31.008316669847,-29.7831154807695,47.6677873531836));
#21969=CARTESIAN_POINT('Ctrl Pts',(29.59966349763,-31.6306797131245,47.7789171424033));
#21970=CARTESIAN_POINT('Ctrl Pts',(30.3877722618167,-33.8162418669164,47.8900469316231));
#21971=CARTESIAN_POINT('Ctrl Pts',(32.6513743681069,-34.3395991604291,48.0011767208428));
#21972=CARTESIAN_POINT('Ctrl Pts',(33.9311686773918,-33.0979137221593,48.0864695038144));
#21973=CARTESIAN_POINT('Ctrl Pts',(34.055073245912,-32.208720246353,48.1347190237126));
#21974=CARTESIAN_POINT('Ctrl Pts',(34.0534017172989,-32.0017453556898,48.1459252805377));
#21975=CARTESIAN_POINT('Origin',(32.,-32.,39.4540747194623));
#21976=CARTESIAN_POINT('',(34.0535341382367,-31.9982258659195,46.7459252805377));
#21977=CARTESIAN_POINT('',(34.0544757027884,-32.0018769326718,46.8040747194623));
#21978=CARTESIAN_POINT('',(34.05475,-31.9999999999998,39.4540747194623));
#21979=CARTESIAN_POINT('Ctrl Pts',(34.0544757027884,-32.0018769326718,46.8040747194623));
#21980=CARTESIAN_POINT('Ctrl Pts',(34.0498160242977,-31.4877588190714,46.831947642954));
#21981=CARTESIAN_POINT('Ctrl Pts',(33.5941431221402,-30.2830100163635,46.896863829519));
#21982=CARTESIAN_POINT('Ctrl Pts',(31.5717539918218,-29.6094732275437,46.9988232791572));
#21983=CARTESIAN_POINT('Ctrl Pts',(29.7593951696295,-31.0631420131788,47.1099530683769));
#21984=CARTESIAN_POINT('Ctrl Pts',(29.9976135898446,-33.3742130685507,47.2210828575967));
#21985=CARTESIAN_POINT('Ctrl Pts',(32.0683943376577,-34.4276192263053,47.3322126468163));
#21986=CARTESIAN_POINT('Ctrl Pts',(33.7730095140328,-33.4359068477222,47.4265432674384));
#21987=CARTESIAN_POINT('Ctrl Pts',(34.0506853650385,-32.3742412257766,47.4838306249869));
#21988=CARTESIAN_POINT('Ctrl Pts',(34.0515290217428,-31.9994832228354,47.5040747194623));
#21989=CARTESIAN_POINT('Ctrl Pts',(34.0535341382367,-31.9982258659195,46.7459252805377));
#21990=CARTESIAN_POINT('Ctrl Pts',(34.0552008741846,-31.7961784564346,46.7568665335004));
#21991=CARTESIAN_POINT('Ctrl Pts',(33.9350054837422,-30.9120087675869,46.8048510495363));
#21992=CARTESIAN_POINT('Ctrl Pts',(32.6680530383748,-29.6651085813628,46.8898788286456));
#21993=CARTESIAN_POINT('Ctrl Pts',(30.4007739163126,-30.172299605471,47.0010086178652));
#21994=CARTESIAN_POINT('Ctrl Pts',(29.5970891631565,-32.3521822100667,47.112138407085));
#21995=CARTESIAN_POINT('Ctrl Pts',(30.9925223493965,-34.2097514752664,47.2232681963047));
#21996=CARTESIAN_POINT('Ctrl Pts',(33.3099881558288,-34.0449801540592,47.3343979855244));
#21997=CARTESIAN_POINT('Ctrl Pts',(34.057041091318,-32.685008900317,47.4086170136021));
#21998=CARTESIAN_POINT('Ctrl Pts',(34.0581465967559,-32.0024781226841,47.4457927786065));
#21999=CARTESIAN_POINT('Ctrl Pts',(34.0581458051732,-32.0000454425691,47.4459252805377));
#22000=CARTESIAN_POINT('Origin',(32.,-32.,39.4540747194623));
#22001=CARTESIAN_POINT('',(34.0518959520928,-32.0010072981031,46.0459252805377));
#22002=CARTESIAN_POINT('',(34.0579058351471,-31.9993626137656,46.1040747194623));
#22003=CARTESIAN_POINT('',(34.05475,-31.9999999999998,39.4540747194623));
#22004=CARTESIAN_POINT('Ctrl Pts',(34.0579058351471,-31.9993626137656,46.1040747194623));
#22005=CARTESIAN_POINT('Ctrl Pts',(34.0580481959426,-31.96440578177,46.1059781347747));
#22006=CARTESIAN_POINT('Ctrl Pts',(34.0414007129417,-31.2492759708491,46.1449248131603));
#22007=CARTESIAN_POINT('Ctrl Pts',(33.2110168535402,-29.8948987972565,46.2209147546191));
#22008=CARTESIAN_POINT('Ctrl Pts',(30.8883310710498,-29.8407860027877,46.3320445438389));
#22009=CARTESIAN_POINT('Ctrl Pts',(29.5830326367871,-31.7627624428669,46.4431743330586));
#22010=CARTESIAN_POINT('Ctrl Pts',(30.4897165224173,-33.9018561225001,46.5543041222784));
#22011=CARTESIAN_POINT('Ctrl Pts',(32.7785954683888,-34.300391703592,46.665433911498));
#22012=CARTESIAN_POINT('Ctrl Pts',(33.9595497245257,-33.0217127890764,46.748690777226));
#22013=CARTESIAN_POINT('Ctrl Pts',(34.0560087617125,-32.1710245173564,46.7949043798808));
#22014=CARTESIAN_POINT('Ctrl Pts',(34.0544757027884,-32.0018769326718,46.8040747194623));
#22015=CARTESIAN_POINT('Ctrl Pts',(34.0518959520928,-32.0010072981031,46.0459252805377));
#22016=CARTESIAN_POINT('Ctrl Pts',(34.0500891203468,-31.5936483306361,46.0679402883943));
#22017=CARTESIAN_POINT('Ctrl Pts',(33.7353983817626,-30.4982792184681,46.1269985593241));
#22018=CARTESIAN_POINT('Ctrl Pts',(31.9525944730258,-29.5718802511161,46.2231000933272));
#22019=CARTESIAN_POINT('Ctrl Pts',(29.9343826179068,-30.7228008652907,46.3342298825469));
#22020=CARTESIAN_POINT('Ctrl Pts',(29.8066013901918,-33.0426002769034,46.4453596717666));
#22021=CARTESIAN_POINT('Ctrl Pts',(31.6861947837558,-34.4082232216233,46.5564894609863));
#22022=CARTESIAN_POINT('Ctrl Pts',(33.6396491312149,-33.6524065822643,46.6566779972434));
#22023=CARTESIAN_POINT('Ctrl Pts',(34.0495578881022,-32.4802404526548,46.7198232704271));
#22024=CARTESIAN_POINT('Ctrl Pts',(34.0535341382367,-31.9982258659195,46.7459252805377));
#22025=CARTESIAN_POINT('Origin',(32.,-32.,39.4540747194623));
#22026=CARTESIAN_POINT('',(34.0572106602559,-32.0012284763881,45.3459252805377));
#22027=CARTESIAN_POINT('',(34.0525988691351,-31.9985278358415,45.4040747194623));
#22028=CARTESIAN_POINT('',(34.05475,-31.9999999999998,39.4540747194623));
#22029=CARTESIAN_POINT('Ctrl Pts',(34.0525988691351,-31.9985278358415,45.4040747194623));
#22030=CARTESIAN_POINT('Ctrl Pts',(34.0541886318456,-31.758608443519,45.4170518896685));
#22031=CARTESIAN_POINT('Ctrl Pts',(33.9044076954203,-30.8357624066553,45.467072322948));
#22032=CARTESIAN_POINT('Ctrl Pts',(32.539107595012,-29.6320101574646,45.5541360193008));
#22033=CARTESIAN_POINT('Ctrl Pts',(30.3030266643161,-30.2626760833603,45.6652658085204));
#22034=CARTESIAN_POINT('Ctrl Pts',(29.6199973275285,-32.4833220172713,45.7763955977403));
#22035=CARTESIAN_POINT('Ctrl Pts',(31.1151206265327,-34.2616368823846,45.88752538696));
#22036=CARTESIAN_POINT('Ctrl Pts',(33.3805969835407,-33.9751191529232,45.9967517608673));
#22037=CARTESIAN_POINT('Ctrl Pts',(34.0552776453628,-32.6447171754051,46.0689348717015));
#22038=CARTESIAN_POINT('Ctrl Pts',(34.0579058351471,-31.9993626137656,46.1040747194623));
#22039=CARTESIAN_POINT('Ctrl Pts',(34.0572106602559,-32.0012284763882,45.3459252805377));
#22040=CARTESIAN_POINT('Ctrl Pts',(34.0529103405582,-31.3929993751285,45.3790140432881));
#22041=CARTESIAN_POINT('Ctrl Pts',(33.4453451554924,-30.0963857660314,45.4491460691118));
#22042=CARTESIAN_POINT('Ctrl Pts',(31.2413200309736,-29.6929634802401,45.5563213580089));
#22043=CARTESIAN_POINT('Ctrl Pts',(29.6503075674633,-31.3860307243948,45.6674511472285));
#22044=CARTESIAN_POINT('Ctrl Pts',(30.2097081368571,-33.6409959913638,45.7785809364483));
#22045=CARTESIAN_POINT('Ctrl Pts',(32.4075644044926,-34.3941395228971,45.8897107256679));
#22046=CARTESIAN_POINT('Ctrl Pts',(33.8709146012435,-33.2410523704688,45.9788255070311));
#22047=CARTESIAN_POINT('Ctrl Pts',(34.0531293619917,-32.2790855330859,46.030897025321));
#22048=CARTESIAN_POINT('Ctrl Pts',(34.0518959520928,-32.0010072981031,46.0459252805377));
#22049=CARTESIAN_POINT('Origin',(32.,-32.,39.4540747194623));
#22050=CARTESIAN_POINT('',(34.0556200578454,-31.9982099716569,44.6459252805377));
#22051=CARTESIAN_POINT('',(34.0525927001132,-32.0014692602189,44.7040747194623));
#22052=CARTESIAN_POINT('',(34.05475,-31.9999999999998,39.4540747194623));
#22053=CARTESIAN_POINT('Ctrl Pts',(34.0525927001132,-32.0014692602189,44.7040747194623));
#22054=CARTESIAN_POINT('Ctrl Pts',(34.0496527323428,-31.5568170867306,44.7281256445624));
#22055=CARTESIAN_POINT('Ctrl Pts',(33.689290920656,-30.4229699899486,44.7892198327358));
#22056=CARTESIAN_POINT('Ctrl Pts',(31.819615432301,-29.5781258700983,44.8873572839824));
#22057=CARTESIAN_POINT('Ctrl Pts',(29.8675011150493,-30.8379064585695,44.9984870732022));
#22058=CARTESIAN_POINT('Ctrl Pts',(29.867026651317,-33.1612224537781,45.1096168624218));
#22059=CARTESIAN_POINT('Ctrl Pts',(31.8186262651666,-34.4218002522221,45.2207466516416));
#22060=CARTESIAN_POINT('Ctrl Pts',(33.6889356864207,-33.5775893888604,45.3188992706551));
#22061=CARTESIAN_POINT('Ctrl Pts',(34.0496506626755,-32.4434570680596,45.3800086265953));
#22062=CARTESIAN_POINT('Ctrl Pts',(34.0525988691351,-31.9985278358415,45.4040747194623));
#22063=CARTESIAN_POINT('Ctrl Pts',(34.0556200578454,-31.9982099716569,44.6459252805377));
#22064=CARTESIAN_POINT('Ctrl Pts',(34.0568191781729,-31.8670821375068,44.6530445351088));
#22065=CARTESIAN_POINT('Ctrl Pts',(33.9856534619524,-31.054959944858,44.6972070527531));
#22066=CARTESIAN_POINT('Ctrl Pts',(32.9043976734169,-29.7460972409556,44.7784128334707));
#22067=CARTESIAN_POINT('Ctrl Pts',(30.5970084672143,-30.0176711781749,44.8895426226904));
#22068=CARTESIAN_POINT('Ctrl Pts',(29.573621897008,-32.1034509556668,45.0006724119102));
#22069=CARTESIAN_POINT('Ctrl Pts',(30.770830253685,-34.0945535404118,45.1118022011299));
#22070=CARTESIAN_POINT('Ctrl Pts',(33.0929614323987,-34.168743439459,45.2229319903496));
#22071=CARTESIAN_POINT('Ctrl Pts',(34.0212425079456,-32.8270078695086,45.3009730168189));
#22072=CARTESIAN_POINT('Ctrl Pts',(34.0577245995579,-32.0739190812136,45.3419707802149));
#22073=CARTESIAN_POINT('Ctrl Pts',(34.0572106602559,-32.0012284763882,45.3459252805377));
#22074=CARTESIAN_POINT('Origin',(32.,-32.,39.4540747194623));
#22075=CARTESIAN_POINT('',(34.0514131663913,-31.9999002048757,43.9459252805377));
#22076=CARTESIAN_POINT('',(34.0579021590917,-32.0006422250077,44.0040747194623));
#22077=CARTESIAN_POINT('',(34.05475,-31.9999999999998,39.4540747194623));
#22078=CARTESIAN_POINT('Ctrl Pts',(34.0579021590918,-32.0006422250077,44.0040747194623));
#22079=CARTESIAN_POINT('Ctrl Pts',(34.0552574521282,-31.3555631515598,44.0391993994563));
#22080=CARTESIAN_POINT('Ctrl Pts',(33.3810889993931,-30.0254049823542,44.1113673425236));
#22081=CARTESIAN_POINT('Ctrl Pts',(31.116044435755,-29.7380018890796,44.220578548664));
#22082=CARTESIAN_POINT('Ctrl Pts',(29.6201949324755,-31.5157059427025,44.3317083378838));
#22083=CARTESIAN_POINT('Ctrl Pts',(30.3023172190834,-33.7366306656069,44.4428381271035));
#22084=CARTESIAN_POINT('Ctrl Pts',(32.538140376183,-34.3682098363267,44.5539679163233));
#22085=CARTESIAN_POINT('Ctrl Pts',(33.9041699601015,-33.1648057121054,44.6410467804428));
#22086=CARTESIAN_POINT('Ctrl Pts',(34.0541808741541,-32.2416708863265,44.6910823814892));
#22087=CARTESIAN_POINT('Ctrl Pts',(34.0525927001132,-32.0014692602189,44.7040747194623));
#22088=CARTESIAN_POINT('Ctrl Pts',(34.0514131663913,-31.9999002048757,43.9459252805377));
#22089=CARTESIAN_POINT('Ctrl Pts',(34.0515591161687,-31.6630643659418,43.9641182900027));
#22090=CARTESIAN_POINT('Ctrl Pts',(33.8137553061809,-30.6405823346687,44.0193545625409));
#22091=CARTESIAN_POINT('Ctrl Pts',(32.2023029066813,-29.5798581998207,44.1116340981523));
#22092=CARTESIAN_POINT('Ctrl Pts',(30.0765282356173,-30.5173438798798,44.2227638873721));
#22093=CARTESIAN_POINT('Ctrl Pts',(29.7110940641655,-32.8117403622951,44.3338936765918));
#22094=CARTESIAN_POINT('Ctrl Pts',(31.4404417830221,-34.3632408681166,44.4450234658115));
#22095=CARTESIAN_POINT('Ctrl Pts',(33.5382982167491,-33.7910911423125,44.5490340004602));
#22096=CARTESIAN_POINT('Ctrl Pts',(34.0505798550385,-32.5493730723421,44.6160012720355));
#22097=CARTESIAN_POINT('Ctrl Pts',(34.0556200578454,-31.9982099716569,44.6459252805377));
#22098=CARTESIAN_POINT('Origin',(32.,-32.,39.4540747194623));
#22099=CARTESIAN_POINT('',(34.055253827614,-32.0018424470648,43.2459252805377));
#22100=CARTESIAN_POINT('',(34.0544840782063,-31.9981228849384,43.3040747194623));
#22101=CARTESIAN_POINT('',(34.05475,-31.9999999999998,39.4540747194623));
#22102=CARTESIAN_POINT('Ctrl Pts',(34.0544840782063,-31.9981228849384,43.3040747194623));
#22103=CARTESIAN_POINT('Ctrl Pts',(34.0560152931149,-31.8292568267182,43.313229891277));
#22104=CARTESIAN_POINT('Ctrl Pts',(33.9597518145395,-30.9788546094819,43.3594283261648));
#22105=CARTESIAN_POINT('Ctrl Pts',(32.7795349677293,-29.699926495664,43.442670024126));
#22106=CARTESIAN_POINT('Ctrl Pts',(30.490493436163,-30.0975271807692,43.5537998133457));
#22107=CARTESIAN_POINT('Ctrl Pts',(29.5829359418664,-32.2362503593823,43.6649296025654));
#22108=CARTESIAN_POINT('Ctrl Pts',(30.887449261624,-34.1587597707098,43.7760593917852));
#22109=CARTESIAN_POINT('Ctrl Pts',(33.2101569520236,-34.1055956508643,43.8871891810049));
#22110=CARTESIAN_POINT('Ctrl Pts',(34.0412597763805,-32.7512874803452,43.9631942902306));
#22111=CARTESIAN_POINT('Ctrl Pts',(34.058046618487,-32.0358777857388,44.0021561363831));
#22112=CARTESIAN_POINT('Ctrl Pts',(34.0579021590918,-32.0006422250077,44.0040747194623));
#22113=CARTESIAN_POINT('Ctrl Pts',(34.055253827614,-32.0018424470648,43.2459252805377));
#22114=CARTESIAN_POINT('Ctrl Pts',(34.0502763403136,-31.462537786081,43.2751920448965));
#22115=CARTESIAN_POINT('Ctrl Pts',(33.5565644616089,-30.2325636359862,43.3415020723286));
#22116=CARTESIAN_POINT('Ctrl Pts',(31.4823524106659,-29.6272265641889,43.444855362834));
#22117=CARTESIAN_POINT('Ctrl Pts',(29.725818144952,-31.1478792982686,43.5559851520537));
#22118=CARTESIAN_POINT('Ctrl Pts',(30.0505904524204,-33.4483836551904,43.6671149412735));
#22119=CARTESIAN_POINT('Ctrl Pts',(32.1594412363987,-34.4233429992207,43.7782447304931));
#22120=CARTESIAN_POINT('Ctrl Pts',(33.8010224036592,-33.3839528343674,43.8711815102479));
#22121=CARTESIAN_POINT('Ctrl Pts',(34.0512619440044,-32.3489046398197,43.9270750269294));
#22122=CARTESIAN_POINT('Ctrl Pts',(34.0514131663913,-31.9999002048757,43.9459252805377));
#22123=CARTESIAN_POINT('Origin',(32.,-32.,39.4540747194623));
#22124=CARTESIAN_POINT('',(34.0574728862044,-31.9989451473756,42.5459252805377));
#22125=CARTESIAN_POINT('',(34.0515269223438,-32.0005123640606,42.6040747194623));
#22126=CARTESIAN_POINT('',(34.05475,-31.9999999999998,39.4540747194623));
#22127=CARTESIAN_POINT('Ctrl Pts',(34.0515269223438,-32.0005123640606,42.6040747194623));
#22128=CARTESIAN_POINT('Ctrl Pts',(34.0506911852892,-31.6260341786675,42.6243036461709));
#22129=CARTESIAN_POINT('Ctrl Pts',(33.7733218188497,-30.564657819967,42.6815758359526));
#22130=CARTESIAN_POINT('Ctrl Pts',(32.0693858594061,-29.572408937857,42.7758912888076));
#22131=CARTESIAN_POINT('Ctrl Pts',(29.9981750364838,-30.6249691844573,42.8870210780273));
#22132=CARTESIAN_POINT('Ctrl Pts',(29.7590127090568,-32.9359427703937,42.9981508672471));
#22133=CARTESIAN_POINT('Ctrl Pts',(31.5707776489307,-34.3903516582226,43.1092806564667));
#22134=CARTESIAN_POINT('Ctrl Pts',(33.5937426045007,-33.717540873949,43.2112552738719));
#22135=CARTESIAN_POINT('Ctrl Pts',(34.0498197571019,-32.5125154203786,43.2761866282037));
#22136=CARTESIAN_POINT('Ctrl Pts',(34.0544840782063,-31.9981228849384,43.3040747194623));
#22137=CARTESIAN_POINT('Ctrl Pts',(34.0574728862044,-31.9989451473756,42.5459252805377));
#22138=CARTESIAN_POINT('Ctrl Pts',(34.057852200887,-31.9383561660562,42.5492225367172));
#22139=CARTESIAN_POINT('Ctrl Pts',(34.0279453325407,-31.1974556320969,42.5895630559699));
#22140=CARTESIAN_POINT('Ctrl Pts',(33.1311710515888,-29.8509388446871,42.6669468382959));
#22141=CARTESIAN_POINT('Ctrl Pts',(30.8080907702464,-29.8840214107802,42.7780766275156));
#22142=CARTESIAN_POINT('Ctrl Pts',(29.5758326618125,-31.8536249348858,42.8892064167354));
#22143=CARTESIAN_POINT('Ctrl Pts',(30.5621463276885,-33.9571891796694,43.0003362059551));
#22144=CARTESIAN_POINT('Ctrl Pts',(32.8643680232945,-34.2695551886057,43.1114659951748));
#22145=CARTESIAN_POINT('Ctrl Pts',(33.9775551442909,-32.9695959350558,43.1933290200357));
#22146=CARTESIAN_POINT('Ctrl Pts',(34.0565764003152,-32.1451415815839,43.2381487818233));
#22147=CARTESIAN_POINT('Ctrl Pts',(34.055253827614,-32.0018424470648,43.2459252805377));
#22148=CARTESIAN_POINT('Origin',(32.,-32.,39.4540747194623));
#22149=CARTESIAN_POINT('',(34.0520872241698,-31.9988339725263,41.8459252805377));
#22150=CARTESIAN_POINT('',(34.056362032224,-32.0016080177294,41.9040747194623));
#22151=CARTESIAN_POINT('',(34.05475,-31.9999999999998,39.4540747194623));
#22152=CARTESIAN_POINT('Ctrl Pts',(34.056362032224,-32.0016080177294,41.9040747194623));
#22153=CARTESIAN_POINT('Ctrl Pts',(34.0514108335821,-31.4255899016838,41.9353774010647));
#22154=CARTESIAN_POINT('Ctrl Pts',(33.4988294221162,-30.1595906875508,42.0037233457404));
#22155=CARTESIAN_POINT('Ctrl Pts',(31.3531125199586,-29.6591578453596,42.1091125534892));
#22156=CARTESIAN_POINT('Ctrl Pts',(29.6825424522475,-31.2737738490384,42.220242342709));
#22157=CARTESIAN_POINT('Ctrl Pts',(30.1328842664196,-33.553027071776,42.3313721319287));
#22158=CARTESIAN_POINT('Ctrl Pts',(32.2919902196474,-34.4109652846105,42.4425019211484));
#22159=CARTESIAN_POINT('Ctrl Pts',(33.8394914966062,-33.3078912260223,42.5334027836596));
#22160=CARTESIAN_POINT('Ctrl Pts',(34.052221589152,-32.3117796033549,42.5872603830976));
#22161=CARTESIAN_POINT('Ctrl Pts',(34.0515269223438,-32.0005123640606,42.6040747194623));
#22162=CARTESIAN_POINT('Ctrl Pts',(34.0520872241698,-31.9988339725263,41.8459252805377));
#22163=CARTESIAN_POINT('Ctrl Pts',(34.053468796887,-31.732976645908,41.860296291611));
#22164=CARTESIAN_POINT('Ctrl Pts',(33.8819549522473,-30.7835444255121,41.9117105657577));
#22165=CARTESIAN_POINT('Ctrl Pts',(32.4498627695247,-29.6134582253175,42.0001681029775));
#22166=CARTESIAN_POINT('Ctrl Pts',(30.2390335714705,-30.327572605785,42.1112978921973));
#22167=CARTESIAN_POINT('Ctrl Pts',(29.6398080047623,-32.5722924533201,42.222427681417));
#22168=CARTESIAN_POINT('Ctrl Pts',(31.200611501379,-34.2932473343971,42.3335574706367));
#22169=CARTESIAN_POINT('Ctrl Pts',(33.4249871850401,-33.9266610466994,42.441390003677));
#22170=CARTESIAN_POINT('Ctrl Pts',(34.0535907626447,-32.6190474597171,42.5121792736439));
#22171=CARTESIAN_POINT('Ctrl Pts',(34.0574728862044,-31.9989451473756,42.5459252805377));
#22172=CARTESIAN_POINT('Origin',(32.,-32.,39.4540747194623));
#22173=CARTESIAN_POINT('',(34.0526762468981,-32.0023611642388,41.1459252805377));
#22174=CARTESIAN_POINT('',(34.0565678057143,-31.9985073856871,41.2040747194623));
#22175=CARTESIAN_POINT('',(34.05475,-31.9999999999998,39.4540747194623));
#22176=CARTESIAN_POINT('',(32.5301702171886,-33.9851743256717,41.));
#22177=CARTESIAN_POINT('Ctrl Pts',(32.5301702171886,-33.9851743256717,41.));
#22178=CARTESIAN_POINT('Ctrl Pts',(33.1902397907527,-33.8088929660699,41.0370432630732));
#22179=CARTESIAN_POINT('Ctrl Pts',(33.9249254184578,-33.112877718512,41.0856850232525));
#22180=CARTESIAN_POINT('Ctrl Pts',(34.0542946290731,-32.2166573957683,41.1343267834317));
#22181=CARTESIAN_POINT('Ctrl Pts',(34.0526762468981,-32.0023611642388,41.1459252805377));
#22182=CARTESIAN_POINT('',(31.4686978381225,-33.9887332741258,41.));
#22183=CARTESIAN_POINT('Origin',(32.,-32.,41.));
#22184=CARTESIAN_POINT('Ctrl Pts',(31.4686972148566,-33.9887352337366,41.));
#22185=CARTESIAN_POINT('Ctrl Pts',(32.1131669671016,-34.1600186174424,41.0363148168372));
#22186=CARTESIAN_POINT('Ctrl Pts',(33.4928784097068,-33.8407638650999,41.1043397233247));
#22187=CARTESIAN_POINT('Ctrl Pts',(34.051713710007,-32.5817335385731,41.1723646298121));
#22188=CARTESIAN_POINT('Ctrl Pts',(34.0565678057143,-31.9985073856871,41.2040747194623));
#22189=CARTESIAN_POINT('Origin',(32.,32.,48.));
#22190=CARTESIAN_POINT('',(33.6684806121724,32.0006140895871,53.3285196366098));
#22191=CARTESIAN_POINT('',(33.6648118697033,32.0014849556936,53.5214803633902));
#22192=CARTESIAN_POINT('',(33.666,32.,48.));
#22193=CARTESIAN_POINT('',(31.3249228143251,30.4769022377466,54.));
#22194=CARTESIAN_POINT('Ctrl Pts',(33.6648118697033,32.0014849556936,53.5214803633902));
#22195=CARTESIAN_POINT('Ctrl Pts',(33.6661630022499,32.1712284034164,53.5328138566339));
#22196=CARTESIAN_POINT('Ctrl Pts',(33.6422867953324,32.3405891079999,53.5441473498775));
#22197=CARTESIAN_POINT('Ctrl Pts',(33.591605099642,32.5014829336479,53.5554808431211));
#22198=CARTESIAN_POINT('Ctrl Pts',(33.4259531381418,33.0273607175068,53.5925241061943));
#22199=CARTESIAN_POINT('Ctrl Pts',(32.9739396808446,33.4627873203686,53.6295673692676));
#22200=CARTESIAN_POINT('Ctrl Pts',(32.4421423739696,33.6090004012271,53.6666106323408));
#22201=CARTESIAN_POINT('Ctrl Pts',(31.9103450670946,33.7552134820855,53.7036538954141));
#22202=CARTESIAN_POINT('Ctrl Pts',(31.2987639106417,33.6122130409406,53.7406971584873));
#22203=CARTESIAN_POINT('Ctrl Pts',(30.8877751036362,33.2444452260279,53.7777404215606));
#22204=CARTESIAN_POINT('Ctrl Pts',(30.4767862966307,32.8766774111153,53.8147836846338));
#22205=CARTESIAN_POINT('Ctrl Pts',(30.2663898390726,32.2841422224349,53.851826947707));
#22206=CARTESIAN_POINT('Ctrl Pts',(30.3518166376656,31.7403141445124,53.8888702107803));
#22207=CARTESIAN_POINT('Ctrl Pts',(30.4372434362585,31.1964860665899,53.9259134738535));
#22208=CARTESIAN_POINT('Ctrl Pts',(30.8184934910026,30.7013650994253,53.9629567369268));
#22209=CARTESIAN_POINT('Ctrl Pts',(31.3249228143251,30.4769022377466,54.));
#22210=CARTESIAN_POINT('',(33.666,32.,54.));
#22211=CARTESIAN_POINT('Origin',(32.,32.,54.));
#22212=CARTESIAN_POINT('',(33.666,32.,55.));
#22213=CARTESIAN_POINT('',(33.666,32.,48.));
#22214=CARTESIAN_POINT('Origin',(32.,32.,55.));
#22215=CARTESIAN_POINT('',(33.6146716715671,31.5775323837617,54.));
#22216=CARTESIAN_POINT('Origin',(32.,32.,54.));
#22217=CARTESIAN_POINT('Ctrl Pts',(33.614673303851,31.5775320375437,54.));
#22218=CARTESIAN_POINT('Ctrl Pts',(33.477140483944,31.0546378042632,53.9636851831628));
#22219=CARTESIAN_POINT('Ctrl Pts',(33.061847656895,30.6037761189473,53.9273703663256));
#22220=CARTESIAN_POINT('Ctrl Pts',(32.5515252260834,30.4251374099372,53.8910555494883));
#22221=CARTESIAN_POINT('Ctrl Pts',(32.0309661346949,30.2429153510298,53.8540122864151));
#22222=CARTESIAN_POINT('Ctrl Pts',(31.411526766352,30.3439469543993,53.8169690233418));
#22223=CARTESIAN_POINT('Ctrl Pts',(30.9761676297192,30.6822522118738,53.7799257602686));
#22224=CARTESIAN_POINT('Ctrl Pts',(30.5408084930864,31.0205574693483,53.7428824971953));
#22225=CARTESIAN_POINT('Ctrl Pts',(30.2895295881637,31.5961363809279,53.7058392341221));
#22226=CARTESIAN_POINT('Ctrl Pts',(30.3375623462193,32.1454810048324,53.6687959710489));
#22227=CARTESIAN_POINT('Ctrl Pts',(30.3855951042748,32.6948256287369,53.6317527079756));
#22228=CARTESIAN_POINT('Ctrl Pts',(30.7329395253087,33.2179359649664,53.5947094449023));
#22229=CARTESIAN_POINT('Ctrl Pts',(31.2205276954254,33.4755032093286,53.5576661818291));
#22230=CARTESIAN_POINT('Ctrl Pts',(31.7081158655422,33.7330704536908,53.5206229187558));
#22231=CARTESIAN_POINT('Ctrl Pts',(32.3359477847419,33.7250946061857,53.4835796556826));
#22232=CARTESIAN_POINT('Ctrl Pts',(32.8167941016275,33.4551932266985,53.4465363926094));
#22233=CARTESIAN_POINT('Ctrl Pts',(33.297640418513,33.1852918472114,53.4094931295362));
#22234=CARTESIAN_POINT('Ctrl Pts',(33.6315011330843,32.6534649357421,53.3724498664629));
#22235=CARTESIAN_POINT('Ctrl Pts',(33.6655715042332,32.1030898398486,53.3354066033897));
#22236=CARTESIAN_POINT('Ctrl Pts',(33.667682922926,32.0689818384882,53.3331109477964));
#22237=CARTESIAN_POINT('Ctrl Pts',(33.6686429776493,32.0348026016404,53.3308152922031));
#22238=CARTESIAN_POINT('Ctrl Pts',(33.6684806121724,32.0006140895871,53.3285196366098));
#22239=CARTESIAN_POINT('Origin',(32.,32.,48.));
#22240=CARTESIAN_POINT('',(33.6641301442348,32.00113043568,52.6285196366098));
#22241=CARTESIAN_POINT('',(33.6637770221358,31.9991035482978,52.8214803633902));
#22242=CARTESIAN_POINT('',(33.666,32.,48.));
#22243=CARTESIAN_POINT('Ctrl Pts',(33.6637770221358,31.9991035482978,52.8214803633902));
#22244=CARTESIAN_POINT('Ctrl Pts',(33.6621336119821,32.3352311296541,52.8438876115277));
#22245=CARTESIAN_POINT('Ctrl Pts',(33.5633565172328,32.6722466375241,52.8662948596652));
#22246=CARTESIAN_POINT('Ctrl Pts',(33.3740882433209,32.9469019105991,52.8887021078027));
#22247=CARTESIAN_POINT('Ctrl Pts',(33.0611933077665,33.400957110619,52.9257453708759));
#22248=CARTESIAN_POINT('Ctrl Pts',(32.5009849585214,33.6845810853147,52.9627886339492));
#22249=CARTESIAN_POINT('Ctrl Pts',(31.9498071626783,33.6679970783992,52.9998318970225));
#22250=CARTESIAN_POINT('Ctrl Pts',(31.3986293668351,33.6514130714837,53.0368751600957));
#22251=CARTESIAN_POINT('Ctrl Pts',(30.856482124394,33.3346210829571,53.073918423169));
#22252=CARTESIAN_POINT('Ctrl Pts',(30.5714576575436,32.862567499063,53.1109616862422));
#22253=CARTESIAN_POINT('Ctrl Pts',(30.2864331906931,32.3905139151689,53.1480049493154));
#22254=CARTESIAN_POINT('Ctrl Pts',(30.2585314994335,31.7631987359073,53.1850482123887));
#22255=CARTESIAN_POINT('Ctrl Pts',(30.5005032533944,31.2677094825492,53.2220914754619));
#22256=CARTESIAN_POINT('Ctrl Pts',(30.7424750073553,30.7722202291911,53.2591347385351));
#22257=CARTESIAN_POINT('Ctrl Pts',(31.2543202065367,30.4085569017365,53.2961780016084));
#22258=CARTESIAN_POINT('Ctrl Pts',(31.8018549039325,30.3430675123084,53.3332212646817));
#22259=CARTESIAN_POINT('Ctrl Pts',(32.3493896013283,30.2775781228804,53.3702645277549));
#22260=CARTESIAN_POINT('Ctrl Pts',(32.9326137969385,30.510262671479,53.4073077908281));
#22261=CARTESIAN_POINT('Ctrl Pts',(33.284580661892,30.9347694282061,53.4443510539014));
#22262=CARTESIAN_POINT('Ctrl Pts',(33.5288622487411,31.2293971175917,53.470060823731));
#22263=CARTESIAN_POINT('Ctrl Pts',(33.6617468564691,31.6164258325067,53.4957705935606));
#22264=CARTESIAN_POINT('Ctrl Pts',(33.6648118697033,32.0014849556936,53.5214803633902));
#22265=CARTESIAN_POINT('Ctrl Pts',(33.6684806121724,32.0006140895871,53.3285196366098));
#22266=CARTESIAN_POINT('Ctrl Pts',(33.6660230083945,31.4831283654114,53.2937720291298));
#22267=CARTESIAN_POINT('Ctrl Pts',(33.4064122708611,30.963517636581,53.2590244216499));
#22268=CARTESIAN_POINT('Ctrl Pts',(32.9900197135209,30.6566480056464,53.2242768141699));
#22269=CARTESIAN_POINT('Ctrl Pts',(32.5461175239329,30.3295045476556,53.1872335510967));
#22270=CARTESIAN_POINT('Ctrl Pts',(31.9240331170303,30.2441409119919,53.1501902880235));
#22271=CARTESIAN_POINT('Ctrl Pts',(31.4084208079463,30.4396231782327,53.1131470249502));
#22272=CARTESIAN_POINT('Ctrl Pts',(30.8928084988622,30.6351054444736,53.076103761877));
#22273=CARTESIAN_POINT('Ctrl Pts',(30.4836682875968,31.1114336126191,53.0390604988037));
#22274=CARTESIAN_POINT('Ctrl Pts',(30.3682246262316,31.650640403094,53.0020172357305));
#22275=CARTESIAN_POINT('Ctrl Pts',(30.2527809648664,32.1898471935689,52.9649739726572));
#22276=CARTESIAN_POINT('Ctrl Pts',(30.4310338534015,32.7919326063733,52.927930709584));
#22277=CARTESIAN_POINT('Ctrl Pts',(30.8214136605767,33.1813866783119,52.8908874465107));
#22278=CARTESIAN_POINT('Ctrl Pts',(31.2117934677519,33.5708407502506,52.8538441834375));
#22279=CARTESIAN_POINT('Ctrl Pts',(31.8143001935672,33.7476634813236,52.8168009203643));
#22280=CARTESIAN_POINT('Ctrl Pts',(32.3532310758874,33.6309412146398,52.779757657291));
#22281=CARTESIAN_POINT('Ctrl Pts',(32.8921619582076,33.514218947956,52.7427143942178));
#22282=CARTESIAN_POINT('Ctrl Pts',(33.3675169970328,33.1039516835154,52.7056711311445));
#22283=CARTESIAN_POINT('Ctrl Pts',(33.5617757744068,32.5878757666476,52.6686278680713));
#22284=CARTESIAN_POINT('Ctrl Pts',(33.6318863726636,32.4016170463641,52.6552584575841));
#22285=CARTESIAN_POINT('Ctrl Pts',(33.6653817959804,32.2015758506439,52.641889047097));
#22286=CARTESIAN_POINT('Ctrl Pts',(33.6641301442348,32.00113043568,52.6285196366098));
#22287=CARTESIAN_POINT('Origin',(32.,32.,48.));
#22288=CARTESIAN_POINT('',(33.6643836268795,31.9987501844045,51.9285196366098));
#22289=CARTESIAN_POINT('',(33.6681252089806,31.9990863473496,52.1214803633902));
#22290=CARTESIAN_POINT('',(33.666,32.,48.));
#22291=CARTESIAN_POINT('Ctrl Pts',(33.6681252089806,31.9990863473496,52.1214803633902));
#22292=CARTESIAN_POINT('Ctrl Pts',(33.6648306921651,32.4979846701634,52.1549613664216));
#22293=CARTESIAN_POINT('Ctrl Pts',(33.4261511788098,32.999617402672,52.188442369453));
#22294=CARTESIAN_POINT('Ctrl Pts',(33.0352551287758,33.3088117148578,52.2219233724844));
#22295=CARTESIAN_POINT('Ctrl Pts',(32.6027691246341,33.6509032058539,52.2589666355576));
#22296=CARTESIAN_POINT('Ctrl Pts',(31.983952861432,33.7574283024602,52.2960098986309));
#22297=CARTESIAN_POINT('Ctrl Pts',(31.461973233789,33.5796418315865,52.3330531617041));
#22298=CARTESIAN_POINT('Ctrl Pts',(30.9399936061459,33.4018553607128,52.3700964247774));
#22299=CARTESIAN_POINT('Ctrl Pts',(30.5148506140619,32.9397573223592,52.4071396878506));
#22300=CARTESIAN_POINT('Ctrl Pts',(30.3810875280695,32.4048010089502,52.4441829509238));
#22301=CARTESIAN_POINT('Ctrl Pts',(30.2473244420771,31.8698446955412,52.481226213997));
#22302=CARTESIAN_POINT('Ctrl Pts',(30.4049412621763,31.2620301070768,52.5182694770704));
#22303=CARTESIAN_POINT('Ctrl Pts',(30.7818131038358,30.859490426737,52.5553127401436));
#22304=CARTESIAN_POINT('Ctrl Pts',(31.1586849454953,30.4569507463972,52.5923560032168));
#22305=CARTESIAN_POINT('Ctrl Pts',(31.7548118087151,30.2596859741819,52.62939926629));
#22306=CARTESIAN_POINT('Ctrl Pts',(32.297409832103,30.357962364395,52.6664425293633));
#22307=CARTESIAN_POINT('Ctrl Pts',(32.8400078554909,30.4562387546082,52.7034857924365));
#22308=CARTESIAN_POINT('Ctrl Pts',(33.3290770390468,30.8500563072498,52.7405290555098));
#22309=CARTESIAN_POINT('Ctrl Pts',(33.5408208698929,31.3592082962425,52.7775723185831));
#22310=CARTESIAN_POINT('Ctrl Pts',(33.6244821246988,31.5603772942523,52.7922083335188));
#22311=CARTESIAN_POINT('Ctrl Pts',(33.6648504683442,31.7795510057075,52.8068443484545));
#22312=CARTESIAN_POINT('Ctrl Pts',(33.6637770221358,31.9991035482978,52.8214803633902));
#22313=CARTESIAN_POINT('Ctrl Pts',(33.6641301442348,32.00113043568,52.6285196366098));
#22314=CARTESIAN_POINT('Ctrl Pts',(33.6619137848118,31.6461921824217,52.6048457840238));
#22315=CARTESIAN_POINT('Ctrl Pts',(33.5507463265447,31.2899864805881,52.5811719314377));
#22316=CARTESIAN_POINT('Ctrl Pts',(33.3409999515945,31.0067929294096,52.5574980788516));
#22317=CARTESIAN_POINT('Ctrl Pts',(33.0128028354855,30.5636705783342,52.5204548157784));
#22318=CARTESIAN_POINT('Ctrl Pts',(32.4432460873448,30.2993104454786,52.4834115527051));
#22319=CARTESIAN_POINT('Ctrl Pts',(31.8929556516761,30.3346823630194,52.4463682896318));
#22320=CARTESIAN_POINT('Ctrl Pts',(31.3426652160074,30.3700542805602,52.4093250265586));
#22321=CARTESIAN_POINT('Ctrl Pts',(30.8116410928108,30.7051582484975,52.3722817634854));
#22322=CARTESIAN_POINT('Ctrl Pts',(30.5428771097717,31.1866524733684,52.3352385004122));
#22323=CARTESIAN_POINT('Ctrl Pts',(30.2741131267324,31.6681466982393,52.2981952373389));
#22324=CARTESIAN_POINT('Ctrl Pts',(30.2676092838506,32.2960311800439,52.2611519742656));
#22325=CARTESIAN_POINT('Ctrl Pts',(30.5263416698789,32.7829894020285,52.2241087111924));
#22326=CARTESIAN_POINT('Ctrl Pts',(30.7850740559072,33.2699476240131,52.1870654481191));
#22327=CARTESIAN_POINT('Ctrl Pts',(31.3090426708456,33.6159795861778,52.1500221850459));
#22328=CARTESIAN_POINT('Ctrl Pts',(31.8584823350187,33.662742930047,52.1129789219727));
#22329=CARTESIAN_POINT('Ctrl Pts',(32.4079219991918,33.7095062739161,52.0759356588994));
#22330=CARTESIAN_POINT('Ctrl Pts',(32.9828327125997,33.4570009994898,52.0388923958262));
#22331=CARTESIAN_POINT('Ctrl Pts',(33.3201384413117,33.0207721556727,52.0018491327529));
#22332=CARTESIAN_POINT('Ctrl Pts',(33.542711158369,32.7329245718267,51.9774059673719));
#22333=CARTESIAN_POINT('Ctrl Pts',(33.6618287603767,32.3650822730844,51.9529628019908));
#22334=CARTESIAN_POINT('Ctrl Pts',(33.6643836268795,31.9987501844045,51.9285196366098));
#22335=CARTESIAN_POINT('Origin',(32.,32.,48.));
#22336=CARTESIAN_POINT('',(33.6686262728084,31.9995820848651,51.2285196366098));
#22337=CARTESIAN_POINT('',(33.6665286630119,32.001478985866,51.4214803633902));
#22338=CARTESIAN_POINT('',(33.666,32.,48.));
#22339=CARTESIAN_POINT('Ctrl Pts',(33.6665286630119,32.001478985866,51.4214803633902));
#22340=CARTESIAN_POINT('Ctrl Pts',(33.6675619157926,32.1136863591203,51.4289918582423));
#22341=CARTESIAN_POINT('Ctrl Pts',(33.6571969840449,32.2257039247924,51.4365033530943));
#22342=CARTESIAN_POINT('Ctrl Pts',(33.6347339453088,32.3352404902405,51.4440148479463));
#22343=CARTESIAN_POINT('Ctrl Pts',(33.5239564942531,32.8754248197198,51.4810581110195));
#22344=CARTESIAN_POINT('Ctrl Pts',(33.1189516224042,33.3552709245807,51.5181013740928));
#22345=CARTESIAN_POINT('Ctrl Pts',(32.6050473636773,33.5552038279757,51.555144637166));
#22346=CARTESIAN_POINT('Ctrl Pts',(32.0911431049504,33.7551367313708,51.5921879002392));
#22347=CARTESIAN_POINT('Ctrl Pts',(31.4683394593454,33.6751564332998,51.6292311633125));
#22348=CARTESIAN_POINT('Ctrl Pts',(31.0216279968823,33.351861486703,51.6662744263857));
#22349=CARTESIAN_POINT('Ctrl Pts',(30.5749165344193,33.0285665401062,51.703317689459));
#22350=CARTESIAN_POINT('Ctrl Pts',(30.3042972550983,32.4619569449836,51.7403609525322));
#22351=CARTESIAN_POINT('Ctrl Pts',(30.3336040761335,31.9113101753598,51.7774042156055));
#22352=CARTESIAN_POINT('Ctrl Pts',(30.3629108971687,31.3606634057361,51.8144474786787));
#22353=CARTESIAN_POINT('Ctrl Pts',(30.6921438185601,30.8259794616112,51.851490741752));
#22354=CARTESIAN_POINT('Ctrl Pts',(31.1706476359806,30.5519268253061,51.8885340048252));
#22355=CARTESIAN_POINT('Ctrl Pts',(31.6491514534012,30.277874189001,51.9255772678984));
#22356=CARTESIAN_POINT('Ctrl Pts',(32.2769261668508,30.2644528605156,51.9626205309717));
#22357=CARTESIAN_POINT('Ctrl Pts',(32.7667054807056,30.5178043497829,51.9996637940449));
#22358=CARTESIAN_POINT('Ctrl Pts',(33.2564847945603,30.7711558390502,52.0367070571182));
#22359=CARTESIAN_POINT('Ctrl Pts',(33.6082687088201,31.2912801460702,52.0737503201914));
#22360=CARTESIAN_POINT('Ctrl Pts',(33.6610827934094,31.8401712422731,52.1107935832647));
#22361=CARTESIAN_POINT('Ctrl Pts',(33.6661616522239,31.8929552752419,52.1143558433065));
#22362=CARTESIAN_POINT('Ctrl Pts',(33.6684757338916,31.9460053342557,52.1179181033484));
#22363=CARTESIAN_POINT('Ctrl Pts',(33.6681252089806,31.9990863473496,52.1214803633902));
#22364=CARTESIAN_POINT('Ctrl Pts',(33.6643836268795,31.9987501844045,51.9285196366098));
#22365=CARTESIAN_POINT('Ctrl Pts',(33.6657006235542,31.8099112990475,51.9159195389176));
#22366=CARTESIAN_POINT('Ctrl Pts',(33.6360439504949,31.6214737147367,51.9033194412254));
#22367=CARTESIAN_POINT('Ctrl Pts',(33.5736181579473,31.444601776518,51.8907193435332));
#22368=CARTESIAN_POINT('Ctrl Pts',(33.390091401855,30.9246126543882,51.85367608046));
#22369=CARTESIAN_POINT('Ctrl Pts',(32.9233371456542,30.5045868233367,51.8166328173867));
#22370=CARTESIAN_POINT('Ctrl Pts',(32.3869396038679,30.3767258273003,51.7795895543135));
#22371=CARTESIAN_POINT('Ctrl Pts',(31.8505420620816,30.248864831264,51.7425462912403));
#22372=CARTESIAN_POINT('Ctrl Pts',(31.2445012347098,30.4131686702428,51.7055030281671));
#22373=CARTESIAN_POINT('Ctrl Pts',(30.8461381193723,30.7944527978433,51.6684597650938));
#22374=CARTESIAN_POINT('Ctrl Pts',(30.4477750040348,31.1757369254437,51.6314165020206));
#22375=CARTESIAN_POINT('Ctrl Pts',(30.2570896007315,31.7740013416658,51.5943732389473));
#22376=CARTESIAN_POINT('Ctrl Pts',(30.3613385154927,32.3154834938915,51.557329975874));
#22377=CARTESIAN_POINT('Ctrl Pts',(30.465587430254,32.8569656461173,51.5202867128007));
#22378=CARTESIAN_POINT('Ctrl Pts',(30.8647706630797,33.3416655343467,51.4832434497275));
#22379=CARTESIAN_POINT('Ctrl Pts',(31.3762241313992,33.5477871177545,51.4462001866543));
#22380=CARTESIAN_POINT('Ctrl Pts',(31.8876775997186,33.7539087011623,51.4091569235811));
#22381=CARTESIAN_POINT('Ctrl Pts',(32.5114013035318,33.6814519797484,51.3721136605078));
#22382=CARTESIAN_POINT('Ctrl Pts',(32.9619826578286,33.3635727564261,51.3350703974346));
#22383=CARTESIAN_POINT('Ctrl Pts',(33.3939981097689,33.0587915331986,51.2995534771596));
#22384=CARTESIAN_POINT('Ctrl Pts',(33.6668456803395,32.5283960695597,51.2640365568847));
#22385=CARTESIAN_POINT('Ctrl Pts',(33.6686262728084,31.9995820848651,51.2285196366098));
#22386=CARTESIAN_POINT('Origin',(32.,32.,48.));
#22387=CARTESIAN_POINT('',(33.6656098327441,32.0015149950249,50.5285196366098));
#22388=CARTESIAN_POINT('',(33.6632910880953,31.9999843288606,50.7214803633902));
#22389=CARTESIAN_POINT('',(33.666,32.,48.));
#22390=CARTESIAN_POINT('Ctrl Pts',(33.6632910880953,31.9999843288606,50.7214803633902));
#22391=CARTESIAN_POINT('Ctrl Pts',(33.6632676777025,32.2789818870778,50.7400656131361));
#22392=CARTESIAN_POINT('Ctrl Pts',(33.5968498065901,32.5579899196603,50.758650862882));
#22393=CARTESIAN_POINT('Ctrl Pts',(33.4640996397272,32.8007206148323,50.7772361126279));
#22394=CARTESIAN_POINT('Ctrl Pts',(33.1995081264924,33.2845202473439,50.8142793757012));
#22395=CARTESIAN_POINT('Ctrl Pts',(32.6714007905922,33.6242022625819,50.8513226387744));
#22396=CARTESIAN_POINT('Ctrl Pts',(32.1214366854017,33.6643300122038,50.8883659018477));
#22397=CARTESIAN_POINT('Ctrl Pts',(31.5714725802113,33.7044577618257,50.9254091649209));
#22398=CARTESIAN_POINT('Ctrl Pts',(30.9996517057307,33.4450312458314,50.9624524279942));
#22399=CARTESIAN_POINT('Ctrl Pts',(30.6676361935327,33.0047626312951,50.9994956910674));
#22400=CARTESIAN_POINT('Ctrl Pts',(30.3356206813347,32.5644940167588,51.0365389541406));
#22401=CARTESIAN_POINT('Ctrl Pts',(30.2434105314195,31.9433833036805,51.0735822172139));
#22402=CARTESIAN_POINT('Ctrl Pts',(30.4332006084387,31.4256473864592,51.1106254802871));
#22403=CARTESIAN_POINT('Ctrl Pts',(30.622990685458,30.907911469238,51.1476687433604));
#22404=CARTESIAN_POINT('Ctrl Pts',(31.0947809894117,30.4935503478738,51.1847120064336));
#22405=CARTESIAN_POINT('Ctrl Pts',(31.6326828353093,30.3721734248677,51.2217552695068));
#22406=CARTESIAN_POINT('Ctrl Pts',(32.1705846812069,30.2507965018616,51.2587985325801));
#22407=CARTESIAN_POINT('Ctrl Pts',(32.7745980690483,30.4224037772137,51.2958417956533));
#22408=CARTESIAN_POINT('Ctrl Pts',(33.1683297478377,30.8084686919385,51.3328850587266));
#22409=CARTESIAN_POINT('Ctrl Pts',(33.4822219839608,31.1162488018455,51.3624168269478));
#22410=CARTESIAN_POINT('Ctrl Pts',(33.6624663848319,31.5603308249559,51.391948595169));
#22411=CARTESIAN_POINT('Ctrl Pts',(33.6665286630119,32.001478985866,51.4214803633902));
#22412=CARTESIAN_POINT('Ctrl Pts',(33.6686262728084,31.9995820848651,51.2285196366098));
#22413=CARTESIAN_POINT('Ctrl Pts',(33.6687027939276,31.9768562569798,51.2269932938115));
#22414=CARTESIAN_POINT('Ctrl Pts',(33.668278692763,31.9541333498619,51.2254669510132));
#22415=CARTESIAN_POINT('Ctrl Pts',(33.6673450880065,31.9314313957851,51.2239406082149));
#22416=CARTESIAN_POINT('Ctrl Pts',(33.6446871591072,31.3804709836974,51.1868973451416));
#22417=CARTESIAN_POINT('Ctrl Pts',(33.3219322965282,30.8418518847528,51.1498540820684));
#22418=CARTESIAN_POINT('Ctrl Pts',(32.8467713752829,30.562043278107,51.1128108189951));
#22419=CARTESIAN_POINT('Ctrl Pts',(32.3716104540377,30.2822346714611,51.0757675559219));
#22420=CARTESIAN_POINT('Ctrl Pts',(31.7440434741263,30.261236557114,51.0387242928486));
#22421=CARTESIAN_POINT('Ctrl Pts',(31.2512416827347,30.5086575583237,51.0016810297754));
#22422=CARTESIAN_POINT('Ctrl Pts',(30.7584398913431,30.7560785595334,50.9646377667022));
#22423=CARTESIAN_POINT('Ctrl Pts',(30.4004032884713,31.2719186763,50.9275945036289));
#22424=CARTESIAN_POINT('Ctrl Pts',(30.3409674822114,31.8201322682224,50.8905512405557));
#22425=CARTESIAN_POINT('Ctrl Pts',(30.2815316759514,32.3683458601448,50.8535079774825));
#22426=CARTESIAN_POINT('Ctrl Pts',(30.5206966663033,32.9489329272231,50.8164647144092));
#22427=CARTESIAN_POINT('Ctrl Pts',(30.949021850505,33.2962199756621,50.7794214513359));
#22428=CARTESIAN_POINT('Ctrl Pts',(31.3773470347066,33.6435070241011,50.7423781882627));
#22429=CARTESIAN_POINT('Ctrl Pts',(31.994832412758,33.7574940539007,50.7053349251895));
#22430=CARTESIAN_POINT('Ctrl Pts',(32.5189200238354,33.5860212182949,50.6682916621162));
#22431=CARTESIAN_POINT('Ctrl Pts',(33.0430076349128,33.4145483826891,50.631248399043));
#22432=CARTESIAN_POINT('Ctrl Pts',(33.4736974790163,32.9576156816778,50.5942051359697));
#22433=CARTESIAN_POINT('Ctrl Pts',(33.6139082188038,32.4243130416287,50.5571618728965));
#22434=CARTESIAN_POINT('Ctrl Pts',(33.6500456862382,32.286861325614,50.5476144608009));
#22435=CARTESIAN_POINT('Ctrl Pts',(33.6668871327276,32.1443364875697,50.5380670487053));
#22436=CARTESIAN_POINT('Ctrl Pts',(33.6656098327441,32.0015149950249,50.5285196366098));
#22437=CARTESIAN_POINT('Origin',(32.,32.,48.));
#22438=CARTESIAN_POINT('',(33.6634354704477,31.999492392636,49.8285196366098));
#22439=CARTESIAN_POINT('',(33.6665861757579,31.9985292434177,50.0214803633902));
#22440=CARTESIAN_POINT('',(33.666,32.,48.));
#22441=CARTESIAN_POINT('Ctrl Pts',(33.6665861757579,31.9985292434177,50.0214803633902));
#22442=CARTESIAN_POINT('Ctrl Pts',(33.6625140098534,32.4415387358119,50.05113936803));
#22443=CARTESIAN_POINT('Ctrl Pts',(33.4805422963843,32.8875029945088,50.0807983726698));
#22444=CARTESIAN_POINT('Ctrl Pts',(33.1642404568284,33.1955272547085,50.1104573773096));
#22445=CARTESIAN_POINT('Ctrl Pts',(32.7691883505449,33.580240897061,50.1475006403828));
#22446=CARTESIAN_POINT('Ctrl Pts',(32.1645905457089,33.7497776897714,50.1845439034561));
#22447=CARTESIAN_POINT('Ctrl Pts',(31.6271077195186,33.6265585157702,50.2215871665293));
#22448=CARTESIAN_POINT('Ctrl Pts',(31.0896248933283,33.503339341769,50.2586304296025));
#22449=CARTESIAN_POINT('Ctrl Pts',(30.6192570457837,33.0873642010562,50.2956736926758));
#22450=CARTESIAN_POINT('Ctrl Pts',(30.4312419534573,32.5689810624913,50.332716955749));
#22451=CARTESIAN_POINT('Ctrl Pts',(30.2432268611308,32.0505979239263,50.3697602188223));
#22452=CARTESIAN_POINT('Ctrl Pts',(30.3375645240227,31.4298067875093,50.4068034818955));
#22453=CARTESIAN_POINT('Ctrl Pts',(30.6710865391189,30.9906783111636,50.4438467449688));
#22454=CARTESIAN_POINT('Ctrl Pts',(31.004608554215,30.5515498348179,50.480890008042));
#22455=CARTESIAN_POINT('Ctrl Pts',(31.5773149215154,30.2940840185436,50.5179332711152));
#22456=CARTESIAN_POINT('Ctrl Pts',(32.1271383127132,30.3360958238199,50.5549765341885));
#22457=CARTESIAN_POINT('Ctrl Pts',(32.6769617039109,30.3781076290962,50.5920197972617));
#22458=CARTESIAN_POINT('Ctrl Pts',(33.2039021190059,30.7195970559231,50.629063060335));
#22459=CARTESIAN_POINT('Ctrl Pts',(33.4668344812687,31.2043003942292,50.6661063234082));
#22460=CARTESIAN_POINT('Ctrl Pts',(33.5978491015855,31.4458196324391,50.6845643367355));
#22461=CARTESIAN_POINT('Ctrl Pts',(33.6633143382183,31.7228968149303,50.7030223500629));
#22462=CARTESIAN_POINT('Ctrl Pts',(33.6632910880953,31.9999843288606,50.7214803633902));
#22463=CARTESIAN_POINT('Ctrl Pts',(33.6656098327441,32.0015149950249,50.5285196366098));
#22464=CARTESIAN_POINT('Ctrl Pts',(33.6619313018869,31.5901995059569,50.5010237856321));
#22465=CARTESIAN_POINT('Ctrl Pts',(33.5079762466969,31.1764235703383,50.4735279346545));
#22466=CARTESIAN_POINT('Ctrl Pts',(33.2318651140294,30.874278170747,50.4460320836768));
#22467=CARTESIAN_POINT('Ctrl Pts',(32.8598796339962,30.467218519001,50.4089888206036));
#22468=CARTESIAN_POINT('Ctrl Pts',(32.2661770384583,30.2627717945958,50.3719455575303));
#22469=CARTESIAN_POINT('Ctrl Pts',(31.7224324159159,30.3544917100529,50.334902294457));
#22470=CARTESIAN_POINT('Ctrl Pts',(31.1786877933735,30.4462116255099,50.2978590313838));
#22471=CARTESIAN_POINT('Ctrl Pts',(30.6849011438266,30.8340981808292,50.2608157683105));
#22472=CARTESIAN_POINT('Ctrl Pts',(30.4670265606612,31.3406565915239,50.2237725052373));
#22473=CARTESIAN_POINT('Ctrl Pts',(30.2491519774957,31.8472150022187,50.1867292421641));
#22474=CARTESIAN_POINT('Ctrl Pts',(30.3071894607117,32.4724452682889,50.1496859790909));
#22475=CARTESIAN_POINT('Ctrl Pts',(30.6145813726846,32.9302454101508,50.1126427160176));
#22476=CARTESIAN_POINT('Ctrl Pts',(30.9219732846575,33.3880455520127,50.0755994529444));
#22477=CARTESIAN_POINT('Ctrl Pts',(31.4787196253875,33.6784155696663,50.0385561898711));
#22478=CARTESIAN_POINT('Ctrl Pts',(32.0300562881877,33.6684837174991,50.0015129267979));
#22479=CARTESIAN_POINT('Ctrl Pts',(32.5813929509879,33.6585518653319,49.9644696637246));
#22480=CARTESIAN_POINT('Ctrl Pts',(33.1273199358584,33.3483181433439,49.9274264006514));
#22481=CARTESIAN_POINT('Ctrl Pts',(33.4180240146883,32.8797438205446,49.8903831375781));
#22482=CARTESIAN_POINT('Ctrl Pts',(33.5798525593878,32.618898836713,49.8697619705887));
#22483=CARTESIAN_POINT('Ctrl Pts',(33.6625899967803,32.3089856338718,49.8491408035992));
#22484=CARTESIAN_POINT('Ctrl Pts',(33.6634354704477,31.999492392636,49.8285196366098));
#22485=CARTESIAN_POINT('Origin',(32.,32.,48.));
#22486=CARTESIAN_POINT('',(33.6674693445231,31.9987546512162,49.1285196366098));
#22487=CARTESIAN_POINT('',(33.6680840189634,32.0009409208067,49.3214803633902));
#22488=CARTESIAN_POINT('',(33.666,32.,48.));
#22489=CARTESIAN_POINT('Ctrl Pts',(33.6680840189634,32.0009409208067,49.3214803633902));
#22490=CARTESIAN_POINT('Ctrl Pts',(33.668455705338,32.0559214501504,49.3251698598506));
#22491=CARTESIAN_POINT('Ctrl Pts',(33.665972975259,32.1108680016515,49.3288593563111));
#22492=CARTESIAN_POINT('Ctrl Pts',(33.6605254320909,32.1655190244238,49.3325488527715));
#22493=CARTESIAN_POINT('Ctrl Pts',(33.6058310376544,32.7142259375462,49.3695921158448));
#22494=CARTESIAN_POINT('Ctrl Pts',(33.2522671445756,33.2331419261279,49.406635378918));
#22495=CARTESIAN_POINT('Ctrl Pts',(32.761622673207,33.4848138474987,49.4436786419912));
#22496=CARTESIAN_POINT('Ctrl Pts',(32.2709782018384,33.7364857688695,49.4807219050644));
#22497=CARTESIAN_POINT('Ctrl Pts',(31.6432531521799,33.7209136230295,49.5177651681377));
#22498=CARTESIAN_POINT('Ctrl Pts',(31.165691103258,33.4452231394785,49.5548084312109));
#22499=CARTESIAN_POINT('Ctrl Pts',(30.6881290543361,33.1695326559275,49.5918516942842));
#22500=CARTESIAN_POINT('Ctrl Pts',(30.3607300061507,32.6337238346656,49.6288949573574));
#22501=CARTESIAN_POINT('Ctrl Pts',(30.3333099879041,32.0829798869999,49.6659382204307));
#22502=CARTESIAN_POINT('Ctrl Pts',(30.3058899696574,31.5322359393341,49.7029814835039));
#22503=CARTESIAN_POINT('Ctrl Pts',(30.5784489813495,30.9665568652646,49.7400247465771));
#22504=CARTESIAN_POINT('Ctrl Pts',(31.0262654971198,30.6447943418184,49.7770680096504));
#22505=CARTESIAN_POINT('Ctrl Pts',(31.47408201289,30.3230318183722,49.8141112727237));
#22506=CARTESIAN_POINT('Ctrl Pts',(32.0971560327385,30.2451858455493,49.8511545357969));
#22507=CARTESIAN_POINT('Ctrl Pts',(32.6103722636605,30.4468783184113,49.8881977988701));
#22508=CARTESIAN_POINT('Ctrl Pts',(33.1235884945826,30.6485707912734,49.9252410619434));
#22509=CARTESIAN_POINT('Ctrl Pts',(33.5269469365783,31.1298017098203,49.9622843250166));
#22510=CARTESIAN_POINT('Ctrl Pts',(33.6358729537107,31.670362415091,49.9993275880898));
#22511=CARTESIAN_POINT('Ctrl Pts',(33.6575864258484,31.7781185795195,50.0067118465233));
#22512=CARTESIAN_POINT('Ctrl Pts',(33.6676000305986,31.8882323329164,50.0140961049567));
#22513=CARTESIAN_POINT('Ctrl Pts',(33.6665861757579,31.9985292434177,50.0214803633902));
#22514=CARTESIAN_POINT('Ctrl Pts',(33.6634354704477,31.999492392636,49.8285196366098));
#22515=CARTESIAN_POINT('Ctrl Pts',(33.6641087810226,31.7530210000391,49.812097540526));
#22516=CARTESIAN_POINT('Ctrl Pts',(33.6128456746512,31.5068159498285,49.7956754444422));
#22517=CARTESIAN_POINT('Ctrl Pts',(33.5082315407763,31.2858719194522,49.7792533483584));
#22518=CARTESIAN_POINT('Ctrl Pts',(33.2722538152451,30.7874892647698,49.7422100852852));
#22519=CARTESIAN_POINT('Ctrl Pts',(32.7648171913937,30.4176388790156,49.7051668222119));
#22520=CARTESIAN_POINT('Ctrl Pts',(32.2181219168358,30.3455622932806,49.6681235591387));
#22521=CARTESIAN_POINT('Ctrl Pts',(31.6714266422779,30.2734857075455,49.6310802960654));
#22522=CARTESIAN_POINT('Ctrl Pts',(31.0854727170135,30.4991829218297,49.5940370329922));
#22523=CARTESIAN_POINT('Ctrl Pts',(30.7283894800409,30.9193761146687,49.5569937699189));
#22524=CARTESIAN_POINT('Ctrl Pts',(30.3713062430682,31.3395693075078,49.5199505068457));
#22525=CARTESIAN_POINT('Ctrl Pts',(30.2430936943872,31.9542584789018,49.4829072437725));
#22526=CARTESIAN_POINT('Ctrl Pts',(30.4024212010707,32.482165197034,49.4458639806992));
#22527=CARTESIAN_POINT('Ctrl Pts',(30.5617487077542,33.0100719151663,49.408820717626));
#22528=CARTESIAN_POINT('Ctrl Pts',(31.0086162698022,33.4511961800368,49.3717774545528));
#22529=CARTESIAN_POINT('Ctrl Pts',(31.53853971386,33.6036819199376,49.3347341914795));
#22530=CARTESIAN_POINT('Ctrl Pts',(32.0684631579178,33.7561676598384,49.2976909284063));
#22531=CARTESIAN_POINT('Ctrl Pts',(32.6814424839853,33.6200148747694,49.260647665333));
#22532=CARTESIAN_POINT('Ctrl Pts',(33.0969816761962,33.2575263409205,49.2236044022598));
#22533=CARTESIAN_POINT('Ctrl Pts',(33.4525249287045,32.9473742427852,49.1919094803764));
#22534=CARTESIAN_POINT('Ctrl Pts',(33.6635254234559,32.4715253702981,49.1602145584931));
#22535=CARTESIAN_POINT('Ctrl Pts',(33.6674693445231,31.9987546512162,49.1285196366098));
#22536=CARTESIAN_POINT('Origin',(32.,32.,48.));
#22537=CARTESIAN_POINT('',(33.6673135177489,32.0013000734092,48.4285196366098));
#22538=CARTESIAN_POINT('',(33.6637467286262,32.0008713513863,48.6214803633902));
#22539=CARTESIAN_POINT('',(33.666,32.,48.));
#22540=CARTESIAN_POINT('Ctrl Pts',(33.6637467286262,32.0008713513863,48.6214803633902));
#22541=CARTESIAN_POINT('Ctrl Pts',(33.6647971283749,32.2223423012086,48.6362436147445));
#22542=CARTESIAN_POINT('Ctrl Pts',(33.623699448009,32.4434392475646,48.6510068660988));
#22543=CARTESIAN_POINT('Ctrl Pts',(33.5386160306917,32.6460665354014,48.6657701174531));
#22544=CARTESIAN_POINT('Ctrl Pts',(33.325128680567,33.154489493801,48.7028133805264));
#22545=CARTESIAN_POINT('Ctrl Pts',(32.8347136828381,33.5466302334562,48.7398566435996));
#22546=CARTESIAN_POINT('Ctrl Pts',(32.2917822813012,33.6430472781955,48.7768999066728));
#22547=CARTESIAN_POINT('Ctrl Pts',(31.7488508797643,33.7394643229347,48.8139431697461));
#22548=CARTESIAN_POINT('Ctrl Pts',(31.1534030744194,33.540157672758,48.8509864328194));
#22549=CARTESIAN_POINT('Ctrl Pts',(30.777912552311,33.1363289700909,48.8880296958926));
#22550=CARTESIAN_POINT('Ctrl Pts',(30.4024220302026,32.7325002674237,48.9250729589658));
#22551=CARTESIAN_POINT('Ctrl Pts',(30.2468887913307,32.1241495122662,48.962116222039));
#22552=CARTESIAN_POINT('Ctrl Pts',(30.3824840024592,31.5896547115336,48.9991594851123));
#22553=CARTESIAN_POINT('Ctrl Pts',(30.5180792135878,31.0551599108011,49.0362027481855));
#22554=CARTESIAN_POINT('Ctrl Pts',(30.9448028747168,30.5945210644937,49.0732460112588));
#22555=CARTESIAN_POINT('Ctrl Pts',(31.4673885523263,30.4185240109715,49.1102892743321));
#22556=CARTESIAN_POINT('Ctrl Pts',(31.9899742299358,30.2425269574493,49.1473325374053));
#22557=CARTESIAN_POINT('Ctrl Pts',(32.6084219240258,30.3511716967123,49.1843758004785));
#22558=CARTESIAN_POINT('Ctrl Pts',(33.0397333231737,30.6947429851753,49.2214190635517));
#22559=CARTESIAN_POINT('Ctrl Pts',(33.4280862529947,31.0040946896297,49.2547728301645));
#22560=CARTESIAN_POINT('Ctrl Pts',(33.6647239017427,31.503906226873,49.2881265967774));
#22561=CARTESIAN_POINT('Ctrl Pts',(33.6680840189634,32.0009409208067,49.3214803633902));
#22562=CARTESIAN_POINT('Ctrl Pts',(33.6674693445231,31.9987546512162,49.1285196366098));
#22563=CARTESIAN_POINT('Ctrl Pts',(33.6681348591936,31.9189772307336,49.1231712954199));
#22564=CARTESIAN_POINT('Ctrl Pts',(33.6629045043801,31.8392874596813,49.11782295423));
#22565=CARTESIAN_POINT('Ctrl Pts',(33.6514779047485,31.7604962919983,49.1124746130401));
#22566=CARTESIAN_POINT('Ctrl Pts',(33.572335882736,31.2147790595537,49.0754313499668));
#22567=CARTESIAN_POINT('Ctrl Pts',(33.1959527803567,30.7121688772935,49.0383880868935));
#22568=CARTESIAN_POINT('Ctrl Pts',(32.6945594644071,30.4826574393297,49.0013448238203));
#22569=CARTESIAN_POINT('Ctrl Pts',(32.1931661484575,30.2531460013658,48.9643015607471));
#22570=CARTESIAN_POINT('Ctrl Pts',(31.5667626189377,30.2967333076982,48.9272582976738));
#22571=CARTESIAN_POINT('Ctrl Pts',(31.1019877344241,30.5934740432916,48.8902150346006));
#22572=CARTESIAN_POINT('Ctrl Pts',(30.6372128499105,30.8902147788851,48.8531717715274));
#22573=CARTESIAN_POINT('Ctrl Pts',(30.3340666104031,31.4401089437394,48.8161285084541));
#22574=CARTESIAN_POINT('Ctrl Pts',(30.3312670913586,31.9915279496943,48.7790852453808));
#22575=CARTESIAN_POINT('Ctrl Pts',(30.3284675723141,32.5429469556492,48.7420419823076));
#22576=CARTESIAN_POINT('Ctrl Pts',(30.6260147737323,33.0958908027046,48.7049987192344));
#22577=CARTESIAN_POINT('Ctrl Pts',(31.0877527096269,33.3973353846611,48.6679554561611));
#22578=CARTESIAN_POINT('Ctrl Pts',(31.5494906455215,33.6987799666177,48.6309121930879));
#22579=CARTESIAN_POINT('Ctrl Pts',(32.1754193158924,33.7487252834754,48.5938689300147));
#22580=CARTESIAN_POINT('Ctrl Pts',(32.6791171551348,33.5243166290574,48.5568256669414));
#22581=CARTESIAN_POINT('Ctrl Pts',(33.1828149943771,33.2999079746393,48.5197824038682));
#22582=CARTESIAN_POINT('Ctrl Pts',(33.564282002491,32.8011453489455,48.4827391407949));
#22583=CARTESIAN_POINT('Ctrl Pts',(33.6489609449821,32.2562598250658,48.4456958777217));
#22584=CARTESIAN_POINT('Ctrl Pts',(33.6620489382515,32.1720422160678,48.4399704640177));
#22585=CARTESIAN_POINT('Ctrl Pts',(33.6680470054324,32.0867227839946,48.4342450503138));
#22586=CARTESIAN_POINT('Ctrl Pts',(33.6673135177489,32.0013000734092,48.4285196366098));
#22587=CARTESIAN_POINT('Origin',(32.,32.,48.));
#22588=CARTESIAN_POINT('',(33.6633884534296,32.0004190051222,47.7285196366098));
#22589=CARTESIAN_POINT('',(33.6649068449334,31.9985848581839,47.9214803633902));
#22590=CARTESIAN_POINT('',(33.666,32.,48.));
#22591=CARTESIAN_POINT('Ctrl Pts',(33.6649068449334,31.9985848581839,47.9214803633902));
#22592=CARTESIAN_POINT('Ctrl Pts',(33.6617821224527,32.3854996191865,47.9473173696384));
#22593=CARTESIAN_POINT('Ctrl Pts',(33.5274209634318,32.7743714298488,47.9731543758866));
#22594=CARTESIAN_POINT('Ctrl Pts',(33.2809047599811,33.0695906945765,47.9989913821348));
#22595=CARTESIAN_POINT('Ctrl Pts',(32.9274673497593,33.4928550922606,48.036034645208));
#22596=CARTESIAN_POINT('Ctrl Pts',(32.3434864284141,33.7236093190898,48.0730779082812));
#22597=CARTESIAN_POINT('Ctrl Pts',(31.7961884990483,33.6562614920799,48.1101211713545));
#22598=CARTESIAN_POINT('Ctrl Pts',(31.2488905696825,33.5889136650699,48.1471644344277));
#22599=CARTESIAN_POINT('Ctrl Pts',(30.7382756322961,33.2234637842209,48.184207697501));
#22600=CARTESIAN_POINT('Ctrl Pts',(30.4979983135429,32.7271397334397,48.2212509605743));
#22601=CARTESIAN_POINT('Ctrl Pts',(30.2577209947897,32.2308156826585,48.2582942236475));
#22602=CARTESIAN_POINT('Ctrl Pts',(30.2877812946696,31.6036174619452,48.2953374867207));
#22603=CARTESIAN_POINT('Ctrl Pts',(30.574423782953,31.1325475762575,48.3323807497939));
#22604=CARTESIAN_POINT('Ctrl Pts',(30.8610662712363,30.6614776905698,48.3694240128672));
#22605=CARTESIAN_POINT('Ctrl Pts',(31.4042909479229,30.3465361399077,48.4064672759405));
#22606=CARTESIAN_POINT('Ctrl Pts',(31.9555211464742,30.3318384701547,48.4435105390137));
#22607=CARTESIAN_POINT('Ctrl Pts',(32.5067513450255,30.3171408004017,48.4805538020869));
#22608=CARTESIAN_POINT('Ctrl Pts',(33.0659870654415,30.6026870115578,48.5175970651601));
#22609=CARTESIAN_POINT('Ctrl Pts',(33.3773250743892,31.0578127057078,48.5546403282334));
#22610=CARTESIAN_POINT('Ctrl Pts',(33.5645821870844,31.3315522458558,48.5769203399523));
#22611=CARTESIAN_POINT('Ctrl Pts',(33.6621615142211,31.6666377033218,48.5992003516713));
#22612=CARTESIAN_POINT('Ctrl Pts',(33.6637467286262,32.0008713513863,48.6214803633902));
#22613=CARTESIAN_POINT('Ctrl Pts',(33.6673135177489,32.0013000734092,48.4285196366098));
#22614=CARTESIAN_POINT('Ctrl Pts',(33.6633013610779,31.5340402872771,48.3972017872405));
#22615=CARTESIAN_POINT('Ctrl Pts',(33.4578771286557,31.0636903473883,48.3658839378712));
#22616=CARTESIAN_POINT('Ctrl Pts',(33.1096935602187,30.7536768081961,48.334566088502));
#22617=CARTESIAN_POINT('Ctrl Pts',(32.6978563560956,30.3869877372719,48.2975228254287));
#22618=CARTESIAN_POINT('Ctrl Pts',(32.086291070981,30.2446180174893,48.2604795623555));
#22619=CARTESIAN_POINT('Ctrl Pts',(31.5548466632686,30.3917152606531,48.2234362992822));
#22620=CARTESIAN_POINT('Ctrl Pts',(31.0234022555563,30.5388125038169,48.186393036209));
#22621=CARTESIAN_POINT('Ctrl Pts',(30.5720787252461,30.9753767099272,48.1493497731357));
#22622=CARTESIAN_POINT('Ctrl Pts',(30.4073992726082,31.5016384654387,48.1123065100625));
#22623=CARTESIAN_POINT('Ctrl Pts',(30.2427198199703,32.0279002209502,48.0752632469893));
#22624=CARTESIAN_POINT('Ctrl Pts',(30.3646844450046,32.6438595258629,48.038219983916));
#22625=CARTESIAN_POINT('Ctrl Pts',(30.717482796621,33.067656742149,48.0011767208428));
#22626=CARTESIAN_POINT('Ctrl Pts',(31.0702811482375,33.4914539584351,47.9641334577695));
#22627=CARTESIAN_POINT('Ctrl Pts',(31.6539132264361,33.7230890860946,47.9270901946963));
#22628=CARTESIAN_POINT('Ctrl Pts',(32.2013121568464,33.6565671466998,47.890046931623));
#22629=CARTESIAN_POINT('Ctrl Pts',(32.7487110872566,33.5900452073049,47.8530036685498));
#22630=CARTESIAN_POINT('Ctrl Pts',(33.2598768698785,33.2253662008556,47.8159604054766));
#22631=CARTESIAN_POINT('Ctrl Pts',(33.5009028142653,32.7294052633136,47.7789171424033));
#22632=CARTESIAN_POINT('Ctrl Pts',(33.610208397529,32.5044863248485,47.7621179738055));
#22633=CARTESIAN_POINT('Ctrl Pts',(33.663956091105,32.2525674922054,47.7453188052076));
#22634=CARTESIAN_POINT('Ctrl Pts',(33.6633884534296,32.0004190051222,47.7285196366098));
#22635=CARTESIAN_POINT('Origin',(32.,32.,48.));
#22636=CARTESIAN_POINT('',(33.66577763495,31.9984781750094,47.0285196366098));
#22637=CARTESIAN_POINT('',(33.668753764066,31.9999631497191,47.2214803633902));
#22638=CARTESIAN_POINT('',(33.666,32.,48.));
#22639=CARTESIAN_POINT('Ctrl Pts',(33.6687533715572,31.9999631549716,47.2214803633902));
#22640=CARTESIAN_POINT('Ctrl Pts',(33.668574581605,32.5494177579999,47.2583911245323));
#22641=CARTESIAN_POINT('Ctrl Pts',(33.3706768371093,33.0990384969375,47.2953018856743));
#22642=CARTESIAN_POINT('Ctrl Pts',(32.9101378227849,33.3987102636369,47.3322126468164));
#22643=CARTESIAN_POINT('Ctrl Pts',(32.4479455694893,33.6994577894531,47.3692559098897));
#22644=CARTESIAN_POINT('Ctrl Pts',(31.8219422540236,33.7484585927198,47.4062991729629));
#22645=CARTESIAN_POINT('Ctrl Pts',(31.3185835991834,33.5232901715579,47.4433424360361));
#22646=CARTESIAN_POINT('Ctrl Pts',(30.8152249443432,33.2981217503961,47.4803856991094));
#22647=CARTESIAN_POINT('Ctrl Pts',(30.4345109501285,32.7987841048057,47.5174289621826));
#22648=CARTESIAN_POINT('Ctrl Pts',(30.3506542759561,32.2537714338632,47.5544722252559));
#22649=CARTESIAN_POINT('Ctrl Pts',(30.2667976017838,31.7087587629208,47.5915154883291));
#22650=CARTESIAN_POINT('Ctrl Pts',(30.4797982476539,31.1180710666263,47.6285587514024));
#22651=CARTESIAN_POINT('Ctrl Pts',(30.8921882729642,30.7520038319335,47.6656020144756));
#22652=CARTESIAN_POINT('Ctrl Pts',(31.3045782982745,30.3859365972407,47.7026452775488));
#22653=CARTESIAN_POINT('Ctrl Pts',(31.916357703025,30.2444898241495,47.7396885406221));
#22654=CARTESIAN_POINT('Ctrl Pts',(32.4475795488375,30.3923887890633,47.7767318036953));
#22655=CARTESIAN_POINT('Ctrl Pts',(32.9788013946501,30.5402877539772,47.8137750667686));
#22656=CARTESIAN_POINT('Ctrl Pts',(33.4294656815247,30.977532456896,47.8508183298418));
#22657=CARTESIAN_POINT('Ctrl Pts',(33.5933508754128,31.5040420926248,47.887861592915));
#22658=CARTESIAN_POINT('Ctrl Pts',(33.6429291096225,31.6633207767725,47.8990678497401));
#22659=CARTESIAN_POINT('Ctrl Pts',(33.6662621274414,31.8307687366275,47.9102741065651));
#22660=CARTESIAN_POINT('Ctrl Pts',(33.6649068449334,31.9985848581839,47.9214803633902));
#22661=CARTESIAN_POINT('Ctrl Pts',(33.6633884534296,32.0004190051222,47.7285196366098));
#22662=CARTESIAN_POINT('Ctrl Pts',(33.6627044129868,31.696563622958,47.7082755421344));
#22663=CARTESIAN_POINT('Ctrl Pts',(33.583144610912,31.3923747406851,47.688031447659));
#22664=CARTESIAN_POINT('Ctrl Pts',(33.4268834926819,31.1346995930135,47.6677873531836));
#22665=CARTESIAN_POINT('Ctrl Pts',(33.14095212056,30.6631977288903,47.6307440901104));
#22666=CARTESIAN_POINT('Ctrl Pts',(32.5982032701644,30.3474368692789,47.5937008270371));
#22667=CARTESIAN_POINT('Ctrl Pts',(32.0469958725032,30.3319074713953,47.5566575639639));
#22668=CARTESIAN_POINT('Ctrl Pts',(31.4957884748419,30.3163780735117,47.5196143008907));
#22669=CARTESIAN_POINT('Ctrl Pts',(30.9361225299148,30.6010801373561,47.4825710378174));
#22670=CARTESIAN_POINT('Ctrl Pts',(30.6240981394585,31.0557355422459,47.4455277747441));
#22671=CARTESIAN_POINT('Ctrl Pts',(30.3120737490021,31.5103909471357,47.4084845116709));
#22672=CARTESIAN_POINT('Ctrl Pts',(30.2476909130165,32.1349996930709,47.3714412485977));
#22673=CARTESIAN_POINT('Ctrl Pts',(30.4604108681471,32.6437442047115,47.3343979855245));
#22674=CARTESIAN_POINT('Ctrl Pts',(30.6731308232777,33.152488716352,47.2973547224512));
#22675=CARTESIAN_POINT('Ctrl Pts',(31.1629535695247,33.5453689936979,47.2603114593779));
#22676=CARTESIAN_POINT('Ctrl Pts',(31.7057388741586,33.6426051521403,47.2232681963047));
#22677=CARTESIAN_POINT('Ctrl Pts',(32.2485241787925,33.7398413105826,47.1862249332314));
#22678=CARTESIAN_POINT('Ctrl Pts',(32.8442720418133,33.5414333501214,47.1491816701582));
#22679=CARTESIAN_POINT('Ctrl Pts',(33.2203714714111,33.1381716776414,47.112138407085));
#22680=CARTESIAN_POINT('Ctrl Pts',(33.5033646463302,32.8347404782366,47.0842654835932));
#22681=CARTESIAN_POINT('Ctrl Pts',(33.6619995478179,32.4153273274213,47.0563925601015));
#22682=CARTESIAN_POINT('Ctrl Pts',(33.66577763495,31.9984781750094,47.0285196366098));
#22683=CARTESIAN_POINT('Origin',(32.,32.,48.));
#22684=CARTESIAN_POINT('',(33.6685588008505,32.0005167954687,46.3285196366098));
#22685=CARTESIAN_POINT('',(33.6650142123929,32.0014384754572,46.5214803633902));
#22686=CARTESIAN_POINT('',(33.666,32.,48.));
#22687=CARTESIAN_POINT('Ctrl Pts',(33.6650142123929,32.0014384754572,46.5214803633902));
#22688=CARTESIAN_POINT('Ctrl Pts',(33.6663656089876,32.1652593743191,46.5324216163529));
#22689=CARTESIAN_POINT('Ctrl Pts',(33.6441442932285,32.3287216649132,46.5433628693156));
#22690=CARTESIAN_POINT('Ctrl Pts',(33.5968494360195,32.4845752126874,46.5543041222783));
#22691=CARTESIAN_POINT('Ctrl Pts',(33.4367255595701,33.0122409188706,46.5913473853516));
#22692=CARTESIAN_POINT('Ctrl Pts',(32.9891929020642,33.4526904053733,46.6283906484248));
#22693=CARTESIAN_POINT('Ctrl Pts',(32.4590399809318,33.6043763754097,46.665433911498));
#22694=CARTESIAN_POINT('Ctrl Pts',(31.9288870597995,33.7560623454462,46.7024771745713));
#22695=CARTESIAN_POINT('Ctrl Pts',(31.3161138750406,33.6189847990163,46.7395204376445));
#22696=CARTESIAN_POINT('Ctrl Pts',(30.9011221133767,33.2558696780945,46.7765637007178));
#22697=CARTESIAN_POINT('Ctrl Pts',(30.4861303517127,32.8927545571726,46.813606963791));
#22698=CARTESIAN_POINT('Ctrl Pts',(30.2689200131437,32.3036018617586,46.8506502268643));
#22699=CARTESIAN_POINT('Ctrl Pts',(30.3488853708247,31.7580046707266,46.8876934899375));
#22700=CARTESIAN_POINT('Ctrl Pts',(30.4288507285058,31.2124074796946,46.9247367530107));
#22701=CARTESIAN_POINT('Ctrl Pts',(30.8059917824369,30.7103657930446,46.961780016084));
#22702=CARTESIAN_POINT('Ctrl Pts',(31.3077308313014,30.4816111643798,46.9988232791572));
#22703=CARTESIAN_POINT('Ctrl Pts',(31.809469880166,30.252856535715,47.0358665422305));
#22704=CARTESIAN_POINT('Ctrl Pts',(32.4358069239639,30.2973889650355,47.0729098053037));
#22705=CARTESIAN_POINT('Ctrl Pts',(32.9001335276246,30.5948306541513,47.109953068377));
#22706=CARTESIAN_POINT('Ctrl Pts',(33.3644601312852,30.892272343267,47.1469963314502));
#22707=CARTESIAN_POINT('Ctrl Pts',(33.6667762948085,31.4426232921781,47.1840395945234));
#22708=CARTESIAN_POINT('Ctrl Pts',(33.6687437810073,31.9940458908165,47.2210828575967));
#22709=CARTESIAN_POINT('Ctrl Pts',(33.6687508186088,31.996018302347,47.2212153595278));
#22710=CARTESIAN_POINT('Ctrl Pts',(33.6687540133758,31.9979907275889,47.221347861459));
#22711=CARTESIAN_POINT('Ctrl Pts',(33.6687533715572,31.9999631549716,47.2214803633902));
#22712=CARTESIAN_POINT('Ctrl Pts',(33.66577763495,31.9984781750094,47.0285196366098));
#22713=CARTESIAN_POINT('Ctrl Pts',(33.6670206456439,31.8613325941729,47.0193492970283));
#22714=CARTESIAN_POINT('Ctrl Pts',(33.6515012597471,31.724464552031,47.0101789574468));
#22715=CARTESIAN_POINT('Ctrl Pts',(33.6181333324057,31.592095826723,47.0010086178653));
#22716=CARTESIAN_POINT('Ctrl Pts',(33.4833447676279,31.0573970327836,46.963965354792));
#22717=CARTESIAN_POINT('Ctrl Pts',(33.0573166418977,30.5961148294036,46.9269220917188));
#22718=CARTESIAN_POINT('Ctrl Pts',(32.5349971155079,30.4193294516512,46.8898788286455));
#22719=CARTESIAN_POINT('Ctrl Pts',(32.0126775891181,30.2425440738987,46.8528355655723));
#22720=CARTESIAN_POINT('Ctrl Pts',(31.3940666620687,30.3502555217738,46.815792302499));
#22721=CARTESIAN_POINT('Ctrl Pts',(30.9622373402994,30.6931756207699,46.7787490394258));
#22722=CARTESIAN_POINT('Ctrl Pts',(30.5304080185301,31.0360957197659,46.7417057763526));
#22723=CARTESIAN_POINT('Ctrl Pts',(30.2853603020409,31.6142244698828,46.7046625132793));
#22724=CARTESIAN_POINT('Ctrl Pts',(30.3392266971815,32.1630132898397,46.6676192502061));
#22725=CARTESIAN_POINT('Ctrl Pts',(30.393093092322,32.7118021097967,46.6305759871328));
#22726=CARTESIAN_POINT('Ctrl Pts',(30.7458735990921,33.2312509995936,46.5935327240596));
#22727=CARTESIAN_POINT('Ctrl Pts',(31.2361377704666,33.4836629638538,46.5564894609863));
#22728=CARTESIAN_POINT('Ctrl Pts',(31.726401941841,33.736074928114,46.5194461979131));
#22729=CARTESIAN_POINT('Ctrl Pts',(32.3541497778197,33.7214499668374,46.4824029348399));
#22730=CARTESIAN_POINT('Ctrl Pts',(32.8321272724797,33.4464803830037,46.4453596717666));
#22731=CARTESIAN_POINT('Ctrl Pts',(33.3101047671398,33.17151079917,46.4083164086934));
#22732=CARTESIAN_POINT('Ctrl Pts',(33.6383119204811,32.6361965927792,46.3712731456201));
#22733=CARTESIAN_POINT('Ctrl Pts',(33.6665629187639,32.0854946420552,46.3342298825469));
#22734=CARTESIAN_POINT('Ctrl Pts',(33.6680145560729,32.0571976066811,46.3323264672345));
#22735=CARTESIAN_POINT('Ctrl Pts',(33.6686742275888,32.0288599434787,46.3304230519221));
#22736=CARTESIAN_POINT('Ctrl Pts',(33.6685588008505,32.0005167954687,46.3285196366098));
#22737=CARTESIAN_POINT('Origin',(32.,32.,48.));
#22738=CARTESIAN_POINT('',(33.664255890244,32.0011936369589,45.6285196366098));
#22739=CARTESIAN_POINT('',(33.6636859641007,31.9991832784139,45.8214803633902));
#22740=CARTESIAN_POINT('',(33.666,32.,48.));
#22741=CARTESIAN_POINT('Ctrl Pts',(33.6636859641007,31.9991832784139,45.8214803633902));
#22742=CARTESIAN_POINT('Ctrl Pts',(33.6622209772371,32.3294716616209,45.8434953712468));
#22743=CARTESIAN_POINT('Ctrl Pts',(33.5671083678426,32.660537694823,45.8655103791034));
#22744=CARTESIAN_POINT('Ctrl Pts',(33.3840134044156,32.932334786686,45.88752538696));
#22745=CARTESIAN_POINT('Ctrl Pts',(33.0759310752249,33.3896705842477,45.9245686500332));
#22746=CARTESIAN_POINT('Ctrl Pts',(32.5187472361758,33.6792002013809,45.9616119131064));
#22747=CARTESIAN_POINT('Ctrl Pts',(31.9674261908138,33.6684364551945,45.9986551761797));
#22748=CARTESIAN_POINT('Ctrl Pts',(31.4161051454517,33.657672709008,46.0356984392529));
#22749=CARTESIAN_POINT('Ctrl Pts',(30.8706468937767,33.3466155995018,46.0727417023262));
#22750=CARTESIAN_POINT('Ctrl Pts',(30.5806501741309,32.877603173349,46.1097849653994));
#22751=CARTESIAN_POINT('Ctrl Pts',(30.2906534544851,32.4085907471962,46.1468282284727));
#22752=CARTESIAN_POINT('Ctrl Pts',(30.2561182668687,31.7816230043967,46.1838714915459));
#22753=CARTESIAN_POINT('Ctrl Pts',(30.4928477258755,31.2835969844646,46.2209147546191));
#22754=CARTESIAN_POINT('Ctrl Pts',(30.7295771848824,30.7855709645325,46.2579580176924));
#22755=CARTESIAN_POINT('Ctrl Pts',(31.2375712905126,30.4164866674678,46.2950012807656));
#22756=CARTESIAN_POINT('Ctrl Pts',(31.784374694513,30.345235066331,46.3320445438389));
#22757=CARTESIAN_POINT('Ctrl Pts',(32.3311780985135,30.2739834651943,46.3690878069121));
#22758=CARTESIAN_POINT('Ctrl Pts',(32.9167908008843,30.5005645599854,46.4061310699854));
#22759=CARTESIAN_POINT('Ctrl Pts',(33.2732396043732,30.9212960703129,46.4431743330586));
#22760=CARTESIAN_POINT('Ctrl Pts',(33.5244061998796,31.2177585637675,46.4692763431691));
#22761=CARTESIAN_POINT('Ctrl Pts',(33.6617902518739,31.6106189986581,46.4953783532797));
#22762=CARTESIAN_POINT('Ctrl Pts',(33.6650142123929,32.0014384754572,46.5214803633902));
#22763=CARTESIAN_POINT('Ctrl Pts',(33.6685588008505,32.0005167954687,46.3285196366098));
#22764=CARTESIAN_POINT('Ctrl Pts',(33.666427853399,31.4772605730014,46.2933797888489));
#22765=CARTESIAN_POINT('Ctrl Pts',(33.4001233193856,30.9521349858584,46.258239941088));
#22766=CARTESIAN_POINT('Ctrl Pts',(32.9757782549176,30.6462651318486,46.2231000933272));
#22767=CARTESIAN_POINT('Ctrl Pts',(32.5284477495642,30.3238272674229,46.1860568302539));
#22768=CARTESIAN_POINT('Ctrl Pts',(31.9054918956329,30.2450412336288,46.1490135671807));
#22769=CARTESIAN_POINT('Ctrl Pts',(31.3919719140453,30.4459590923308,46.1119703041074));
#22770=CARTESIAN_POINT('Ctrl Pts',(30.8784519324577,30.6468769510328,46.0749270410342));
#22771=CARTESIAN_POINT('Ctrl Pts',(30.4743678232137,31.127498702231,46.037883777961));
#22772=CARTESIAN_POINT('Ctrl Pts',(30.3646262836486,31.66789443864,46.0008405148877));
#22773=CARTESIAN_POINT('Ctrl Pts',(30.2548847440835,32.208290175049,45.9637972518145));
#22774=CARTESIAN_POINT('Ctrl Pts',(30.4394857741973,32.8084598966689,45.9267539887412));
#22775=CARTESIAN_POINT('Ctrl Pts',(30.8339569435673,33.1937691931711,45.889710725668));
#22776=CARTESIAN_POINT('Ctrl Pts',(31.2284281129373,33.5790784896733,45.8526674625947));
#22777=CARTESIAN_POINT('Ctrl Pts',(31.8327694215635,33.7495273610579,45.8156241995215));
#22778=CARTESIAN_POINT('Ctrl Pts',(32.3704375635228,33.6271193279998,45.7785809364483));
#22779=CARTESIAN_POINT('Ctrl Pts',(32.9081057054821,33.5047112949417,45.741537673375));
#22780=CARTESIAN_POINT('Ctrl Pts',(33.3791006807746,33.0894463574409,45.7044944103018));
#22781=CARTESIAN_POINT('Ctrl Pts',(33.5678977425703,32.5713474992175,45.6674511472285));
#22782=CARTESIAN_POINT('Ctrl Pts',(33.6340380175379,32.3898446695792,45.6544739770223));
#22783=CARTESIAN_POINT('Ctrl Pts',(33.665544876609,32.1957213003327,45.641496806816));
#22784=CARTESIAN_POINT('Ctrl Pts',(33.664255890244,32.0011936369589,45.6285196366098));
#22785=CARTESIAN_POINT('Origin',(32.,32.,48.));
#22786=CARTESIAN_POINT('',(33.6642508883749,31.9988087175676,44.9285196366098));
#22787=CARTESIAN_POINT('',(33.6679951520813,31.9990039461198,45.1214803633902));
#22788=CARTESIAN_POINT('',(33.666,32.,48.));
#22789=CARTESIAN_POINT('Ctrl Pts',(33.6679951520813,31.9990039461198,45.1214803633902));
#22790=CARTESIAN_POINT('Ctrl Pts',(33.6645084345824,32.4921586880507,45.1545691261406));
#22791=CARTESIAN_POINT('Ctrl Pts',(33.4320886779645,32.9881690369999,45.1876578888911));
#22792=CARTESIAN_POINT('Ctrl Pts',(33.0490210948825,33.2978042997919,45.2207466516416));
#22793=CARTESIAN_POINT('Ctrl Pts',(32.6201723838579,33.6444446556993,45.2577899147148));
#22794=CARTESIAN_POINT('Ctrl Pts',(32.002515719258,33.7574998385532,45.2948331777881));
#22795=CARTESIAN_POINT('Ctrl Pts',(31.4786874417,33.5852364096959,45.3318764408613));
#22796=CARTESIAN_POINT('Ctrl Pts',(30.954859164142,33.4129729808386,45.3689197039346));
#22797=CARTESIAN_POINT('Ctrl Pts',(30.5248592736258,32.9553909402701,45.4059629670078));
#22798=CARTESIAN_POINT('Ctrl Pts',(30.3854533884744,32.4218773486192,45.4430062300811));
#22799=CARTESIAN_POINT('Ctrl Pts',(30.246047503323,31.8883637569683,45.4800494931543));
#22800=CARTESIAN_POINT('Ctrl Pts',(30.3972356235363,31.2789186142351,45.5170927562275));
#22801=CARTESIAN_POINT('Ctrl Pts',(30.7698348850881,30.8724207131555,45.5541360193008));
#22802=CARTESIAN_POINT('Ctrl Pts',(31.14243414664,30.465922812076,45.591179282374));
#22803=CARTESIAN_POINT('Ctrl Pts',(31.7364445495304,30.2623721526502,45.6282225454473));
#22804=CARTESIAN_POINT('Ctrl Pts',(32.280050154284,30.3549124129238,45.6652658085205));
#22805=CARTESIAN_POINT('Ctrl Pts',(32.8236557590377,30.4474526731974,45.7023090715938));
#22806=CARTESIAN_POINT('Ctrl Pts',(33.3168565656545,30.8360838531705,45.739352334667));
#22807=CARTESIAN_POINT('Ctrl Pts',(33.5339665592967,31.3429704321522,45.7763955977402));
#22808=CARTESIAN_POINT('Ctrl Pts',(33.6220469313765,31.5486116268756,45.7914238529569));
#22809=CARTESIAN_POINT('Ctrl Pts',(33.664686018092,31.7737162629005,45.8064521081735));
#22810=CARTESIAN_POINT('Ctrl Pts',(33.6636859641007,31.9991832784139,45.8214803633902));
#22811=CARTESIAN_POINT('Ctrl Pts',(33.664255890244,32.0011936369589,45.6285196366098));
#22812=CARTESIAN_POINT('Ctrl Pts',(33.6618654719116,31.640443123746,45.6044535437428));
#22813=CARTESIAN_POINT('Ctrl Pts',(33.5466852070223,31.2783021822037,45.5803874508758));
#22814=CARTESIAN_POINT('Ctrl Pts',(33.3304349107605,30.9926846351569,45.5563213580088));
#22815=CARTESIAN_POINT('Ctrl Pts',(32.997575868856,30.553053408266,45.5192780949356));
#22816=CARTESIAN_POINT('Ctrl Pts',(32.4252586367481,30.2947237334304,45.4822348318623));
#22817=CARTESIAN_POINT('Ctrl Pts',(31.8753724765885,30.3359058691205,45.4451915687891));
#22818=CARTESIAN_POINT('Ctrl Pts',(31.3254863164288,30.3770880048106,45.4081483057158));
#22819=CARTESIAN_POINT('Ctrl Pts',(30.7980312282173,30.7177819510265,45.3711050426426));
#22820=CARTESIAN_POINT('Ctrl Pts',(30.5343678003135,31.2020880053156,45.3340617795693));
#22821=CARTESIAN_POINT('Ctrl Pts',(30.2707043724096,31.6863940596048,45.2970185164961));
#22822=CARTESIAN_POINT('Ctrl Pts',(30.2708326048134,32.3143122219674,45.2599752534229));
#22823=CARTESIAN_POINT('Ctrl Pts',(30.5346938190722,32.7985105460506,45.2229319903496));
#22824=CARTESIAN_POINT('Ctrl Pts',(30.798555033331,33.2827088701339,45.1858887272764));
#22825=CARTESIAN_POINT('Ctrl Pts',(31.3261492294448,33.6231873559379,45.1488454642032));
#22826=CARTESIAN_POINT('Ctrl Pts',(31.8760521640323,33.6641448945264,45.1118022011299));
#22827=CARTESIAN_POINT('Ctrl Pts',(32.4259550986198,33.7051024331148,45.0747589380567));
#22828=CARTESIAN_POINT('Ctrl Pts',(32.9981667716809,33.4465390244878,45.0377156749834));
#22829=CARTESIAN_POINT('Ctrl Pts',(33.3308462243117,33.0067718824314,45.0006724119102));
#22830=CARTESIAN_POINT('Ctrl Pts',(33.5468436266396,32.7212461020977,44.97662148681));
#22831=CARTESIAN_POINT('Ctrl Pts',(33.6618671500066,32.3593345903844,44.9525705617099));
#22832=CARTESIAN_POINT('Ctrl Pts',(33.6642508883749,31.9988087175676,44.9285196366098));
#22833=CARTESIAN_POINT('Origin',(32.,32.,48.));
#22834=CARTESIAN_POINT('',(33.6685558202892,31.9994792812332,44.2285196366098));
#22835=CARTESIAN_POINT('',(33.6667054848825,32.0014513625929,44.4214803633902));
#22836=CARTESIAN_POINT('',(33.666,32.,48.));
#22837=CARTESIAN_POINT('Ctrl Pts',(33.6667054848825,32.0014513625929,44.4214803633902));
#22838=CARTESIAN_POINT('Ctrl Pts',(33.6676777367435,32.1077703681721,44.4285996179613));
#22839=CARTESIAN_POINT('Ctrl Pts',(33.6583759250957,32.2139199029793,44.4357188725324));
#22840=CARTESIAN_POINT('Ctrl Pts',(33.6381835786891,32.3179556896481,44.4428381271035));
#22841=CARTESIAN_POINT('Ctrl Pts',(33.5331177473534,32.8592799218571,44.4798813901767));
#22842=CARTESIAN_POINT('Ctrl Pts',(33.133203613556,33.3433769320565,44.51692465325));
#22843=CARTESIAN_POINT('Ctrl Pts',(32.6214397164782,33.5487265532852,44.5539679163233));
#22844=CARTESIAN_POINT('Ctrl Pts',(32.1096758194004,33.7540761745139,44.5910111793965));
#22845=CARTESIAN_POINT('Ctrl Pts',(31.4860621590421,33.6806784067719,44.6280544424697));
#22846=CARTESIAN_POINT('Ctrl Pts',(31.0359609649793,33.3621196705955,44.665097705543));
#22847=CARTESIAN_POINT('Ctrl Pts',(30.5858597709165,33.043560934419,44.7021409686162));
#22848=CARTESIAN_POINT('Ctrl Pts',(30.3092710431491,32.4798412298081,44.7391842316895));
#22849=CARTESIAN_POINT('Ctrl Pts',(30.3327602837635,31.9289156369497,44.7762274947627));
#22850=CARTESIAN_POINT('Ctrl Pts',(30.3562495243778,31.3779900440912,44.813270757836));
#22851=CARTESIAN_POINT('Ctrl Pts',(30.679816733374,30.8398585629853,44.8503140209092));
#22852=CARTESIAN_POINT('Ctrl Pts',(31.1553993103854,30.5607672414896,44.8873572839824));
#22853=CARTESIAN_POINT('Ctrl Pts',(31.6309818873969,30.2816759199939,44.9244005470557));
#22854=CARTESIAN_POINT('Ctrl Pts',(32.2585798324236,30.2616247581084,44.9614438101289));
#22855=CARTESIAN_POINT('Ctrl Pts',(32.7510077288296,30.509789058789,44.9984870732022));
#22856=CARTESIAN_POINT('Ctrl Pts',(33.2434356252356,30.7579533594696,45.0355303362754));
#22857=CARTESIAN_POINT('Ctrl Pts',(33.6006934730207,31.2743331227162,45.0725735993486));
#22858=CARTESIAN_POINT('Ctrl Pts',(33.6593020181886,31.8226357688199,45.1096168624218));
#22859=CARTESIAN_POINT('Ctrl Pts',(33.6655586892147,31.8811690299613,45.1135713627446));
#22860=CARTESIAN_POINT('Ctrl Pts',(33.668411856253,31.9400660945945,45.1175258630674));
#22861=CARTESIAN_POINT('Ctrl Pts',(33.6679951520813,31.9990039461198,45.1214803633902));
#22862=CARTESIAN_POINT('Ctrl Pts',(33.6642508883749,31.9988087175676,44.9285196366098));
#22863=CARTESIAN_POINT('Ctrl Pts',(33.6655385866398,31.8040522178409,44.9155272986367));
#22864=CARTESIAN_POINT('Ctrl Pts',(33.6339560460374,31.6097000715273,44.9025349606635));
#22865=CARTESIAN_POINT('Ctrl Pts',(33.5676642525274,31.4280121615218,44.8895426226904));
#22866=CARTESIAN_POINT('Ctrl Pts',(33.3786555959121,30.9099904581544,44.8524993596172));
#22867=CARTESIAN_POINT('Ctrl Pts',(32.9074910504814,30.4949179269053,44.815456096544));
#22868=CARTESIAN_POINT('Ctrl Pts',(32.3697729574409,30.3727295074374,44.7784128334707));
#22869=CARTESIAN_POINT('Ctrl Pts',(31.8320548644005,30.2505410879696,44.7413695703975));
#22870=CARTESIAN_POINT('Ctrl Pts',(31.2277832237503,30.4212367802829,44.7043263073242));
#22871=CARTESIAN_POINT('Ctrl Pts',(30.8334694617253,30.806707161133,44.667283044251));
#22872=CARTESIAN_POINT('Ctrl Pts',(30.4391556997004,31.1921775419831,44.6302397811777));
#22873=CARTESIAN_POINT('Ctrl Pts',(30.2547998163006,31.79242261137,44.5931965181045));
#22874=CARTESIAN_POINT('Ctrl Pts',(30.3647620641418,32.332773480237,44.5561532550313));
#22875=CARTESIAN_POINT('Ctrl Pts',(30.4747243119829,32.873124349104,44.519109991958));
#22876=CARTESIAN_POINT('Ctrl Pts',(30.8790046910649,33.353581017451,44.4820667288848));
#22877=CARTESIAN_POINT('Ctrl Pts',(31.3926066920388,33.5542891190076,44.4450234658115));
#22878=CARTESIAN_POINT('Ctrl Pts',(31.9062086930126,33.7549972205642,44.4079802027383));
#22879=CARTESIAN_POINT('Ctrl Pts',(32.5291323158784,33.6759567553303,44.370936939665));
#22880=CARTESIAN_POINT('Ctrl Pts',(32.9763310884756,33.3533362116233,44.3338936765918));
#22881=CARTESIAN_POINT('Ctrl Pts',(33.4003680786871,33.0474251655366,44.2987689965978));
#22882=CARTESIAN_POINT('Ctrl Pts',(33.6664114806385,32.5225121367035,44.2636443166038));
#22883=CARTESIAN_POINT('Ctrl Pts',(33.6685558202892,31.9994792812332,44.2285196366098));
#22884=CARTESIAN_POINT('Origin',(32.,32.,48.));
#22885=CARTESIAN_POINT('',(33.6657844257744,32.0015219728729,43.5285196366098));
#22886=CARTESIAN_POINT('',(33.6632945194008,32.000080914311,43.7214803633902));
#22887=CARTESIAN_POINT('',(33.666,32.,48.));
#22888=CARTESIAN_POINT('Ctrl Pts',(33.6632945194008,32.000080914311,43.7214803633902));
#22889=CARTESIAN_POINT('Ctrl Pts',(33.663412856101,32.273188844988,43.7396733728552));
#22890=CARTESIAN_POINT('Ctrl Pts',(33.5999068196939,32.5462449457584,43.7578663823202));
#22891=CARTESIAN_POINT('Ctrl Pts',(33.472475203927,32.7852120935461,43.7760593917852));
#22892=CARTESIAN_POINT('Ctrl Pts',(33.2130083534433,33.2717793620567,43.8131026548584));
#22893=CARTESIAN_POINT('Ctrl Pts',(32.6885182052593,33.6170203129166,43.8501459179316));
#22894=CARTESIAN_POINT('Ctrl Pts',(32.1390086072293,33.6629545589702,43.8871891810049));
#22895=CARTESIAN_POINT('Ctrl Pts',(31.5894990091993,33.7088888050238,43.9242324440781));
#22896=CARTESIAN_POINT('Ctrl Pts',(31.0149699613232,33.4555163462711,43.9612757071514));
#22897=CARTESIAN_POINT('Ctrl Pts',(30.678322840668,33.0187790459991,43.9983189702246));
#22898=CARTESIAN_POINT('Ctrl Pts',(30.3416757200127,32.5820417457271,44.0353622332979));
#22899=CARTESIAN_POINT('Ctrl Pts',(30.2429105265783,31.961939603936,44.0724054963711));
#22900=CARTESIAN_POINT('Ctrl Pts',(30.4272216773419,31.4422279983368,44.1094487594443));
#22901=CARTESIAN_POINT('Ctrl Pts',(30.6115328281055,30.9225163927377,44.1464920225176));
#22902=CARTESIAN_POINT('Ctrl Pts',(31.078920323067,30.5031953233307,44.1835352855908));
#22903=CARTESIAN_POINT('Ctrl Pts',(31.6155101788386,30.3761438378069,44.220578548664));
#22904=CARTESIAN_POINT('Ctrl Pts',(32.1521000346101,30.2490923522831,44.2576218117373));
#22905=CARTESIAN_POINT('Ctrl Pts',(32.7578922511917,30.4143104506425,44.2946650748106));
#22906=CARTESIAN_POINT('Ctrl Pts',(33.1556795950453,30.7961952269315,44.3317083378838));
#22907=CARTESIAN_POINT('Ctrl Pts',(33.4770171574514,31.1046864975282,44.3616323463859));
#22908=CARTESIAN_POINT('Ctrl Pts',(33.662618867012,31.5545659766137,44.3915563548881));
#22909=CARTESIAN_POINT('Ctrl Pts',(33.6667054848825,32.0014513625929,44.4214803633902));
#22910=CARTESIAN_POINT('Ctrl Pts',(33.6685558202892,31.9994792812332,44.2285196366098));
#22911=CARTESIAN_POINT('Ctrl Pts',(33.6686729485811,31.9709101387794,44.2266010535306));
#22912=CARTESIAN_POINT('Ctrl Pts',(33.6680027151203,31.9423466059576,44.2246824704513));
#22913=CARTESIAN_POINT('Ctrl Pts',(33.6665278606096,31.9138246796869,44.2227638873721));
#22914=CARTESIAN_POINT('Ctrl Pts',(33.6380519378177,31.3631343136376,44.1857206242988));
#22915=CARTESIAN_POINT('Ctrl Pts',(33.3096261699052,30.827954203719,44.1486773612256));
#22916=CARTESIAN_POINT('Ctrl Pts',(32.8315364074553,30.5531798663578,44.1116340981523));
#22917=CARTESIAN_POINT('Ctrl Pts',(32.3534466450053,30.2784055289966,44.0745908350791));
#22918=CARTESIAN_POINT('Ctrl Pts',(31.725692888018,30.2640369641928,44.0375475720059));
#22919=CARTESIAN_POINT('Ctrl Pts',(31.2355318518357,30.5166491492484,44.0005043089327));
#22920=CARTESIAN_POINT('Ctrl Pts',(30.7453708156534,30.769261334304,43.9634610458594));
#22921=CARTESIAN_POINT('Ctrl Pts',(30.3928025002761,31.288854269219,43.9264177827861));
#22922=CARTESIAN_POINT('Ctrl Pts',(30.3391602551023,31.8376650444346,43.8893745197129));
#22923=CARTESIAN_POINT('Ctrl Pts',(30.2855180099285,32.3864758196501,43.8523312566396));
#22924=CARTESIAN_POINT('Ctrl Pts',(30.530801834958,32.9645044351661,43.8152879935664));
#22925=CARTESIAN_POINT('Ctrl Pts',(30.9627711818461,33.3072481305883,43.7782447304932));
#22926=CARTESIAN_POINT('Ctrl Pts',(31.3947405287341,33.6499918260105,43.7412014674199));
#22927=CARTESIAN_POINT('Ctrl Pts',(32.0133953974807,33.7574506013388,43.7041582043467));
#22928=CARTESIAN_POINT('Ctrl Pts',(32.5356426746786,33.5804519039783,43.6671149412734));
#22929=CARTESIAN_POINT('Ctrl Pts',(33.0578899518765,33.4034532066179,43.6300716782002));
#22930=CARTESIAN_POINT('Ctrl Pts',(33.4837296375257,32.9419970365686,43.593028415127));
#22931=CARTESIAN_POINT('Ctrl Pts',(33.6182998004632,32.4072432344611,43.5559851520537));
#22932=CARTESIAN_POINT('Ctrl Pts',(33.6515585595629,32.2750798522248,43.5468299802391));
#22933=CARTESIAN_POINT('Ctrl Pts',(33.6670259413327,32.138439290855,43.5376748084244));
#22934=CARTESIAN_POINT('Ctrl Pts',(33.6657844257744,32.0015219728729,43.5285196366098));
#22935=CARTESIAN_POINT('Origin',(32.,32.,48.));
#22936=CARTESIAN_POINT('',(33.6633867512256,31.999584573057,42.8285196366098));
#22937=CARTESIAN_POINT('',(33.6664085438525,31.9985061360825,43.0214803633902));
#22938=CARTESIAN_POINT('',(33.666,32.,48.));
#22939=CARTESIAN_POINT('Ctrl Pts',(33.6664085438525,31.9985061360825,43.0214803633902));
#22940=CARTESIAN_POINT('Ctrl Pts',(33.6623727759815,32.4357766487213,43.0507471277491));
#22941=CARTESIAN_POINT('Ctrl Pts',(33.4856937087816,32.8759335396009,43.0800138921079));
#22942=CARTESIAN_POINT('Ctrl Pts',(33.1768027043535,33.1831638308965,43.1092806564668));
#22943=CARTESIAN_POINT('Ctrl Pts',(32.7858359887411,33.5720285637718,43.14632391954));
#22944=CARTESIAN_POINT('Ctrl Pts',(32.1830625609484,33.7479416781363,43.1833671826133));
#22945=CARTESIAN_POINT('Ctrl Pts',(31.6443082716033,33.6304062847013,43.2204104456865));
#22946=CARTESIAN_POINT('Ctrl Pts',(31.1055539822583,33.5128708912663,43.2574537087598));
#22947=CARTESIAN_POINT('Ctrl Pts',(30.6308188313608,33.1018869900318,43.294496971833));
#22948=CARTESIAN_POINT('Ctrl Pts',(30.437339050589,32.585518586748,43.3315402349062));
#22949=CARTESIAN_POINT('Ctrl Pts',(30.2438592698172,32.0691501834641,43.3685834979795));
#22950=CARTESIAN_POINT('Ctrl Pts',(30.3316348591709,31.4473972781309,43.4056267610527));
#22951=CARTESIAN_POINT('Ctrl Pts',(30.6605001845156,31.0047706284025,43.442670024126));
#22952=CARTESIAN_POINT('Ctrl Pts',(30.9893655098603,30.5621439786741,43.4797132871992));
#22953=CARTESIAN_POINT('Ctrl Pts',(31.5593205711959,30.2986435845506,43.5167565502724));
#22954=CARTESIAN_POINT('Ctrl Pts',(32.1095570231048,30.3348457978698,43.5537998133457));
#22955=CARTESIAN_POINT('Ctrl Pts',(32.6597934750136,30.3710480111891,43.5908430764189));
#22956=CARTESIAN_POINT('Ctrl Pts',(33.1903113174957,30.7069528319511,43.6278863394922));
#22957=CARTESIAN_POINT('Ctrl Pts',(33.458348462345,31.1888520354127,43.6649296025654));
#22958=CARTESIAN_POINT('Ctrl Pts',(33.5947448739368,31.4340767117839,43.6837798561737));
#22959=CARTESIAN_POINT('Ctrl Pts',(33.6631719076463,31.7171066342395,43.7026301097819));
#22960=CARTESIAN_POINT('Ctrl Pts',(33.6632945194008,32.000080914311,43.7214803633902));
#22961=CARTESIAN_POINT('Ctrl Pts',(33.6657844257744,32.0015219728729,43.5285196366098));
#22962=CARTESIAN_POINT('Ctrl Pts',(33.6620025743914,31.5844503180668,43.5006315453512));
#22963=CARTESIAN_POINT('Ctrl Pts',(33.5031776477221,31.1648106184981,43.4727434540926));
#22964=CARTESIAN_POINT('Ctrl Pts',(33.2199064985647,30.8613299724877,43.444855362834));
#22965=CARTESIAN_POINT('Ctrl Pts',(32.843642393503,30.4582219467875,43.4078120997608));
#22966=CARTESIAN_POINT('Ctrl Pts',(32.2478135431539,30.2600573295529,43.3707688366875));
#22967=CARTESIAN_POINT('Ctrl Pts',(31.7050679985738,30.357515172611,43.3337255736143));
#22968=CARTESIAN_POINT('Ctrl Pts',(31.1623224539937,30.454973015669,43.296682310541));
#22969=CARTESIAN_POINT('Ctrl Pts',(30.6726602151827,30.8480533190197,43.2596390474678));
#22970=CARTESIAN_POINT('Ctrl Pts',(30.4601480677671,31.356884672221,43.2225957843945));
#22971=CARTESIAN_POINT('Ctrl Pts',(30.2476359203515,31.8657160254224,43.1855525213213));
#22972=CARTESIAN_POINT('Ctrl Pts',(30.3122738643314,32.4902984284745,43.1485092582481));
#22973=CARTESIAN_POINT('Ctrl Pts',(30.6244839265721,32.9448263505345,43.1114659951748));
#22974=CARTESIAN_POINT('Ctrl Pts',(30.9366939888128,33.3993542725945,43.0744227321016));
#22975=CARTESIAN_POINT('Ctrl Pts',(31.4964761693141,33.6838277136625,43.0373794690283));
#22976=CARTESIAN_POINT('Ctrl Pts',(32.0476771784704,33.6680731891249,43.0003362059551));
#22977=CARTESIAN_POINT('Ctrl Pts',(32.5988781876267,33.6523186645873,42.9632929428818));
#22978=CARTESIAN_POINT('Ctrl Pts',(33.1414980254379,33.3363361744442,42.9262496798086));
#22979=CARTESIAN_POINT('Ctrl Pts',(33.4272367945752,32.8647175541852,42.8892064167354));
#22980=CARTESIAN_POINT('Ctrl Pts',(33.5832756566817,32.6071717088116,42.8689774900269));
#22981=CARTESIAN_POINT('Ctrl Pts',(33.6627091320695,32.3032130779553,42.8487485633184));
#22982=CARTESIAN_POINT('Ctrl Pts',(33.6633867512256,31.999584573057,42.8285196366098));
#22983=CARTESIAN_POINT('Origin',(32.,32.,48.));
#22984=CARTESIAN_POINT('',(33.6673070786563,31.998696213291,42.1285196366098));
#22985=CARTESIAN_POINT('',(33.6682077659727,32.0008552789479,42.3214803633902));
#22986=CARTESIAN_POINT('',(33.666,32.,48.));
#22987=CARTESIAN_POINT('Ctrl Pts',(33.6682077659727,32.0008552789479,42.3214803633902));
#22988=CARTESIAN_POINT('Ctrl Pts',(33.6685153159273,32.0499810826626,42.3247776195697));
#22989=CARTESIAN_POINT('Ctrl Pts',(33.6665333409633,32.0990817203467,42.3280748757492));
#22990=CARTESIAN_POINT('Ctrl Pts',(33.6621810758368,32.1479713477299,42.3313721319287));
#22991=CARTESIAN_POINT('Ctrl Pts',(33.6132852384284,32.6972254032584,42.368415395002));
#22992=CARTESIAN_POINT('Ctrl Pts',(33.2652217688373,33.2198466637373,42.4054586580752));
#22993=CARTESIAN_POINT('Ctrl Pts',(32.7772628054379,33.4766867130642,42.4425019211484));
#22994=CARTESIAN_POINT('Ctrl Pts',(32.2893038420385,33.7335267623911,42.4795451842217));
#22995=CARTESIAN_POINT('Ctrl Pts',(31.6614493848307,33.7245856005659,42.5165884472949));
#22996=CARTESIAN_POINT('Ctrl Pts',(31.1810021371072,33.4539545340837,42.5536317103682));
#22997=CARTESIAN_POINT('Ctrl Pts',(30.7005548893838,33.1833234676016,42.5906749734414));
#22998=CARTESIAN_POINT('Ctrl Pts',(30.3675148511445,32.6510024964624,42.6277182365146));
#22999=CARTESIAN_POINT('Ctrl Pts',(30.3342793844886,32.1005788716261,42.6647614995879));
#23000=CARTESIAN_POINT('Ctrl Pts',(30.3010439178327,31.5501552467898,42.7018047626611));
#23001=CARTESIAN_POINT('Ctrl Pts',(30.5676130227601,30.9816289682562,42.7388480257344));
#23002=CARTESIAN_POINT('Ctrl Pts',(31.0120060988108,30.6551545475858,42.7758912888076));
#23003=CARTESIAN_POINT('Ctrl Pts',(31.4563991748616,30.3286801269153,42.8129345518809));
#23004=CARTESIAN_POINT('Ctrl Pts',(32.0786162220357,30.2442575641079,42.8499778149541));
#23005=CARTESIAN_POINT('Ctrl Pts',(32.5939341052261,30.4405181816957,42.8870210780273));
#23006=CARTESIAN_POINT('Ctrl Pts',(33.1092519884165,30.6367787992834,42.9240643411006));
#23007=CARTESIAN_POINT('Ctrl Pts',(33.5176707076233,31.1137225972663,42.9611076041738));
#23008=CARTESIAN_POINT('Ctrl Pts',(33.6323000655106,31.6531026719508,42.9981508672471));
#23009=CARTESIAN_POINT('Ctrl Pts',(33.656364226718,31.7663348256369,43.0059273659615));
#23010=CARTESIAN_POINT('Ctrl Pts',(33.6674808914231,31.882318588403,43.0137038646758));
#23011=CARTESIAN_POINT('Ctrl Pts',(33.6664085438525,31.9985061360825,43.0214803633902));
#23012=CARTESIAN_POINT('Ctrl Pts',(33.6633867512256,31.999584573057,42.8285196366098));
#23013=CARTESIAN_POINT('Ctrl Pts',(33.6639499900263,31.7472077720117,42.8117053002451));
#23014=CARTESIAN_POINT('Ctrl Pts',(33.6101009847085,31.495059054249,42.7948909638803));
#23015=CARTESIAN_POINT('Ctrl Pts',(33.5006047722315,31.2699817522125,42.7780766275156));
#23016=CARTESIAN_POINT('Ctrl Pts',(33.2593762802871,30.7741193208738,42.7410333644424));
#23017=CARTESIAN_POINT('Ctrl Pts',(32.7480615959347,30.4096492085713,42.7039901013691));
#23018=CARTESIAN_POINT('Ctrl Pts',(32.2006355392698,30.3433508109352,42.6669468382959));
#23019=CARTESIAN_POINT('Ctrl Pts',(31.653209482605,30.277052413299,42.6299035752227));
#23020=CARTESIAN_POINT('Ctrl Pts',(31.0696720536276,30.508925730329,42.5928603121494));
#23021=CARTESIAN_POINT('Ctrl Pts',(30.7170468295479,30.9328670893641,42.5558170490762));
#23022=CARTESIAN_POINT('Ctrl Pts',(30.3644216054682,31.3568084483991,42.5187737860029));
#23023=CARTESIAN_POINT('Ctrl Pts',(30.242708586286,31.9728178494392,42.4817305229297));
#23024=CARTESIAN_POINT('Ctrl Pts',(30.4076029622781,32.4990121369647,42.4446872598564));
#23025=CARTESIAN_POINT('Ctrl Pts',(30.5724973382702,33.0252064244902,42.4076439967832));
#23026=CARTESIAN_POINT('Ctrl Pts',(31.0239991094365,33.4615855985011,42.37060073371));
#23027=CARTESIAN_POINT('Ctrl Pts',(31.5555035675824,33.6084660906392,42.3335574706367));
#23028=CARTESIAN_POINT('Ctrl Pts',(32.0870080257284,33.7553465827773,42.2965142075635));
#23029=CARTESIAN_POINT('Ctrl Pts',(32.698515170854,33.6127283930426,42.2594709444902));
#23030=CARTESIAN_POINT('Ctrl Pts',(33.1102025419581,33.2458705045939,42.222427681417));
#23031=CARTESIAN_POINT('Ctrl Pts',(33.4580908657248,32.9358644542971,42.1911249998146));
#23032=CARTESIAN_POINT('Ctrl Pts',(33.6632926257187,32.4657341508945,42.1598223182122));
#23033=CARTESIAN_POINT('Ctrl Pts',(33.6673070786563,31.998696213291,42.1285196366098));
#23034=CARTESIAN_POINT('Origin',(32.,32.,48.));
#23035=CARTESIAN_POINT('',(33.6674739163907,32.0012102324881,41.4285196366098));
#23036=CARTESIAN_POINT('',(33.6638410485742,32.0009454217316,41.6214803633902));
#23037=CARTESIAN_POINT('',(33.666,32.,48.));
#23038=CARTESIAN_POINT('',(30.7309291201476,33.0793586530485,41.));
#23039=CARTESIAN_POINT('Ctrl Pts',(33.6674739163907,32.0012102324881,41.4285196366098));
#23040=CARTESIAN_POINT('Ctrl Pts',(33.6635382116946,31.5283279659125,41.3968095469596));
#23041=CARTESIAN_POINT('Ctrl Pts',(33.4523210017542,31.0524651525534,41.3650994573094));
#23042=CARTESIAN_POINT('Ctrl Pts',(33.0964756390096,30.7421790963558,41.3333893676592));
#23043=CARTESIAN_POINT('Ctrl Pts',(32.6807822893234,30.3797074624224,41.296346104586));
#23044=CARTESIAN_POINT('Ctrl Pts',(32.067721107232,30.2431913221054,41.2593028415127));
#23045=CARTESIAN_POINT('Ctrl Pts',(31.5378645260577,30.3962173009215,41.2222595784394));
#23046=CARTESIAN_POINT('Ctrl Pts',(31.0080079448833,30.5492432797376,41.1852163153662));
#23047=CARTESIAN_POINT('Ctrl Pts',(30.5613559646262,30.9918113776869,41.148173052293));
#23048=CARTESIAN_POINT('Ctrl Pts',(30.4023646913452,31.5188488463209,41.1111297892197));
#23049=CARTESIAN_POINT('Ctrl Pts',(30.2433734180642,32.0458863149549,41.0740865261465));
#23050=CARTESIAN_POINT('Ctrl Pts',(30.3720428517593,32.6573931542737,41.0370432630732));
#23051=CARTESIAN_POINT('Ctrl Pts',(30.7309291201476,33.0793586530485,41.));
#23052=CARTESIAN_POINT('',(33.2714670682823,33.0812099660022,41.));
#23053=CARTESIAN_POINT('Origin',(32.,32.,41.));
#23054=CARTESIAN_POINT('Ctrl Pts',(33.2714683883714,33.0812109859128,41.));
#23055=CARTESIAN_POINT('Ctrl Pts',(32.9206802907987,33.4926491725661,41.0363148168372));
#23056=CARTESIAN_POINT('Ctrl Pts',(32.350892837512,33.7186726653411,41.0726296336745));
#23057=CARTESIAN_POINT('Ctrl Pts',(31.8135997899101,33.6581999673401,41.1089444505117));
#23058=CARTESIAN_POINT('Ctrl Pts',(31.2655290726889,33.5965142352919,41.145987713585));
#23059=CARTESIAN_POINT('Ctrl Pts',(30.7512694596539,33.2367232647846,41.1830309766582));
#23060=CARTESIAN_POINT('Ctrl Pts',(30.5058095822466,32.7430255187007,41.2200742397314));
#23061=CARTESIAN_POINT('Ctrl Pts',(30.2603497048393,32.2493277726168,41.2571175028047));
#23062=CARTESIAN_POINT('Ctrl Pts',(30.2836895630596,31.6217232509564,41.2941607658779));
#23063=CARTESIAN_POINT('Ctrl Pts',(30.5653172802778,31.1476214797862,41.3312040289512));
#23064=CARTESIAN_POINT('Ctrl Pts',(30.8469449974961,30.6735197086161,41.3682472920244));
#23065=CARTESIAN_POINT('Ctrl Pts',(31.3868605737123,30.3529206879363,41.4052905550977));
#23066=CARTESIAN_POINT('Ctrl Pts',(31.9379165708235,30.3324171997514,41.4423338181709));
#23067=CARTESIAN_POINT('Ctrl Pts',(32.4889725679347,30.3119137115664,41.4793770812441));
#23068=CARTESIAN_POINT('Ctrl Pts',(33.0511689859409,30.5915057558763,41.5164203443174));
#23069=CARTESIAN_POINT('Ctrl Pts',(33.3672907256419,31.0433098899838,41.5534636073906));
#23070=CARTESIAN_POINT('Ctrl Pts',(33.5607723779188,31.3198356691197,41.5761358593905));
#23071=CARTESIAN_POINT('Ctrl Pts',(33.6620738029635,31.6608725539045,41.5988081113903));
#23072=CARTESIAN_POINT('Ctrl Pts',(33.6638410485742,32.0009454217316,41.6214803633902));
#23073=CARTESIAN_POINT('Origin',(32.,32.,39.4540747194623));
#23074=CARTESIAN_POINT('',(34.0532846274147,32.0018314602113,53.7459252805377));
#23075=CARTESIAN_POINT('',(34.0546389144305,31.9981689288227,53.8040747194623));
#23076=CARTESIAN_POINT('',(34.05475,32.0000000000002,39.4540747194623));
#23077=CARTESIAN_POINT('',(31.6163320011532,34.0186125009919,54.));
#23078=CARTESIAN_POINT('Ctrl Pts',(34.0546389144305,31.9981689288227,53.8040747194623));
#23079=CARTESIAN_POINT('Ctrl Pts',(34.049372166387,32.5196382919465,53.832339883235));
#23080=CARTESIAN_POINT('Ctrl Pts',(33.5817166966653,33.7322181453664,53.8976483100809));
#23081=CARTESIAN_POINT('Ctrl Pts',(32.2875197530249,34.146181938655,53.9629567369268));
#23082=CARTESIAN_POINT('Ctrl Pts',(31.6163320011532,34.0186125009919,54.));
#23083=CARTESIAN_POINT('',(30.6584342291726,33.5612633655757,54.));
#23084=CARTESIAN_POINT('Origin',(32.,32.,54.));
#23085=CARTESIAN_POINT('Ctrl Pts',(34.0532846274147,32.0018314602113,53.7459252805377));
#23086=CARTESIAN_POINT('Ctrl Pts',(34.0549510377389,32.2111834105163,53.7572587737813));
#23087=CARTESIAN_POINT('Ctrl Pts',(33.9292547992907,33.10278246478,53.8056355300982));
#23088=CARTESIAN_POINT('Ctrl Pts',(32.6546770842451,34.3305889284731,53.8903271032523));
#23089=CARTESIAN_POINT('Ctrl Pts',(31.1647629090491,33.9952107638275,53.9636851831627));
#23090=CARTESIAN_POINT('Ctrl Pts',(30.6584328166059,33.5612648614875,54.));
#23091=CARTESIAN_POINT('Origin',(32.,32.,39.4540747194623));
#23092=CARTESIAN_POINT('',(34.0520083050621,31.9988943672661,53.0459252805377));
#23093=CARTESIAN_POINT('',(34.0578094464953,32.0007573833008,53.1040747194624));
#23094=CARTESIAN_POINT('',(34.05475,32.0000000000002,39.4540747194623));
#23095=CARTESIAN_POINT('Ctrl Pts',(34.0578094464953,32.0007573833008,53.1040747194624));
#23096=CARTESIAN_POINT('Ctrl Pts',(34.0580096988745,32.0429235568551,53.1063703750556));
#23097=CARTESIAN_POINT('Ctrl Pts',(34.037719062628,32.7652974437369,53.1457092937222));
#23098=CARTESIAN_POINT('Ctrl Pts',(33.188671276515,34.1177969804317,53.2220914754619));
#23099=CARTESIAN_POINT('Ctrl Pts',(30.8656743329815,34.1473078555715,53.3332212646817));
#23100=CARTESIAN_POINT('Ctrl Pts',(29.5804895506539,32.2117839119326,53.4443510539014));
#23101=CARTESIAN_POINT('Ctrl Pts',(30.5102290402516,30.0821246648111,53.5554808431211));
#23102=CARTESIAN_POINT('Ctrl Pts',(32.8021732937378,29.7083047001831,53.6666106323408));
#23103=CARTESIAN_POINT('Ctrl Pts',(33.9655643210943,30.9925292306587,53.7494752577879));
#23104=CARTESIAN_POINT('Ctrl Pts',(34.0562745687535,31.8362201112415,53.7952966201617));
#23105=CARTESIAN_POINT('Ctrl Pts',(34.0546389144305,31.9981689288227,53.8040747194623));
#23106=CARTESIAN_POINT('Ctrl Pts',(34.0520083050621,31.9988943672661,53.0459252805377));
#23107=CARTESIAN_POINT('Ctrl Pts',(34.0499814160986,32.4134550802263,53.0683325286752));
#23108=CARTESIAN_POINT('Ctrl Pts',(33.7267546549923,33.5162657199585,53.127783039886));
#23109=CARTESIAN_POINT('Ctrl Pts',(31.9269572256365,34.4274725972727,53.2242768141699));
#23110=CARTESIAN_POINT('Ctrl Pts',(29.9209961576786,33.2553327321614,53.3354066033897));
#23111=CARTESIAN_POINT('Ctrl Pts',(29.8177590626321,30.9342477419074,53.4465363926093));
#23112=CARTESIAN_POINT('Ctrl Pts',(31.7116016611041,29.5886825160599,53.5576661818292));
#23113=CARTESIAN_POINT('Ctrl Pts',(33.6494719816339,30.36181998904,53.6574624778052));
#23114=CARTESIAN_POINT('Ctrl Pts',(34.0495044137635,31.5269213561486,53.7202155107081));
#23115=CARTESIAN_POINT('Ctrl Pts',(34.0532846274147,32.0018314602113,53.7459252805377));
#23116=CARTESIAN_POINT('Origin',(32.,32.,39.4540747194623));
#23117=CARTESIAN_POINT('',(34.0573711123367,31.9988731525912,52.3459252805377));
#23118=CARTESIAN_POINT('',(34.0524438258503,32.0013942153142,52.4040747194624));
#23119=CARTESIAN_POINT('',(34.05475,32.0000000000002,39.4540747194623));
#23120=CARTESIAN_POINT('Ctrl Pts',(34.0524438258503,32.0013942153142,52.4040747194623));
#23121=CARTESIAN_POINT('Ctrl Pts',(34.0539875421913,32.2486122323593,52.4174441299495));
#23122=CARTESIAN_POINT('Ctrl Pts',(33.8982128380036,33.1789291235334,52.4678568035099));
#23123=CARTESIAN_POINT('Ctrl Pts',(32.5140660369754,34.3735522478524,52.5553127401435));
#23124=CARTESIAN_POINT('Ctrl Pts',(30.2847730690242,33.7193028360775,52.6664425293633));
#23125=CARTESIAN_POINT('Ctrl Pts',(29.6252320317178,31.4915687389112,52.7775723185829));
#23126=CARTESIAN_POINT('Ctrl Pts',(31.1390630925179,29.7291402212096,52.8887021078028));
#23127=CARTESIAN_POINT('Ctrl Pts',(33.3932462266972,30.0384636275678,52.9975362414291));
#23128=CARTESIAN_POINT('Ctrl Pts',(34.0547783772501,31.3625198132227,53.0693271119824));
#23129=CARTESIAN_POINT('Ctrl Pts',(34.0578094464953,32.0007573833008,53.1040747194624));
#23130=CARTESIAN_POINT('Ctrl Pts',(34.0573711123367,31.9988731525912,52.3459252805377));
#23131=CARTESIAN_POINT('Ctrl Pts',(34.0533078419724,32.6141860750411,52.3794062835691));
#23132=CARTESIAN_POINT('Ctrl Pts',(33.4332399393382,33.917382784162,52.4499305496737));
#23133=CARTESIAN_POINT('Ctrl Pts',(31.216995453309,34.2988945058415,52.5574980788517));
#23134=CARTESIAN_POINT('Ctrl Pts',(29.6439536232049,32.5891178954443,52.6686278680713));
#23135=CARTESIAN_POINT('Ctrl Pts',(30.2271405879685,30.340185676392,52.7797576572911));
#23136=CARTESIAN_POINT('Ctrl Pts',(32.4328278728442,29.6103000988841,52.8908874465108));
#23137=CARTESIAN_POINT('Ctrl Pts',(33.8775323764099,30.773632426936,52.979609987593));
#23138=CARTESIAN_POINT('Ctrl Pts',(34.0533322327912,31.7281107016673,53.031289265602));
#23139=CARTESIAN_POINT('Ctrl Pts',(34.0520083050621,31.9988943672661,53.0459252805377));
#23140=CARTESIAN_POINT('Origin',(32.,32.,39.4540747194623));
#23141=CARTESIAN_POINT('',(34.0554020230033,32.0018240973642,51.6459252805377));
#23142=CARTESIAN_POINT('',(34.0527564569811,31.9984585482624,51.7040747194623));
#23143=CARTESIAN_POINT('',(34.05475,32.0000000000002,39.4540747194623));
#23144=CARTESIAN_POINT('Ctrl Pts',(34.0527564569812,31.9984585482624,51.7040747194623));
#23145=CARTESIAN_POINT('Ctrl Pts',(34.0496054294021,32.4502717890878,51.7285178848434));
#23146=CARTESIAN_POINT('Ctrl Pts',(33.6800481554996,33.5914868140557,51.7900043132977));
#23147=CARTESIAN_POINT('Ctrl Pts',(31.7940455819115,34.4198338709223,51.8885340048252));
#23148=CARTESIAN_POINT('Ctrl Pts',(29.8553459812909,33.1395052258002,51.9996637940449));
#23149=CARTESIAN_POINT('Ctrl Pts',(29.879410395147,30.8163137990511,52.1107935832647));
#23150=CARTESIAN_POINT('Ctrl Pts',(31.8442155880729,29.5764190605415,52.2219233724844));
#23151=CARTESIAN_POINT('Ctrl Pts',(33.6980657674601,30.436884819778,52.3196837512169));
#23152=CARTESIAN_POINT('Ctrl Pts',(34.0497102937227,31.5636334854927,52.3804008668763));
#23153=CARTESIAN_POINT('Ctrl Pts',(34.0524438258503,32.0013942153142,52.4040747194623));
#23154=CARTESIAN_POINT('Ctrl Pts',(34.0554020230033,32.0018240973642,51.6459252805377));
#23155=CARTESIAN_POINT('Ctrl Pts',(34.0566763784363,32.1402143135672,51.6534367753898));
#23156=CARTESIAN_POINT('Ctrl Pts',(33.9808503772797,32.9596933290486,51.697991533315));
#23157=CARTESIAN_POINT('Ctrl Pts',(32.8805414680095,34.2633293614917,51.7795895543134));
#23158=CARTESIAN_POINT('Ctrl Pts',(30.5761492876849,33.9673998582603,51.8907193435333));
#23159=CARTESIAN_POINT('Ctrl Pts',(29.5748498323699,31.8709273512164,52.0018491327529));
#23160=CARTESIAN_POINT('Ctrl Pts',(30.7930215224583,29.8925807110175,52.1129789219727));
#23161=CARTESIAN_POINT('Ctrl Pts',(33.1158068029996,29.8429213928206,52.2241087111924));
#23162=CARTESIAN_POINT('Ctrl Pts',(34.0252705758902,31.1875940610687,52.3017574973808));
#23163=CARTESIAN_POINT('Ctrl Pts',(34.0578034299003,31.9334060387527,52.3423630204959));
#23164=CARTESIAN_POINT('Ctrl Pts',(34.0573711123367,31.9988731525912,52.3459252805377));
#23165=CARTESIAN_POINT('Origin',(32.,32.,39.4540747194623));
#23166=CARTESIAN_POINT('',(34.0514089815509,31.9999806721048,50.9459252805377));
#23167=CARTESIAN_POINT('',(34.0579890960703,31.9994845671529,51.0040747194623));
#23168=CARTESIAN_POINT('',(34.05475,32.0000000000002,39.4540747194623));
#23169=CARTESIAN_POINT('Ctrl Pts',(34.0579890960703,31.9994845671529,51.0040747194623));
#23170=CARTESIAN_POINT('Ctrl Pts',(34.0557930142123,32.6516937718654,51.0395916397372));
#23171=CARTESIAN_POINT('Ctrl Pts',(33.3683017971665,33.9881257659273,51.1121518230855));
#23172=CARTESIAN_POINT('Ctrl Pts',(31.0922024415436,34.2525356254733,51.2217552695068));
#23173=CARTESIAN_POINT('Ctrl Pts',(29.6152124997993,32.4591314922087,51.3328850587266));
#23174=CARTESIAN_POINT('Ctrl Pts',(30.3207542148726,30.2455351970729,51.4440148479463));
#23175=CARTESIAN_POINT('Ctrl Pts',(32.5631234646485,29.6376060617633,51.5551446371661));
#23176=CARTESIAN_POINT('Ctrl Pts',(33.9102709101462,30.8498857953214,51.6418312610047));
#23177=CARTESIAN_POINT('Ctrl Pts',(34.0543807660552,31.7655553671776,51.6914746217701));
#23178=CARTESIAN_POINT('Ctrl Pts',(34.0527564569812,31.9984585482624,51.7040747194623));
#23179=CARTESIAN_POINT('Ctrl Pts',(34.0514089815509,31.9999806721048,50.9459252805377));
#23180=CARTESIAN_POINT('Ctrl Pts',(34.0513801084989,32.3440804516646,50.9645105302836));
#23181=CARTESIAN_POINT('Ctrl Pts',(33.8061927971795,33.3740627169736,51.0201390431027));
#23182=CARTESIAN_POINT('Ctrl Pts',(32.1767300276281,34.4221435893461,51.1128108189952));
#23183=CARTESIAN_POINT('Ctrl Pts',(30.0609756305588,33.4622576942574,51.2239406082148));
#23184=CARTESIAN_POINT('Ctrl Pts',(29.7197953084608,31.1641294150899,51.3350703974346));
#23185=CARTESIAN_POINT('Ctrl Pts',(31.4654335924627,29.6309808302345,51.4462001866543));
#23186=CARTESIAN_POINT('Ctrl Pts',(33.5492418761722,30.2230151611312,51.549818481022));
#23187=CARTESIAN_POINT('Ctrl Pts',(34.0503918392758,31.457736952328,51.6163935123165));
#23188=CARTESIAN_POINT('Ctrl Pts',(34.0554020230033,32.0018240973642,51.6459252805377));
#23189=CARTESIAN_POINT('Origin',(32.,32.,39.4540747194623));
#23190=CARTESIAN_POINT('',(34.0554729559656,31.9981860521685,50.2459252805377));
#23191=CARTESIAN_POINT('',(34.0542687898145,32.00186850902,50.3040747194623));
#23192=CARTESIAN_POINT('',(34.05475,32.0000000000002,39.4540747194623));
#23193=CARTESIAN_POINT('Ctrl Pts',(34.0542687898145,32.00186850902,50.3040747194623));
#23194=CARTESIAN_POINT('Ctrl Pts',(34.0558441392389,32.1780164452784,50.3136221315579));
#23195=CARTESIAN_POINT('Ctrl Pts',(33.9544817783467,33.0358200834104,50.3602128067267));
#23196=CARTESIAN_POINT('Ctrl Pts',(32.7551980676263,34.3081787255302,50.4438467449689));
#23197=CARTESIAN_POINT('Ctrl Pts',(30.4704836368621,33.8864232942922,50.5549765341884));
#23198=CARTESIAN_POINT('Ctrl Pts',(29.5855659947393,31.7382337215207,50.6661063234083));
#23199=CARTESIAN_POINT('Ctrl Pts',(30.910312170761,29.8296098080883,50.7772361126278));
#23200=CARTESIAN_POINT('Ctrl Pts',(33.2323288309766,29.9073034613682,50.8883659018477));
#23201=CARTESIAN_POINT('Ctrl Pts',(34.0448660563587,31.2632801450257,50.9639787707924));
#23202=CARTESIAN_POINT('Ctrl Pts',(34.0580834728828,31.9714558187451,51.002548376664));
#23203=CARTESIAN_POINT('Ctrl Pts',(34.0579890960703,31.9994845671529,51.0040747194623));
#23204=CARTESIAN_POINT('Ctrl Pts',(34.0554729559656,31.9981860521685,50.2459252805377));
#23205=CARTESIAN_POINT('Ctrl Pts',(34.0504505772786,32.544568857989,50.2755842851775));
#23206=CARTESIAN_POINT('Ctrl Pts',(33.5457057188836,33.7815642256422,50.3422865528905));
#23207=CARTESIAN_POINT('Ctrl Pts',(31.4573199785767,34.3671737292195,50.4460320836768));
#23208=CARTESIAN_POINT('Ctrl Pts',(29.7169448259793,32.828053224334,50.5571618728965));
#23209=CARTESIAN_POINT('Ctrl Pts',(30.0659970099416,30.5311073884045,50.6682916621163));
#23210=CARTESIAN_POINT('Ctrl Pts',(32.1850277570195,29.5784761411241,50.7794214513359));
#23211=CARTESIAN_POINT('Ctrl Pts',(33.8086577448288,30.6306870895215,50.8719659908098));
#23212=CARTESIAN_POINT('Ctrl Pts',(34.0514376569353,31.6582366329401,50.9274672672104));
#23213=CARTESIAN_POINT('Ctrl Pts',(34.0514089815509,31.9999806721048,50.9459252805377));
#23214=CARTESIAN_POINT('Origin',(32.,32.,39.4540747194623));
#23215=CARTESIAN_POINT('',(34.0573203109033,32.0011604784082,49.5459252805377));
#23216=CARTESIAN_POINT('',(34.0515870545632,31.9993739458396,49.6040747194623));
#23217=CARTESIAN_POINT('',(34.05475,32.0000000000002,39.4540747194623));
#23218=CARTESIAN_POINT('Ctrl Pts',(34.0515870545632,31.9993739458396,49.6040747194623));
#23219=CARTESIAN_POINT('Ctrl Pts',(34.0505442952487,32.3810853728681,49.6246958864518));
#23220=CARTESIAN_POINT('Ctrl Pts',(33.7651923599736,33.4499404762536,49.6823603165144));
#23221=CARTESIAN_POINT('Ctrl Pts',(32.0437417130131,34.4281885867619,49.7770680096504));
#23222=CARTESIAN_POINT('Ctrl Pts',(29.9837635432384,33.3538108068575,49.8881977988701));
#23223=CARTESIAN_POINT('Ctrl Pts',(29.7690231135183,31.0404400579838,49.9993275880899));
#23224=CARTESIAN_POINT('Ctrl Pts',(31.5960485363689,29.6052481620493,50.1104573773095));
#23225=CARTESIAN_POINT('Ctrl Pts',(33.6040409849523,30.2967180694215,50.2120397544338));
#23226=CARTESIAN_POINT('Ctrl Pts',(34.0497318982905,31.4945752910354,50.2765788684846));
#23227=CARTESIAN_POINT('Ctrl Pts',(34.0542687898145,32.00186850902,50.3040747194623));
#23228=CARTESIAN_POINT('Ctrl Pts',(34.0573203109033,32.0011604784082,49.5459252805377));
#23229=CARTESIAN_POINT('Ctrl Pts',(34.0577787278171,32.0689703479572,49.5496147769981));
#23230=CARTESIAN_POINT('Ctrl Pts',(34.023973004455,32.8171418610241,49.5903475365318));
#23231=CARTESIAN_POINT('Ctrl Pts',(33.1084096674749,34.160888955732,49.6681235591387));
#23232=CARTESIAN_POINT('Ctrl Pts',(30.7858081444514,34.1032715487725,49.7792533483584));
#23233=CARTESIAN_POINT('Ctrl Pts',(29.5744218402637,32.1207628294065,49.8903831375782));
#23234=CARTESIAN_POINT('Ctrl Pts',(30.5828983635668,30.0277332781861,50.0015129267979));
#23235=CARTESIAN_POINT('Ctrl Pts',(32.8882909367063,29.7397008424277,50.1126427160176));
#23236=CARTESIAN_POINT('Ctrl Pts',(33.9824181138614,31.0450604721018,50.1941135005975));
#23237=CARTESIAN_POINT('Ctrl Pts',(34.0567233870784,31.8621520924731,50.2385410221042));
#23238=CARTESIAN_POINT('Ctrl Pts',(34.0554729559656,31.9981860521685,50.2459252805377));
#23239=CARTESIAN_POINT('Origin',(32.,32.,39.4540747194623));
#23240=CARTESIAN_POINT('',(34.0519709427639,32.0010746754271,48.8459252805377));
#23241=CARTESIAN_POINT('',(34.0565622062779,31.9984640573749,48.9040747194623));
#23242=CARTESIAN_POINT('',(34.05475,32.0000000000002,39.4540747194623));
#23243=CARTESIAN_POINT('Ctrl Pts',(34.0565622062779,31.9984640573749,48.9040747194623));
#23244=CARTESIAN_POINT('Ctrl Pts',(34.0516979975066,32.5815526738416,48.9357696413457));
#23245=CARTESIAN_POINT('Ctrl Pts',(33.4873125068621,33.8543563214718,49.0045078263022));
#23246=CARTESIAN_POINT('Ctrl Pts',(31.3284246119414,34.3338808128292,49.1102892743321));
#23247=CARTESIAN_POINT('Ctrl Pts',(29.6750012209723,32.7017077937846,49.2214190635517));
#23248=CARTESIAN_POINT('Ctrl Pts',(30.1493914990076,30.4273394115725,49.3325488527715));
#23249=CARTESIAN_POINT('Ctrl Pts',(32.3174386081376,29.5922529450954,49.4436786419912));
#23250=CARTESIAN_POINT('Ctrl Pts',(33.8465760377496,30.7067804380472,49.5341872642215));
#23251=CARTESIAN_POINT('Ctrl Pts',(34.0524174776748,31.6953900959366,49.5876526233785));
#23252=CARTESIAN_POINT('Ctrl Pts',(34.0515870545632,31.9993739458396,49.6040747194623));
#23253=CARTESIAN_POINT('Ctrl Pts',(34.0519709427639,32.0010746754271,48.8459252805377));
#23254=CARTESIAN_POINT('Ctrl Pts',(34.0532664462955,32.2742243958035,48.860688531892));
#23255=CARTESIAN_POINT('Ctrl Pts',(33.8753960544161,33.231129995864,48.9124950463196));
#23256=CARTESIAN_POINT('Ctrl Pts',(32.4246384893326,34.3911702623054,49.0013448238203));
#23257=CARTESIAN_POINT('Ctrl Pts',(30.221463738974,33.6537296750593,49.1124746130401));
#23258=CARTESIAN_POINT('Ctrl Pts',(29.6459860872837,31.4028136231505,49.2236044022597));
#23259=CARTESIAN_POINT('Ctrl Pts',(31.2248764402936,29.6984360671178,49.3347341914796));
#23260=CARTESIAN_POINT('Ctrl Pts',(33.4371809965651,30.0870788803797,49.4421744842388));
#23261=CARTESIAN_POINT('Ctrl Pts',(34.0531761327167,31.3881460502207,49.5125715139249));
#23262=CARTESIAN_POINT('Ctrl Pts',(34.0573203109033,32.0011604784082,49.5459252805377));
#23263=CARTESIAN_POINT('Origin',(32.,32.,39.4540747194623));
#23264=CARTESIAN_POINT('',(34.0534017644819,31.9982546442701,48.1459252805377));
#23265=CARTESIAN_POINT('',(34.056370018364,32.0016034368772,48.2040747194623));
#23266=CARTESIAN_POINT('',(34.05475,32.0000000000002,39.4540747194623));
#23267=CARTESIAN_POINT('Ctrl Pts',(34.056370018364,32.0016034368772,48.2040747194623));
#23268=CARTESIAN_POINT('Ctrl Pts',(34.0572746605115,32.1069589678349,48.2098001331663));
#23269=CARTESIAN_POINT('Ctrl Pts',(34.0020142307117,32.893010264768,48.2525688099435));
#23270=CARTESIAN_POINT('Ctrl Pts',(32.9883371997446,34.2183784009811,48.3323807497939));
#23271=CARTESIAN_POINT('Ctrl Pts',(30.672382333998,34.0335792296485,48.4435105390137));
#23272=CARTESIAN_POINT('Ctrl Pts',(29.5714487587624,31.98767040059,48.5546403282333));
#23273=CARTESIAN_POINT('Ctrl Pts',(30.6930989429659,29.9530454872026,48.6657701174531));
#23274=CARTESIAN_POINT('Ctrl Pts',(33.0108108018152,29.7917711456301,48.7768999066728));
#23275=CARTESIAN_POINT('Ctrl Pts',(34.0062530028036,31.1210534192114,48.8563347740093));
#23276=CARTESIAN_POINT('Ctrl Pts',(34.0573830143626,31.9000711073529,48.8987263782724));
#23277=CARTESIAN_POINT('Ctrl Pts',(34.0565622062779,31.9984640573749,48.9040747194623));
#23278=CARTESIAN_POINT('Ctrl Pts',(34.0534017644819,31.9982546442701,48.1459252805377));
#23279=CARTESIAN_POINT('Ctrl Pts',(34.0495479088292,32.475453386869,48.1717622867859));
#23280=CARTESIAN_POINT('Ctrl Pts',(33.6462463167416,33.6427000934394,48.2346425561073));
#23281=CARTESIAN_POINT('Ctrl Pts',(31.7033877194777,34.4104012580895,48.3345660885019));
#23282=CARTESIAN_POINT('Ctrl Pts',(29.81409712657,33.0582257310643,48.4456958777218));
#23283=CARTESIAN_POINT('Ctrl Pts',(29.9253211382958,30.7375734909492,48.5568256669414));
#23284=CARTESIAN_POINT('Ctrl Pts',(31.935268745298,29.572280301472,48.6679554561612));
#23285=CARTESIAN_POINT('Ctrl Pts',(33.7295722946507,30.4884531450101,48.7643219940265));
#23286=CARTESIAN_POINT('Ctrl Pts',(34.0500158291392,31.5888498324735,48.8236452688188));
#23287=CARTESIAN_POINT('Ctrl Pts',(34.0519709427639,32.0010746754271,48.8459252805377));
#23288=CARTESIAN_POINT('Origin',(32.,32.,39.4540747194623));
#23289=CARTESIAN_POINT('',(34.0581463365634,31.9999545509518,47.4459252805377));
#23290=CARTESIAN_POINT('',(34.0515290664373,32.0005167771758,47.5040747194623));
#23291=CARTESIAN_POINT('',(34.05475,32.0000000000002,39.4540747194623));
#23292=CARTESIAN_POINT('Ctrl Pts',(34.0515290664373,32.0005167771758,47.5040747194623));
#23293=CARTESIAN_POINT('Ctrl Pts',(34.0522291585822,32.311502433739,47.5208738880601));
#23294=CARTESIAN_POINT('Ctrl Pts',(33.8397674344737,33.3073239463972,47.5747163197312));
#23295=CARTESIAN_POINT('Ctrl Pts',(32.2929749187864,34.410846085361,47.6656020144756));
#23296=CARTESIAN_POINT('Ctrl Pts',(30.1335187134828,33.5537891611861,47.7767318036953));
#23297=CARTESIAN_POINT('Ctrl Pts',(29.682245940453,31.2747212468355,47.8878615929151));
#23298=CARTESIAN_POINT('Ctrl Pts',(31.3521565477245,29.6594205820605,47.9989913821348));
#23299=CARTESIAN_POINT('Ctrl Pts',(33.4983863486385,30.1590534794509,48.1043957576505));
#23300=CARTESIAN_POINT('Ctrl Pts',(34.0514216516656,31.4253116928468,48.172756870093));
#23301=CARTESIAN_POINT('Ctrl Pts',(34.056370018364,32.0016034368772,48.2040747194623));
#23302=CARTESIAN_POINT('Ctrl Pts',(34.0581458524653,31.9999545574299,47.4459252805377));
#23303=CARTESIAN_POINT('Ctrl Pts',(34.0579253430689,32.6776207312427,47.4828360416797));
#23304=CARTESIAN_POINT('Ctrl Pts',(33.3217860203539,34.0357962998308,47.5567900658952));
#23305=CARTESIAN_POINT('Ctrl Pts',(31.0083166470601,34.21688457017,47.6677873531835));
#23306=CARTESIAN_POINT('Ctrl Pts',(29.5996634424752,32.3693202953617,47.7789171424034));
#23307=CARTESIAN_POINT('Ctrl Pts',(30.387772224771,30.1837580913501,47.890046931623));
#23308=CARTESIAN_POINT('Ctrl Pts',(32.6513743830742,29.6604007858116,48.0011767208428));
#23309=CARTESIAN_POINT('Ctrl Pts',(33.9311687217662,30.9020862526129,48.0864695038143));
#23310=CARTESIAN_POINT('Ctrl Pts',(34.0550732931334,31.791279748851,48.1347190237126));
#23311=CARTESIAN_POINT('Ctrl Pts',(34.0534017644819,31.9982546442701,48.1459252805377));
#23312=CARTESIAN_POINT('Origin',(32.,32.,39.4540747194623));
#23313=CARTESIAN_POINT('',(34.0535341854227,32.0017741341213,46.7459252805377));
#23314=CARTESIAN_POINT('',(34.0544757475471,31.9981230672873,46.8040747194623));
#23315=CARTESIAN_POINT('',(34.05475,32.0000000000002,39.4540747194623));
#23316=CARTESIAN_POINT('Ctrl Pts',(34.0544757475471,31.9981230672873,46.8040747194623));
#23317=CARTESIAN_POINT('Ctrl Pts',(34.0498160689549,32.5122411920882,46.831947642954));
#23318=CARTESIAN_POINT('Ctrl Pts',(33.5941431568701,33.7169900210427,46.896863829519));
#23319=CARTESIAN_POINT('Ctrl Pts',(31.571753982492,34.3905268245362,46.9988232791573));
#23320=CARTESIAN_POINT('Ctrl Pts',(29.7593951208157,32.9368580072316,47.1099530683769));
#23321=CARTESIAN_POINT('Ctrl Pts',(29.9976135462207,30.6257869015107,47.2210828575967));
#23322=CARTESIAN_POINT('Ctrl Pts',(32.0683943391477,29.5723807208067,47.3322126468164));
#23323=CARTESIAN_POINT('Ctrl Pts',(33.7730095526596,30.5640931209952,47.4265432674383));
#23324=CARTESIAN_POINT('Ctrl Pts',(34.0506854097146,31.6257587660702,47.4838306249869));
#23325=CARTESIAN_POINT('Ctrl Pts',(34.0515290664373,32.0005167771758,47.5040747194623));
#23326=CARTESIAN_POINT('Ctrl Pts',(34.0535341854227,32.0017741341213,46.7459252805377));
#23327=CARTESIAN_POINT('Ctrl Pts',(34.055200921409,32.2038215482488,46.7568665335004));
#23328=CARTESIAN_POINT('Ctrl Pts',(33.9350055282046,33.0879912574129,46.8048510495364));
#23329=CARTESIAN_POINT('Ctrl Pts',(32.6680530537252,34.3348914722883,46.8898788286455));
#23330=CARTESIAN_POINT('Ctrl Pts',(30.4007738795658,33.8277004365258,47.0010086178653));
#23331=CARTESIAN_POINT('Ctrl Pts',(29.5970891079424,31.6478177818408,47.112138407085));
#23332=CARTESIAN_POINT('Ctrl Pts',(30.9925223262469,29.790248473958,47.2232681963047));
#23333=CARTESIAN_POINT('Ctrl Pts',(33.3099881859296,29.9550197989514,47.3343979855245));
#23334=CARTESIAN_POINT('Ctrl Pts',(34.0570411385846,31.3149910839429,47.4086170136021));
#23335=CARTESIAN_POINT('Ctrl Pts',(34.058146644048,31.9975218772589,47.4457927786065));
#23336=CARTESIAN_POINT('Ctrl Pts',(34.0581458524653,31.9999545574299,47.4459252805377));
#23337=CARTESIAN_POINT('Origin',(32.,32.,39.4540747194623));
#23338=CARTESIAN_POINT('',(34.0518959992412,31.9989927018737,46.0459252805377));
#23339=CARTESIAN_POINT('',(34.0579058799806,32.0006373862481,46.1040747194624));
#23340=CARTESIAN_POINT('',(34.05475,32.0000000000002,39.4540747194623));
#23341=CARTESIAN_POINT('Ctrl Pts',(34.0579058799806,32.0006373862481,46.1040747194624));
#23342=CARTESIAN_POINT('Ctrl Pts',(34.0580482407791,32.0355942190053,46.1059781347747));
#23343=CARTESIAN_POINT('Ctrl Pts',(34.0414007574156,32.7507240455061,46.1449248131603));
#23344=CARTESIAN_POINT('Ctrl Pts',(33.2110168799234,34.1051012486052,46.2209147546191));
#23345=CARTESIAN_POINT('Ctrl Pts',(30.8883310468311,34.1592140442528,46.3320445438389));
#23346=CARTESIAN_POINT('Ctrl Pts',(29.5830325841312,32.2372375623016,46.4431743330585));
#23347=CARTESIAN_POINT('Ctrl Pts',(30.4897164895143,30.0981438360661,46.5543041222784));
#23348=CARTESIAN_POINT('Ctrl Pts',(32.7785954853513,29.6996082462917,46.665433911498));
#23349=CARTESIAN_POINT('Ctrl Pts',(33.9595497672164,30.9782871886646,46.7486907772261));
#23350=CARTESIAN_POINT('Ctrl Pts',(34.0560088065047,31.8289754789177,46.7949043798808));
#23351=CARTESIAN_POINT('Ctrl Pts',(34.0544757475471,31.9981230672873,46.8040747194623));
#23352=CARTESIAN_POINT('Ctrl Pts',(34.0518959992412,31.9989927018737,46.0459252805377));
#23353=CARTESIAN_POINT('Ctrl Pts',(34.0500891674537,32.406351678701,46.0679402883943));
#23354=CARTESIAN_POINT('Ctrl Pts',(33.7353984216385,33.5017208160384,46.1269985593241));
#23355=CARTESIAN_POINT('Ctrl Pts',(31.9525944719365,34.4281198046771,46.2231000933271));
#23356=CARTESIAN_POINT('Ctrl Pts',(29.9343825704431,33.2771991640567,46.3342298825469));
#23357=CARTESIAN_POINT('Ctrl Pts',(29.806601339792,30.9573996991398,46.4453596717666));
#23358=CARTESIAN_POINT('Ctrl Pts',(31.6861947765452,29.5917767230407,46.5564894609864));
#23359=CARTESIAN_POINT('Ctrl Pts',(33.6396491688907,30.3475933797668,46.6566779972434));
#23360=CARTESIAN_POINT('Ctrl Pts',(34.0495579351968,31.5197595363103,46.7198232704272));
#23361=CARTESIAN_POINT('Ctrl Pts',(34.0535341854227,32.0017741341213,46.7459252805377));
#23362=CARTESIAN_POINT('Origin',(32.,32.,39.4540747194623));
#23363=CARTESIAN_POINT('',(34.0572107075264,31.9987715235836,45.3459252805377));
#23364=CARTESIAN_POINT('',(34.0525989138529,32.0014721641904,45.4040747194623));
#23365=CARTESIAN_POINT('',(34.05475,32.0000000000002,39.4540747194623));
#23366=CARTESIAN_POINT('Ctrl Pts',(34.0525989138529,32.0014721641904,45.4040747194623));
#23367=CARTESIAN_POINT('Ctrl Pts',(34.0541886765981,32.2413915617398,45.4170518896686));
#23368=CARTESIAN_POINT('Ctrl Pts',(33.9044077369096,33.1642376187088,45.4670723229481));
#23369=CARTESIAN_POINT('Ctrl Pts',(32.539107606757,34.3679898941243,45.5541360193008));
#23370=CARTESIAN_POINT('Ctrl Pts',(30.3030266273459,33.737323954489,45.6652658085205));
#23371=CARTESIAN_POINT('Ctrl Pts',(29.6199972756779,31.516677972199,45.7763955977403));
#23372=CARTESIAN_POINT('Ctrl Pts',(31.1151206072547,29.7383630683434,45.88752538696));
#23373=CARTESIAN_POINT('Ctrl Pts',(33.3805970136183,30.0248808040469,45.9967517608673));
#23374=CARTESIAN_POINT('Ctrl Pts',(34.055277690139,31.355282810549,46.0689348717015));
#23375=CARTESIAN_POINT('Ctrl Pts',(34.0579058799806,32.0006373862481,46.1040747194624));
#23376=CARTESIAN_POINT('Ctrl Pts',(34.0572107075264,31.9987715235836,45.3459252805377));
#23377=CARTESIAN_POINT('Ctrl Pts',(34.0529103877299,32.6070006388191,45.3790140432882));
#23378=CARTESIAN_POINT('Ctrl Pts',(33.4453451887035,33.9036142777098,45.4491460691119));
#23379=CARTESIAN_POINT('Ctrl Pts',(31.2413200135407,34.3070365727709,45.5563213580088));
#23380=CARTESIAN_POINT('Ctrl Pts',(29.6503075134721,32.6139692897129,45.6674511472286));
#23381=CARTESIAN_POINT('Ctrl Pts',(30.2097080957199,30.3590039709295,45.7785809364483));
#23382=CARTESIAN_POINT('Ctrl Pts',(32.4075644138576,29.6058604220904,45.889710725668));
#23383=CARTESIAN_POINT('Ctrl Pts',(33.8709146442334,30.7589476010144,45.9788255070311));
#23384=CARTESIAN_POINT('Ctrl Pts',(34.0531294091684,31.7209144605013,46.030897025321));
#23385=CARTESIAN_POINT('Ctrl Pts',(34.0518959992412,31.9989927018737,46.0459252805377));
#23386=CARTESIAN_POINT('Origin',(32.,32.,39.4540747194623));
#23387=CARTESIAN_POINT('',(34.0556201050794,32.0017900283843,44.6459252805377));
#23388=CARTESIAN_POINT('',(34.0525927448309,31.9985307397491,44.7040747194623));
#23389=CARTESIAN_POINT('',(34.05475,32.0000000000002,39.4540747194623));
#23390=CARTESIAN_POINT('Ctrl Pts',(34.0525927448309,31.9985307397491,44.7040747194623));
#23391=CARTESIAN_POINT('Ctrl Pts',(34.0496527769965,32.4431829229246,44.7281256445624));
#23392=CARTESIAN_POINT('Ctrl Pts',(33.6892909574588,33.5770300444085,44.7892198327358));
#23393=CARTESIAN_POINT('Ctrl Pts',(31.8196154283712,34.4218741826645,44.8873572839824));
#23394=CARTESIAN_POINT('Ctrl Pts',(29.8675010685907,33.1620935667478,44.9984870732022));
#23395=CARTESIAN_POINT('Ctrl Pts',(29.8670266048481,30.8387775209235,45.1096168624218));
#23396=CARTESIAN_POINT('Ctrl Pts',(31.8186262612152,29.5781996950166,45.2207466516417));
#23397=CARTESIAN_POINT('Ctrl Pts',(33.6889357232157,30.4224105767702,45.318899270655));
#23398=CARTESIAN_POINT('Ctrl Pts',(34.0496507073291,31.5565429222791,45.3800086265953));
#23399=CARTESIAN_POINT('Ctrl Pts',(34.0525989138529,32.0014721641904,45.4040747194623));
#23400=CARTESIAN_POINT('Ctrl Pts',(34.0556201050794,32.0017900283843,44.6459252805377));
#23401=CARTESIAN_POINT('Ctrl Pts',(34.0568192254344,32.1329178655474,44.6530445351088));
#23402=CARTESIAN_POINT('Ctrl Pts',(33.9856535075787,32.9450400768571,44.6972070527531));
#23403=CARTESIAN_POINT('Ctrl Pts',(32.9043976941981,34.2539028108345,44.7784128334707));
#23404=CARTESIAN_POINT('Ctrl Pts',(30.5970084349764,33.9823288673751,44.8895426226904));
#23405=CARTESIAN_POINT('Ctrl Pts',(29.5736218412549,31.8965490419561,45.0006724119102));
#23406=CARTESIAN_POINT('Ctrl Pts',(30.7708302254411,29.9054464114596,45.1118022011299));
#23407=CARTESIAN_POINT('Ctrl Pts',(33.0929614575128,29.8312565107077,45.2229319903496));
#23408=CARTESIAN_POINT('Ctrl Pts',(34.0212425543896,31.1729921114884,45.3009730168189));
#23409=CARTESIAN_POINT('Ctrl Pts',(34.0577246468402,31.9260809170879,45.3419707802149));
#23410=CARTESIAN_POINT('Ctrl Pts',(34.0572107075264,31.9987715235836,45.3459252805377));
#23411=CARTESIAN_POINT('Origin',(32.,32.,39.4540747194623));
#23412=CARTESIAN_POINT('',(34.0514132135286,32.0000997951266,43.9459252805377));
#23413=CARTESIAN_POINT('',(34.0579022039251,31.9993577749783,44.0040747194624));
#23414=CARTESIAN_POINT('',(34.05475,32.0000000000002,39.4540747194623));
#23415=CARTESIAN_POINT('Ctrl Pts',(34.0579022039251,31.9993577749783,44.0040747194624));
#23416=CARTESIAN_POINT('Ctrl Pts',(34.0552574969039,32.6444368624799,44.0391993994564));
#23417=CARTESIAN_POINT('Ctrl Pts',(33.3810890294814,33.9745950606643,44.1113673425235));
#23418=CARTESIAN_POINT('Ctrl Pts',(31.1160444164971,34.2619981602002,44.2205785486641));
#23419=CARTESIAN_POINT('Ctrl Pts',(29.6201948806291,32.4842940678484,44.3317083378838));
#23420=CARTESIAN_POINT('Ctrl Pts',(30.3023171820977,30.2633692965589,44.4428381271035));
#23421=CARTESIAN_POINT('Ctrl Pts',(32.5381403879069,29.6317901120796,44.5539679163233));
#23422=CARTESIAN_POINT('Ctrl Pts',(33.9041700015856,30.8351942625182,44.6410467804428));
#23423=CARTESIAN_POINT('Ctrl Pts',(34.0541809189064,31.7583291084085,44.6910823814892));
#23424=CARTESIAN_POINT('Ctrl Pts',(34.0525927448309,31.9985307397491,44.7040747194623));
#23425=CARTESIAN_POINT('Ctrl Pts',(34.0514132135286,32.0000997951266,43.9459252805377));
#23426=CARTESIAN_POINT('Ctrl Pts',(34.0515591633093,32.3369356418003,43.9641182900027));
#23427=CARTESIAN_POINT('Ctrl Pts',(33.8137553478573,33.359417696568,44.0193545625409));
#23428=CARTESIAN_POINT('Ctrl Pts',(32.2023029113298,34.4201418557892,44.1116340981523));
#23429=CARTESIAN_POINT('Ctrl Pts',(30.0765281914199,33.4826561541886,44.2227638873721));
#23430=CARTESIAN_POINT('Ctrl Pts',(29.7110940115711,31.1882596190528,44.3338936765918));
#23431=CARTESIAN_POINT('Ctrl Pts',(31.4404417701646,29.6367590775809,44.4450234658115));
#23432=CARTESIAN_POINT('Ctrl Pts',(33.5382982520961,30.2089088165319,44.5490340004602));
#23433=CARTESIAN_POINT('Ctrl Pts',(34.0505799021566,31.4506269150344,44.6160012720355));
#23434=CARTESIAN_POINT('Ctrl Pts',(34.0556201050794,32.0017900283843,44.6459252805377));
#23435=CARTESIAN_POINT('Origin',(32.,32.,39.4540747194623));
#23436=CARTESIAN_POINT('',(34.0552538748384,31.9981575528908,43.2459252805377));
#23437=CARTESIAN_POINT('',(34.0544841229652,32.0018771151024,43.3040747194623));
#23438=CARTESIAN_POINT('',(34.05475,32.0000000000002,39.4540747194623));
#23439=CARTESIAN_POINT('Ctrl Pts',(34.0544841229652,32.0018771151024,43.3040747194623));
#23440=CARTESIAN_POINT('Ctrl Pts',(34.0560153379072,32.1707431770014,43.313229891277));
#23441=CARTESIAN_POINT('Ctrl Pts',(33.9597518572347,33.021145412764,43.3594283261648));
#23442=CARTESIAN_POINT('Ctrl Pts',(32.7795349847121,34.3000735544458,43.442670024126));
#23443=CARTESIAN_POINT('Ctrl Pts',(30.490493403277,33.9024728606777,43.5537998133457));
#23444=CARTESIAN_POINT('Ctrl Pts',(29.5829358892083,31.763749635471,43.6649296025654));
#23445=CARTESIAN_POINT('Ctrl Pts',(30.887449237386,29.8412401822595,43.7760593917852));
#23446=CARTESIAN_POINT('Ctrl Pts',(33.2101569783881,29.8944043032633,43.8871891810048));
#23447=CARTESIAN_POINT('Ctrl Pts',(34.0412598208513,31.2487125032873,43.9631942902306));
#23448=CARTESIAN_POINT('Ctrl Pts',(34.0580466633235,31.9641222134796,44.0021561363831));
#23449=CARTESIAN_POINT('Ctrl Pts',(34.0579022039251,31.9993577749783,44.0040747194624));
#23450=CARTESIAN_POINT('Ctrl Pts',(34.0552538748384,31.9981575528908,43.2459252805377));
#23451=CARTESIAN_POINT('Ctrl Pts',(34.0502763874237,32.5374622262668,43.2751920448965));
#23452=CARTESIAN_POINT('Ctrl Pts',(33.5565644973773,33.767436404629,43.3415020723287));
#23453=CARTESIAN_POINT('Ctrl Pts',(31.4823523987704,34.3727734903307,43.444855362834));
#23454=CARTESIAN_POINT('Ctrl Pts',(29.7258180926964,32.8521207213123,43.5559851520537));
#23455=CARTESIAN_POINT('Ctrl Pts',(30.0505904076267,30.5516163115282,43.6671149412734));
#23456=CARTESIAN_POINT('Ctrl Pts',(32.1594412400625,29.576656945096,43.7782447304932));
#23457=CARTESIAN_POINT('Ctrl Pts',(33.801022445043,30.6160471338321,43.8711815102479));
#23458=CARTESIAN_POINT('Ctrl Pts',(34.0512619911382,31.6510953521632,43.9270750269294));
#23459=CARTESIAN_POINT('Ctrl Pts',(34.0514132135286,32.0000997951266,43.9459252805377));
#23460=CARTESIAN_POINT('Origin',(32.,32.,39.4540747194623));
#23461=CARTESIAN_POINT('',(34.0574729334528,32.0010548525921,42.5459252805377));
#23462=CARTESIAN_POINT('',(34.0515269670353,31.9994876359477,42.6040747194623));
#23463=CARTESIAN_POINT('',(34.05475,32.0000000000002,39.4540747194623));
#23464=CARTESIAN_POINT('Ctrl Pts',(34.0515269670353,31.9994876359477,42.6040747194623));
#23465=CARTESIAN_POINT('Ctrl Pts',(34.0506912299639,32.3739658294889,42.6243036461709));
#23466=CARTESIAN_POINT('Ctrl Pts',(33.7733218574882,33.4353422112672,42.6815758359526));
#23467=CARTESIAN_POINT('Ctrl Pts',(32.0693858609145,34.4275911150555,42.7758912888076));
#23468=CARTESIAN_POINT('Ctrl Pts',(29.9981749928738,33.3750308454857,42.8870210780274));
#23469=CARTESIAN_POINT('Ctrl Pts',(29.7590126602339,31.0640572092229,42.9981508672471));
#23470=CARTESIAN_POINT('Ctrl Pts',(31.5707776395802,29.6096482896975,43.1092806564668));
#23471=CARTESIAN_POINT('Ctrl Pts',(33.5937426392217,30.2824590886342,43.2112552738719));
#23472=CARTESIAN_POINT('Ctrl Pts',(34.0498198017591,31.487484568456,43.2761866282037));
#23473=CARTESIAN_POINT('Ctrl Pts',(34.0544841229652,32.0018771151024,43.3040747194623));
#23474=CARTESIAN_POINT('Ctrl Pts',(34.0574729334528,32.0010548525921,42.5459252805377));
#23475=CARTESIAN_POINT('Ctrl Pts',(34.0578522481403,32.0616438352948,42.5492225367172));
#23476=CARTESIAN_POINT('Ctrl Pts',(34.0279453790661,32.8025443861859,42.5895630559699));
#23477=CARTESIAN_POINT('Ctrl Pts',(33.1311710776567,34.1490612048519,42.6669468382959));
#23478=CARTESIAN_POINT('Ctrl Pts',(30.8080907428172,34.1159786377566,42.7780766275156));
#23479=CARTESIAN_POINT('Ctrl Pts',(29.5758326061327,32.1463750685223,42.8892064167354));
#23480=CARTESIAN_POINT('Ctrl Pts',(30.5621462946373,30.0428107753347,43.0003362059551));
#23481=CARTESIAN_POINT('Ctrl Pts',(32.8643680431626,29.7304447592571,43.1114659951748));
#23482=CARTESIAN_POINT('Ctrl Pts',(33.9775551897302,31.0304040426633,43.1933290200357));
#23483=CARTESIAN_POINT('Ctrl Pts',(34.05657644757,31.8548584150789,43.2381487818233));
#23484=CARTESIAN_POINT('Ctrl Pts',(34.0552538748384,31.9981575528908,43.2459252805377));
#23485=CARTESIAN_POINT('Origin',(32.,32.,39.4540747194623));
#23486=CARTESIAN_POINT('',(34.0520872716434,32.0011660295939,41.8459252805377));
#23487=CARTESIAN_POINT('',(34.0563620767522,31.9983919833491,41.9040747194623));
#23488=CARTESIAN_POINT('',(34.05475,32.0000000000002,39.4540747194623));
#23489=CARTESIAN_POINT('Ctrl Pts',(34.0563620767522,31.9983919833491,41.9040747194623));
#23490=CARTESIAN_POINT('Ctrl Pts',(34.0514108779685,32.574410111975,41.9353774010647));
#23491=CARTESIAN_POINT('Ctrl Pts',(33.4988294551637,33.8404093508007,42.0037233457404));
#23492=CARTESIAN_POINT('Ctrl Pts',(31.3531125056534,34.3408422066741,42.1091125534892));
#23493=CARTESIAN_POINT('Ctrl Pts',(29.6825424018648,32.7262261662198,42.220242342709));
#23494=CARTESIAN_POINT('Ctrl Pts',(30.1328842256904,30.4469728946945,42.3313721319287));
#23495=CARTESIAN_POINT('Ctrl Pts',(32.2919902260347,29.5890346627002,42.4425019211484));
#23496=CARTESIAN_POINT('Ctrl Pts',(33.8394915366755,30.6921087455261,42.5334027836596));
#23497=CARTESIAN_POINT('Ctrl Pts',(34.0522216338574,31.6882203898806,42.5872603830976));
#23498=CARTESIAN_POINT('Ctrl Pts',(34.0515269670353,31.9994876359477,42.6040747194623));
#23499=CARTESIAN_POINT('Ctrl Pts',(34.0520872716434,32.0011660295939,41.8459252805377));
#23500=CARTESIAN_POINT('Ctrl Pts',(34.0534688437858,32.267023360204,41.860296291611));
#23501=CARTESIAN_POINT('Ctrl Pts',(33.8819549930642,33.2164555944441,41.9117105657577));
#23502=CARTESIAN_POINT('Ctrl Pts',(32.4498627820811,34.3865418359406,42.0001681029776));
#23503=CARTESIAN_POINT('Ctrl Pts',(30.2390335296879,33.6724274291408,42.1112978921972));
#23504=CARTESIAN_POINT('Ctrl Pts',(29.6398079512964,31.4277075354308,42.222427681417));
#23505=CARTESIAN_POINT('Ctrl Pts',(31.2006114825729,29.706752611882,42.3335574706367));
#23506=CARTESIAN_POINT('Ctrl Pts',(33.4249872180097,30.0733389095352,42.4413900036769));
#23507=CARTESIAN_POINT('Ctrl Pts',(34.053590809844,31.3809525260924,42.5121792736439));
#23508=CARTESIAN_POINT('Ctrl Pts',(34.0574729334528,32.0010548525921,42.5459252805377));
#23509=CARTESIAN_POINT('Origin',(32.,32.,39.4540747194623));
#23510=CARTESIAN_POINT('',(34.052676219088,31.9976391197374,41.1459252805377));
#23511=CARTESIAN_POINT('',(34.0565678449602,32.0014926321758,41.2040747194623));
#23512=CARTESIAN_POINT('',(34.05475,32.0000000000002,39.4540747194623));
#23513=CARTESIAN_POINT('',(32.5301702171886,30.0148256743283,41.));
#23514=CARTESIAN_POINT('Ctrl Pts',(32.5301702171886,30.0148256743283,41.));
#23515=CARTESIAN_POINT('Ctrl Pts',(33.1902397907527,30.1911070339301,41.0370432630732));
#23516=CARTESIAN_POINT('Ctrl Pts',(33.9249253440543,30.8871227497852,41.0856850232525));
#23517=CARTESIAN_POINT('Ctrl Pts',(34.0542945901694,31.7833429360997,41.1343267834317));
#23518=CARTESIAN_POINT('Ctrl Pts',(34.052676219088,31.9976391197375,41.1459252805377));
#23519=CARTESIAN_POINT('',(31.4686977725381,30.0112667465652,41.));
#23520=CARTESIAN_POINT('Origin',(32.,32.,41.));
#23521=CARTESIAN_POINT('Ctrl Pts',(31.4686971487471,30.0112647854283,41.));
#23522=CARTESIAN_POINT('Ctrl Pts',(32.1131668553171,29.8399814440384,41.0363148168372));
#23523=CARTESIAN_POINT('Ctrl Pts',(33.4928785396173,30.1592359611441,41.1043397233247));
#23524=CARTESIAN_POINT('Ctrl Pts',(34.0517137697956,31.4182664393509,41.1723646298121));
#23525=CARTESIAN_POINT('Ctrl Pts',(34.0565678449602,32.0014926321758,41.2040747194623));
#23526=CARTESIAN_POINT('Origin',(-32.,32.,48.));
#23527=CARTESIAN_POINT('',(-30.3315194671681,32.0006140847627,53.3285196366098));
#23528=CARTESIAN_POINT('',(-30.335188098255,32.0014849307108,53.5214803633902));
#23529=CARTESIAN_POINT('',(-30.334,32.,48.));
#23530=CARTESIAN_POINT('',(-32.6750771856749,30.4769022377466,54.));
#23531=CARTESIAN_POINT('Ctrl Pts',(-30.335188098255,32.0014849307108,53.5214803633902));
#23532=CARTESIAN_POINT('Ctrl Pts',(-30.3338369653803,32.1712283781921,53.5328138566338));
#23533=CARTESIAN_POINT('Ctrl Pts',(-30.3577131720504,32.3405890855005,53.5441473498775));
#23534=CARTESIAN_POINT('Ctrl Pts',(-30.4083948673629,32.5014829194567,53.5554808431211));
#23535=CARTESIAN_POINT('Ctrl Pts',(-30.5740468276277,33.027360730471,53.5925241061943));
#23536=CARTESIAN_POINT('Ctrl Pts',(-31.0260602822948,33.4627874201365,53.6295673692676));
#23537=CARTESIAN_POINT('Ctrl Pts',(-31.5578576126045,33.6090004762337,53.6666106323408));
#23538=CARTESIAN_POINT('Ctrl Pts',(-32.0896549429143,33.755213532331,53.7036538954141));
#23539=CARTESIAN_POINT('Ctrl Pts',(-32.7012361488668,33.61221295486,53.7406971584873));
#23540=CARTESIAN_POINT('Ctrl Pts',(-33.112224935063,33.2444451932609,53.7777404215606));
#23541=CARTESIAN_POINT('Ctrl Pts',(-33.5232137212592,32.8766774316618,53.8147836846338));
#23542=CARTESIAN_POINT('Ctrl Pts',(-33.7336100876993,32.2841424859346,53.851826947707));
#23543=CARTESIAN_POINT('Ctrl Pts',(-33.6481832846338,31.7403144028754,53.8888702107803));
#23544=CARTESIAN_POINT('Ctrl Pts',(-33.5627564815683,31.1964863198163,53.9259134738535));
#23545=CARTESIAN_POINT('Ctrl Pts',(-33.1815065089974,30.7013650994253,53.9629567369268));
#23546=CARTESIAN_POINT('Ctrl Pts',(-32.6750771856749,30.4769022377466,54.));
#23547=CARTESIAN_POINT('',(-30.334,32.,54.));
#23548=CARTESIAN_POINT('Origin',(-32.,32.,54.));
#23549=CARTESIAN_POINT('',(-30.334,32.,55.));
#23550=CARTESIAN_POINT('',(-30.334,32.,48.));
#23551=CARTESIAN_POINT('Origin',(-32.,32.,55.));
#23552=CARTESIAN_POINT('',(-30.3853283554254,31.5775322576866,54.));
#23553=CARTESIAN_POINT('Origin',(-32.,32.,54.));
#23554=CARTESIAN_POINT('Ctrl Pts',(-30.3853267261146,31.5775319120267,54.));
#23555=CARTESIAN_POINT('Ctrl Pts',(-30.5228595194004,31.054637565178,53.9636851831627));
#23556=CARTESIAN_POINT('Ctrl Pts',(-30.9381524315377,30.6037762063905,53.9273703663255));
#23557=CARTESIAN_POINT('Ctrl Pts',(-31.4484748501057,30.4251375769901,53.8910555494883));
#23558=CARTESIAN_POINT('Ctrl Pts',(-31.969033929005,30.2429155992892,53.8540122864151));
#23559=CARTESIAN_POINT('Ctrl Pts',(-32.5884731835828,30.343947026941,53.8169690233418));
#23560=CARTESIAN_POINT('Ctrl Pts',(-33.0238322854568,30.6822522289001,53.7799257602686));
#23561=CARTESIAN_POINT('Ctrl Pts',(-33.4591913873308,31.0205574308592,53.7428824971953));
#23562=CARTESIAN_POINT('Ctrl Pts',(-33.7104703365009,31.5961364071255,53.7058392341221));
#23563=CARTESIAN_POINT('Ctrl Pts',(-33.6624375910167,32.145481024569,53.6687959710488));
#23564=CARTESIAN_POINT('Ctrl Pts',(-33.6144048455325,32.6948256420124,53.6317527079756));
#23565=CARTESIAN_POINT('Ctrl Pts',(-33.267060405394,33.2179359006329,53.5947094449024));
#23566=CARTESIAN_POINT('Ctrl Pts',(-32.7794722527579,33.4755031203564,53.5576661818291));
#23567=CARTESIAN_POINT('Ctrl Pts',(-32.2918841001217,33.7330703400798,53.5206229187559));
#23568=CARTESIAN_POINT('Ctrl Pts',(-31.6640522349879,33.7250945209062,53.4835796556826));
#23569=CARTESIAN_POINT('Ctrl Pts',(-31.1832059468561,33.4551931614016,53.4465363926094));
#23570=CARTESIAN_POINT('Ctrl Pts',(-30.7023596587244,33.1852918018969,53.4094931295361));
#23571=CARTESIAN_POINT('Ctrl Pts',(-30.3684989475947,32.6534649020614,53.3724498664629));
#23572=CARTESIAN_POINT('Ctrl Pts',(-30.3344285753632,32.1030898303843,53.3354066033897));
#23573=CARTESIAN_POINT('Ctrl Pts',(-30.3323171566033,32.0689818305247,53.3331109477964));
#23574=CARTESIAN_POINT('Ctrl Pts',(-30.3313571017956,32.0348025952259,53.3308152922031));
#23575=CARTESIAN_POINT('Ctrl Pts',(-30.3315194671681,32.0006140847627,53.3285196366098));
#23576=CARTESIAN_POINT('Origin',(-32.,32.,48.));
#23577=CARTESIAN_POINT('',(-30.3358699394038,32.0011304355222,52.6285196366098));
#23578=CARTESIAN_POINT('',(-30.3362229430458,31.9991035479857,52.8214803633902));
#23579=CARTESIAN_POINT('',(-30.334,32.,48.));
#23580=CARTESIAN_POINT('Ctrl Pts',(-30.3362229430458,31.9991035479857,52.8214803633902));
#23581=CARTESIAN_POINT('Ctrl Pts',(-30.3378663531425,32.3352311359495,52.8438876115277));
#23582=CARTESIAN_POINT('Ctrl Pts',(-30.4366434498682,32.6722466504923,52.8662948596652));
#23583=CARTESIAN_POINT('Ctrl Pts',(-30.6259117277904,32.9469019296561,52.8887021078027));
#23584=CARTESIAN_POINT('Ctrl Pts',(-30.9388066699745,33.400957139742,52.925745370876));
#23585=CARTESIAN_POINT('Ctrl Pts',(-31.4990150314079,33.6845811229079,52.9627886339492));
#23586=CARTESIAN_POINT('Ctrl Pts',(-32.0501928386486,33.6679971146088,52.9998318970225));
#23587=CARTESIAN_POINT('Ctrl Pts',(-32.6013706458894,33.6514131063097,53.0368751600957));
#23588=CARTESIAN_POINT('Ctrl Pts',(-33.1435178989375,33.3346211065456,53.0739184231689));
#23589=CARTESIAN_POINT('Ctrl Pts',(-33.4285423718774,32.862567514634,53.1109616862422));
#23590=CARTESIAN_POINT('Ctrl Pts',(-33.7135668448172,32.3905139227225,53.1480049493154));
#23591=CARTESIAN_POINT('Ctrl Pts',(-33.7414685376489,31.7631987386633,53.1850482123887));
#23592=CARTESIAN_POINT('Ctrl Pts',(-33.4994967785869,31.2677094716929,53.222091475462));
#23593=CARTESIAN_POINT('Ctrl Pts',(-33.2575250195249,30.7722202047225,53.2591347385352));
#23594=CARTESIAN_POINT('Ctrl Pts',(-32.7456798085692,30.4085568548408,53.2961780016084));
#23595=CARTESIAN_POINT('Ctrl Pts',(-32.1981450993846,30.3430674696929,53.3332212646816));
#23596=CARTESIAN_POINT('Ctrl Pts',(-31.6506103901999,30.2775780845449,53.3702645277548));
#23597=CARTESIAN_POINT('Ctrl Pts',(-31.0673861827863,30.5102626641308,53.4073077908281));
#23598=CARTESIAN_POINT('Ctrl Pts',(-30.7154193120108,30.9347694201052,53.4443510539014));
#23599=CARTESIAN_POINT('Ctrl Pts',(-30.4711377211209,31.2293971089682,53.470060823731));
#23600=CARTESIAN_POINT('Ctrl Pts',(-30.3382531122335,31.6164258080716,53.4957705935606));
#23601=CARTESIAN_POINT('Ctrl Pts',(-30.335188098255,32.0014849307108,53.5214803633902));
#23602=CARTESIAN_POINT('Ctrl Pts',(-30.3315194671681,32.0006140847627,53.3285196366098));
#23603=CARTESIAN_POINT('Ctrl Pts',(-30.3339770693666,31.4831283846537,53.2937720291299));
#23604=CARTESIAN_POINT('Ctrl Pts',(-30.5935878007645,30.9635176892697,53.2590244216499));
#23605=CARTESIAN_POINT('Ctrl Pts',(-31.0099803387083,30.6566480755526,53.2242768141699));
#23606=CARTESIAN_POINT('Ctrl Pts',(-31.4538825076184,30.3295046359168,53.1872335510967));
#23607=CARTESIAN_POINT('Ctrl Pts',(-32.0759668787719,30.2441410001639,53.1501902880235));
#23608=CARTESIAN_POINT('Ctrl Pts',(-32.5915791609355,30.4396232555466,53.1131470249502));
#23609=CARTESIAN_POINT('Ctrl Pts',(-33.1071914430991,30.6351055109293,53.076103761877));
#23610=CARTESIAN_POINT('Ctrl Pts',(-33.5163316362729,31.1114336574476,53.0390604988037));
#23611=CARTESIAN_POINT('Ctrl Pts',(-33.6317752923808,31.6506404213303,53.0020172357305));
#23612=CARTESIAN_POINT('Ctrl Pts',(-33.7472189484887,32.1898471852129,52.9649739726572));
#23613=CARTESIAN_POINT('Ctrl Pts',(-33.5689660675308,32.7919325664598,52.927930709584));
#23614=CARTESIAN_POINT('Ctrl Pts',(-33.1785862796925,33.1813866185031,52.8908874465107));
#23615=CARTESIAN_POINT('Ctrl Pts',(-32.7882064918542,33.5708406705464,52.8538441834375));
#23616=CARTESIAN_POINT('Ctrl Pts',(-32.1856997971356,33.7476633933861,52.8168009203643));
#23617=CARTESIAN_POINT('Ctrl Pts',(-31.6467689421153,33.6309411327337,52.779757657291));
#23618=CARTESIAN_POINT('Ctrl Pts',(-31.1078380870949,33.5142188720812,52.7427143942178));
#23619=CARTESIAN_POINT('Ctrl Pts',(-30.6324830717728,33.1039516279366,52.7056711311445));
#23620=CARTESIAN_POINT('Ctrl Pts',(-30.4382243040802,32.5878757369611,52.6686278680713));
#23621=CARTESIAN_POINT('Ctrl Pts',(-30.3681137093176,32.4016170260225,52.6552584575841));
#23622=CARTESIAN_POINT('Ctrl Pts',(-30.3346182876945,32.2015758403761,52.641889047097));
#23623=CARTESIAN_POINT('Ctrl Pts',(-30.3358699394038,32.0011304355222,52.6285196366098));
#23624=CARTESIAN_POINT('Origin',(-32.,32.,48.));
#23625=CARTESIAN_POINT('',(-30.3356164568928,31.9987501844668,51.9285196366098));
#23626=CARTESIAN_POINT('',(-30.3318747561565,31.9990863473369,52.1214803633902));
#23627=CARTESIAN_POINT('',(-30.334,32.,48.));
#23628=CARTESIAN_POINT('Ctrl Pts',(-30.3318747561565,31.9990863473369,52.1214803633902));
#23629=CARTESIAN_POINT('Ctrl Pts',(-30.3351692730374,32.4979846805671,52.1549613664216));
#23630=CARTESIAN_POINT('Ctrl Pts',(-30.573848791373,32.9996174235339,52.188442369453));
#23631=CARTESIAN_POINT('Ctrl Pts',(-30.9647448495809,33.3088117421955,52.2219233724844));
#23632=CARTESIAN_POINT('Ctrl Pts',(-31.3972308627662,33.6509032403563,52.2589666355576));
#23633=CARTESIAN_POINT('Ctrl Pts',(-32.0160471389214,33.7574283392523,52.2960098986309));
#23634=CARTESIAN_POINT('Ctrl Pts',(-32.5380267774666,33.5796418646352,52.3330531617041));
#23635=CARTESIAN_POINT('Ctrl Pts',(-33.0600064160119,33.4018553900181,52.3700964247773));
#23636=CARTESIAN_POINT('Ctrl Pts',(-33.4851494169471,32.939757341888,52.4071396878506));
#23637=CARTESIAN_POINT('Ctrl Pts',(-33.6189125057485,32.4048010173491,52.4441829509238));
#23638=CARTESIAN_POINT('Ctrl Pts',(-33.7526755945498,31.8698446928101,52.4812262139971));
#23639=CARTESIAN_POINT('Ctrl Pts',(-33.5950587712171,31.2620300918623,52.5182694770703));
#23640=CARTESIAN_POINT('Ctrl Pts',(-33.2181869216583,30.8594904030147,52.5553127401436));
#23641=CARTESIAN_POINT('Ctrl Pts',(-32.8413150720994,30.4569507141672,52.5923560032168));
#23642=CARTESIAN_POINT('Ctrl Pts',(-32.2451881963143,30.2596859374199,52.62939926629));
#23643=CARTESIAN_POINT('Ctrl Pts',(-31.702590161623,30.3579623298606,52.6664425293633));
#23644=CARTESIAN_POINT('Ctrl Pts',(-31.1599921269317,30.4562387223013,52.7034857924365));
#23645=CARTESIAN_POINT('Ctrl Pts',(-30.6709229333342,30.85005628393,52.7405290555098));
#23646=CARTESIAN_POINT('Ctrl Pts',(-30.4591790980028,31.3592082832473,52.777572318583));
#23647=CARTESIAN_POINT('Ctrl Pts',(-30.3755178414248,31.5603772853363,52.7922083335188));
#23648=CARTESIAN_POINT('Ctrl Pts',(-30.3351494968746,31.7795510010796,52.8068443484545));
#23649=CARTESIAN_POINT('Ctrl Pts',(-30.3362229430458,31.9991035479857,52.8214803633902));
#23650=CARTESIAN_POINT('Ctrl Pts',(-30.3358699394038,32.0011304355222,52.6285196366098));
#23651=CARTESIAN_POINT('Ctrl Pts',(-30.3380862987625,31.6461922001661,52.6048457840237));
#23652=CARTESIAN_POINT('Ctrl Pts',(-30.4492537515405,31.289986516348,52.5811719314377));
#23653=CARTESIAN_POINT('Ctrl Pts',(-30.6590001159673,31.0067929794516,52.5574980788516));
#23654=CARTESIAN_POINT('Ctrl Pts',(-30.9871972156101,30.5636706507241,52.5204548157783));
#23655=CARTESIAN_POINT('Ctrl Pts',(-31.5567539349585,30.2993105310754,52.4834115527051));
#23656=CARTESIAN_POINT('Ctrl Pts',(-32.1070443429008,30.3346824468124,52.4463682896318));
#23657=CARTESIAN_POINT('Ctrl Pts',(-32.657334750843,30.3700543625495,52.4093250265586));
#23658=CARTESIAN_POINT('Ctrl Pts',(-33.1883588473791,30.7051583136722,52.3722817634854));
#23659=CARTESIAN_POINT('Ctrl Pts',(-33.4571228169063,31.1866525143206,52.3352385004121));
#23660=CARTESIAN_POINT('Ctrl Pts',(-33.7258867864335,31.668146714969,52.2981952373389));
#23661=CARTESIAN_POINT('Ctrl Pts',(-33.7323906289517,32.2960311651429,52.2611519742656));
#23662=CARTESIAN_POINT('Ctrl Pts',(-33.4736582559377,32.7829893626111,52.2241087111924));
#23663=CARTESIAN_POINT('Ctrl Pts',(-33.2149258829237,33.2699475600792,52.1870654481191));
#23664=CARTESIAN_POINT('Ctrl Pts',(-32.6909572943775,33.6159795048416,52.1500221850459));
#23665=CARTESIAN_POINT('Ctrl Pts',(-32.1415176578637,33.6627428463605,52.1129789219727));
#23666=CARTESIAN_POINT('Ctrl Pts',(-31.5920780213499,33.7095061878793,52.0759356588994));
#23667=CARTESIAN_POINT('Ctrl Pts',(-31.0171673368685,33.4570009261547,52.0388923958262));
#23668=CARTESIAN_POINT('Ctrl Pts',(-30.6798616251316,33.0207721042924,52.0018491327529));
#23669=CARTESIAN_POINT('Ctrl Pts',(-30.4572889192754,32.7329245349333,51.9774059673719));
#23670=CARTESIAN_POINT('Ctrl Pts',(-30.3381713232652,32.3650822547069,51.9529628019909));
#23671=CARTESIAN_POINT('Ctrl Pts',(-30.3356164568928,31.9987501844668,51.9285196366098));
#23672=CARTESIAN_POINT('Origin',(-32.,32.,48.));
#23673=CARTESIAN_POINT('',(-30.3313738111782,31.9995820848862,51.2285196366098));
#23674=CARTESIAN_POINT('',(-30.3334713021565,32.0014789858971,51.4214803633902));
#23675=CARTESIAN_POINT('',(-30.334,32.,48.));
#23676=CARTESIAN_POINT('Ctrl Pts',(-30.3334713021565,32.0014789858971,51.4214803633902));
#23677=CARTESIAN_POINT('Ctrl Pts',(-30.3324380493541,32.1136863614967,51.4289918582422));
#23678=CARTESIAN_POINT('Ctrl Pts',(-30.3428029813185,32.22570392951,51.4365033530943));
#23679=CARTESIAN_POINT('Ctrl Pts',(-30.3652660205241,32.3352404972475,51.4440148479463));
#23680=CARTESIAN_POINT('Ctrl Pts',(-30.4760434738951,32.8754248380169,51.4810581110195));
#23681=CARTESIAN_POINT('Ctrl Pts',(-30.8810483542085,33.3552709529063,51.5181013740927));
#23682=CARTESIAN_POINT('Ctrl Pts',(-31.3949526236766,33.5552038604804,51.555144637166));
#23683=CARTESIAN_POINT('Ctrl Pts',(-31.9088568931446,33.7551367680545,51.5921879002392));
#23684=CARTESIAN_POINT('Ctrl Pts',(-32.5316605517672,33.6751564683133,51.6292311633125));
#23685=CARTESIAN_POINT('Ctrl Pts',(-32.9783720235667,33.3518615149587,51.6662744263858));
#23686=CARTESIAN_POINT('Ctrl Pts',(-33.4250834953661,33.0285665616042,51.703317689459));
#23687=CARTESIAN_POINT('Ctrl Pts',(-33.6957027803424,32.4619569546363,51.7403609525322));
#23688=CARTESIAN_POINT('Ctrl Pts',(-33.666395958695,31.9113101735047,51.7774042156054));
#23689=CARTESIAN_POINT('Ctrl Pts',(-33.6370891370477,31.3606633923732,51.8144474786787));
#23690=CARTESIAN_POINT('Ctrl Pts',(-33.3078562087767,30.8259794370781,51.851490741752));
#23691=CARTESIAN_POINT('Ctrl Pts',(-32.8293523813543,30.5519267950428,51.8885340048252));
#23692=CARTESIAN_POINT('Ctrl Pts',(-32.350848553932,30.2778741530076,51.9255772678985));
#23693=CARTESIAN_POINT('Ctrl Pts',(-31.7230738273582,30.2644528242322,51.9626205309717));
#23694=CARTESIAN_POINT('Ctrl Pts',(-31.233294503268,30.5178043187989,51.9996637940449));
#23695=CARTESIAN_POINT('Ctrl Pts',(-30.7435151791779,30.7711558133657,52.0367070571181));
#23696=CARTESIAN_POINT('Ctrl Pts',(-30.3917312575714,31.2912801312746,52.0737503201914));
#23697=CARTESIAN_POINT('Ctrl Pts',(-30.3389171718758,31.8401712389419,52.1107935832646));
#23698=CARTESIAN_POINT('Ctrl Pts',(-30.3338383129549,31.8929552730132,52.1143558433065));
#23699=CARTESIAN_POINT('Ctrl Pts',(-30.3315242312385,31.9460053331347,52.1179181033484));
#23700=CARTESIAN_POINT('Ctrl Pts',(-30.3318747561565,31.9990863473369,52.1214803633902));
#23701=CARTESIAN_POINT('Ctrl Pts',(-30.3356164568928,31.9987501844668,51.9285196366098));
#23702=CARTESIAN_POINT('Ctrl Pts',(-30.3342994602853,31.8099113086153,51.9159195389176));
#23703=CARTESIAN_POINT('Ctrl Pts',(-30.3639561318528,31.6214737337898,51.9033194412254));
#23704=CARTESIAN_POINT('Ctrl Pts',(-30.4263819212587,31.4446018044738,51.8907193435332));
#23705=CARTESIAN_POINT('Ctrl Pts',(-30.609908668115,30.9246127085175,51.85367608046));
#23706=CARTESIAN_POINT('Ctrl Pts',(-31.0766629008198,30.5045868986048,51.8166328173867));
#23707=CARTESIAN_POINT('Ctrl Pts',(-31.613060415607,30.3767259090036,51.7795895543135));
#23708=CARTESIAN_POINT('Ctrl Pts',(-32.1494579303943,30.2488649194023,51.7425462912402));
#23709=CARTESIAN_POINT('Ctrl Pts',(-32.7554987272639,30.4131687501125,51.705503028167));
#23710=CARTESIAN_POINT('Ctrl Pts',(-33.1538618225511,30.7944528585221,51.6684597650938));
#23711=CARTESIAN_POINT('Ctrl Pts',(-33.5522249178383,31.1757369669317,51.6314165020206));
#23712=CARTESIAN_POINT('Ctrl Pts',(-33.742910311543,31.7740013530409,51.5943732389473));
#23713=CARTESIAN_POINT('Ctrl Pts',(-33.6386614020287,32.3154834780122,51.557329975874));
#23714=CARTESIAN_POINT('Ctrl Pts',(-33.5344124925144,32.8569656029835,51.5202867128008));
#23715=CARTESIAN_POINT('Ctrl Pts',(-33.1352292797811,33.341665466817,51.4832434497276));
#23716=CARTESIAN_POINT('Ctrl Pts',(-32.6237758372046,33.5477870398502,51.4462001866543));
#23717=CARTESIAN_POINT('Ctrl Pts',(-32.1123223946281,33.7539086128834,51.4091569235811));
#23718=CARTESIAN_POINT('Ctrl Pts',(-31.4885987222084,33.6814518951163,51.3721136605078));
#23719=CARTESIAN_POINT('Ctrl Pts',(-31.0380173905906,33.3635726877936,51.3350703974346));
#23720=CARTESIAN_POINT('Ctrl Pts',(-30.6060019603948,33.0587914799067,51.2995534771596));
#23721=CARTESIAN_POINT('Ctrl Pts',(-30.3331544035574,32.5283960429641,51.2640365568847));
#23722=CARTESIAN_POINT('Ctrl Pts',(-30.3313738111782,31.9995820848862,51.2285196366098));
#23723=CARTESIAN_POINT('Origin',(-32.,32.,48.));
#23724=CARTESIAN_POINT('',(-30.3343902510906,32.0015149949486,50.5285196366098));
#23725=CARTESIAN_POINT('',(-30.3367088771406,31.9999843288602,50.7214803633902));
#23726=CARTESIAN_POINT('',(-30.334,32.,48.));
#23727=CARTESIAN_POINT('Ctrl Pts',(-30.3367088771406,31.9999843288602,50.7214803633902));
#23728=CARTESIAN_POINT('Ctrl Pts',(-30.3367322875339,32.2789818929087,50.7400656131361));
#23729=CARTESIAN_POINT('Ctrl Pts',(-30.4031501600345,32.5579899313227,50.758650862882));
#23730=CARTESIAN_POINT('Ctrl Pts',(-30.5359003296719,32.800720631568,50.777236112628));
#23731=CARTESIAN_POINT('Ctrl Pts',(-30.8004918484369,33.2845202741914,50.8142793757012));
#23732=CARTESIAN_POINT('Ctrl Pts',(-31.328599195375,33.624202296529,50.8513226387744));
#23733=CARTESIAN_POINT('Ctrl Pts',(-31.8785633120601,33.6643300469896,50.8883659018476));
#23734=CARTESIAN_POINT('Ctrl Pts',(-32.4285274287452,33.7044577974502,50.9254091649209));
#23735=CARTESIAN_POINT('Ctrl Pts',(-33.0003483151774,33.4450312760337,50.9624524279942));
#23736=CARTESIAN_POINT('Ctrl Pts',(-33.3323638343148,33.0047626522954,50.9994956910674));
#23737=CARTESIAN_POINT('Ctrl Pts',(-33.6643793534521,32.5644940285572,51.0365389541407));
#23738=CARTESIAN_POINT('Ctrl Pts',(-33.7565895052947,31.9433833024971,51.0735822172138));
#23739=CARTESIAN_POINT('Ctrl Pts',(-33.5667994243086,31.4256473744548,51.1106254802871));
#23740=CARTESIAN_POINT('Ctrl Pts',(-33.3770093433226,30.9079114464125,51.1476687433603));
#23741=CARTESIAN_POINT('Ctrl Pts',(-32.9052190295081,30.4935503163879,51.1847120064336));
#23742=CARTESIAN_POINT('Ctrl Pts',(-32.3673171723679,30.3721733908449,51.2217552695068));
#23743=CARTESIAN_POINT('Ctrl Pts',(-31.8294153152277,30.2507964653019,51.2587985325801));
#23744=CARTESIAN_POINT('Ctrl Pts',(-31.2254019147619,30.4224037442404,51.2958417956533));
#23745=CARTESIAN_POINT('Ctrl Pts',(-30.8316702277433,30.8084686670345,51.3328850587265));
#23746=CARTESIAN_POINT('Ctrl Pts',(-30.5177779850596,31.1162487833744,51.3624168269478));
#23747=CARTESIAN_POINT('Ctrl Pts',(-30.3375335804213,31.5603308157666,51.391948595169));
#23748=CARTESIAN_POINT('Ctrl Pts',(-30.3334713021565,32.0014789858971,51.4214803633902));
#23749=CARTESIAN_POINT('Ctrl Pts',(-30.3313738111782,31.9995820848862,51.2285196366098));
#23750=CARTESIAN_POINT('Ctrl Pts',(-30.3312972900628,31.9768562581447,51.2269932938115));
#23751=CARTESIAN_POINT('Ctrl Pts',(-30.3317213912061,31.9541333521705,51.2254669510132));
#23752=CARTESIAN_POINT('Ctrl Pts',(-30.3326549959156,31.9314313992364,51.2239406082148));
#23753=CARTESIAN_POINT('Ctrl Pts',(-30.3553129236745,31.38047101488,51.1868973451416));
#23754=CARTESIAN_POINT('Ctrl Pts',(-30.6780677700083,30.8418519430456,51.1498540820683));
#23755=CARTESIAN_POINT('Ctrl Pts',(-31.1532286673374,30.5620433504833,51.1128108189951));
#23756=CARTESIAN_POINT('Ctrl Pts',(-31.6283895646664,30.2822347579209,51.0757675559219));
#23757=CARTESIAN_POINT('Ctrl Pts',(-32.2559565129908,30.2612366446307,51.0387242928487));
#23758=CARTESIAN_POINT('Ctrl Pts',(-32.7487582795783,30.5086576333871,51.0016810297754));
#23759=CARTESIAN_POINT('Ctrl Pts',(-33.2415600461658,30.7560786221434,50.9646377667022));
#23760=CARTESIAN_POINT('Ctrl Pts',(-33.5995966310166,31.2719187129463,50.9275945036289));
#23761=CARTESIAN_POINT('Ctrl Pts',(-33.659032434285,31.8201322772756,50.8905512405557));
#23762=CARTESIAN_POINT('Ctrl Pts',(-33.7184682375533,32.3683458416049,50.8535079774824));
#23763=CARTESIAN_POINT('Ctrl Pts',(-33.4793032592393,32.9489328794607,50.8164647144092));
#23764=CARTESIAN_POINT('Ctrl Pts',(-33.0509780965965,33.2962199104198,50.7794214513359));
#23765=CARTESIAN_POINT('Ctrl Pts',(-32.6226529339536,33.6435069413789,50.7423781882627));
#23766=CARTESIAN_POINT('Ctrl Pts',(-32.005167586982,33.7574939654412,50.7053349251895));
#23767=CARTESIAN_POINT('Ctrl Pts',(-31.4810800022833,33.5860211384661,50.6682916621163));
#23768=CARTESIAN_POINT('Ctrl Pts',(-30.9569924175846,33.414548311491,50.631248399043));
#23769=CARTESIAN_POINT('Ctrl Pts',(-30.5263025951589,32.9576156334784,50.5942051359698));
#23770=CARTESIAN_POINT('Ctrl Pts',(-30.3860918624286,32.4243130202719,50.5571618728965));
#23771=CARTESIAN_POINT('Ctrl Pts',(-30.3499543968131,32.2868613111755,50.5476144608009));
#23772=CARTESIAN_POINT('Ctrl Pts',(-30.3331129511714,32.1443364803049,50.5380670487054));
#23773=CARTESIAN_POINT('Ctrl Pts',(-30.3343902510906,32.0015149949486,50.5285196366098));
#23774=CARTESIAN_POINT('Origin',(-32.,32.,48.));
#23775=CARTESIAN_POINT('',(-30.3365646132776,31.9994923926615,49.8285196366098));
#23776=CARTESIAN_POINT('',(-30.3334137894091,31.9985292433869,50.0214803633902));
#23777=CARTESIAN_POINT('',(-30.334,32.,48.));
#23778=CARTESIAN_POINT('Ctrl Pts',(-30.3334137894091,31.9985292433869,50.0214803633902));
#23779=CARTESIAN_POINT('Ctrl Pts',(-30.3374859553988,32.4415387450404,50.05113936803));
#23780=CARTESIAN_POINT('Ctrl Pts',(-30.5194576726712,32.8875030130583,50.0807983726698));
#23781=CARTESIAN_POINT('Ctrl Pts',(-30.8357595188381,33.195527279696,50.1104573773096));
#23782=CARTESIAN_POINT('Ctrl Pts',(-31.2308116333785,33.5802409300893,50.1475006403828));
#23783=CARTESIAN_POINT('Ctrl Pts',(-31.835409450851,33.7497777263432,50.184543903456));
#23784=CARTESIAN_POINT('Ctrl Pts',(-32.3728922882751,33.6265585497666,50.2215871665293));
#23785=CARTESIAN_POINT('Ctrl Pts',(-32.9103751256992,33.50333937319,50.2586304296025));
#23786=CARTESIAN_POINT('Ctrl Pts',(-33.380742983075,33.087364223783,50.2956736926758));
#23787=CARTESIAN_POINT('Ctrl Pts',(-33.5687580793311,32.5689810743834,50.332716955749));
#23788=CARTESIAN_POINT('Ctrl Pts',(-33.7567731755871,32.0505979249839,50.3697602188223));
#23789=CARTESIAN_POINT('Ctrl Pts',(-33.6624355107235,31.4298067755918,50.4068034818955));
#23790=CARTESIAN_POINT('Ctrl Pts',(-33.3289134886565,30.990678290068,50.4438467449687));
#23791=CARTESIAN_POINT('Ctrl Pts',(-32.9953914665895,30.5515498045442,50.480890008042));
#23792=CARTESIAN_POINT('Ctrl Pts',(-32.422685087319,30.2940839828886,50.5179332711152));
#23793=CARTESIAN_POINT('Ctrl Pts',(-31.8728616846295,30.3360957890429,50.5549765341885));
#23794=CARTESIAN_POINT('Ctrl Pts',(-31.3230382819401,30.3781075951973,50.5920197972617));
#23795=CARTESIAN_POINT('Ctrl Pts',(-30.7960978558316,30.7195970291617,50.629063060335));
#23796=CARTESIAN_POINT('Ctrl Pts',(-30.5331654880733,31.2043003775985,50.6661063234082));
#23797=CARTESIAN_POINT('Ctrl Pts',(-30.4021508650182,31.4458196208563,50.6845643367355));
#23798=CARTESIAN_POINT('Ctrl Pts',(-30.3366856270171,31.7228968091386,50.7030223500629));
#23799=CARTESIAN_POINT('Ctrl Pts',(-30.3367088771406,31.9999843288602,50.7214803633902));
#23800=CARTESIAN_POINT('Ctrl Pts',(-30.3343902510906,32.0015149949486,50.5285196366098));
#23801=CARTESIAN_POINT('Ctrl Pts',(-30.3380687817627,31.5901995265833,50.5010237856321));
#23802=CARTESIAN_POINT('Ctrl Pts',(-30.4920238292037,31.1764236117912,50.4735279346544));
#23803=CARTESIAN_POINT('Ctrl Pts',(-30.7681349479738,30.8742782274076,50.4460320836768));
#23804=CARTESIAN_POINT('Ctrl Pts',(-31.1401204092839,30.4672185961501,50.4089888206035));
#23805=CARTESIAN_POINT('Ctrl Pts',(-31.7338229749391,30.2627718820353,50.3719455575303));
#23806=CARTESIAN_POINT('Ctrl Pts',(-32.2775675701133,30.3544917928758,50.334902294457));
#23807=CARTESIAN_POINT('Ctrl Pts',(-32.8213121652876,30.4462117037163,50.2978590313838));
#23808=CARTESIAN_POINT('Ctrl Pts',(-33.3150987899808,30.8340982395122,50.2608157683106));
#23809=CARTESIAN_POINT('Ctrl Pts',(-33.53297336218,31.3406566247105,50.2237725052373));
#23810=CARTESIAN_POINT('Ctrl Pts',(-33.7508479343793,31.8472150099088,50.1867292421641));
#23811=CARTESIAN_POINT('Ctrl Pts',(-33.6928104540846,32.4724452445095,50.1496859790908));
#23812=CARTESIAN_POINT('Ctrl Pts',(-33.3854185575835,32.930245363329,50.1126427160176));
#23813=CARTESIAN_POINT('Ctrl Pts',(-33.0780266610825,33.3880454821486,50.0755994529444));
#23814=CARTESIAN_POINT('Ctrl Pts',(-32.521280348375,33.678415485187,50.0385561898711));
#23815=CARTESIAN_POINT('Ctrl Pts',(-31.9699437133251,33.6684836335197,50.0015129267979));
#23816=CARTESIAN_POINT('Ctrl Pts',(-31.4186070782752,33.6585517818524,49.9644696637246));
#23817=CARTESIAN_POINT('Ctrl Pts',(-30.8726801208827,33.3483180754794,49.9274264006514));
#23818=CARTESIAN_POINT('Ctrl Pts',(-30.5819760566847,32.8797437762647,49.8903831375782));
#23819=CARTESIAN_POINT('Ctrl Pts',(-30.4201475201305,32.6188988055621,49.8697619705887));
#23820=CARTESIAN_POINT('Ctrl Pts',(-30.3374100869024,32.3089856183198,49.8491408035992));
#23821=CARTESIAN_POINT('Ctrl Pts',(-30.3365646132776,31.9994923926615,49.8285196366098));
#23822=CARTESIAN_POINT('Origin',(-32.,32.,48.));
#23823=CARTESIAN_POINT('',(-30.3325307394052,31.9987546512789,49.1285196366098));
#23824=CARTESIAN_POINT('',(-30.3319159461724,32.0009409208263,49.3214803633902));
#23825=CARTESIAN_POINT('',(-30.334,32.,48.));
#23826=CARTESIAN_POINT('Ctrl Pts',(-30.3319159461724,32.0009409208263,49.3214803633902));
#23827=CARTESIAN_POINT('Ctrl Pts',(-30.33154425979,32.0559214513191,49.3251698598506));
#23828=CARTESIAN_POINT('Ctrl Pts',(-30.3340269899209,32.1108680039687,49.3288593563111));
#23829=CARTESIAN_POINT('Ctrl Pts',(-30.3394745332028,32.1655190278833,49.3325488527715));
#23830=CARTESIAN_POINT('Ctrl Pts',(-30.3941689287825,32.7142259524741,49.3695921158447));
#23831=CARTESIAN_POINT('Ctrl Pts',(-30.747732829251,33.2331419519015,49.406635378918));
#23832=CARTESIAN_POINT('Ctrl Pts',(-31.2383773108745,33.4848138785325,49.4436786419912));
#23833=CARTESIAN_POINT('Ctrl Pts',(-31.729021792498,33.7364858051635,49.4807219050645));
#23834=CARTESIAN_POINT('Ctrl Pts',(-32.3567468552764,33.7209136589979,49.5177651681377));
#23835=CARTESIAN_POINT('Ctrl Pts',(-32.8343089141797,33.4452231696848,49.5548084312109));
#23836=CARTESIAN_POINT('Ctrl Pts',(-33.3118709730831,33.1695326803716,49.5918516942842));
#23837=CARTESIAN_POINT('Ctrl Pts',(-33.6392700281113,32.6337238479109,49.6288949573574));
#23838=CARTESIAN_POINT('Ctrl Pts',(-33.6666900469311,32.0829798887342,49.6659382204307));
#23839=CARTESIAN_POINT('Ctrl Pts',(-33.6941100657508,31.5322359295575,49.7029814835039));
#23840=CARTESIAN_POINT('Ctrl Pts',(-33.421551048362,30.9665568436648,49.7400247465772));
#23841=CARTESIAN_POINT('Ctrl Pts',(-32.9737345232321,30.6447943134935,49.7770680096504));
#23842=CARTESIAN_POINT('Ctrl Pts',(-32.5259179981021,30.3230317833222,49.8141112727237));
#23843=CARTESIAN_POINT('Ctrl Pts',(-31.9028439652309,30.2451858088723,49.8511545357969));
#23844=CARTESIAN_POINT('Ctrl Pts',(-31.3896277235822,30.4468782859499,49.8881977988701));
#23845=CARTESIAN_POINT('Ctrl Pts',(-30.8764114819335,30.6485707630274,49.9252410619434));
#23846=CARTESIAN_POINT('Ctrl Pts',(-30.4730530315072,31.1298016916325,49.9622843250166));
#23847=CARTESIAN_POINT('Ctrl Pts',(-30.3641270120983,31.6703624082013,49.9993275880899));
#23848=CARTESIAN_POINT('Ctrl Pts',(-30.3424135395067,31.778118574882,50.0067118465233));
#23849=CARTESIAN_POINT('Ctrl Pts',(-30.3323999345472,31.8882323305804,50.0140961049568));
#23850=CARTESIAN_POINT('Ctrl Pts',(-30.3334137894091,31.9985292433869,50.0214803633902));
#23851=CARTESIAN_POINT('Ctrl Pts',(-30.3365646132776,31.9994923926615,49.8285196366098));
#23852=CARTESIAN_POINT('Ctrl Pts',(-30.3358913027366,31.7530210124703,49.812097540526));
#23853=CARTESIAN_POINT('Ctrl Pts',(-30.3871544065278,31.5068159746518,49.7956754444422));
#23854=CARTESIAN_POINT('Ctrl Pts',(-30.4917685351372,31.2858719553962,49.7792533483584));
#23855=CARTESIAN_POINT('Ctrl Pts',(-30.7277462487909,30.7874893257988,49.7422100852852));
#23856=CARTESIAN_POINT('Ctrl Pts',(-31.2351828471017,30.4176389586602,49.7051668222119));
#23857=CARTESIAN_POINT('Ctrl Pts',(-31.7818780941429,30.345562376553,49.6681235591387));
#23858=CARTESIAN_POINT('Ctrl Pts',(-32.3285733411841,30.2734857944457,49.6310802960654));
#23859=CARTESIAN_POINT('Ctrl Pts',(-32.9145272369558,30.4991829973699,49.5940370329922));
#23860=CARTESIAN_POINT('Ctrl Pts',(-33.2716104559555,30.9193761690595,49.556993769919));
#23861=CARTESIAN_POINT('Ctrl Pts',(-33.6286936749552,31.3395693407491,49.5199505068457));
#23862=CARTESIAN_POINT('Ctrl Pts',(-33.7569062171829,31.954258481204,49.4829072437725));
#23863=CARTESIAN_POINT('Ctrl Pts',(-33.5975787185188,32.4821651727653,49.4458639806992));
#23864=CARTESIAN_POINT('Ctrl Pts',(-33.4382512198546,33.0100718643266,49.408820717626));
#23865=CARTESIAN_POINT('Ctrl Pts',(-32.9913836802987,33.4511961069941,49.3717774545528));
#23866=CARTESIAN_POINT('Ctrl Pts',(-32.4614602629135,33.6036818392199,49.3347341914795));
#23867=CARTESIAN_POINT('Ctrl Pts',(-31.9315368455282,33.7561675714457,49.2976909284063));
#23868=CARTESIAN_POINT('Ctrl Pts',(-31.3185575503135,33.6200147932296,49.260647665333));
#23869=CARTESIAN_POINT('Ctrl Pts',(-30.9030183790179,33.2575262776258,49.2236044022598));
#23870=CARTESIAN_POINT('Ctrl Pts',(-30.547475144405,32.9473741951013,49.1919094803764));
#23871=CARTESIAN_POINT('Ctrl Pts',(-30.3364746602739,32.471525346565,49.1602145584931));
#23872=CARTESIAN_POINT('Ctrl Pts',(-30.3325307394052,31.9987546512789,49.1285196366098));
#23873=CARTESIAN_POINT('Origin',(-32.,32.,48.));
#23874=CARTESIAN_POINT('',(-30.3326865661716,32.0013000733437,48.4285196366098));
#23875=CARTESIAN_POINT('',(-30.3362532366002,32.0008713514045,48.6214803633902));
#23876=CARTESIAN_POINT('',(-30.334,32.,48.));
#23877=CARTESIAN_POINT('Ctrl Pts',(-30.3362532366002,32.0008713514045,48.6214803633902));
#23878=CARTESIAN_POINT('Ctrl Pts',(-30.3352028368295,32.2223423058557,48.6362436147445));
#23879=CARTESIAN_POINT('Ctrl Pts',(-30.3763005180544,32.4434392568329,48.6510068660988));
#23880=CARTESIAN_POINT('Ctrl Pts',(-30.46138393715,32.6460665489047,48.6657701174531));
#23881=CARTESIAN_POINT('Ctrl Pts',(-30.6748712917368,33.1544895179307,48.7028133805264));
#23882=CARTESIAN_POINT('Ctrl Pts',(-31.1652862997157,33.546630265782,48.7398566435996));
#23883=CARTESIAN_POINT('Ctrl Pts',(-31.7082177126003,33.6430473125364,48.7768999066728));
#23884=CARTESIAN_POINT('Ctrl Pts',(-32.2511491254849,33.7394643592909,48.8139431697461));
#23885=CARTESIAN_POINT('Ctrl Pts',(-32.8465969432752,33.5401577049485,48.8509864328194));
#23886=CARTESIAN_POINT('Ctrl Pts',(-33.2220874732316,33.1363289938411,48.8880296958926));
#23887=CARTESIAN_POINT('Ctrl Pts',(-33.5975780031881,32.7325002827336,48.9250729589659));
#23888=CARTESIAN_POINT('Ctrl Pts',(-33.7531112453107,32.1241495148609,48.9621162220391));
#23889=CARTESIAN_POINT('Ctrl Pts',(-33.6175160313481,31.589654702957,48.9991594851123));
#23890=CARTESIAN_POINT('Ctrl Pts',(-33.4819208173855,31.0551598910532,49.0362027481855));
#23891=CARTESIAN_POINT('Ctrl Pts',(-33.0551971473377,30.5945210351181,49.0732460112588));
#23892=CARTESIAN_POINT('Ctrl Pts',(-32.5326114588057,30.4185239779174,49.110289274332));
#23893=CARTESIAN_POINT('Ctrl Pts',(-32.0100257702738,30.2425269207167,49.1473325374053));
#23894=CARTESIAN_POINT('Ctrl Pts',(-31.3915780632577,30.3511716622505,49.1843758004785));
#23895=CARTESIAN_POINT('Ctrl Pts',(-30.9602666550951,30.6947429578944,49.2214190635518));
#23896=CARTESIAN_POINT('Ctrl Pts',(-30.5719137171571,31.0040946688145,49.2547728301646));
#23897=CARTESIAN_POINT('Ctrl Pts',(-30.3352760634632,31.5039062165043,49.2881265967774));
#23898=CARTESIAN_POINT('Ctrl Pts',(-30.3319159461724,32.0009409208263,49.3214803633902));
#23899=CARTESIAN_POINT('Ctrl Pts',(-30.3325307394052,31.9987546512789,49.1285196366098));
#23900=CARTESIAN_POINT('Ctrl Pts',(-30.3318652247682,31.9189772348117,49.1231712954199));
#23901=CARTESIAN_POINT('Ctrl Pts',(-30.3370955793185,31.8392874677704,49.11782295423));
#23902=CARTESIAN_POINT('Ctrl Pts',(-30.3485221783749,31.7604963040532,49.1124746130401));
#23903=CARTESIAN_POINT('Ctrl Pts',(-30.427664196404,31.2147790990761,49.0754313499668));
#23904=CARTESIAN_POINT('Ctrl Pts',(-30.8040472798389,30.7121689421136,49.0383880868936));
#23905=CARTESIAN_POINT('Ctrl Pts',(-31.305440570552,30.4826575157017,49.0013448238203));
#23906=CARTESIAN_POINT('Ctrl Pts',(-31.806833861265,30.2531460892897,48.9643015607471));
#23907=CARTESIAN_POINT('Ctrl Pts',(-32.4332373592563,30.2967333934283,48.9272582976738));
#23908=CARTESIAN_POINT('Ctrl Pts',(-32.8980122203765,30.593474114086,48.8902150346006));
#23909=CARTESIAN_POINT('Ctrl Pts',(-33.3627870814967,30.8902148347436,48.8531717715274));
#23910=CARTESIAN_POINT('Ctrl Pts',(-33.6659333057459,31.4401089719203,48.8161285084541));
#23911=CARTESIAN_POINT('Ctrl Pts',(-33.6687328246495,31.9915279501207,48.7790852453809));
#23912=CARTESIAN_POINT('Ctrl Pts',(-33.6715323435531,32.5429469283212,48.7420419823076));
#23913=CARTESIAN_POINT('Ctrl Pts',(-33.3739851571112,33.0958907475454,48.7049987192344));
#23914=CARTESIAN_POINT('Ctrl Pts',(-32.9122472444572,33.3973353143294,48.6679554561611));
#23915=CARTESIAN_POINT('Ctrl Pts',(-32.4505093318031,33.6987798811135,48.6309121930879));
#23916=CARTESIAN_POINT('Ctrl Pts',(-31.824580692937,33.7487251954573,48.5938689300146));
#23917=CARTESIAN_POINT('Ctrl Pts',(-31.3208828790471,33.5243165523343,48.5568256669414));
#23918=CARTESIAN_POINT('Ctrl Pts',(-30.8171850651572,33.2999079092114,48.5197824038682));
#23919=CARTESIAN_POINT('Ctrl Pts',(-30.4357180762436,32.8011453086217,48.4827391407949));
#23920=CARTESIAN_POINT('Ctrl Pts',(-30.3510391380146,32.2562598121675,48.4456958777217));
#23921=CARTESIAN_POINT('Ctrl Pts',(-30.337951145404,32.1720422074084,48.4399704640177));
#23922=CARTESIAN_POINT('Ctrl Pts',(-30.331953078525,32.0867227796296,48.4342450503138));
#23923=CARTESIAN_POINT('Ctrl Pts',(-30.3326865661716,32.0013000733437,48.4285196366098));
#23924=CARTESIAN_POINT('Origin',(-32.,32.,48.));
#23925=CARTESIAN_POINT('',(-30.3366116302933,32.0004190051012,47.7285196366098));
#23926=CARTESIAN_POINT('',(-30.3350931202687,31.9985848581543,47.9214803633902));
#23927=CARTESIAN_POINT('',(-30.334,32.,48.));
#23928=CARTESIAN_POINT('Ctrl Pts',(-30.3350931202687,31.9985848581543,47.9214803633902));
#23929=CARTESIAN_POINT('Ctrl Pts',(-30.3382178428148,32.3854996272437,47.9473173696384));
#23930=CARTESIAN_POINT('Ctrl Pts',(-30.4725790046439,32.7743714460338,47.9731543758866));
#23931=CARTESIAN_POINT('Ctrl Pts',(-30.719095213247,33.0695907169318,47.9989913821348));
#23932=CARTESIAN_POINT('Ctrl Pts',(-31.0725326308559,33.4928551234624,48.036034645208));
#23933=CARTESIAN_POINT('Ctrl Pts',(-31.6565135644067,33.7236093551146,48.0730779082813));
#23934=CARTESIAN_POINT('Ctrl Pts',(-32.2038115052115,33.6562615266971,48.1101211713545));
#23935=CARTESIAN_POINT('Ctrl Pts',(-32.7511094460163,33.5889136982795,48.1471644344277));
#23936=CARTESIAN_POINT('Ctrl Pts',(-33.2617243940749,33.2234638097922,48.1842076975009));
#23937=CARTESIAN_POINT('Ctrl Pts',(-33.5020017178502,32.7271397486375,48.2212509605742));
#23938=CARTESIAN_POINT('Ctrl Pts',(-33.7422790416254,32.2308156874827,48.2582942236474));
#23939=CARTESIAN_POINT('Ctrl Pts',(-33.7122187411171,31.6036174536605,48.2953374867207));
#23940=CARTESIAN_POINT('Ctrl Pts',(-33.4255762468427,31.1325475581271,48.332380749794));
#23941=CARTESIAN_POINT('Ctrl Pts',(-33.1389337525684,30.6614776625936,48.3694240128672));
#23942=CARTESIAN_POINT('Ctrl Pts',(-32.5957090645279,30.346536105349,48.4064672759404));
#23943=CARTESIAN_POINT('Ctrl Pts',(-32.0444788544554,30.3318384352888,48.4435105390137));
#23944=CARTESIAN_POINT('Ctrl Pts',(-31.493248644383,30.3171407652286,48.4805538020869));
#23945=CARTESIAN_POINT('Ctrl Pts',(-30.9340129122786,30.6026869823528,48.5175970651601));
#23946=CARTESIAN_POINT('Ctrl Pts',(-30.6226748968236,31.0578126860153,48.5546403282334));
#23947=CARTESIAN_POINT('Ctrl Pts',(-30.4354177802146,31.3315522318847,48.5769203399523));
#23948=CARTESIAN_POINT('Ctrl Pts',(-30.3378384510384,31.6666376963542,48.5992003516713));
#23949=CARTESIAN_POINT('Ctrl Pts',(-30.3362532366002,32.0008713514045,48.6214803633902));
#23950=CARTESIAN_POINT('Ctrl Pts',(-30.3326865661716,32.0013000733437,48.4285196366098));
#23951=CARTESIAN_POINT('Ctrl Pts',(-30.3366987226406,31.5340403107302,48.3972017872405));
#23952=CARTESIAN_POINT('Ctrl Pts',(-30.5421229447233,31.0636903945153,48.3658839378712));
#23953=CARTESIAN_POINT('Ctrl Pts',(-30.8903064956353,30.753676870927,48.334566088502));
#23954=CARTESIAN_POINT('Ctrl Pts',(-31.3021436790294,30.3869878184592,48.2975228254287));
#23955=CARTESIAN_POINT('Ctrl Pts',(-31.9137089333623,30.2446181058425,48.2604795623555));
#23956=CARTESIAN_POINT('Ctrl Pts',(-32.4451533143256,30.3917153416025,48.2234362992823));
#23957=CARTESIAN_POINT('Ctrl Pts',(-32.9765976952889,30.5388125773625,48.186393036209));
#23958=CARTESIAN_POINT('Ctrl Pts',(-33.4279212028827,30.9753767614993,48.1493497731358));
#23959=CARTESIAN_POINT('Ctrl Pts',(-33.5926006472318,31.5016384905226,48.1123065100625));
#23960=CARTESIAN_POINT('Ctrl Pts',(-33.757280091581,32.0279002195459,48.0752632469893));
#23961=CARTESIAN_POINT('Ctrl Pts',(-33.6353154726855,32.6438594934557,48.0382199839161));
#23962=CARTESIAN_POINT('Ctrl Pts',(-33.2825171388263,33.0676566884109,48.0011767208428));
#23963=CARTESIAN_POINT('Ctrl Pts',(-32.9297188049672,33.4914538833661,47.9641334577696));
#23964=CARTESIAN_POINT('Ctrl Pts',(-32.3460867561444,33.7230889993668,47.9270901946963));
#23965=CARTESIAN_POINT('Ctrl Pts',(-31.7986878532862,33.6565670633202,47.890046931623));
#23966=CARTESIAN_POINT('Ctrl Pts',(-31.2512889504281,33.5900451272736,47.8530036685498));
#23967=CARTESIAN_POINT('Ctrl Pts',(-30.7401231935345,33.2253661391796,47.8159604054766));
#23968=CARTESIAN_POINT('Ctrl Pts',(-30.4990972612792,32.7294052266006,47.7789171424033));
#23969=CARTESIAN_POINT('Ctrl Pts',(-30.3897916835172,32.5044862994563,47.7621179738055));
#23970=CARTESIAN_POINT('Ctrl Pts',(-30.3360439926465,32.252567479493,47.7453188052076));
#23971=CARTESIAN_POINT('Ctrl Pts',(-30.3366116302933,32.0004190051012,47.7285196366098));
#23972=CARTESIAN_POINT('Origin',(-32.,32.,48.));
#23973=CARTESIAN_POINT('',(-30.3342224488932,31.998478175086,47.0285196366098));
#23974=CARTESIAN_POINT('',(-30.3312462010541,31.9999631497184,47.2214803633902));
#23975=CARTESIAN_POINT('',(-30.334,32.,48.));
#23976=CARTESIAN_POINT('Ctrl Pts',(-30.3312465935645,31.9999631549708,47.2214803633902));
#23977=CARTESIAN_POINT('Ctrl Pts',(-30.3314253835204,32.5494177694831,47.2583911245323));
#23978=CARTESIAN_POINT('Ctrl Pts',(-30.6293231342425,33.0990385199082,47.2953018856743));
#23979=CARTESIAN_POINT('Ctrl Pts',(-31.0898621581925,33.3987102928711,47.3322126468164));
#23980=CARTESIAN_POINT('Ctrl Pts',(-31.5520544211483,33.6994578249731,47.3692559098896));
#23981=CARTESIAN_POINT('Ctrl Pts',(-32.1780577496979,33.748458629264,47.4062991729629));
#23982=CARTESIAN_POINT('Ctrl Pts',(-32.6814164150587,33.5232902033959,47.4433424360361));
#23983=CARTESIAN_POINT('Ctrl Pts',(-33.1847750804195,33.2981217775279,47.4803856991094));
#23984=CARTESIAN_POINT('Ctrl Pts',(-33.5654890825915,32.7987841215009,47.5174289621826));
#23985=CARTESIAN_POINT('Ctrl Pts',(-33.6493457585165,32.2537714391672,47.5544722252558));
#23986=CARTESIAN_POINT('Ctrl Pts',(-33.7332024344415,31.7087587568336,47.5915154883291));
#23987=CARTESIAN_POINT('Ctrl Pts',(-33.5202017841195,31.1180710481933,47.6285587514023));
#23988=CARTESIAN_POINT('Ctrl Pts',(-33.10781175019,30.7520038058494,47.6656020144756));
#23989=CARTESIAN_POINT('Ctrl Pts',(-32.6954217162604,30.3859365635055,47.7026452775488));
#23990=CARTESIAN_POINT('Ctrl Pts',(-32.0836422987232,30.2444897874579,47.7396885406221));
#23991=CARTESIAN_POINT('Ctrl Pts',(-31.5524204418077,30.392388755463,47.7767318036953));
#23992=CARTESIAN_POINT('Ctrl Pts',(-31.0211985848922,30.540287723468,47.8137750667685));
#23993=CARTESIAN_POINT('Ctrl Pts',(-30.5705342885984,30.9775324355256,47.8508183298418));
#23994=CARTESIAN_POINT('Ctrl Pts',(-30.4066490912849,31.5040420822589,47.887861592915));
#23995=CARTESIAN_POINT('Ctrl Pts',(-30.357070856039,31.6633207697356,47.8990678497401));
#23996=CARTESIAN_POINT('Ctrl Pts',(-30.3337378377324,31.8307687330905,47.9102741065651));
#23997=CARTESIAN_POINT('Ctrl Pts',(-30.3350931202687,31.9985848581543,47.9214803633902));
#23998=CARTESIAN_POINT('Ctrl Pts',(-30.3366116302933,32.0004190051012,47.7285196366098));
#23999=CARTESIAN_POINT('Ctrl Pts',(-30.3372956707017,31.6965636382308,47.7082755421344));
#24000=CARTESIAN_POINT('Ctrl Pts',(-30.416855468772,31.3923747712685,47.688031447659));
#24001=CARTESIAN_POINT('Ctrl Pts',(-30.573116579137,31.1346996365665,47.6677873531836));
#24002=CARTESIAN_POINT('Ctrl Pts',(-30.8590479368673,30.6631977961753,47.6307440901104));
#24003=CARTESIAN_POINT('Ctrl Pts',(-31.4017967599448,30.3474369524569,47.5937008270371));
#24004=CARTESIAN_POINT('Ctrl Pts',(-31.9530041298623,30.331907555355,47.5566575639639));
#24005=CARTESIAN_POINT('Ctrl Pts',(-32.5042114997798,30.3163781582531,47.5196143008906));
#24006=CARTESIAN_POINT('Ctrl Pts',(-33.0638774165373,30.6010802077676,47.4825710378174));
#24007=CARTESIAN_POINT('Ctrl Pts',(-33.3759017912886,31.0557355897734,47.4455277747441));
#24008=CARTESIAN_POINT('Ctrl Pts',(-33.6879261660399,31.5103909717791,47.4084845116709));
#24009=CARTESIAN_POINT('Ctrl Pts',(-33.752308998785,32.134999686276,47.3714412485977));
#24010=CARTESIAN_POINT('Ctrl Pts',(-33.5395890543612,32.6437441723101,47.3343979855244));
#24011=CARTESIAN_POINT('Ctrl Pts',(-33.3268691099373,33.1524886583441,47.2973547224512));
#24012=CARTESIAN_POINT('Ctrl Pts',(-32.8370463883445,33.5453689159152,47.260311459378));
#24013=CARTESIAN_POINT('Ctrl Pts',(-32.2942611110305,33.6426050694634,47.2232681963047));
#24014=CARTESIAN_POINT('Ctrl Pts',(-31.7514758337164,33.7398412230116,47.1862249332315));
#24015=CARTESIAN_POINT('Ctrl Pts',(-31.1557280006812,33.5414332725369,47.1491816701582));
#24016=CARTESIAN_POINT('Ctrl Pts',(-30.7796285900135,33.1381716203541,47.112138407085));
#24017=CARTESIAN_POINT('Ctrl Pts',(-30.4966354293383,32.8347404362218,47.0842654835932));
#24018=CARTESIAN_POINT('Ctrl Pts',(-30.3380005358351,32.4153273065168,47.0563925601015));
#24019=CARTESIAN_POINT('Ctrl Pts',(-30.3342224488932,31.998478175086,47.0285196366098));
#24020=CARTESIAN_POINT('Origin',(-32.,32.,48.));
#24021=CARTESIAN_POINT('',(-30.3314412831326,32.0005167954427,46.3285196366098));
#24022=CARTESIAN_POINT('',(-30.334985752807,32.0014384754872,46.5214803633902));
#24023=CARTESIAN_POINT('',(-30.334,32.,48.));
#24024=CARTESIAN_POINT('Ctrl Pts',(-30.334985752807,32.0014384754872,46.5214803633902));
#24025=CARTESIAN_POINT('Ctrl Pts',(-30.333634356184,32.1652593777732,46.5324216163529));
#24026=CARTESIAN_POINT('Ctrl Pts',(-30.3558556724076,32.3287216717838,46.5433628693156));
#24027=CARTESIAN_POINT('Ctrl Pts',(-30.403150530605,32.4845752228154,46.5543041222783));
#24028=CARTESIAN_POINT('Ctrl Pts',(-30.5632744104012,33.0122409400272,46.5913473853516));
#24029=CARTESIAN_POINT('Ctrl Pts',(-31.0108070772609,33.4526904357357,46.6283906484248));
#24030=CARTESIAN_POINT('Ctrl Pts',(-31.5409600094739,33.6043764089425,46.665433911498));
#24031=CARTESIAN_POINT('Ctrl Pts',(-32.0711129416868,33.7560623821493,46.7024771745713));
#24032=CARTESIAN_POINT('Ctrl Pts',(-32.6838861392531,33.6189848328544,46.7395204376445));
#24033=CARTESIAN_POINT('Ctrl Pts',(-33.0988779095908,33.2558697043431,46.7765637007178));
#24034=CARTESIAN_POINT('Ctrl Pts',(-33.5138696799284,32.8927545758318,46.813606963791));
#24035=CARTESIAN_POINT('Ctrl Pts',(-33.7310800230373,32.3036018681042,46.8506502268642));
#24036=CARTESIAN_POINT('Ctrl Pts',(-33.6511146636849,31.7580046656688,46.8876934899375));
#24037=CARTESIAN_POINT('Ctrl Pts',(-33.5711493043325,31.2124074632333,46.9247367530107));
#24038=CARTESIAN_POINT('Ctrl Pts',(-33.1940082425188,30.7103657660902,46.961780016084));
#24039=CARTESIAN_POINT('Ctrl Pts',(-32.6922691831675,30.4816111326442,46.9988232791572));
#24040=CARTESIAN_POINT('Ctrl Pts',(-32.1905301238162,30.2528564991983,47.0358665422305));
#24041=CARTESIAN_POINT('Ctrl Pts',(-31.5641930669273,30.2973889294496,47.0729098053037));
#24042=CARTESIAN_POINT('Ctrl Pts',(-31.0998664535619,30.5948306247821,47.109953068377));
#24043=CARTESIAN_POINT('Ctrl Pts',(-30.6355398401965,30.8922723201147,47.1469963314502));
#24044=CARTESIAN_POINT('Ctrl Pts',(-30.3332236703546,31.4426232805285,47.1840395945234));
#24045=CARTESIAN_POINT('Ctrl Pts',(-30.3312561841146,31.9940458906921,47.2210828575967));
#24046=CARTESIAN_POINT('Ctrl Pts',(-30.331249146513,31.9960183022638,47.2212153595278));
#24047=CARTESIAN_POINT('Ctrl Pts',(-30.3312459517459,31.9979907275468,47.221347861459));
#24048=CARTESIAN_POINT('Ctrl Pts',(-30.3312465935646,31.9999631549708,47.2214803633902));
#24049=CARTESIAN_POINT('Ctrl Pts',(-30.3342224488932,31.998478175086,47.0285196366098));
#24050=CARTESIAN_POINT('Ctrl Pts',(-30.3329794382619,31.8613326011525,47.0193492970283));
#24051=CARTESIAN_POINT('Ctrl Pts',(-30.3484988233775,31.7244645658994,47.0101789574468));
#24052=CARTESIAN_POINT('Ctrl Pts',(-30.3818667490394,31.592095847254,47.0010086178652));
#24053=CARTESIAN_POINT('Ctrl Pts',(-30.5166553070329,31.0573970802274,46.963965354792));
#24054=CARTESIAN_POINT('Ctrl Pts',(-30.9426834113199,30.596114900065,46.9269220917188));
#24055=CARTESIAN_POINT('Ctrl Pts',(-31.46500291142,30.4193295312107,46.8898788286455));
#24056=CARTESIAN_POINT('Ctrl Pts',(-31.98732241152,30.2425441623563,46.8528355655723));
#24057=CARTESIAN_POINT('Ctrl Pts',(-32.605933307433,30.35025560481,46.815792302499));
#24058=CARTESIAN_POINT('Ctrl Pts',(-33.0377626074672,30.6931756865459,46.7787490394258));
#24059=CARTESIAN_POINT('Ctrl Pts',(-33.4695919075013,31.0360957682818,46.7417057763525));
#24060=CARTESIAN_POINT('Ctrl Pts',(-33.7146396116566,31.6142244892999,46.7046625132793));
#24061=CARTESIAN_POINT('Ctrl Pts',(-33.6607732192273,32.1630132816348,46.6676192502061));
#24062=CARTESIAN_POINT('Ctrl Pts',(-33.606906826798,32.7118020739697,46.6305759871328));
#24063=CARTESIAN_POINT('Ctrl Pts',(-33.2541263377842,33.2312509376214,46.5935327240596));
#24064=CARTESIAN_POINT('Ctrl Pts',(-32.7638621910861,33.483662889177,46.5564894609863));
#24065=CARTESIAN_POINT('Ctrl Pts',(-32.273598044388,33.7360748407326,46.5194461979131));
#24066=CARTESIAN_POINT('Ctrl Pts',(-31.6458502400056,33.7214498801921,46.4824029348399));
#24067=CARTESIAN_POINT('Ctrl Pts',(-31.1678727694035,33.4464803101984,46.4453596717666));
#24068=CARTESIAN_POINT('Ctrl Pts',(-30.6898952988014,33.1715107402047,46.4083164086934));
#24069=CARTESIAN_POINT('Ctrl Pts',(-30.3616881619796,32.6361965607576,46.3712731456201));
#24070=CARTESIAN_POINT('Ctrl Pts',(-30.3334371651187,32.085494637752,46.3342298825469));
#24071=CARTESIAN_POINT('Ctrl Pts',(-30.3319855278829,32.0571976038022,46.3323264672345));
#24072=CARTESIAN_POINT('Ctrl Pts',(-30.3313258564002,32.0288599420261,46.3304230519221));
#24073=CARTESIAN_POINT('Ctrl Pts',(-30.3314412831326,32.0005167954427,46.3285196366098));
#24074=CARTESIAN_POINT('Origin',(-32.,32.,48.));
#24075=CARTESIAN_POINT('',(-30.3357441935225,32.0011936368988,45.6285196366098));
#24076=CARTESIAN_POINT('',(-30.336314001127,31.9991832783969,45.8214803633902));
#24077=CARTESIAN_POINT('',(-30.334,32.,48.));
#24078=CARTESIAN_POINT('Ctrl Pts',(-30.336314001127,31.9991832783969,45.8214803633902));
#24079=CARTESIAN_POINT('Ctrl Pts',(-30.3377789880212,32.3294716685071,45.8434953712468));
#24080=CARTESIAN_POINT('Ctrl Pts',(-30.4328915994036,32.6605377086288,45.8655103791034));
#24081=CARTESIAN_POINT('Ctrl Pts',(-30.6159865666574,32.9323348061725,45.88752538696));
#24082=CARTESIAN_POINT('Ctrl Pts',(-30.9240689022873,33.3896706132929,45.9245686500332));
#24083=CARTESIAN_POINT('Ctrl Pts',(-31.4812527529819,33.6792002364776,45.9616119131064));
#24084=CARTESIAN_POINT('Ctrl Pts',(-32.032573809867,33.6684364900661,45.9986551761797));
#24085=CARTESIAN_POINT('Ctrl Pts',(-32.5838948667521,33.6576727436547,46.0356984392529));
#24086=CARTESIAN_POINT('Ctrl Pts',(-33.1293531298277,33.3466156276472,46.0727417023262));
#24087=CARTESIAN_POINT('Ctrl Pts',(-33.4193498555347,32.8776031916916,46.1097849653994));
#24088=CARTESIAN_POINT('Ctrl Pts',(-33.7093465812416,32.408590755736,46.1468282284727));
#24089=CARTESIAN_POINT('Ctrl Pts',(-33.7438817695798,31.7816229998324,46.1838714915459));
#24090=CARTESIAN_POINT('Ctrl Pts',(-33.5071523056252,31.2835969694912,46.2209147546192));
#24091=CARTESIAN_POINT('Ctrl Pts',(-33.2704228416705,30.78557093915,46.2579580176924));
#24092=CARTESIAN_POINT('Ctrl Pts',(-32.7624287254228,30.4164866343711,46.2950012807656));
#24093=CARTESIAN_POINT('Ctrl Pts',(-32.2156253099937,30.3452350317451,46.3320445438389));
#24094=CARTESIAN_POINT('Ctrl Pts',(-31.6688218945646,30.2739834291191,46.3690878069121));
#24095=CARTESIAN_POINT('Ctrl Pts',(-31.0832091799541,30.500564528646,46.4061310699853));
#24096=CARTESIAN_POINT('Ctrl Pts',(-30.7267603690151,30.9212960477671,46.4431743330586));
#24097=CARTESIAN_POINT('Ctrl Pts',(-30.4755937682591,31.217758547418,46.4692763431691));
#24098=CARTESIAN_POINT('Ctrl Pts',(-30.3382097133934,31.6106189905197,46.4953783532797));
#24099=CARTESIAN_POINT('Ctrl Pts',(-30.334985752807,32.0014384754872,46.5214803633902));
#24100=CARTESIAN_POINT('Ctrl Pts',(-30.3314412831326,32.0005167954427,46.3285196366098));
#24101=CARTESIAN_POINT('Ctrl Pts',(-30.3335722304769,31.4772605993123,46.2933797888489));
#24102=CARTESIAN_POINT('Ctrl Pts',(-30.5998767510865,30.9521350386003,46.258239941088));
#24103=CARTESIAN_POINT('Ctrl Pts',(-31.0242217941959,30.6462651999857,46.2231000933271));
#24104=CARTESIAN_POINT('Ctrl Pts',(-31.471552277034,30.3238273517893,46.1860568302539));
#24105=CARTESIAN_POINT('Ctrl Pts',(-32.0945080996103,30.2450413219607,46.1490135671807));
#24106=CARTESIAN_POINT('Ctrl Pts',(-32.608028055351,30.4459591705499,46.1119703041074));
#24107=CARTESIAN_POINT('Ctrl Pts',(-33.1215480110917,30.6468770191392,46.0749270410342));
#24108=CARTESIAN_POINT('Ctrl Pts',(-33.525632099997,31.1274987461464,46.0378837779609));
#24109=CARTESIAN_POINT('Ctrl Pts',(-33.6353736340385,31.6678944553558,46.0008405148877));
#24110=CARTESIAN_POINT('Ctrl Pts',(-33.74511516808,32.2082901645652,45.9637972518145));
#24111=CARTESIAN_POINT('Ctrl Pts',(-33.5605141472577,32.8084598559768,45.9267539887412));
#24112=CARTESIAN_POINT('Ctrl Pts',(-33.1660429977425,33.1937691330854,45.889710725668));
#24113=CARTESIAN_POINT('Ctrl Pts',(-32.7715718482274,33.5790784101939,45.8526674625947));
#24114=CARTESIAN_POINT('Ctrl Pts',(-32.1672305700194,33.7495272729993,45.8156241995215));
#24115=CARTESIAN_POINT('Ctrl Pts',(-31.6295624551223,33.6271192461024,45.7785809364482));
#24116=CARTESIAN_POINT('Ctrl Pts',(-31.0918943402253,33.5047112192054,45.741537673375));
#24117=CARTESIAN_POINT('Ctrl Pts',(-30.6208993886393,33.0894463026061,45.7044944103018));
#24118=CARTESIAN_POINT('Ctrl Pts',(-30.4321023363463,32.57134747046,45.6674511472285));
#24119=CARTESIAN_POINT('Ctrl Pts',(-30.3659620647077,32.3898446499573,45.6544739770223));
#24120=CARTESIAN_POINT('Ctrl Pts',(-30.3344552072224,32.1957212904815,45.641496806816));
#24121=CARTESIAN_POINT('Ctrl Pts',(-30.3357441935225,32.0011936368988,45.6285196366098));
#24122=CARTESIAN_POINT('Origin',(-32.,32.,48.));
#24123=CARTESIAN_POINT('',(-30.3357491953914,31.9988087176276,44.9285196366098));
#24124=CARTESIAN_POINT('',(-30.3320048130563,31.999003946099,45.1214803633902));
#24125=CARTESIAN_POINT('',(-30.334,32.,48.));
#24126=CARTESIAN_POINT('Ctrl Pts',(-30.3320048130563,31.999003946099,45.1214803633902));
#24127=CARTESIAN_POINT('Ctrl Pts',(-30.3354915306281,32.4921586983372,45.1545691261407));
#24128=CARTESIAN_POINT('Ctrl Pts',(-30.5679112921037,32.9881690576534,45.1876578888911));
#24129=CARTESIAN_POINT('Ctrl Pts',(-30.9509788831921,33.297804326917,45.2207466516416));
#24130=CARTESIAN_POINT('Ctrl Pts',(-31.3798276031801,33.6444446900695,45.2577899147148));
#24131=CARTESIAN_POINT('Ctrl Pts',(-31.9974842806894,33.7574998752863,45.2948331777881));
#24132=CARTESIAN_POINT('Ctrl Pts',(-32.5213125691959,33.5852364428286,45.3318764408614));
#24133=CARTESIAN_POINT('Ctrl Pts',(-33.0451408577023,33.4129730103709,45.3689197039346));
#24134=CARTESIAN_POINT('Ctrl Pts',(-33.4751407572058,32.9553909602385,45.4059629670078));
#24135=CARTESIAN_POINT('Ctrl Pts',(-33.6145466452709,32.4218773574368,45.443006230081));
#24136=CARTESIAN_POINT('Ctrl Pts',(-33.7539525333361,31.888363754635,45.4800494931543));
#24137=CARTESIAN_POINT('Ctrl Pts',(-33.6027644099628,31.2789185991639,45.5170927562275));
#24138=CARTESIAN_POINT('Ctrl Pts',(-33.2301651406233,30.8724206895882,45.5541360193008));
#24139=CARTESIAN_POINT('Ctrl Pts',(-32.8575658712839,30.4659227800126,45.591179282374));
#24140=CARTESIAN_POINT('Ctrl Pts',(-32.2635554559781,30.2623721163323,45.6282225454473));
#24141=CARTESIAN_POINT('Ctrl Pts',(-31.7199498398627,30.3549123785401,45.6652658085205));
#24142=CARTESIAN_POINT('Ctrl Pts',(-31.1763442237472,30.4474526407479,45.7023090715938));
#24143=CARTESIAN_POINT('Ctrl Pts',(-30.6831434068221,30.8360838288437,45.739352334667));
#24144=CARTESIAN_POINT('Ctrl Pts',(-30.4660334086422,31.3429704184197,45.7763955977402));
#24145=CARTESIAN_POINT('Ctrl Pts',(-30.3779530347214,31.5486116174412,45.7914238529569));
#24146=CARTESIAN_POINT('Ctrl Pts',(-30.3353139471148,31.7737162581709,45.8064521081735));
#24147=CARTESIAN_POINT('Ctrl Pts',(-30.336314001127,31.9991832783969,45.8214803633902));
#24148=CARTESIAN_POINT('Ctrl Pts',(-30.3357441935225,32.0011936368988,45.6285196366098));
#24149=CARTESIAN_POINT('Ctrl Pts',(-30.3381346117347,31.6404431418435,45.6044535437428));
#24150=CARTESIAN_POINT('Ctrl Pts',(-30.4533148708266,31.2783022185287,45.5803874508758));
#24151=CARTESIAN_POINT('Ctrl Pts',(-30.6695651562039,30.9926846858579,45.5563213580088));
#24152=CARTESIAN_POINT('Ctrl Pts',(-31.0024241813547,30.5530534810948,45.5192780949355));
#24153=CARTESIAN_POINT('Ctrl Pts',(-31.5747413846563,30.2947238192617,45.4822348318623));
#24154=CARTESIAN_POINT('Ctrl Pts',(-32.1246275171387,30.335905952879,45.4451915687891));
#24155=CARTESIAN_POINT('Ctrl Pts',(-32.6745136496211,30.3770880864963,45.4081483057158));
#24156=CARTESIAN_POINT('Ctrl Pts',(-33.2019687112843,30.717782015564,45.3711050426426));
#24157=CARTESIAN_POINT('Ctrl Pts',(-33.4656321259172,31.2020880454767,45.3340617795694));
#24158=CARTESIAN_POINT('Ctrl Pts',(-33.7292955405502,31.6863940753895,45.2970185164961));
#24159=CARTESIAN_POINT('Ctrl Pts',(-33.7291673081528,32.3143122061471,45.2599752534228));
#24160=CARTESIAN_POINT('Ctrl Pts',(-33.4653061071749,32.7985105058593,45.2229319903496));
#24161=CARTESIAN_POINT('Ctrl Pts',(-33.2014449061969,33.2827088055716,45.1858887272763));
#24162=CARTESIAN_POINT('Ctrl Pts',(-32.6738507366385,33.6231872742384,45.1488454642032));
#24163=CARTESIAN_POINT('Ctrl Pts',(-32.1239478297291,33.6641448107654,45.1118022011299));
#24164=CARTESIAN_POINT('Ctrl Pts',(-31.5740449228197,33.7051023472924,45.0747589380567));
#24165=CARTESIAN_POINT('Ctrl Pts',(-31.0018332785595,33.4465389516795,45.0377156749834));
#24166=CARTESIAN_POINT('Ctrl Pts',(-30.6691538426735,33.0067718317578,45.0006724119101));
#24167=CARTESIAN_POINT('Ctrl Pts',(-30.4531564512173,32.7212460657954,44.97662148681));
#24168=CARTESIAN_POINT('Ctrl Pts',(-30.3381329336397,32.3593345722981,44.9525705617099));
#24169=CARTESIAN_POINT('Ctrl Pts',(-30.3357491953914,31.9988087176276,44.9285196366098));
#24170=CARTESIAN_POINT('Origin',(-32.,32.,48.));
#24171=CARTESIAN_POINT('',(-30.3314442636938,31.9994792812594,44.2285196366098));
#24172=CARTESIAN_POINT('',(-30.333294480282,32.0014513626233,44.4214803633902));
#24173=CARTESIAN_POINT('',(-30.334,32.,48.));
#24174=CARTESIAN_POINT('Ctrl Pts',(-30.333294480282,32.0014513626233,44.4214803633902));
#24175=CARTESIAN_POINT('Ctrl Pts',(-30.3323222284007,32.1077703704247,44.4285996179613));
#24176=CARTESIAN_POINT('Ctrl Pts',(-30.3416240402429,32.2139199074504,44.4357188725324));
#24177=CARTESIAN_POINT('Ctrl Pts',(-30.3618163870715,32.3179556962936,44.4428381271035));
#24178=CARTESIAN_POINT('Ctrl Pts',(-30.4668822206032,32.8592799398168,44.4798813901767));
#24179=CARTESIAN_POINT('Ctrl Pts',(-30.8667963627591,33.3433769601342,44.51692465325));
#24180=CARTESIAN_POINT('Ctrl Pts',(-31.3785602705332,33.5487265856548,44.5539679163233));
#24181=CARTESIAN_POINT('Ctrl Pts',(-31.8903241783073,33.7540762111755,44.5910111793965));
#24182=CARTESIAN_POINT('Ctrl Pts',(-32.5139378516996,33.6806784418995,44.6280544424697));
#24183=CARTESIAN_POINT('Ctrl Pts',(-32.9640390551699,33.3621196990649,44.6650977055429));
#24184=CARTESIAN_POINT('Ctrl Pts',(-33.4141402586402,33.0435609562303,44.7021409686162));
#24185=CARTESIAN_POINT('Ctrl Pts',(-33.6907289921885,32.4798412398371,44.7391842316895));
#24186=CARTESIAN_POINT('Ctrl Pts',(-33.6672397510832,31.9289156354639,44.7762274947627));
#24187=CARTESIAN_POINT('Ctrl Pts',(-33.6437505099779,31.3779900310907,44.813270757836));
#24188=CARTESIAN_POINT('Ctrl Pts',(-33.3201832942189,30.8398585387374,44.8503140209091));
#24189=CARTESIAN_POINT('Ctrl Pts',(-32.8446007072674,30.5607672114085,44.8873572839824));
#24190=CARTESIAN_POINT('Ctrl Pts',(-32.3690181203159,30.2816758840796,44.9244005470556));
#24191=CARTESIAN_POINT('Ctrl Pts',(-31.7414201621719,30.261624721775,44.9614438101289));
#24192=CARTESIAN_POINT('Ctrl Pts',(-31.2489922554738,30.5097890276424,44.9984870732021));
#24193=CARTESIAN_POINT('Ctrl Pts',(-30.7565643487757,30.7579533335098,45.0355303362754));
#24194=CARTESIAN_POINT('Ctrl Pts',(-30.3993064935235,31.2743331075492,45.0725735993487));
#24195=CARTESIAN_POINT('Ctrl Pts',(-30.3406979471307,31.8226357651129,45.1096168624219));
#24196=CARTESIAN_POINT('Ctrl Pts',(-30.3344412759738,31.8811690274777,45.1135713627447));
#24197=CARTESIAN_POINT('Ctrl Pts',(-30.3315881088759,31.9400660933418,45.1175258630674));
#24198=CARTESIAN_POINT('Ctrl Pts',(-30.3320048130563,31.999003946099,45.1214803633902));
#24199=CARTESIAN_POINT('Ctrl Pts',(-30.3357491953914,31.9988087176276,44.9285196366098));
#24200=CARTESIAN_POINT('Ctrl Pts',(-30.3344614971914,31.8040522277035,44.9155272986367));
#24201=CARTESIAN_POINT('Ctrl Pts',(-30.3660440362041,31.6097000911722,44.9025349606636));
#24202=CARTESIAN_POINT('Ctrl Pts',(-30.4323358263775,31.4280121903116,44.8895426226905));
#24203=CARTESIAN_POINT('Ctrl Pts',(-30.6213444734794,30.9099905130176,44.8524993596172));
#24204=CARTESIAN_POINT('Ctrl Pts',(-31.0925089951951,30.4949180026602,44.815456096544));
#24205=CARTESIAN_POINT('Ctrl Pts',(-31.6302270611707,30.3727295893424,44.7784128334707));
#24206=CARTESIAN_POINT('Ctrl Pts',(-32.1679451271464,30.2505411760246,44.7413695703975));
#24207=CARTESIAN_POINT('Ctrl Pts',(-32.7722167373819,30.4212368597464,44.7043263073242));
#24208=CARTESIAN_POINT('Ctrl Pts',(-33.16653047956,30.8067072211947,44.667283044251));
#24209=CARTESIAN_POINT('Ctrl Pts',(-33.5608442217381,31.1921775826431,44.6302397811777));
#24210=CARTESIAN_POINT('Ctrl Pts',(-33.7452000958586,31.792422621818,44.5931965181045));
#24211=CARTESIAN_POINT('Ctrl Pts',(-33.6352378535522,32.3327734634876,44.5561532550313));
#24212=CARTESIAN_POINT('Ctrl Pts',(-33.5252756112458,32.8731243051572,44.519109991958));
#24213=CARTESIAN_POINT('Ctrl Pts',(-33.1209952525124,33.3535809493216,44.4820667288848));
#24214=CARTESIAN_POINT('Ctrl Pts',(-32.6073932773895,33.554289040776,44.4450234658115));
#24215=CARTESIAN_POINT('Ctrl Pts',(-32.0937913022666,33.7549971322304,44.4079802027383));
#24216=CARTESIAN_POINT('Ctrl Pts',(-31.4708677107543,33.6759566709748,44.370936939665));
#24217=CARTESIAN_POINT('Ctrl Pts',(-31.0236689606658,33.3533361435062,44.3338936765918));
#24218=CARTESIAN_POINT('Ctrl Pts',(-30.5996319917973,33.0474251128168,44.2987689965978));
#24219=CARTESIAN_POINT('Ctrl Pts',(-30.3335886032366,32.522512110404,44.2636443166038));
#24220=CARTESIAN_POINT('Ctrl Pts',(-30.3314442636938,31.9994792812594,44.2285196366098));
#24221=CARTESIAN_POINT('Origin',(-32.,32.,48.));
#24222=CARTESIAN_POINT('',(-30.3342156580691,32.0015219727962,43.5285196366098));
#24223=CARTESIAN_POINT('',(-30.3367054458351,32.0000809143127,43.7214803633902));
#24224=CARTESIAN_POINT('',(-30.334,32.,48.));
#24225=CARTESIAN_POINT('Ctrl Pts',(-30.3367054458351,32.0000809143127,43.7214803633902));
#24226=CARTESIAN_POINT('Ctrl Pts',(-30.3365871091324,32.2731888506978,43.7396733728552));
#24227=CARTESIAN_POINT('Ctrl Pts',(-30.4000931468668,32.5462449571753,43.7578663823202));
#24228=CARTESIAN_POINT('Ctrl Pts',(-30.5275247652971,32.7852121099577,43.7760593917851));
#24229=CARTESIAN_POINT('Ctrl Pts',(-30.7869916212039,33.2717793886379,43.8131026548584));
#24230=CARTESIAN_POINT('Ctrl Pts',(-31.3114817803501,33.6170203467136,43.8501459179317));
#24231=CARTESIAN_POINT('Ctrl Pts',(-31.8609913898654,33.6629545937273,43.8871891810049));
#24232=CARTESIAN_POINT('Ctrl Pts',(-32.4105009993806,33.7088888407409,43.9242324440781));
#24233=CARTESIAN_POINT('Ctrl Pts',(-32.9850300592647,33.4555163766925,43.9612757071513));
#24234=CARTESIAN_POINT('Ctrl Pts',(-33.3216771869561,33.0187790672924,43.9983189702246));
#24235=CARTESIAN_POINT('Ctrl Pts',(-33.6583243146476,32.5820417578923,44.0353622332978));
#24236=CARTESIAN_POINT('Ctrl Pts',(-33.7570895101463,31.9619396031405,44.0724054963711));
#24237=CARTESIAN_POINT('Ctrl Pts',(-33.5727783555304,31.442227986679,44.1094487594444));
#24238=CARTESIAN_POINT('Ctrl Pts',(-33.3884672009146,30.9225163702175,44.1464920225176));
#24239=CARTESIAN_POINT('Ctrl Pts',(-32.9210796961843,30.5031952920463,44.1835352855908));
#24240=CARTESIAN_POINT('Ctrl Pts',(-32.3844898291976,30.376143803867,44.220578548664));
#24241=CARTESIAN_POINT('Ctrl Pts',(-31.8478999622109,30.2490923156877,44.2576218117373));
#24242=CARTESIAN_POINT('Ctrl Pts',(-31.2421077329678,30.4143104175003,44.2946650748106));
#24243=CARTESIAN_POINT('Ctrl Pts',(-30.8443203808,30.796195201771,44.3317083378838));
#24244=CARTESIAN_POINT('Ctrl Pts',(-30.5229828116778,31.1046864788154,44.361632346386));
#24245=CARTESIAN_POINT('Ctrl Pts',(-30.337381098238,31.5545659673038,44.3915563548881));
#24246=CARTESIAN_POINT('Ctrl Pts',(-30.333294480282,32.0014513626233,44.4214803633902));
#24247=CARTESIAN_POINT('Ctrl Pts',(-30.3314442636938,31.9994792812594,44.2285196366098));
#24248=CARTESIAN_POINT('Ctrl Pts',(-30.3313271354078,31.9709101402436,44.2266010535305));
#24249=CARTESIAN_POINT('Ctrl Pts',(-30.3319973688349,31.9423466088594,44.2246824704513));
#24250=CARTESIAN_POINT('Ctrl Pts',(-30.3334722232713,31.9138246840243,44.2227638873721));
#24251=CARTESIAN_POINT('Ctrl Pts',(-30.36194814463,31.3631343456928,44.1857206242988));
#24252=CARTESIAN_POINT('Ctrl Pts',(-30.6903738960118,30.8279542627113,44.1486773612256));
#24253=CARTESIAN_POINT('Ctrl Pts',(-31.1684636343982,30.5531799391802,44.1116340981524));
#24254=CARTESIAN_POINT('Ctrl Pts',(-31.6465533727846,30.2784056156492,44.0745908350791));
#24255=CARTESIAN_POINT('Ctrl Pts',(-32.2743070981754,30.2640370515686,44.0375475720059));
#24256=CARTESIAN_POINT('Ctrl Pts',(-32.7644681096866,30.5166492239095,44.0005043089326));
#24257=CARTESIAN_POINT('Ctrl Pts',(-33.2546291211977,30.7692613962504,43.9634610458594));
#24258=CARTESIAN_POINT('Ctrl Pts',(-33.6071974188292,31.2888543050128,43.9264177827861));
#24259=CARTESIAN_POINT('Ctrl Pts',(-33.6608396613031,31.8376650526052,43.8893745197129));
#24260=CARTESIAN_POINT('Ctrl Pts',(-33.7144819037769,32.3864758001977,43.8523312566396));
#24261=CARTESIAN_POINT('Ctrl Pts',(-33.4691980910932,32.9645043866202,43.8152879935664));
#24262=CARTESIAN_POINT('Ctrl Pts',(-33.0372287659473,33.307248064791,43.7782447304932));
#24263=CARTESIAN_POINT('Ctrl Pts',(-32.6052594408015,33.6499917429618,43.7412014674199));
#24264=CARTESIAN_POINT('Ctrl Pts',(-31.9866046031935,33.757450512881,43.7041582043467));
#24265=CARTESIAN_POINT('Ctrl Pts',(-31.4643573522818,33.5804518244296,43.6671149412734));
#24266=CARTESIAN_POINT('Ctrl Pts',(-30.94211010137,33.4034531359782,43.6300716782002));
#24267=CARTESIAN_POINT('Ctrl Pts',(-30.5162704371545,32.9419969891563,43.593028415127));
#24268=CARTESIAN_POINT('Ctrl Pts',(-30.3817002809903,32.4072432139639,43.5559851520537));
#24269=CARTESIAN_POINT('Ctrl Pts',(-30.3484415235646,32.2750798383797,43.5468299802391));
#24270=CARTESIAN_POINT('Ctrl Pts',(-30.3329741425732,32.1384392838872,43.5376748084244));
#24271=CARTESIAN_POINT('Ctrl Pts',(-30.3342156580691,32.0015219727962,43.5285196366098));
#24272=CARTESIAN_POINT('Origin',(-32.,32.,48.));
#24273=CARTESIAN_POINT('',(-30.3366133324916,31.9995845730415,42.8285196366098));
#24274=CARTESIAN_POINT('',(-30.3335914213191,31.9985061360497,43.0214803633902));
#24275=CARTESIAN_POINT('',(-30.334,32.,48.));
#24276=CARTESIAN_POINT('Ctrl Pts',(-30.3335914213191,31.9985061360497,43.0214803633902));
#24277=CARTESIAN_POINT('Ctrl Pts',(-30.3376271892743,32.435776657828,43.050747127749));
#24278=CARTESIAN_POINT('Ctrl Pts',(-30.5143062601661,32.8759335579088,43.0800138921079));
#24279=CARTESIAN_POINT('Ctrl Pts',(-30.82319727105,33.1831638556262,43.1092806564668));
#24280=CARTESIAN_POINT('Ctrl Pts',(-31.2141639948336,33.5720285966297,43.14632391954));
#24281=CARTESIAN_POINT('Ctrl Pts',(-31.8169374352255,33.7479417146696,43.1833671826133));
#24282=CARTESIAN_POINT('Ctrl Pts',(-32.3556917358311,33.6304063187777,43.2204104456866));
#24283=CARTESIAN_POINT('Ctrl Pts',(-32.8944460364368,33.5128709228859,43.2574537087598));
#24284=CARTESIAN_POINT('Ctrl Pts',(-33.3691811972561,33.1018870130622,43.294496971833));
#24285=CARTESIAN_POINT('Ctrl Pts',(-33.5626609820717,32.585518598986,43.3315402349062));
#24286=CARTESIAN_POINT('Ctrl Pts',(-33.7561407668874,32.0691501849098,43.3685834979795));
#24287=CARTESIAN_POINT('Ctrl Pts',(-33.6683651756993,31.447397266581,43.4056267610527));
#24288=CARTESIAN_POINT('Ctrl Pts',(-33.3394998434811,31.0047706076013,43.442670024126));
#24289=CARTESIAN_POINT('Ctrl Pts',(-33.0106345112629,30.5621439486216,43.4797132871992));
#24290=CARTESIAN_POINT('Ctrl Pts',(-32.4406794380146,30.2986435489909,43.5167565502724));
#24291=CARTESIAN_POINT('Ctrl Pts',(-31.8904429746054,30.3348457630668,43.5537998133457));
#24292=CARTESIAN_POINT('Ctrl Pts',(-31.3402065111961,30.3710479771428,43.5908430764189));
#24293=CARTESIAN_POINT('Ctrl Pts',(-30.8096886576259,30.7069528049254,43.6278863394922));
#24294=CARTESIAN_POINT('Ctrl Pts',(-30.5416515071744,31.1888520184591,43.6649296025654));
#24295=CARTESIAN_POINT('Ctrl Pts',(-30.4052550927318,31.4340766999556,43.6837798561737));
#24296=CARTESIAN_POINT('Ctrl Pts',(-30.3368280575922,31.7171066283268,43.7026301097819));
#24297=CARTESIAN_POINT('Ctrl Pts',(-30.3367054458351,32.0000809143127,43.7214803633902));
#24298=CARTESIAN_POINT('Ctrl Pts',(-30.3342156580691,32.0015219727962,43.5285196366098));
#24299=CARTESIAN_POINT('Ctrl Pts',(-30.3379975092617,31.5844503389818,43.5006315453512));
#24300=CARTESIAN_POINT('Ctrl Pts',(-30.4968224279369,31.1648106605338,43.4727434540926));
#24301=CARTESIAN_POINT('Ctrl Pts',(-30.7800935628365,30.8613300297991,43.444855362834));
#24302=CARTESIAN_POINT('Ctrl Pts',(-31.1563576489599,30.4582220243893,43.4078120997608));
#24303=CARTESIAN_POINT('Ctrl Pts',(-31.7521864693196,30.2600574171324,43.3707688366875));
#24304=CARTESIAN_POINT('Ctrl Pts',(-32.2949319865817,30.3575152552835,43.3337255736143));
#24305=CARTESIAN_POINT('Ctrl Pts',(-32.8376775038437,30.4549730934347,43.296682310541));
#24306=CARTESIAN_POINT('Ctrl Pts',(-33.3273397180079,30.8480533769938,43.2596390474678));
#24307=CARTESIAN_POINT('Ctrl Pts',(-33.5398518547276,31.3568847045873,43.2225957843945));
#24308=CARTESIAN_POINT('Ctrl Pts',(-33.7523639914472,31.8657160321808,43.1855525213213));
#24309=CARTESIAN_POINT('Ctrl Pts',(-33.6877260507221,32.4902984038087,43.1485092582481));
#24310=CARTESIAN_POINT('Ctrl Pts',(-33.3755160041951,32.9448263029854,43.1114659951748));
#24311=CARTESIAN_POINT('Ctrl Pts',(-33.0633059576681,33.3993542021622,43.0744227321016));
#24312=CARTESIAN_POINT('Ctrl Pts',(-32.5035238053391,33.6838276288878,43.0373794690283));
#24313=CARTESIAN_POINT('Ctrl Pts',(-31.9523228239278,33.6680731051537,43.0003362059551));
#24314=CARTESIAN_POINT('Ctrl Pts',(-31.4011218425165,33.6523185814197,42.9632929428818));
#24315=CARTESIAN_POINT('Ctrl Pts',(-30.8585020320229,33.3363361072259,42.9262496798086));
#24316=CARTESIAN_POINT('Ctrl Pts',(-30.5727632772645,32.864717510685,42.8892064167354));
#24317=CARTESIAN_POINT('Ctrl Pts',(-30.4167244230102,32.6071716782637,42.8689774900269));
#24318=CARTESIAN_POINT('Ctrl Pts',(-30.3372909516162,32.3032130626764,42.8487485633183));
#24319=CARTESIAN_POINT('Ctrl Pts',(-30.3366133324916,31.9995845730415,42.8285196366098));
#24320=CARTESIAN_POINT('Origin',(-32.,32.,48.));
#24321=CARTESIAN_POINT('',(-30.3326930047543,31.9986962112692,42.1285196366098));
#24322=CARTESIAN_POINT('',(-30.3317921991812,32.000855278924,42.3214803633902));
#24323=CARTESIAN_POINT('',(-30.334,32.,48.));
#24324=CARTESIAN_POINT('Ctrl Pts',(-30.3317921991812,32.000855278924,42.3214803633902));
#24325=CARTESIAN_POINT('Ctrl Pts',(-30.331484649223,32.049981083659,42.3247776195697));
#24326=CARTESIAN_POINT('Ctrl Pts',(-30.3334666242309,32.0990817223638,42.3280748757492));
#24327=CARTESIAN_POINT('Ctrl Pts',(-30.3378188894502,32.1479713507645,42.3313721319287));
#24328=CARTESIAN_POINT('Ctrl Pts',(-30.3867147279015,32.6972254177245,42.368415395002));
#24329=CARTESIAN_POINT('Ctrl Pts',(-30.734778204715,33.219846689238,42.4054586580752));
#24330=CARTESIAN_POINT('Ctrl Pts',(-31.2227371783014,33.476686743959,42.4425019211484));
#24331=CARTESIAN_POINT('Ctrl Pts',(-31.7106961518878,33.7335267986801,42.4795451842217));
#24332=CARTESIAN_POINT('Ctrl Pts',(-32.3385506222471,33.7245856366086,42.5165884472949));
#24333=CARTESIAN_POINT('Ctrl Pts',(-32.8189978800188,33.4539545644561,42.5536317103681));
#24334=CARTESIAN_POINT('Ctrl Pts',(-33.2994451377906,33.1833234923036,42.5906749734414));
#24335=CARTESIAN_POINT('Ctrl Pts',(-33.6324851829748,32.6510025100702,42.6277182365147));
#24336=CARTESIAN_POINT('Ctrl Pts',(-33.6657206503217,32.100578873737,42.6647614995879));
#24337=CARTESIAN_POINT('Ctrl Pts',(-33.6989561176687,31.5501552374038,42.7018047626611));
#24338=CARTESIAN_POINT('Ctrl Pts',(-33.4323870071784,30.9816289469708,42.7388480257344));
#24339=CARTESIAN_POINT('Ctrl Pts',(-32.9879939218415,30.6551545194728,42.7758912888076));
#24340=CARTESIAN_POINT('Ctrl Pts',(-32.5436008365046,30.3286800919748,42.8129345518808));
#24341=CARTESIAN_POINT('Ctrl Pts',(-31.9213837763209,30.2442575274118,42.8499778149541));
#24342=CARTESIAN_POINT('Ctrl Pts',(-31.4060658823589,30.4405181491037,42.8870210780273));
#24343=CARTESIAN_POINT('Ctrl Pts',(-30.8907479883968,30.6367787707956,42.9240643411006));
#24344=CARTESIAN_POINT('Ctrl Pts',(-30.4823292606563,31.1137225787423,42.9611076041738));
#24345=CARTESIAN_POINT('Ctrl Pts',(-30.3676999003737,31.6531026646991,42.9981508672471));
#24346=CARTESIAN_POINT('Ctrl Pts',(-30.3436357386635,31.7663348207516,43.0059273659614));
#24347=CARTESIAN_POINT('Ctrl Pts',(-30.3325190737261,31.8823185859417,43.0137038646758));
#24348=CARTESIAN_POINT('Ctrl Pts',(-30.3335914213191,31.9985061360497,43.0214803633902));
#24349=CARTESIAN_POINT('Ctrl Pts',(-30.3366133324916,31.9995845730415,42.8285196366098));
#24350=CARTESIAN_POINT('Ctrl Pts',(-30.3360500937171,31.7472077846831,42.8117053002451));
#24351=CARTESIAN_POINT('Ctrl Pts',(-30.3898990963236,31.4950590796035,42.7948909638804));
#24352=CARTESIAN_POINT('Ctrl Pts',(-30.4993953032921,31.2699817889122,42.7780766275156));
#24353=CARTESIAN_POINT('Ctrl Pts',(-30.740623783101,30.7741193825682,42.7410333644424));
#24354=CARTESIAN_POINT('Ctrl Pts',(-31.2519384417417,30.4096492887681,42.7039901013691));
#24355=CARTESIAN_POINT('Ctrl Pts',(-31.7993644708408,30.3433508944012,42.6669468382959));
#24356=CARTESIAN_POINT('Ctrl Pts',(-32.3467904999399,30.2770525000343,42.6299035752227));
#24357=CARTESIAN_POINT('Ctrl Pts',(-32.9303278994973,30.5089258051006,42.5928603121494));
#24358=CARTESIAN_POINT('Ctrl Pts',(-33.2829531058532,30.9328671429222,42.5558170490762));
#24359=CARTESIAN_POINT('Ctrl Pts',(-33.6355783122092,31.3568084807439,42.518773786003));
#24360=CARTESIAN_POINT('Ctrl Pts',(-33.7572913253637,31.972817851321,42.4817305229297));
#24361=CARTESIAN_POINT('Ctrl Pts',(-33.5923969576212,32.4990121121331,42.4446872598564));
#24362=CARTESIAN_POINT('Ctrl Pts',(-33.4275025898788,33.0252063729452,42.4076439967832));
#24363=CARTESIAN_POINT('Ctrl Pts',(-32.9760008412393,33.4615855239924,42.3706007337099));
#24364=CARTESIAN_POINT('Ctrl Pts',(-32.444496409946,33.6084660091537,42.3335574706367));
#24365=CARTESIAN_POINT('Ctrl Pts',(-31.9129919786527,33.755346494315,42.2965142075635));
#24366=CARTESIAN_POINT('Ctrl Pts',(-31.3014848647057,33.6127283135904,42.2594709444903));
#24367=CARTESIAN_POINT('Ctrl Pts',(-30.8897975141205,33.245870442855,42.222427681417));
#24368=CARTESIAN_POINT('Ctrl Pts',(-30.5419092076928,32.9358644075266,42.1911249998146));
#24369=CARTESIAN_POINT('Ctrl Pts',(-30.3367074574263,32.4657341253069,42.1598223182122));
#24370=CARTESIAN_POINT('Ctrl Pts',(-30.3326930047543,31.9986962112692,42.1285196366098));
#24371=CARTESIAN_POINT('Origin',(-32.,32.,48.));
#24372=CARTESIAN_POINT('',(-30.3325261571163,32.001210199007,41.4285196366098));
#24373=CARTESIAN_POINT('',(-30.3361589164137,32.0009454232939,41.6214803633902));
#24374=CARTESIAN_POINT('',(-30.334,32.,48.));
#24375=CARTESIAN_POINT('',(-33.2690708798524,33.0793586530485,41.));
#24376=CARTESIAN_POINT('Ctrl Pts',(-30.3325261571163,32.001210199007,41.4285196366098));
#24377=CARTESIAN_POINT('Ctrl Pts',(-30.3364619003144,31.5283280072703,41.3968095469596));
#24378=CARTESIAN_POINT('Ctrl Pts',(-30.5476791715277,31.0524653264148,41.3650994573094));
#24379=CARTESIAN_POINT('Ctrl Pts',(-30.9035244685572,30.7421792451538,41.3333893676592));
#24380=CARTESIAN_POINT('Ctrl Pts',(-31.3192177414759,30.3797075819416,41.2963461045859));
#24381=CARTESIAN_POINT('Ctrl Pts',(-31.9322786735049,30.243191197321,41.2593028415127));
#24382=CARTESIAN_POINT('Ctrl Pts',(-32.4621353555657,30.3962172700897,41.2222595784394));
#24383=CARTESIAN_POINT('Ctrl Pts',(-32.9919920376265,30.5492433428584,41.1852163153662));
#24384=CARTESIAN_POINT('Ctrl Pts',(-33.4386444697191,30.9918118730164,41.148173052293));
#24385=CARTESIAN_POINT('Ctrl Pts',(-33.5976357473726,31.5188493258702,41.1111297892197));
#24386=CARTESIAN_POINT('Ctrl Pts',(-33.7566270250261,32.0458867787241,41.0740865261465));
#24387=CARTESIAN_POINT('Ctrl Pts',(-33.6279571482407,32.6573931542737,41.0370432630732));
#24388=CARTESIAN_POINT('Ctrl Pts',(-33.2690708798524,33.0793586530485,41.));
#24389=CARTESIAN_POINT('',(-30.7285328989217,33.0812099237989,41.));
#24390=CARTESIAN_POINT('Origin',(-32.,32.,41.));
#24391=CARTESIAN_POINT('Ctrl Pts',(-30.728531577822,33.0812109444531,41.));
#24392=CARTESIAN_POINT('Ctrl Pts',(-31.0793196648972,33.4926490838295,41.0363148168372));
#24393=CARTESIAN_POINT('Ctrl Pts',(-31.6491071451624,33.71867271397,41.0726296336745));
#24394=CARTESIAN_POINT('Ctrl Pts',(-32.1864002116813,33.6582000435223,41.1089444505117));
#24395=CARTESIAN_POINT('Ctrl Pts',(-32.734470948199,33.5965143395801,41.145987713585));
#24396=CARTESIAN_POINT('Ctrl Pts',(-33.2487305721424,33.2367232829171,41.1830309766582));
#24397=CARTESIAN_POINT('Ctrl Pts',(-33.4941904525548,32.7430255098163,41.2200742397314));
#24398=CARTESIAN_POINT('Ctrl Pts',(-33.7396503329672,32.2493277367155,41.2571175028047));
#24399=CARTESIAN_POINT('Ctrl Pts',(-33.7163104698485,31.621723247177,41.2941607658779));
#24400=CARTESIAN_POINT('Ctrl Pts',(-33.434682746762,31.1476214758446,41.3312040289512));
#24401=CARTESIAN_POINT('Ctrl Pts',(-33.1530550236755,30.6735197045122,41.3682472920244));
#24402=CARTESIAN_POINT('Ctrl Pts',(-32.6131394406212,30.352920651386,41.4052905550976));
#24403=CARTESIAN_POINT('Ctrl Pts',(-32.0620834325308,30.3324171571387,41.4423338181709));
#24404=CARTESIAN_POINT('Ctrl Pts',(-31.5110274244403,30.3119136628915,41.4793770812441));
#24405=CARTESIAN_POINT('Ctrl Pts',(-30.9488309913136,30.5915057275232,41.5164203443174));
#24406=CARTESIAN_POINT('Ctrl Pts',(-30.6327092444556,31.0433098742836,41.5534636073906));
#24407=CARTESIAN_POINT('Ctrl Pts',(-30.4392275877983,31.3198356611636,41.5761358593905));
#24408=CARTESIAN_POINT('Ctrl Pts',(-30.3379261613561,31.6608725508196,41.5988081113903));
#24409=CARTESIAN_POINT('Ctrl Pts',(-30.3361589164137,32.0009454232939,41.6214803633902));
#24410=CARTESIAN_POINT('Origin',(-32.,32.,39.4540747194623));
#24411=CARTESIAN_POINT('',(-29.9467153330669,32.0018314293989,53.7459252805377));
#24412=CARTESIAN_POINT('',(-29.9453611728806,31.9981689810755,53.8040747194623));
#24413=CARTESIAN_POINT('',(-29.94525,32.0000000000002,39.4540747194623));
#24414=CARTESIAN_POINT('',(-32.3836679988468,34.0186125009919,54.));
#24415=CARTESIAN_POINT('Ctrl Pts',(-29.9453611728806,31.9981689810755,53.8040747194623));
#24416=CARTESIAN_POINT('Ctrl Pts',(-29.9506279893844,32.5196386238579,53.832339883235));
#24417=CARTESIAN_POINT('Ctrl Pts',(-30.4182837037984,33.7322194813403,53.8976483100809));
#24418=CARTESIAN_POINT('Ctrl Pts',(-31.7124802469751,34.146181938655,53.9629567369268));
#24419=CARTESIAN_POINT('Ctrl Pts',(-32.3836679988468,34.0186125009919,54.));
#24420=CARTESIAN_POINT('',(-33.3415658188825,33.5612633204521,54.));
#24421=CARTESIAN_POINT('Origin',(-32.,32.,54.));
#24422=CARTESIAN_POINT('Ctrl Pts',(-29.9467153330669,32.0018314293989,53.7459252805377));
#24423=CARTESIAN_POINT('Ctrl Pts',(-29.9450489223381,32.2111833794062,53.7572587737813));
#24424=CARTESIAN_POINT('Ctrl Pts',(-30.0707451594838,33.1027824480144,53.8056355300982));
#24425=CARTESIAN_POINT('Ctrl Pts',(-31.3453228671131,34.3305891564746,53.8903271032523));
#24426=CARTESIAN_POINT('Ctrl Pts',(-32.8352371619566,33.9952106642201,53.9636851831628));
#24427=CARTESIAN_POINT('Ctrl Pts',(-33.3415672325378,33.5612648174638,54.));
#24428=CARTESIAN_POINT('Origin',(-32.,32.,39.4540747194623));
#24429=CARTESIAN_POINT('',(-29.9479916519948,31.9988943668812,53.0459252805377));
#24430=CARTESIAN_POINT('',(-29.9421906513588,32.0007573773506,53.1040747194623));
#24431=CARTESIAN_POINT('',(-29.94525,32.0000000000002,39.4540747194623));
#24432=CARTESIAN_POINT('Ctrl Pts',(-29.9421906513588,32.0007573773506,53.1040747194623));
#24433=CARTESIAN_POINT('Ctrl Pts',(-29.9419903991083,32.0429235489439,53.1063703750556));
#24434=CARTESIAN_POINT('Ctrl Pts',(-29.9622810371399,32.7652974030863,53.1457092937221));
#24435=CARTESIAN_POINT('Ctrl Pts',(-30.8113288145004,34.117796910195,53.2220914754619));
#24436=CARTESIAN_POINT('Ctrl Pts',(-33.1343255579885,34.1473076805079,53.3332212646816));
#24437=CARTESIAN_POINT('Ctrl Pts',(-34.4195104110039,32.2117840240242,53.4443510539014));
#24438=CARTESIAN_POINT('Ctrl Pts',(-33.4897707576895,30.0821245375598,53.5554808431211));
#24439=CARTESIAN_POINT('Ctrl Pts',(-31.1978269251376,29.7083052230924,53.6666106323408));
#24440=CARTESIAN_POINT('Ctrl Pts',(-30.0344356528229,30.992528820682,53.7494752577879));
#24441=CARTESIAN_POINT('Ctrl Pts',(-29.9437254972964,31.8362200766428,53.7952966201617));
#24442=CARTESIAN_POINT('Ctrl Pts',(-29.9453611728806,31.9981689810755,53.8040747194623));
#24443=CARTESIAN_POINT('Ctrl Pts',(-29.9479916519948,31.9988943668812,53.0459252805377));
#24444=CARTESIAN_POINT('Ctrl Pts',(-29.9500185408881,32.4134550879906,53.0683325286752));
#24445=CARTESIAN_POINT('Ctrl Pts',(-30.2732453084617,33.516265749558,53.127783039886));
#24446=CARTESIAN_POINT('Ctrl Pts',(-32.0730427769752,34.4274726540847,53.2242768141699));
#24447=CARTESIAN_POINT('Ctrl Pts',(-34.0790038841791,33.2553327473947,53.3354066033897));
#24448=CARTESIAN_POINT('Ctrl Pts',(-34.182240985042,30.9342477393896,53.4465363926094));
#24449=CARTESIAN_POINT('Ctrl Pts',(-32.288398343005,29.5886824305611,53.5576661818291));
#24450=CARTESIAN_POINT('Ctrl Pts',(-30.3505279832561,30.3618200065023,53.6574624778052));
#24451=CARTESIAN_POINT('Ctrl Pts',(-29.950495547636,31.5269213260117,53.7202155107081));
#24452=CARTESIAN_POINT('Ctrl Pts',(-29.9467153330669,32.0018314293989,53.7459252805377));
#24453=CARTESIAN_POINT('Origin',(-32.,32.,39.4540747194623));
#24454=CARTESIAN_POINT('',(-29.9426288446654,31.9988731525755,52.3459252805377));
#24455=CARTESIAN_POINT('',(-29.9475562773048,32.0013942151196,52.4040747194623));
#24456=CARTESIAN_POINT('',(-29.94525,32.0000000000002,39.4540747194623));
#24457=CARTESIAN_POINT('Ctrl Pts',(-29.9475562773048,32.0013942151196,52.4040747194623));
#24458=CARTESIAN_POINT('Ctrl Pts',(-29.9460125610086,32.2486122196956,52.4174441299495));
#24459=CARTESIAN_POINT('Ctrl Pts',(-30.1017872573193,33.1789290640202,52.4678568035099));
#24460=CARTESIAN_POINT('Ctrl Pts',(-31.4859339899109,34.3735521292407,52.5553127401435));
#24461=CARTESIAN_POINT('Ctrl Pts',(-33.7152268428034,33.7193027479294,52.6664425293632));
#24462=CARTESIAN_POINT('Ctrl Pts',(-34.3747678520742,31.4915687675265,52.777572318583));
#24463=CARTESIAN_POINT('Ctrl Pts',(-32.8609368582137,29.729140329846,52.8887021078027));
#24464=CARTESIAN_POINT('Ctrl Pts',(-30.6067538535749,30.0384637365273,52.9975362414292));
#24465=CARTESIAN_POINT('Ctrl Pts',(-29.945221718656,31.3625198369552,53.0693271119824));
#24466=CARTESIAN_POINT('Ctrl Pts',(-29.9421906513588,32.0007573773506,53.1040747194623));
#24467=CARTESIAN_POINT('Ctrl Pts',(-29.9426288446654,31.9988731525755,52.3459252805377));
#24468=CARTESIAN_POINT('Ctrl Pts',(-29.9466921151103,32.6141860878724,52.3794062835691));
#24469=CARTESIAN_POINT('Ctrl Pts',(-30.5667600306827,33.917382824163,52.4499305496737));
#24470=CARTESIAN_POINT('Ctrl Pts',(-32.7830045631024,34.2988945540426,52.5574980788516));
#24471=CARTESIAN_POINT('Ctrl Pts',(-34.3560464259567,32.5891179074725,52.6686278680713));
#24472=CARTESIAN_POINT('Ctrl Pts',(-33.7728594492291,30.3401856422308,52.7797576572911));
#24473=CARTESIAN_POINT('Ctrl Pts',(-31.5671721178615,29.6103000479543,52.8908874465108));
#24474=CARTESIAN_POINT('Ctrl Pts',(-30.1224675846331,30.7736324025542,52.979609987593));
#24475=CARTESIAN_POINT('Ctrl Pts',(-29.9466677243116,31.7281106959594,53.0312892656019));
#24476=CARTESIAN_POINT('Ctrl Pts',(-29.9479916519948,31.9988943668812,53.0459252805377));
#24477=CARTESIAN_POINT('Origin',(-32.,32.,39.4540747194623));
#24478=CARTESIAN_POINT('',(-29.9445979340372,32.0018240974026,51.6459252805377));
#24479=CARTESIAN_POINT('',(-29.9472436463387,31.9984585483392,51.7040747194623));
#24480=CARTESIAN_POINT('',(-29.94525,32.0000000000002,39.4540747194623));
#24481=CARTESIAN_POINT('Ctrl Pts',(-29.9472436463387,31.9984585483392,51.7040747194623));
#24482=CARTESIAN_POINT('Ctrl Pts',(-29.9503946737569,32.450271766422,51.7285178848434));
#24483=CARTESIAN_POINT('Ctrl Pts',(-30.3199519290529,33.5914867339453,51.7900043132976));
#24484=CARTESIAN_POINT('Ctrl Pts',(-32.2059544077473,34.4198337491439,51.8885340048253));
#24485=CARTESIAN_POINT('Ctrl Pts',(-34.1446539107159,33.1395051684107,51.9996637940449));
#24486=CARTESIAN_POINT('Ctrl Pts',(-34.1205894982053,30.816313858696,52.1107935832648));
#24487=CARTESIAN_POINT('Ctrl Pts',(-32.1557844039238,29.5764191824004,52.2219233724843));
#24488=CARTESIAN_POINT('Ctrl Pts',(-30.3019343182528,30.4368848986496,52.3196837512169));
#24489=CARTESIAN_POINT('Ctrl Pts',(-29.9502898093531,31.5636335073777,52.3804008668763));
#24490=CARTESIAN_POINT('Ctrl Pts',(-29.9475562773048,32.0013942151196,52.4040747194623));
#24491=CARTESIAN_POINT('Ctrl Pts',(-29.9445979340372,32.0018240974026,51.6459252805377));
#24492=CARTESIAN_POINT('Ctrl Pts',(-29.9433235785776,32.1402143164981,51.6534367753897));
#24493=CARTESIAN_POINT('Ctrl Pts',(-30.019149581319,32.9596933491072,51.697991533315));
#24494=CARTESIAN_POINT('Ctrl Pts',(-31.1194585135859,34.2633294087954,51.7795895543135));
#24495=CARTESIAN_POINT('Ctrl Pts',(-33.423850742076,33.9673998993839,51.8907193435332));
#24496=CARTESIAN_POINT('Ctrl Pts',(-34.4251502183154,31.8709273485123,52.001849132753));
#24497=CARTESIAN_POINT('Ctrl Pts',(-33.2069785027727,29.8925806669829,52.1129789219727));
#24498=CARTESIAN_POINT('Ctrl Pts',(-30.8841931736715,29.8429213477129,52.2241087111924));
#24499=CARTESIAN_POINT('Ctrl Pts',(-29.9747293817875,31.1875940441121,52.3017574973808));
#24500=CARTESIAN_POINT('Ctrl Pts',(-29.9421965270932,31.9334060373702,52.3423630204959));
#24501=CARTESIAN_POINT('Ctrl Pts',(-29.9426288446654,31.9988731525755,52.3459252805377));
#24502=CARTESIAN_POINT('Origin',(-32.,32.,39.4540747194623));
#24503=CARTESIAN_POINT('',(-29.948590975573,31.9999806721044,50.9459252805377));
#24504=CARTESIAN_POINT('',(-29.942011007514,31.9994845671788,51.0040747194623));
#24505=CARTESIAN_POINT('',(-29.94525,32.0000000000002,39.4540747194623));
#24506=CARTESIAN_POINT('Ctrl Pts',(-29.942011007514,31.9994845671788,51.0040747194623));
#24507=CARTESIAN_POINT('Ctrl Pts',(-29.9442070892614,32.6516937390639,51.0395916397372));
#24508=CARTESIAN_POINT('Ctrl Pts',(-30.6316982717036,33.9881256658593,51.1121518230854));
#24509=CARTESIAN_POINT('Ctrl Pts',(-32.907797512765,34.2525355120973,51.2217552695069));
#24510=CARTESIAN_POINT('Ctrl Pts',(-34.3847873801667,32.4591314690988,51.3328850587265));
#24511=CARTESIAN_POINT('Ctrl Pts',(-33.6792457006084,30.2455352853812,51.4440148479464));
#24512=CARTESIAN_POINT('Ctrl Pts',(-31.4368765636913,29.6376061806665,51.5551446371659));
#24513=CARTESIAN_POINT('Ctrl Pts',(-30.0897291860077,30.8498858532132,51.6418312610047));
#24514=CARTESIAN_POINT('Ctrl Pts',(-29.9456193373476,31.765555378978,51.6914746217701));
#24515=CARTESIAN_POINT('Ctrl Pts',(-29.9472436463387,31.9984585483392,51.7040747194623));
#24516=CARTESIAN_POINT('Ctrl Pts',(-29.948590975573,31.9999806721044,50.9459252805377));
#24517=CARTESIAN_POINT('Ctrl Pts',(-29.9486198486256,32.3440804588562,50.9645105302836));
#24518=CARTESIAN_POINT('Ctrl Pts',(-30.1938071650696,33.3740627456927,51.0201390431028));
#24519=CARTESIAN_POINT('Ctrl Pts',(-31.8232699686781,34.4221436399707,51.1128108189951));
#24520=CARTESIAN_POINT('Ctrl Pts',(-33.9390244099684,33.4622577248198,51.2239406082149));
#24521=CARTESIAN_POINT('Ctrl Pts',(-34.2802047391973,31.1641293976194,51.3350703974346));
#24522=CARTESIAN_POINT('Ctrl Pts',(-32.5345664187102,29.6309807807203,51.4462001866543));
#24523=CARTESIAN_POINT('Ctrl Pts',(-30.4507580914472,30.2230151239904,51.549818481022));
#24524=CARTESIAN_POINT('Ctrl Pts',(-29.9496081178695,31.4577369409946,51.6163935123165));
#24525=CARTESIAN_POINT('Ctrl Pts',(-29.9445979340372,32.0018240974026,51.6459252805377));
#24526=CARTESIAN_POINT('Origin',(-32.,32.,39.4540747194623));
#24527=CARTESIAN_POINT('',(-29.9445270010734,31.9981860521306,50.2459252805377));
#24528=CARTESIAN_POINT('',(-29.9457313135825,32.001868508926,50.3040747194623));
#24529=CARTESIAN_POINT('',(-29.94525,32.0000000000002,39.4540747194623));
#24530=CARTESIAN_POINT('Ctrl Pts',(-29.9457313135825,32.001868508926,50.3040747194623));
#24531=CARTESIAN_POINT('Ctrl Pts',(-29.9441559642374,32.1780164363184,50.3136221315579));
#24532=CARTESIAN_POINT('Ctrl Pts',(-30.0455183200277,33.0358200312748,50.3602128067267));
#24533=CARTESIAN_POINT('Ctrl Pts',(-31.2448019703849,34.3081786093532,50.4438467449688));
#24534=CARTESIAN_POINT('Ctrl Pts',(-33.5295162861532,33.8864231993434,50.5549765341884));
#24535=CARTESIAN_POINT('Ctrl Pts',(-34.4144338837356,31.738233734696,50.6661063234082));
#24536=CARTESIAN_POINT('Ctrl Pts',(-33.0896877743921,29.8296099173301,50.7772361126279));
#24537=CARTESIAN_POINT('Ctrl Pts',(-30.7676712310498,29.9073035666993,50.8883659018476));
#24538=CARTESIAN_POINT('Ctrl Pts',(-29.9551340465651,31.2632801821069,50.9639787707925));
#24539=CARTESIAN_POINT('Ctrl Pts',(-29.9419166307062,31.9714558201818,51.002548376664));
#24540=CARTESIAN_POINT('Ctrl Pts',(-29.942011007514,31.9994845671788,51.0040747194623));
#24541=CARTESIAN_POINT('Ctrl Pts',(-29.9445270010734,31.9981860521306,50.2459252805377));
#24542=CARTESIAN_POINT('Ctrl Pts',(-29.9495493798654,32.544568869371,50.2755842851775));
#24543=CARTESIAN_POINT('Ctrl Pts',(-30.4542942488099,33.7815642628783,50.3422865528905));
#24544=CARTESIAN_POINT('Ctrl Pts',(-32.5426800327657,34.3671737786953,50.4460320836768));
#24545=CARTESIAN_POINT('Ctrl Pts',(-34.2830552217384,32.828053241641,50.5571618728965));
#24546=CARTESIAN_POINT('Ctrl Pts',(-33.9340030304806,30.5311073577035,50.6682916621162));
#24547=CARTESIAN_POINT('Ctrl Pts',(-31.8149722391133,29.5784760905123,50.779421451336));
#24548=CARTESIAN_POINT('Ctrl Pts',(-30.1913422173688,30.6306870609017,50.8719659908098));
#24549=CARTESIAN_POINT('Ctrl Pts',(-29.948562300188,31.6582366257969,50.9274672672103));
#24550=CARTESIAN_POINT('Ctrl Pts',(-29.948590975573,31.9999806721044,50.9459252805377));
#24551=CARTESIAN_POINT('Origin',(-32.,32.,39.4540747194623));
#24552=CARTESIAN_POINT('',(-29.942679646097,32.0011604784324,49.5459252805377));
#24553=CARTESIAN_POINT('',(-29.9484130486988,31.9993739458711,49.6040747194623));
#24554=CARTESIAN_POINT('',(-29.94525,32.0000000000002,39.4540747194623));
#24555=CARTESIAN_POINT('Ctrl Pts',(-29.9484130486988,31.9993739458711,49.6040747194623));
#24556=CARTESIAN_POINT('Ctrl Pts',(-29.9494558079608,32.381085353687,49.6246958864518));
#24557=CARTESIAN_POINT('Ctrl Pts',(-30.2348077288734,33.4499404032741,49.6823603165144));
#24558=CARTESIAN_POINT('Ctrl Pts',(-31.9562582891885,34.4281884645445,49.7770680096504));
#24559=CARTESIAN_POINT('Ctrl Pts',(-34.0162363552789,33.3538107387165,49.8881977988702));
#24560=CARTESIAN_POINT('Ctrl Pts',(-34.2309767741905,31.040440106281,49.9993275880898));
#24561=CARTESIAN_POINT('Ctrl Pts',(-32.4039514432991,29.6052482825838,50.1104573773096));
#24562=CARTESIAN_POINT('Ctrl Pts',(-30.3959590957835,30.2967181551523,50.2120397544338));
#24563=CARTESIAN_POINT('Ctrl Pts',(-29.9502682048781,31.4945753164748,50.2765788684846));
#24564=CARTESIAN_POINT('Ctrl Pts',(-29.9457313135825,32.001868508926,50.3040747194623));
#24565=CARTESIAN_POINT('Ctrl Pts',(-29.942679646097,32.0011604784324,49.5459252805377));
#24566=CARTESIAN_POINT('Ctrl Pts',(-29.9422212291737,32.0689703493988,49.5496147769981));
#24567=CARTESIAN_POINT('Ctrl Pts',(-29.9760269532423,32.817141878103,49.5903475365318));
#24568=CARTESIAN_POINT('Ctrl Pts',(-30.8915903093585,34.1608890008963,49.6681235591386));
#24569=CARTESIAN_POINT('Ctrl Pts',(-33.2141918809262,34.1032715927325,49.7792533483584));
#24570=CARTESIAN_POINT('Ctrl Pts',(-34.4255782104328,32.1207628319306,49.8903831375781));
#24571=CARTESIAN_POINT('Ctrl Pts',(-33.4171016660518,30.0277332369641,50.0015129267978));
#24572=CARTESIAN_POINT('Ctrl Pts',(-31.1117090447276,29.7397007951857,50.1126427160176));
#24573=CARTESIAN_POINT('Ctrl Pts',(-30.0175818447045,31.0450604521428,50.1941135005975));
#24574=CARTESIAN_POINT('Ctrl Pts',(-29.9432765699345,31.862152089592,50.2385410221043));
#24575=CARTESIAN_POINT('Ctrl Pts',(-29.9445270010734,31.9981860521306,50.2459252805377));
#24576=CARTESIAN_POINT('Origin',(-32.,32.,39.4540747194623));
#24577=CARTESIAN_POINT('',(-29.9480290143483,32.0010746754496,48.8459252805377));
#24578=CARTESIAN_POINT('',(-29.9434378972346,31.9984640574522,48.9040747194623));
#24579=CARTESIAN_POINT('',(-29.94525,32.0000000000002,39.4540747194623));
#24580=CARTESIAN_POINT('Ctrl Pts',(-29.9434378972346,31.9984640574522,48.9040747194623));
#24581=CARTESIAN_POINT('Ctrl Pts',(-29.948302105761,32.5815526445705,48.9357696413457));
#24582=CARTESIAN_POINT('Ctrl Pts',(-30.5126875679984,33.8543562281369,49.0045078263022));
#24583=CARTESIAN_POINT('Ctrl Pts',(-32.6715753542565,34.3338806953585,49.110289274332));
#24584=CARTESIAN_POINT('Ctrl Pts',(-34.3249986620041,32.7017077584658,49.2214190635518));
#24585=CARTESIAN_POINT('Ctrl Pts',(-33.8506084078462,30.4273394907288,49.3325488527714));
#24586=CARTESIAN_POINT('Ctrl Pts',(-31.6825614078399,29.5922530662839,49.4436786419912));
#24587=CARTESIAN_POINT('Ctrl Pts',(-30.1534240551937,30.7067805031385,49.5341872642215));
#24588=CARTESIAN_POINT('Ctrl Pts',(-29.9475826256291,31.6953901112685,49.5876526233785));
#24589=CARTESIAN_POINT('Ctrl Pts',(-29.9484130486988,31.9993739458711,49.6040747194623));
#24590=CARTESIAN_POINT('Ctrl Pts',(-29.9480290143483,32.0010746754496,48.8459252805377));
#24591=CARTESIAN_POINT('Ctrl Pts',(-29.9467335107896,32.2742244015351,48.860688531892));
#24592=CARTESIAN_POINT('Ctrl Pts',(-30.1246039063867,33.2311300215956,48.9124950463196));
#24593=CARTESIAN_POINT('Ctrl Pts',(-31.5753615017921,34.3911703122827,49.0013448238203));
#24594=CARTESIAN_POINT('Ctrl Pts',(-33.7785362981989,33.6537297096236,49.1124746130401));
#24595=CARTESIAN_POINT('Ctrl Pts',(-34.354013961917,31.4028136106688,49.2236044022597));
#24596=CARTESIAN_POINT('Ctrl Pts',(-32.7751235759071,29.6984360190133,49.3347341914796));
#24597=CARTESIAN_POINT('Ctrl Pts',(-30.5628189733967,30.0870788403981,49.4421744842387));
#24598=CARTESIAN_POINT('Ctrl Pts',(-29.9468238243703,31.3881460374325,49.5125715139249));
#24599=CARTESIAN_POINT('Ctrl Pts',(-29.942679646097,32.0011604784324,49.5459252805377));
#24600=CARTESIAN_POINT('Origin',(-32.,32.,39.4540747194623));
#24601=CARTESIAN_POINT('',(-29.9465981926003,31.9982546442336,48.1459252805377));
#24602=CARTESIAN_POINT('',(-29.9436300851387,32.0016034367965,48.2040747194623));
#24603=CARTESIAN_POINT('',(-29.94525,32.0000000000002,39.4540747194623));
#24604=CARTESIAN_POINT('Ctrl Pts',(-29.9436300851387,32.0016034367965,48.2040747194624));
#24605=CARTESIAN_POINT('Ctrl Pts',(-29.9427254430368,32.1069589624514,48.2098001331663));
#24606=CARTESIAN_POINT('Ctrl Pts',(-29.9979858700552,32.8930102198204,48.2525688099435));
#24607=CARTESIAN_POINT('Ctrl Pts',(-31.0116628500012,34.2183782893241,48.3323807497939));
#24608=CARTESIAN_POINT('Ctrl Pts',(-33.3276175991793,34.0335791272928,48.4435105390137));
#24609=CARTESIAN_POINT('Ctrl Pts',(-34.4285511190019,31.9876704012107,48.5546403282334));
#24610=CARTESIAN_POINT('Ctrl Pts',(-33.3069009912542,29.9530455902315,48.6657701174531));
#24611=CARTESIAN_POINT('Ctrl Pts',(-30.9891892490617,29.7917712567763,48.7768999066728));
#24612=CARTESIAN_POINT('Ctrl Pts',(-29.9937470981767,31.1210534634512,48.8563347740093));
#24613=CARTESIAN_POINT('Ctrl Pts',(-29.9426170891911,31.9000711123825,48.8987263782724));
#24614=CARTESIAN_POINT('Ctrl Pts',(-29.9434378972346,31.9984640574522,48.9040747194623));
#24615=CARTESIAN_POINT('Ctrl Pts',(-29.9465981926003,31.9982546442336,48.1459252805377));
#24616=CARTESIAN_POINT('Ctrl Pts',(-29.9504520483336,32.4754533968064,48.1717622867859));
#24617=CARTESIAN_POINT('Ctrl Pts',(-30.3537536488506,33.6427001277731,48.2346425561073));
#24618=CARTESIAN_POINT('Ctrl Pts',(-32.2966122867217,34.4104013084688,48.3345660885019));
#24619=CARTESIAN_POINT('Ctrl Pts',(-34.1859029191172,33.0582257531821,48.4456958777217));
#24620=CARTESIAN_POINT('Ctrl Pts',(-34.0746789050666,30.7375734645635,48.5568256669414));
#24621=CARTESIAN_POINT('Ctrl Pts',(-32.064731256055,29.5722802507307,48.6679554561612));
#24622=CARTESIAN_POINT('Ctrl Pts',(-30.2704276691999,30.4884531134176,48.7643219940265));
#24623=CARTESIAN_POINT('Ctrl Pts',(-29.9499841280138,31.5888498238801,48.8236452688188));
#24624=CARTESIAN_POINT('Ctrl Pts',(-29.9480290143483,32.0010746754496,48.8459252805377));
#24625=CARTESIAN_POINT('Origin',(-32.,32.,39.4540747194623));
#24626=CARTESIAN_POINT('',(-29.9418536204177,31.9999545509509,47.4459252805377));
#24627=CARTESIAN_POINT('',(-29.9484710368218,32.0005167771498,47.5040747194623));
#24628=CARTESIAN_POINT('',(-29.94525,32.0000000000002,39.4540747194623));
#24629=CARTESIAN_POINT('Ctrl Pts',(-29.9484710368218,32.0005167771498,47.5040747194623));
#24630=CARTESIAN_POINT('Ctrl Pts',(-29.9477709447121,32.3115024180602,47.5208738880602));
#24631=CARTESIAN_POINT('Ctrl Pts',(-30.1602326581268,33.307323880596,47.5747163197312));
#24632=CARTESIAN_POINT('Ctrl Pts',(-31.7070250959598,34.4108459640165,47.6656020144756));
#24633=CARTESIAN_POINT('Ctrl Pts',(-33.8664811925721,33.5537890829796,47.7767318036953));
#24634=CARTESIAN_POINT('Ctrl Pts',(-34.317753942888,31.2747212833408,47.8878615929151));
#24635=CARTESIAN_POINT('Ctrl Pts',(-32.6478434196678,29.6594206998682,47.9989913821348));
#24636=CARTESIAN_POINT('Ctrl Pts',(-30.5016137267794,30.1590535721108,48.1043957576505));
#24637=CARTESIAN_POINT('Ctrl Pts',(-29.9485784515881,31.4253117217724,48.1727568700931));
#24638=CARTESIAN_POINT('Ctrl Pts',(-29.9436300851387,32.0016034367965,48.2040747194624));
#24639=CARTESIAN_POINT('Ctrl Pts',(-29.9418541045178,31.9999545574289,47.4459252805377));
#24640=CARTESIAN_POINT('Ctrl Pts',(-29.9420746139188,32.6776207454055,47.4828360416798));
#24641=CARTESIAN_POINT('Ctrl Pts',(-30.6782139520197,34.0357963423805,47.556790065895));
#24642=CARTESIAN_POINT('Ctrl Pts',(-32.9916833736669,34.2168846165047,47.6677873531836));
#24643=CARTESIAN_POINT('Ctrl Pts',(-34.4003366076938,32.3693203030807,47.7789171424033));
#24644=CARTESIAN_POINT('Ctrl Pts',(-33.6122278089259,30.1837580533892,47.890046931623));
#24645=CARTESIAN_POINT('Ctrl Pts',(-31.3486256033116,29.6604007369121,48.0011767208428));
#24646=CARTESIAN_POINT('Ctrl Pts',(-30.0688312378708,30.9020862296657,48.0864695038143));
#24647=CARTESIAN_POINT('Ctrl Pts',(-29.944926663914,31.7912797444886,48.1347190237126));
#24648=CARTESIAN_POINT('Ctrl Pts',(-29.9465981926003,31.9982546442336,48.1459252805377));
#24649=CARTESIAN_POINT('Origin',(-32.,32.,39.4540747194623));
#24650=CARTESIAN_POINT('',(-29.9464657716568,32.0017741341583,46.7459252805377));
#24651=CARTESIAN_POINT('',(-29.9455243558603,31.9981230673818,46.8040747194623));
#24652=CARTESIAN_POINT('',(-29.94525,32.0000000000002,39.4540747194623));
#24653=CARTESIAN_POINT('Ctrl Pts',(-29.9455243558603,31.9981230673818,46.8040747194623));
#24654=CARTESIAN_POINT('Ctrl Pts',(-29.950184034218,32.5122411663057,46.831947642954));
#24655=CARTESIAN_POINT('Ctrl Pts',(-30.4058569233675,33.7169899346219,46.896863829519));
#24656=CARTESIAN_POINT('Ctrl Pts',(-32.4282459959531,34.3905267042144,46.9988232791572));
#24657=CARTESIAN_POINT('Ctrl Pts',(-34.2406047664085,32.9368579600769,47.109953068377));
#24658=CARTESIAN_POINT('Ctrl Pts',(-34.0023863529936,30.6257869706786,47.2210828575967));
#24659=CARTESIAN_POINT('Ctrl Pts',(-31.9316056642948,29.5723808429954,47.3322126468164));
#24660=CARTESIAN_POINT('Ctrl Pts',(-30.2269905365809,30.5640931932684,47.4265432674383));
#24661=CARTESIAN_POINT('Ctrl Pts',(-29.949314693502,31.6257587849068,47.4838306249869));
#24662=CARTESIAN_POINT('Ctrl Pts',(-29.9484710368218,32.0005167771498,47.5040747194623));
#24663=CARTESIAN_POINT('Ctrl Pts',(-29.9464657716568,32.0017741341583,46.7459252805377));
#24664=CARTESIAN_POINT('Ctrl Pts',(-29.9447990356357,32.2038215525088,46.7568665335004));
#24665=CARTESIAN_POINT('Ctrl Pts',(-30.0649944313522,33.0879912801528,46.8048510495363));
#24666=CARTESIAN_POINT('Ctrl Pts',(-31.3319469323119,34.3348915210894,46.8898788286455));
#24667=CARTESIAN_POINT('Ctrl Pts',(-33.5992261538594,33.8277004747262,47.0010086178653));
#24668=CARTESIAN_POINT('Ctrl Pts',(-34.4029109422803,31.64781777448,47.1121384070849));
#24669=CARTESIAN_POINT('Ctrl Pts',(-33.0074776948103,29.7902484277724,47.2232681963048));
#24670=CARTESIAN_POINT('Ctrl Pts',(-30.6900117866906,29.9550197562096,47.3343979855244));
#24671=CARTESIAN_POINT('Ctrl Pts',(-29.9429588184216,31.3149910696256,47.4086170136021));
#24672=CARTESIAN_POINT('Ctrl Pts',(-29.9418533129351,31.9975218772071,47.4457927786065));
#24673=CARTESIAN_POINT('Ctrl Pts',(-29.9418541045178,31.9999545574289,47.4459252805377));
#24674=CARTESIAN_POINT('Origin',(-32.,32.,39.4540747194623));
#24675=CARTESIAN_POINT('',(-29.9481039578725,31.9989927018527,46.0459252805377));
#24676=CARTESIAN_POINT('',(-29.9420942235994,32.000637386216,46.1040747194623));
#24677=CARTESIAN_POINT('',(-29.94525,32.0000000000002,39.4540747194623));
#24678=CARTESIAN_POINT('Ctrl Pts',(-29.9420942235994,32.000637386216,46.1040747194623));
#24679=CARTESIAN_POINT('Ctrl Pts',(-29.9419518628081,32.0355942172137,46.1059781347746));
#24680=CARTESIAN_POINT('Ctrl Pts',(-29.9585993453337,32.7507240077201,46.1449248131603));
#24681=CARTESIAN_POINT('Ctrl Pts',(-30.7889831810305,34.1051011426497,46.2209147546192));
#24682=CARTESIAN_POINT('Ctrl Pts',(-33.1116688972156,34.1592139355736,46.3320445438388));
#24683=CARTESIAN_POINT('Ctrl Pts',(-34.4169672942162,32.2372375503608,46.4431743330586));
#24684=CARTESIAN_POINT('Ctrl Pts',(-33.510283434469,30.0981439317918,46.5543041222783));
#24685=CARTESIAN_POINT('Ctrl Pts',(-31.2214045538376,29.6996083620767,46.665433911498));
#24686=CARTESIAN_POINT('Ctrl Pts',(-30.0404503314131,30.9782872400902,46.7486907772261));
#24687=CARTESIAN_POINT('Ctrl Pts',(-29.9439912969799,31.8289754875258,46.7949043798808));
#24688=CARTESIAN_POINT('Ctrl Pts',(-29.9455243558603,31.9981230673818,46.8040747194623));
#24689=CARTESIAN_POINT('Ctrl Pts',(-29.9481039578725,31.9989927018527,46.0459252805377));
#24690=CARTESIAN_POINT('Ctrl Pts',(-29.9499107896978,32.4063516871941,46.0679402883943));
#24691=CARTESIAN_POINT('Ctrl Pts',(-30.2646015420902,33.5017208474256,46.1269985593241));
#24692=CARTESIAN_POINT('Ctrl Pts',(-32.0474055290543,34.4281198554267,46.2231000933271));
#24693=CARTESIAN_POINT('Ctrl Pts',(-34.0656174727299,33.2771991907512,46.3342298825469));
#24694=CARTESIAN_POINT('Ctrl Pts',(-34.1933987060518,30.9573996773486,46.4453596717666));
#24695=CARTESIAN_POINT('Ctrl Pts',(-32.3138052300136,29.5917766727069,46.5564894609864));
#24696=CARTESIAN_POINT('Ctrl Pts',(-30.3603507968393,30.3475933452302,46.6566779972433));
#24697=CARTESIAN_POINT('Ctrl Pts',(-29.9504420219658,31.5197595262729,46.7198232704271));
#24698=CARTESIAN_POINT('Ctrl Pts',(-29.9464657716568,32.0017741341583,46.7459252805377));
#24699=CARTESIAN_POINT('Origin',(-32.,32.,39.4540747194623));
#24700=CARTESIAN_POINT('',(-29.9427892494762,31.998771523558,45.3459252805377));
#24701=CARTESIAN_POINT('',(-29.9474011894601,32.0014721641163,45.4040747194623));
#24702=CARTESIAN_POINT('',(-29.94525,32.0000000000002,39.4540747194623));
#24703=CARTESIAN_POINT('Ctrl Pts',(-29.9474011894601,32.0014721641163,45.4040747194623));
#24704=CARTESIAN_POINT('Ctrl Pts',(-29.9458114267949,32.2413915495899,45.4170518896686));
#24705=CARTESIAN_POINT('Ctrl Pts',(-30.0955923589444,33.1642375601095,45.4670723229481));
#24706=CARTESIAN_POINT('Ctrl Pts',(-31.4608924203777,34.3679897749369,45.5541360193008));
#24707=CARTESIAN_POINT('Ctrl Pts',(-33.6969732872408,33.7373238670447,45.6652658085205));
#24708=CARTESIAN_POINT('Ctrl Pts',(-34.38000260453,31.5166779965259,45.7763955977402));
#24709=CARTESIAN_POINT('Ctrl Pts',(-32.8848793482069,29.7383631821778,45.88752538696));
#24710=CARTESIAN_POINT('Ctrl Pts',(-30.6194030558709,30.0248809034601,45.9967517608674));
#24711=CARTESIAN_POINT('Ctrl Pts',(-29.9447224133088,31.3552828429994,46.0689348717014));
#24712=CARTESIAN_POINT('Ctrl Pts',(-29.9420942235994,32.000637386216,46.1040747194623));
#24713=CARTESIAN_POINT('Ctrl Pts',(-29.9427892494762,31.998771523558,45.3459252805377));
#24714=CARTESIAN_POINT('Ctrl Pts',(-29.9470895693626,32.6070006515059,45.3790140432882));
#24715=CARTESIAN_POINT('Ctrl Pts',(-30.5546547810877,33.9036143174968,45.4491460691119));
#24716=CARTESIAN_POINT('Ctrl Pts',(-32.7586800023163,34.3070366209898,45.5563213580088));
#24717=CARTESIAN_POINT('Ctrl Pts',(-34.3496925356383,32.6139693025454,45.6674511472286));
#24718=CARTESIAN_POINT('Ctrl Pts',(-33.7902919416986,30.3590039366313,45.7785809364482));
#24719=CARTESIAN_POINT('Ctrl Pts',(-31.592435577624,29.605860372051,45.889710725668));
#24720=CARTESIAN_POINT('Ctrl Pts',(-30.129085316663,30.7589475750754,45.9788255070311));
#24721=CARTESIAN_POINT('Ctrl Pts',(-29.9468705479196,31.7209144546682,46.030897025321));
#24722=CARTESIAN_POINT('Ctrl Pts',(-29.9481039578725,31.9989927018527,46.0459252805377));
#24723=CARTESIAN_POINT('Origin',(-32.,32.,39.4540747194623));
#24724=CARTESIAN_POINT('',(-29.9443798519565,32.0017900284217,44.6459252805377));
#24725=CARTESIAN_POINT('',(-29.9474073584817,31.9985307398231,44.7040747194623));
#24726=CARTESIAN_POINT('',(-29.94525,32.0000000000002,39.4540747194623));
#24727=CARTESIAN_POINT('Ctrl Pts',(-29.9474073584817,31.9985307398231,44.7040747194623));
#24728=CARTESIAN_POINT('Ctrl Pts',(-29.9503473261682,32.443182900618,44.7281256445624));
#24729=CARTESIAN_POINT('Ctrl Pts',(-30.3107091275678,33.5770299650323,44.7892198327357));
#24730=CARTESIAN_POINT('Ctrl Pts',(-32.1803845625496,34.421874060765,44.8873572839825));
#24731=CARTESIAN_POINT('Ctrl Pts',(-34.1324988240748,33.1620935082564,44.9984870732021));
#24732=CARTESIAN_POINT('Ctrl Pts',(-34.1329732877935,30.8387775793711,45.109616862422));
#24733=CARTESIAN_POINT('Ctrl Pts',(-32.1813737296557,29.5781998169125,45.2207466516415));
#24734=CARTESIAN_POINT('Ctrl Pts',(-30.311064361793,30.4224106561746,45.3188992706551));
#24735=CARTESIAN_POINT('Ctrl Pts',(-29.9503493958354,31.5565429445996,45.3800086265953));
#24736=CARTESIAN_POINT('Ctrl Pts',(-29.9474011894601,32.0014721641163,45.4040747194623));
#24737=CARTESIAN_POINT('Ctrl Pts',(-29.9443798519565,32.0017900284217,44.6459252805377));
#24738=CARTESIAN_POINT('Ctrl Pts',(-29.9431807315765,32.1329178683255,44.6530445351087));
#24739=CARTESIAN_POINT('Ctrl Pts',(-30.0143464509196,32.9450400966092,44.6972070527531));
#24740=CARTESIAN_POINT('Ctrl Pts',(-31.0956022868993,34.2539028579429,44.7784128334708));
#24741=CARTESIAN_POINT('Ctrl Pts',(-33.4029915943473,33.9823289088073,44.8895426226903));
#24742=CARTESIAN_POINT('Ctrl Pts',(-34.4263782094584,31.8965490397939,45.0006724119102));
#24743=CARTESIAN_POINT('Ctrl Pts',(-33.2291698002495,29.9054463676817,45.1118022011298));
#24744=CARTESIAN_POINT('Ctrl Pts',(-30.9070385196435,29.8312564653792,45.2229319903496));
#24745=CARTESIAN_POINT('Ctrl Pts',(-29.9787574033648,31.1729920942033,45.3009730168189));
#24746=CARTESIAN_POINT('Ctrl Pts',(-29.9422753101516,31.926080915543,45.3419707802149));
#24747=CARTESIAN_POINT('Ctrl Pts',(-29.9427892494762,31.998771523558,45.3459252805377));
#24748=CARTESIAN_POINT('Origin',(-32.,32.,39.4540747194623));
#24749=CARTESIAN_POINT('',(-29.9485867435952,32.0000997951286,43.9459252805377));
#24750=CARTESIAN_POINT('',(-29.9420978996548,31.9993577750107,44.0040747194623));
#24751=CARTESIAN_POINT('',(-29.94525,32.0000000000002,39.4540747194623));
#24752=CARTESIAN_POINT('Ctrl Pts',(-29.9420978996548,31.9993577750107,44.0040747194623));
#24753=CARTESIAN_POINT('Ctrl Pts',(-29.9447426065428,32.6444368300436,44.0391993994563));
#24754=CARTESIAN_POINT('Ctrl Pts',(-30.6189110400326,33.9745949612775,44.1113673425235));
#24755=CARTESIAN_POINT('Ctrl Pts',(-32.883955539011,34.2619980463476,44.2205785486641));
#24756=CARTESIAN_POINT('Ctrl Pts',(-34.3798049995887,32.4842940434725,44.3317083378838));
#24757=CARTESIAN_POINT('Ctrl Pts',(-33.6976827324532,30.2633693839683,44.4428381271035));
#24758=CARTESIAN_POINT('Ctrl Pts',(-31.4618596391792,29.6317902312781,44.5539679163232));
#24759=CARTESIAN_POINT('Ctrl Pts',(-30.0958300942565,30.8351943211461,44.6410467804429));
#24760=CARTESIAN_POINT('Ctrl Pts',(-29.9458191844862,31.7583291205725,44.6910823814892));
#24761=CARTESIAN_POINT('Ctrl Pts',(-29.9474073584817,31.9985307398231,44.7040747194623));
#24762=CARTESIAN_POINT('Ctrl Pts',(-29.9485867435952,32.0000997951286,43.9459252805377));
#24763=CARTESIAN_POINT('Ctrl Pts',(-29.9484407938114,32.3369356488425,43.9641182900026));
#24764=CARTESIAN_POINT('Ctrl Pts',(-30.1862446142337,33.3594177249809,44.0193545625408));
#24765=CARTESIAN_POINT('Ctrl Pts',(-31.7976970844419,34.4201419063721,44.1116340981524));
#24766=CARTESIAN_POINT('Ctrl Pts',(-33.9234718487822,33.4826561851773,44.2227638873721));
#24767=CARTESIAN_POINT('Ctrl Pts',(-34.2889060362689,31.1882596020868,44.3338936765918));
#24768=CARTESIAN_POINT('Ctrl Pts',(-32.5595582415307,29.6367590281872,44.4450234658115));
#24769=CARTESIAN_POINT('Ctrl Pts',(-30.4617017157523,30.2089087790966,44.5490340004602));
#24770=CARTESIAN_POINT('Ctrl Pts',(-29.9494200549846,31.4506269035521,44.6160012720355));
#24771=CARTESIAN_POINT('Ctrl Pts',(-29.9443798519565,32.0017900284217,44.6459252805377));
#24772=CARTESIAN_POINT('Origin',(-32.,32.,39.4540747194623));
#24773=CARTESIAN_POINT('',(-29.9447460822062,31.9981575528504,43.2459252805377));
#24774=CARTESIAN_POINT('',(-29.9455159804426,32.0018771150079,43.3040747194623));
#24775=CARTESIAN_POINT('',(-29.94525,32.0000000000002,39.4540747194623));
#24776=CARTESIAN_POINT('Ctrl Pts',(-29.9455159804426,32.0018771150079,43.3040747194623));
#24777=CARTESIAN_POINT('Ctrl Pts',(-29.9439847655777,32.1707431684077,43.3132298912769));
#24778=CARTESIAN_POINT('Ctrl Pts',(-30.0402482414051,33.0211453613684,43.3594283261648));
#24779=CARTESIAN_POINT('Ctrl Pts',(-31.2204650545239,34.3000734386756,43.442670024126));
#24780=CARTESIAN_POINT('Ctrl Pts',(-33.5095065207455,33.9024727649217,43.5537998133457));
#24781=CARTESIAN_POINT('Ctrl Pts',(-34.4170639891342,31.7637496473617,43.6649296025654));
#24782=CARTESIAN_POINT('Ctrl Pts',(-33.1125507066162,29.841240290916,43.7760593917852));
#24783=CARTESIAN_POINT('Ctrl Pts',(-30.7898430825224,29.8944044092436,43.8871891810048));
#24784=CARTESIAN_POINT('Ctrl Pts',(-29.9587402818909,31.2487125411017,43.9631942902306));
#24785=CARTESIAN_POINT('Ctrl Pts',(-29.9419534402637,31.9641222152855,44.0021561363831));
#24786=CARTESIAN_POINT('Ctrl Pts',(-29.9420978996548,31.9993577750107,44.0040747194623));
#24787=CARTESIAN_POINT('Ctrl Pts',(-29.9447460822062,31.9981575528504,43.2459252805377));
#24788=CARTESIAN_POINT('Ctrl Pts',(-29.9497235697248,32.5374622374985,43.2751920448966));
#24789=CARTESIAN_POINT('Ctrl Pts',(-30.4434354700877,33.7674364415726,43.3415020723286));
#24790=CARTESIAN_POINT('Ctrl Pts',(-32.5176476120498,34.372773539922,43.4448553628341));
#24791=CARTESIAN_POINT('Ctrl Pts',(-34.2741819548352,32.8521207391232,43.5559851520537));
#24792=CARTESIAN_POINT('Ctrl Pts',(-33.9494096331178,30.5516162812554,43.6671149412735));
#24793=CARTESIAN_POINT('Ctrl Pts',(-31.8405587566049,29.5766568944465,43.7782447304931));
#24794=CARTESIAN_POINT('Ctrl Pts',(-30.1989775173142,30.6160471049063,43.871181510248));
#24795=CARTESIAN_POINT('Ctrl Pts',(-29.9487379659889,31.6510953448708,43.9270750269294));
#24796=CARTESIAN_POINT('Ctrl Pts',(-29.9485867435952,32.0000997951286,43.9459252805377));
#24797=CARTESIAN_POINT('Origin',(-32.,32.,39.4540747194623));
#24798=CARTESIAN_POINT('',(-29.94252702357,32.0010548525627,42.5459252805377));
#24799=CARTESIAN_POINT('',(-29.9484731362167,31.9994876359286,42.6040747194623));
#24800=CARTESIAN_POINT('',(-29.94525,32.0000000000002,39.4540747194623));
#24801=CARTESIAN_POINT('Ctrl Pts',(-29.9484731362167,31.9994876359286,42.6040747194623));
#24802=CARTESIAN_POINT('Ctrl Pts',(-29.9493088732493,32.3739658106449,42.6243036461709));
#24803=CARTESIAN_POINT('Ctrl Pts',(-30.2266782317794,33.4353421391061,42.6815758359526));
#24804=CARTESIAN_POINT('Ctrl Pts',(-31.9306141425706,34.4275909928101,42.7758912888076));
#24805=CARTESIAN_POINT('Ctrl Pts',(-34.0018249063725,33.3750307763075,42.8870210780274));
#24806=CARTESIAN_POINT('Ctrl Pts',(-34.2409872269693,31.0640572563152,42.998150867247));
#24807=CARTESIAN_POINT('Ctrl Pts',(-32.4292223388168,29.6096484100191,43.1092806564668));
#24808=CARTESIAN_POINT('Ctrl Pts',(-30.4062574409955,30.2824591750793,43.2112552738719));
#24809=CARTESIAN_POINT('Ctrl Pts',(-29.9501803014138,31.4874845942514,43.2761866282037));
#24810=CARTESIAN_POINT('Ctrl Pts',(-29.9455159804426,32.0018771150079,43.3040747194623));
#24811=CARTESIAN_POINT('Ctrl Pts',(-29.94252702357,32.0010548525627,42.5459252805377));
#24812=CARTESIAN_POINT('Ctrl Pts',(-29.9421477088781,32.0616438365238,42.5492225367172));
#24813=CARTESIAN_POINT('Ctrl Pts',(-29.9720545786143,32.8025444028162,42.58956305597));
#24814=CARTESIAN_POINT('Ctrl Pts',(-30.8688288986318,34.1490612499125,42.6669468382959));
#24815=CARTESIAN_POINT('Ctrl Pts',(-33.1919092821327,34.1159786819058,42.7780766275156));
#24816=CARTESIAN_POINT('Ctrl Pts',(-34.4241674445136,32.1463750716222,42.8892064167354));
#24817=CARTESIAN_POINT('Ctrl Pts',(-33.4378537354262,30.0428107344064,43.0003362059551));
#24818=CARTESIAN_POINT('Ctrl Pts',(-31.1356319387654,29.7304447118329,43.1114659951747));
#24819=CARTESIAN_POINT('Ctrl Pts',(-30.0224447689381,31.0304040223966,43.1933290200357));
#24820=CARTESIAN_POINT('Ctrl Pts',(-29.943423509447,31.8548584120434,43.2381487818233));
#24821=CARTESIAN_POINT('Ctrl Pts',(-29.9447460822062,31.9981575528504,43.2459252805377));
#24822=CARTESIAN_POINT('Origin',(-32.,32.,39.4540747194623));
#24823=CARTESIAN_POINT('',(-29.9479126851747,32.0011660315207,41.8459252805377));
#24824=CARTESIAN_POINT('',(-29.9436380261218,31.9983919808556,41.9040747194623));
#24825=CARTESIAN_POINT('',(-29.94525,32.0000000000002,39.4540747194623));
#24826=CARTESIAN_POINT('Ctrl Pts',(-29.9436380261218,31.9983919808556,41.9040747194623));
#24827=CARTESIAN_POINT('Ctrl Pts',(-29.9485892245779,32.5744100804168,41.9353774010647));
#24828=CARTESIAN_POINT('Ctrl Pts',(-30.5011706211881,33.8404092621993,42.0037233457404));
#24829=CARTESIAN_POINT('Ctrl Pts',(-32.6468874612962,34.3408420864571,42.1091125534892));
#24830=CARTESIAN_POINT('Ctrl Pts',(-34.3174574817349,32.7262261309694,42.220242342709));
#24831=CARTESIAN_POINT('Ctrl Pts',(-33.8671156802116,30.446972972158,42.3313721319287));
#24832=CARTESIAN_POINT('Ctrl Pts',(-31.708009788722,29.5890347844302,42.4425019211484));
#24833=CARTESIAN_POINT('Ctrl Pts',(-30.1605085558978,30.6921088112584,42.5334027836596));
#24834=CARTESIAN_POINT('Ctrl Pts',(-29.9477784694269,31.6882204055088,42.5872603830976));
#24835=CARTESIAN_POINT('Ctrl Pts',(-29.9484731362167,31.9994876359286,42.6040747194623));
#24836=CARTESIAN_POINT('Ctrl Pts',(-29.9479126851747,32.0011660315207,41.8459252805377));
#24837=CARTESIAN_POINT('Ctrl Pts',(-29.9465311135547,32.2670233657638,41.8602962916111));
#24838=CARTESIAN_POINT('Ctrl Pts',(-30.1180449698071,33.2164556126041,41.9117105657577));
#24839=CARTESIAN_POINT('Ctrl Pts',(-31.5501372064992,34.3865418916543,42.0001681029775));
#24840=CARTESIAN_POINT('Ctrl Pts',(-33.7609665083167,33.6724274609132,42.1112978921974));
#24841=CARTESIAN_POINT('Ctrl Pts',(-34.3601920973369,31.4277075251964,42.2224276814169));
#24842=CARTESIAN_POINT('Ctrl Pts',(-32.7993885345327,29.7067525630187,42.3335574706368));
#24843=CARTESIAN_POINT('Ctrl Pts',(-30.5750127520012,30.0733388697254,42.4413900036769));
#24844=CARTESIAN_POINT('Ctrl Pts',(-29.9464091472235,31.3809525131846,42.5121792736439));
#24845=CARTESIAN_POINT('Ctrl Pts',(-29.94252702357,32.0010548525627,42.5459252805377));
#24846=CARTESIAN_POINT('Origin',(-32.,32.,39.4540747194623));
#24847=CARTESIAN_POINT('',(-29.9473238061977,31.9976393779993,41.1459252805377));
#24848=CARTESIAN_POINT('',(-29.9434322456991,32.0014925908821,41.2040747194623));
#24849=CARTESIAN_POINT('',(-29.94525,32.0000000000002,39.4540747194623));
#24850=CARTESIAN_POINT('',(-31.4698297828114,30.0148256743283,41.));
#24851=CARTESIAN_POINT('Ctrl Pts',(-31.4698297828114,30.0148256743283,41.));
#24852=CARTESIAN_POINT('Ctrl Pts',(-30.8097602092473,30.1911070339301,41.0370432630732));
#24853=CARTESIAN_POINT('Ctrl Pts',(-30.0750747235939,30.8871231756006,41.0856850232525));
#24854=CARTESIAN_POINT('Ctrl Pts',(-29.9457054452028,31.7833432379,41.1343267834317));
#24855=CARTESIAN_POINT('Ctrl Pts',(-29.9473238061977,31.9976393779993,41.1459252805377));
#24856=CARTESIAN_POINT('',(-32.5313020758336,30.0112666986537,41.));
#24857=CARTESIAN_POINT('Origin',(-32.,32.,41.));
#24858=CARTESIAN_POINT('Ctrl Pts',(-32.5313026984106,30.0112647410448,41.));
#24859=CARTESIAN_POINT('Ctrl Pts',(-31.8868328863034,29.8399813018842,41.0363148168372));
#24860=CARTESIAN_POINT('Ctrl Pts',(-30.5071217606431,30.1592363627283,41.1043397233247));
#24861=CARTESIAN_POINT('Ctrl Pts',(-29.94828636835,31.4182664903594,41.1723646298121));
#24862=CARTESIAN_POINT('Ctrl Pts',(-29.9434322456991,32.0014925908821,41.2040747194623));
#24863=CARTESIAN_POINT('Origin',(-32.,-32.,48.));
#24864=CARTESIAN_POINT('',(-30.3315194597827,-31.9993859147877,53.3285196366098));
#24865=CARTESIAN_POINT('',(-30.3351880693888,-31.9985150917772,53.5214803633902));
#24866=CARTESIAN_POINT('',(-30.334,-32.,48.));
#24867=CARTESIAN_POINT('',(-32.6750771856749,-33.5230977622534,54.));
#24868=CARTESIAN_POINT('Ctrl Pts',(-30.3351880693888,-31.9985150917772,
53.5214803633902));
#24869=CARTESIAN_POINT('Ctrl Pts',(-30.3338369362185,-31.8287716445104,
53.5328138566338));
#24870=CARTESIAN_POINT('Ctrl Pts',(-30.3577131426661,-31.6594109347466,
53.5441473498775));
#24871=CARTESIAN_POINT('Ctrl Pts',(-30.4083948376391,-31.4985170933091,
53.5554808431211));
#24872=CARTESIAN_POINT('Ctrl Pts',(-30.5740467967946,-30.9726392578427,
53.5925241061943));
#24873=CARTESIAN_POINT('Ctrl Pts',(-31.0260602491034,-30.5372124900351,
53.6295673692676));
#24874=CARTESIAN_POINT('Ctrl Pts',(-31.5578576005161,-30.3909994562276,
53.6666106323408));
#24875=CARTESIAN_POINT('Ctrl Pts',(-32.0896549519289,-30.2447864224201,
53.703653895414));
#24876=CARTESIAN_POINT('Ctrl Pts',(-32.7012362024457,-30.3877871226129,
53.7406971584873));
#24877=CARTESIAN_POINT('Ctrl Pts',(-33.1122249699019,-30.7555548361959,
53.7777404215605));
#24878=CARTESIAN_POINT('Ctrl Pts',(-33.5232137373581,-31.1233225497789,
53.8147836846338));
#24879=CARTESIAN_POINT('Ctrl Pts',(-33.7336100217538,-31.7158572767522,
53.851826947707));
#24880=CARTESIAN_POINT('Ctrl Pts',(-33.6481832146636,-32.2596853644512,
53.8888702107803));
#24881=CARTESIAN_POINT('Ctrl Pts',(-33.5627564075734,-32.8035134521501,
53.9259134738535));
#24882=CARTESIAN_POINT('Ctrl Pts',(-33.1815065089974,-33.2986349005747,
53.9629567369268));
#24883=CARTESIAN_POINT('Ctrl Pts',(-32.6750771856749,-33.5230977622534,
54.));
#24884=CARTESIAN_POINT('',(-30.334,-32.,54.));
#24885=CARTESIAN_POINT('Origin',(-32.,-32.,54.));
#24886=CARTESIAN_POINT('',(-30.334,-32.,55.));
#24887=CARTESIAN_POINT('',(-30.334,-32.,48.));
#24888=CARTESIAN_POINT('Origin',(-32.,-32.,55.));
#24889=CARTESIAN_POINT('',(-30.3853283529176,-32.4224677305593,54.));
#24890=CARTESIAN_POINT('Origin',(-32.,-32.,54.));
#24891=CARTESIAN_POINT('Ctrl Pts',(-30.3853267233299,-32.4224680762712,
54.));
#24892=CARTESIAN_POINT('Ctrl Pts',(-30.5228595190938,-32.9453624125461,
53.9636851831628));
#24893=CARTESIAN_POINT('Ctrl Pts',(-30.9381524233032,-33.3962238017523,
53.9273703663256));
#24894=CARTESIAN_POINT('Ctrl Pts',(-31.4484748430102,-33.5748624385682,
53.8910555494883));
#24895=CARTESIAN_POINT('Ctrl Pts',(-31.9690339230712,-33.7570844238332,
53.8540122864151));
#24896=CARTESIAN_POINT('Ctrl Pts',(-32.5884731882451,-33.6560529798102,
53.8169690233418));
#24897=CARTESIAN_POINT('Ctrl Pts',(-33.0238322933555,-33.3177477726804,
53.7799257602686));
#24898=CARTESIAN_POINT('Ctrl Pts',(-33.4591913984659,-32.9794425655507,
53.7428824971953));
#24899=CARTESIAN_POINT('Ctrl Pts',(-33.7104703435129,-32.4038635953142,
53.7058392341221));
#24900=CARTESIAN_POINT('Ctrl Pts',(-33.6624375968578,-31.8545189772709,
53.6687959710488));
#24901=CARTESIAN_POINT('Ctrl Pts',(-33.6144048502027,-31.3051743592277,
53.6317527079756));
#24902=CARTESIAN_POINT('Ctrl Pts',(-33.2670604118455,-30.7820640933777,
53.5947094449024));
#24903=CARTESIAN_POINT('Ctrl Pts',(-32.7794722575826,-30.5244968713596,
53.5576661818291));
#24904=CARTESIAN_POINT('Ctrl Pts',(-32.2918841033197,-30.2669296493415,
53.5206229187559));
#24905=CARTESIAN_POINT('Ctrl Pts',(-31.6640522331509,-30.2749054711554,
53.4835796556826));
#24906=CARTESIAN_POINT('Ctrl Pts',(-31.1832059423421,-30.5448068325208,
53.4465363926094));
#24907=CARTESIAN_POINT('Ctrl Pts',(-30.7023596515333,-30.8147081938862,
53.4094931295362));
#24908=CARTESIAN_POINT('Ctrl Pts',(-30.3684989400844,-31.3465350948031,
53.3724498664629));
#24909=CARTESIAN_POINT('Ctrl Pts',(-30.3344285679539,-31.8969101687342,
53.3354066033897));
#24910=CARTESIAN_POINT('Ctrl Pts',(-30.3323171492003,-31.9310181687335,
53.3331109477964));
#24911=CARTESIAN_POINT('Ctrl Pts',(-30.3313570944005,-31.9651974041764,
53.3308152922031));
#24912=CARTESIAN_POINT('Ctrl Pts',(-30.3315194597827,-31.9993859147877,
53.3285196366098));
#24913=CARTESIAN_POINT('Origin',(-32.,-32.,48.));
#24914=CARTESIAN_POINT('',(-30.3358699316178,-31.9988695644631,52.6285196366098));
#24915=CARTESIAN_POINT('',(-30.3362229116815,-32.0008964522951,52.8214803633902));
#24916=CARTESIAN_POINT('',(-30.334,-32.,48.));
#24917=CARTESIAN_POINT('Ctrl Pts',(-30.3362229116815,-32.0008964522951,
52.8214803633902));
#24918=CARTESIAN_POINT('Ctrl Pts',(-30.3378663217269,-31.664768858379,52.8438876115277));
#24919=CARTESIAN_POINT('Ctrl Pts',(-30.436643420233,-31.3277533378251,52.8662948596652));
#24920=CARTESIAN_POINT('Ctrl Pts',(-30.6259117017676,-31.0530980531767,
52.8887021078027));
#24921=CARTESIAN_POINT('Ctrl Pts',(-30.9388066499237,-30.5990428340239,
52.925745370876));
#24922=CARTESIAN_POINT('Ctrl Pts',(-31.499015022336,-30.3154188432304,52.9627886339492));
#24923=CARTESIAN_POINT('Ctrl Pts',(-32.0501928398437,-30.332002852775,52.9998318970224));
#24924=CARTESIAN_POINT('Ctrl Pts',(-32.6013706573514,-30.3485868623195,
53.0368751600957));
#24925=CARTESIAN_POINT('Ctrl Pts',(-33.1435179199545,-30.6653788722021,
53.073918423169));
#24926=CARTESIAN_POINT('Ctrl Pts',(-33.4285423983798,-31.1374324713373,
53.1109616862422));
#24927=CARTESIAN_POINT('Ctrl Pts',(-33.713566876805,-31.6094860704725,53.1480049493154));
#24928=CARTESIAN_POINT('Ctrl Pts',(-33.7414685710525,-32.2368012588603,
53.1850482123887));
#24929=CARTESIAN_POINT('Ctrl Pts',(-33.4994968073952,-32.7322905380902,
53.2220914754619));
#24930=CARTESIAN_POINT('Ctrl Pts',(-33.257525043738,-33.2277798173201,53.2591347385351));
#24931=CARTESIAN_POINT('Ctrl Pts',(-32.745679822176,-33.5914431873922,53.2961780016084));
#24932=CARTESIAN_POINT('Ctrl Pts',(-32.1981451023726,-33.6569325686885,
53.3332212646817));
#24933=CARTESIAN_POINT('Ctrl Pts',(-31.6506103825692,-33.7224219499848,
53.3702645277549));
#24934=CARTESIAN_POINT('Ctrl Pts',(-31.0673861645244,-33.4897373425053,
53.4073077908281));
#24935=CARTESIAN_POINT('Ctrl Pts',(-30.715419288503,-33.065230587203,53.4443510539014));
#24936=CARTESIAN_POINT('Ctrl Pts',(-30.4711376939722,-32.7706028988063,
53.470060823731));
#24937=CARTESIAN_POINT('Ctrl Pts',(-30.3382530840379,-32.3835742139296,
53.4957705935606));
#24938=CARTESIAN_POINT('Ctrl Pts',(-30.3351880693888,-31.9985150917772,
53.5214803633902));
#24939=CARTESIAN_POINT('Ctrl Pts',(-30.3315194597827,-31.9993859147877,
53.3285196366098));
#24940=CARTESIAN_POINT('Ctrl Pts',(-30.3339770621283,-32.5168716171368,
53.2937720291299));
#24941=CARTESIAN_POINT('Ctrl Pts',(-30.5935877940968,-33.0364823156352,
53.2590244216499));
#24942=CARTESIAN_POINT('Ctrl Pts',(-31.0099803338461,-33.3433519309553,
53.2242768141699));
#24943=CARTESIAN_POINT('Ctrl Pts',(-31.4538825046809,-33.6704953723,53.1872335510967));
#24944=CARTESIAN_POINT('Ctrl Pts',(-32.0759668791627,-33.7558590080441,
53.1501902880235));
#24945=CARTESIAN_POINT('Ctrl Pts',(-32.5915791638324,-33.5603767516504,
53.1131470249502));
#24946=CARTESIAN_POINT('Ctrl Pts',(-33.1071914485022,-33.3648944952568,
53.076103761877));
#24947=CARTESIAN_POINT('Ctrl Pts',(-33.5163316433599,-32.8885663467255,
53.0390604988037));
#24948=CARTESIAN_POINT('Ctrl Pts',(-33.6317752999571,-32.3493595803674,
53.0020172357305));
#24949=CARTESIAN_POINT('Ctrl Pts',(-33.7472189565544,-31.8101528140094,
52.9649739726572));
#24950=CARTESIAN_POINT('Ctrl Pts',(-33.5689660748913,-31.2080674298246,
52.927930709584));
#24951=CARTESIAN_POINT('Ctrl Pts',(-33.1785862852529,-30.8186133759292,
52.8908874465108));
#24952=CARTESIAN_POINT('Ctrl Pts',(-32.7882064956146,-30.4291593220338,
52.8538441834375));
#24953=CARTESIAN_POINT('Ctrl Pts',(-32.1856997980011,-30.2523365984278,
52.8168009203643));
#24954=CARTESIAN_POINT('Ctrl Pts',(-31.6467689404394,-30.3690588596417,
52.779757657291));
#24955=CARTESIAN_POINT('Ctrl Pts',(-31.1078380828777,-30.4857811208556,
52.7427143942178));
#24956=CARTESIAN_POINT('Ctrl Pts',(-30.6324830653677,-30.8960483668895,
52.7056711311446));
#24957=CARTESIAN_POINT('Ctrl Pts',(-30.4382242967739,-31.4121242602753,
52.6686278680713));
#24958=CARTESIAN_POINT('Ctrl Pts',(-30.3681137016859,-31.5983829720839,
52.6552584575841));
#24959=CARTESIAN_POINT('Ctrl Pts',(-30.3346182799052,-31.798424158668,52.641889047097));
#24960=CARTESIAN_POINT('Ctrl Pts',(-30.3358699316178,-31.9988695644631,
52.6285196366098));
#24961=CARTESIAN_POINT('Origin',(-32.,-32.,48.));
#24962=CARTESIAN_POINT('',(-30.3356164490944,-32.001249815539,51.9285196366098));
#24963=CARTESIAN_POINT('',(-30.3318747247521,-32.0009136526746,52.1214803633902));
#24964=CARTESIAN_POINT('',(-30.334,-32.,48.));
#24965=CARTESIAN_POINT('Ctrl Pts',(-30.3318747247521,-32.0009136526746,
52.1214803633902));
#24966=CARTESIAN_POINT('Ctrl Pts',(-30.335169241692,-31.5020153100613,52.1549613664216));
#24967=CARTESIAN_POINT('Ctrl Pts',(-30.5738487645137,-31.0003825576738,
52.188442369453));
#24968=CARTESIAN_POINT('Ctrl Pts',(-30.9647448300847,-30.6911882331788,
52.2219233724844));
#24969=CARTESIAN_POINT('Ctrl Pts',(-31.3972308514164,-30.3490967285641,
52.2589666355576));
#24970=CARTESIAN_POINT('Ctrl Pts',(-32.0160471392396,-30.2425716276057,
52.2960098986309));
#24971=CARTESIAN_POINT('Ctrl Pts',(-32.5380267876055,-30.4203581055947,
52.3330531617041));
#24972=CARTESIAN_POINT('Ctrl Pts',(-33.0600064359714,-30.5981445835838,
52.3700964247774));
#24973=CARTESIAN_POINT('Ctrl Pts',(-33.48514944488,-31.0602426405203,52.4071396878506));
#24974=CARTESIAN_POINT('Ctrl Pts',(-33.6189125362116,-31.5951989750851,
52.4441829509238));
#24975=CARTESIAN_POINT('Ctrl Pts',(-33.7526756275432,-32.1301553096499,
52.4812262139971));
#24976=CARTESIAN_POINT('Ctrl Pts',(-33.5950588012977,-32.7379699218431,
52.5182694770703));
#24977=CARTESIAN_POINT('Ctrl Pts',(-33.2181869446231,-33.1405096183543,
52.5553127401436));
#24978=CARTESIAN_POINT('Ctrl Pts',(-32.8413150879486,-33.5430493148655,
52.5923560032168));
#24979=CARTESIAN_POINT('Ctrl Pts',(-32.2451882008448,-33.7403140956948,
52.62939926629));
#24980=CARTESIAN_POINT('Ctrl Pts',(-31.7025901559714,-33.6420377012477,
52.6664425293633));
#24981=CARTESIAN_POINT('Ctrl Pts',(-31.159992111098,-33.5437613068006,52.7034857924365));
#24982=CARTESIAN_POINT('Ctrl Pts',(-30.6709229084549,-33.149943737077,52.7405290555098));
#24983=CARTESIAN_POINT('Ctrl Pts',(-30.4591790690833,-32.6407917284592,
52.777572318583));
#24984=CARTESIAN_POINT('Ctrl Pts',(-30.3755178109089,-32.4396227226955,
52.7922083335188));
#24985=CARTESIAN_POINT('Ctrl Pts',(-30.3351494655438,-32.2204490030893,
52.8068443484545));
#24986=CARTESIAN_POINT('Ctrl Pts',(-30.3362229116815,-32.0008964522951,
52.8214803633902));
#24987=CARTESIAN_POINT('Ctrl Pts',(-30.3358699316178,-31.9988695644631,
52.6285196366098));
#24988=CARTESIAN_POINT('Ctrl Pts',(-30.3380862909825,-32.3538078014858,
52.6048457840237));
#24989=CARTESIAN_POINT('Ctrl Pts',(-30.4492537442715,-32.7100134869809,
52.5811719314377));
#24990=CARTESIAN_POINT('Ctrl Pts',(-30.659000109678,-32.9932070252068,52.5574980788516));
#24991=CARTESIAN_POINT('Ctrl Pts',(-30.9871972108535,-33.4363293560148,
52.5204548157783));
#24992=CARTESIAN_POINT('Ctrl Pts',(-31.5567539328823,-33.7006894768929,
52.4834115527051));
#24993=CARTESIAN_POINT('Ctrl Pts',(-32.1070443434056,-33.6653175609879,
52.4463682896319));
#24994=CARTESIAN_POINT('Ctrl Pts',(-32.6573347539289,-33.6299456450829,
52.4093250265586));
#24995=CARTESIAN_POINT('Ctrl Pts',(-33.1883588529469,-33.2948416923949,
52.3722817634853));
#24996=CARTESIAN_POINT('Ctrl Pts',(-33.4571228237319,-32.8133474894917,
52.3352385004121));
#24997=CARTESIAN_POINT('Ctrl Pts',(-33.7258867945169,-32.3318532865884,
52.2981952373388));
#24998=CARTESIAN_POINT('Ctrl Pts',(-33.7323906370689,-31.7039688334699,
52.2611519742656));
#24999=CARTESIAN_POINT('Ctrl Pts',(-33.4736582628434,-31.2170106337195,
52.2241087111924));
#25000=CARTESIAN_POINT('Ctrl Pts',(-33.2149258886179,-30.7300524339691,
52.1870654481192));
#25001=CARTESIAN_POINT('Ctrl Pts',(-32.6909572976149,-30.3840204875868,
52.1500221850459));
#25002=CARTESIAN_POINT('Ctrl Pts',(-32.1415176585263,-30.3372571458491,
52.1129789219727));
#25003=CARTESIAN_POINT('Ctrl Pts',(-31.5920780194377,-30.2904938041115,
52.0759356588994));
#25004=CARTESIAN_POINT('Ctrl Pts',(-31.0171673322635,-30.5429990670185,
52.0388923958262));
#25005=CARTESIAN_POINT('Ctrl Pts',(-30.6798616189464,-30.9792278909246,
52.001849132753));
#25006=CARTESIAN_POINT('Ctrl Pts',(-30.4572889120474,-31.2670754616322,
51.9774059673719));
#25007=CARTESIAN_POINT('Ctrl Pts',(-30.3381713154789,-31.6349177435823,
51.9529628019908));
#25008=CARTESIAN_POINT('Ctrl Pts',(-30.3356164490944,-32.001249815539,51.9285196366098));
#25009=CARTESIAN_POINT('Origin',(-32.,-32.,48.));
#25010=CARTESIAN_POINT('',(-30.3313738033598,-32.0004179151157,51.2285196366098));
#25011=CARTESIAN_POINT('',(-30.3334712707803,-31.9985210140748,51.4214803633902));
#25012=CARTESIAN_POINT('',(-30.334,-32.,48.));
#25013=CARTESIAN_POINT('Ctrl Pts',(-30.3334712707803,-31.9985210140748,
51.4214803633902));
#25014=CARTESIAN_POINT('Ctrl Pts',(-30.3324380179584,-31.8863136363627,
51.4289918582422));
#25015=CARTESIAN_POINT('Ctrl Pts',(-30.342802950118,-31.7742960662403,51.4365033530942));
#25016=CARTESIAN_POINT('Ctrl Pts',(-30.3652659897465,-31.6647594964407,
51.4440148479463));
#25017=CARTESIAN_POINT('Ctrl Pts',(-30.476043445203,-31.1245751455012,51.4810581110195));
#25018=CARTESIAN_POINT('Ctrl Pts',(-30.8810483331414,-30.6447290215782,
51.5181013740928));
#25019=CARTESIAN_POINT('Ctrl Pts',(-31.394952612285,-30.4447961102396,51.555144637166));
#25020=CARTESIAN_POINT('Ctrl Pts',(-31.9088568914286,-30.244863198901,51.5921879002393));
#25021=CARTESIAN_POINT('Ctrl Pts',(-32.5316605617774,-30.3248435001467,
51.6292311633125));
#25022=CARTESIAN_POINT('Ctrl Pts',(-32.9783720419871,-30.6481384595887,
51.6662744263857));
#25023=CARTESIAN_POINT('Ctrl Pts',(-33.4250835221967,-30.9714334190306,
51.703317689459));
#25024=CARTESIAN_POINT('Ctrl Pts',(-33.6957028122672,-31.5380430366686,
51.7403609525323));
#25025=CARTESIAN_POINT('Ctrl Pts',(-33.6663959900684,-32.0886898281663,
51.7774042156055));
#25026=CARTESIAN_POINT('Ctrl Pts',(-33.6370891678696,-32.639336619664,51.8144474786788));
#25027=CARTESIAN_POINT('Ctrl Pts',(-33.3078562334017,-33.1740205850213,
51.8514907417519));
#25028=CARTESIAN_POINT('Ctrl Pts',(-32.8293523969697,-33.4480732322182,
51.8885340048252));
#25029=CARTESIAN_POINT('Ctrl Pts',(-32.3508485605377,-33.7221258794152,
51.9255772678984));
#25030=CARTESIAN_POINT('Ctrl Pts',(-31.7230738221416,-33.7355472084518,
51.9626205309717));
#25031=CARTESIAN_POINT('Ctrl Pts',(-31.2332944888314,-33.4821957091113,
51.9996637940449));
#25032=CARTESIAN_POINT('Ctrl Pts',(-30.7435151555213,-33.2288442097708,
52.0367070571182));
#25033=CARTESIAN_POINT('Ctrl Pts',(-30.3917312272969,-32.7087198820532,
52.0737503201914));
#25034=CARTESIAN_POINT('Ctrl Pts',(-30.3389171406048,-32.1598287640589,
52.1107935832647));
#25035=CARTESIAN_POINT('Ctrl Pts',(-30.3338382815881,-32.1070447289945,
52.1143558433065));
#25036=CARTESIAN_POINT('Ctrl Pts',(-30.3315241998278,-32.0539946678751,
52.1179181033483));
#25037=CARTESIAN_POINT('Ctrl Pts',(-30.3318747247521,-32.0009136526746,
52.1214803633902));
#25038=CARTESIAN_POINT('Ctrl Pts',(-30.3356164490944,-32.001249815539,51.9285196366098));
#25039=CARTESIAN_POINT('Ctrl Pts',(-30.3342994524806,-32.1900886922754,
51.9159195389176));
#25040=CARTESIAN_POINT('Ctrl Pts',(-30.363956124187,-32.3785262679839,51.9033194412254));
#25041=CARTESIAN_POINT('Ctrl Pts',(-30.4263819138854,-32.5553981981287,
51.8907193435332));
#25042=CARTESIAN_POINT('Ctrl Pts',(-30.6099086616014,-33.0753872965215,
51.8536760804599));
#25043=CARTESIAN_POINT('Ctrl Pts',(-31.0766628964935,-33.4954131084019,
51.8166328173867));
#25044=CARTESIAN_POINT('Ctrl Pts',(-31.6130604137941,-33.6232740986022,
51.7795895543135));
#25045=CARTESIAN_POINT('Ctrl Pts',(-32.1494579310947,-33.7511350888025,
51.7425462912403));
#25046=CARTESIAN_POINT('Ctrl Pts',(-32.7554987308038,-33.5868312573226,
51.705503028167));
#25047=CARTESIAN_POINT('Ctrl Pts',(-33.1538618279575,-33.2055471471265,
51.6684597650937));
#25048=CARTESIAN_POINT('Ctrl Pts',(-33.5522249251112,-32.8242630369304,
51.6314165020205));
#25049=CARTESIAN_POINT('Ctrl Pts',(-33.7429103197094,-32.2259986480181,
51.5943732389473));
#25050=CARTESIAN_POINT('Ctrl Pts',(-33.6386614097067,-31.6845165205096,
51.557329975874));
#25051=CARTESIAN_POINT('Ctrl Pts',(-33.5344124997039,-31.1430343930012,
51.5202867128008));
#25052=CARTESIAN_POINT('Ctrl Pts',(-33.1352292851002,-30.6583345268966,
51.4832434497276));
#25053=CARTESIAN_POINT('Ctrl Pts',(-32.6237758401273,-30.4522129528976,
51.4462001866543));
#25054=CARTESIAN_POINT('Ctrl Pts',(-32.1123223951544,-30.2460913788987,
51.4091569235811));
#25055=CARTESIAN_POINT('Ctrl Pts',(-31.4885987198123,-30.3185480970053,
51.3721136605078));
#25056=CARTESIAN_POINT('Ctrl Pts',(-31.0380173860832,-30.6364273058174,
51.3350703974346));
#25057=CARTESIAN_POINT('Ctrl Pts',(-30.6060019538632,-30.9412085151324,
51.2995534771597));
#25058=CARTESIAN_POINT('Ctrl Pts',(-30.3331543957474,-31.4716039545601,
51.2640365568847));
#25059=CARTESIAN_POINT('Ctrl Pts',(-30.3313738033598,-32.0004179151157,
51.2285196366098));
#25060=CARTESIAN_POINT('Origin',(-32.,-32.,48.));
#25061=CARTESIAN_POINT('',(-30.3343902432864,-31.9984850050443,50.5285196366098));
#25062=CARTESIAN_POINT('',(-30.3367088458252,-32.0000156711401,50.7214803633902));
#25063=CARTESIAN_POINT('',(-30.334,-32.,48.));
#25064=CARTESIAN_POINT('Ctrl Pts',(-30.3367088458252,-32.0000156711401,
50.7214803633902));
#25065=CARTESIAN_POINT('Ctrl Pts',(-30.336732256219,-31.7210181018388,50.7400656131361));
#25066=CARTESIAN_POINT('Ctrl Pts',(-30.4031501299701,-31.4420100581718,
50.758650862882));
#25067=CARTESIAN_POINT('Ctrl Pts',(-30.5359003021068,-31.1992793533566,
50.7772361126279));
#25068=CARTESIAN_POINT('Ctrl Pts',(-30.8004918258534,-30.7154797016245,
50.8142793757012));
#25069=CARTESIAN_POINT('Ctrl Pts',(-31.3285991827343,-30.3757976728916,
50.8513226387744));
#25070=CARTESIAN_POINT('Ctrl Pts',(-31.8785633097738,-30.3356699216755,
50.8883659018477));
#25071=CARTESIAN_POINT('Ctrl Pts',(-32.4285274368133,-30.2955421704594,
50.9254091649209));
#25072=CARTESIAN_POINT('Ctrl Pts',(-33.0003483340113,-30.5549686967602,
50.9624524279941));
#25073=CARTESIAN_POINT('Ctrl Pts',(-33.3323638593996,-30.9952373287875,
50.9994956910674));
#25074=CARTESIAN_POINT('Ctrl Pts',(-33.664379384788,-31.4355059608149,51.0365389541406));
#25075=CARTESIAN_POINT('Ctrl Pts',(-33.7565895383665,-32.0566166985689,
51.0735822172139));
#25076=CARTESIAN_POINT('Ctrl Pts',(-33.5667994538073,-32.5743526363588,
51.1106254802872));
#25077=CARTESIAN_POINT('Ctrl Pts',(-33.3770093692481,-33.0920885741487,
51.1476687433604));
#25078=CARTESIAN_POINT('Ctrl Pts',(-32.905219046551,-33.5064497119744,51.1847120064336));
#25079=CARTESIAN_POINT('Ctrl Pts',(-32.3673171792835,-33.6278266398027,
51.2217552695068));
#25080=CARTESIAN_POINT('Ctrl Pts',(-31.8294153120161,-33.7492035676309,
51.25879853258));
#25081=CARTESIAN_POINT('Ctrl Pts',(-31.2254019001782,-33.5775962854617,
51.2958417956533));
#25082=CARTESIAN_POINT('Ctrl Pts',(-30.8316702057467,-33.191531355399,51.3328850587266));
#25083=CARTESIAN_POINT('Ctrl Pts',(-30.5177779571533,-32.8837512332643,
51.3624168269478));
#25084=CARTESIAN_POINT('Ctrl Pts',(-30.3375335491216,-32.4396691925109,
51.391948595169));
#25085=CARTESIAN_POINT('Ctrl Pts',(-30.3334712707803,-31.9985210140748,
51.4214803633902));
#25086=CARTESIAN_POINT('Ctrl Pts',(-30.3313738033598,-32.0004179151157,
51.2285196366098));
#25087=CARTESIAN_POINT('Ctrl Pts',(-30.3312972822441,-32.0231437419637,
51.2269932938115));
#25088=CARTESIAN_POINT('Ctrl Pts',(-30.3317213833894,-32.0458666480444,
51.2254669510132));
#25089=CARTESIAN_POINT('Ctrl Pts',(-30.3326549881033,-32.0685686010849,
51.2239406082149));
#25090=CARTESIAN_POINT('Ctrl Pts',(-30.3553129159683,-32.6195289880228,
51.1868973451416));
#25091=CARTESIAN_POINT('Ctrl Pts',(-30.6780677638144,-33.1581480623809,
51.1498540820684));
#25092=CARTESIAN_POINT('Ctrl Pts',(-31.1532286633698,-33.4379566562543,
51.1128108189951));
#25093=CARTESIAN_POINT('Ctrl Pts',(-31.6283895629253,-33.7177652501277,
51.0757675559219));
#25094=CARTESIAN_POINT('Ctrl Pts',(-32.25595651419,-33.7387633635163,51.0387242928487));
#25095=CARTESIAN_POINT('Ctrl Pts',(-32.7487582830866,-33.4913423736006,
51.0016810297754));
#25096=CARTESIAN_POINT('Ctrl Pts',(-33.2415600519832,-33.243921383685,50.9646377667022));
#25097=CARTESIAN_POINT('Ctrl Pts',(-33.5995966385115,-32.7280812904652,
50.9275945036289));
#25098=CARTESIAN_POINT('Ctrl Pts',(-33.6590324420583,-32.1798677235672,
50.8905512405557));
#25099=CARTESIAN_POINT('Ctrl Pts',(-33.7184682456052,-31.6316541566692,
50.8535079774824));
#25100=CARTESIAN_POINT('Ctrl Pts',(-33.4793032661706,-31.0510671160931,
50.8164647144092));
#25101=CARTESIAN_POINT('Ctrl Pts',(-33.0509781015208,-30.7037800835068,
50.7794214513359));
#25102=CARTESIAN_POINT('Ctrl Pts',(-32.622652936871,-30.3564930509205,50.7423781882627));
#25103=CARTESIAN_POINT('Ctrl Pts',(-32.0051675870062,-30.2425060263241,
50.7053349251895));
#25104=CARTESIAN_POINT('Ctrl Pts',(-31.4810799998519,-30.4139788541026,
50.6682916621162));
#25105=CARTESIAN_POINT('Ctrl Pts',(-30.9569924126976,-30.5854516818812,
50.631248399043));
#25106=CARTESIAN_POINT('Ctrl Pts',(-30.5263025882539,-31.0423843620347,
50.5942051359698));
#25107=CARTESIAN_POINT('Ctrl Pts',(-30.3860918548667,-31.57568697774,50.5571618728965));
#25108=CARTESIAN_POINT('Ctrl Pts',(-30.3499543890818,-31.7131386874804,
50.5476144608009));
#25109=CARTESIAN_POINT('Ctrl Pts',(-30.3331129433613,-31.8556635190189,
50.5380670487054));
#25110=CARTESIAN_POINT('Ctrl Pts',(-30.3343902432864,-31.9984850050443,
50.5285196366098));
#25111=CARTESIAN_POINT('Origin',(-32.,-32.,48.));
#25112=CARTESIAN_POINT('',(-30.3365646054836,-32.0005076073409,49.8285196366098));
#25113=CARTESIAN_POINT('',(-30.3334137580317,-32.0014707566408,50.0214803633902));
#25114=CARTESIAN_POINT('',(-30.334,-32.,48.));
#25115=CARTESIAN_POINT('Ctrl Pts',(-30.3334137580317,-32.0014707566408,
50.0214803633902));
#25116=CARTESIAN_POINT('Ctrl Pts',(-30.337485924098,-31.5584612466466,50.05113936803));
#25117=CARTESIAN_POINT('Ctrl Pts',(-30.5194576447965,-31.1124969702324,
50.0807983726698));
#25118=CARTESIAN_POINT('Ctrl Pts',(-30.8357594969185,-30.8044726977954,
50.1104573773095));
#25119=CARTESIAN_POINT('Ctrl Pts',(-31.2308116188967,-30.419759040159,50.1475006403828));
#25120=CARTESIAN_POINT('Ctrl Pts',(-31.8354094477522,-30.2502222407132,
50.1845439034561));
#25121=CARTESIAN_POINT('Ctrl Pts',(-32.3728922952957,-30.3734414196097,
50.2215871665293));
#25122=CARTESIAN_POINT('Ctrl Pts',(-32.9103751428392,-30.4966605985061,
50.2586304296025));
#25123=CARTESIAN_POINT('Ctrl Pts',(-33.3807430090707,-30.9126357557449,
50.2956736926757));
#25124=CARTESIAN_POINT('Ctrl Pts',(-33.5687581088666,-31.4310189149042,
50.332716955749));
#25125=CARTESIAN_POINT('Ctrl Pts',(-33.7567732086625,-31.9494020740635,
50.3697602188222));
#25126=CARTESIAN_POINT('Ctrl Pts',(-33.6624355420228,-32.5701932351434,
50.4068034818955));
#25127=CARTESIAN_POINT('Ctrl Pts',(-33.3289135136764,-33.0093217289349,
50.4438467449688));
#25128=CARTESIAN_POINT('Ctrl Pts',(-32.99539148533,-33.4484502227263,50.480890008042));
#25129=CARTESIAN_POINT('Ctrl Pts',(-32.422685095277,-33.7059160492293,50.5179332711152));
#25130=CARTESIAN_POINT('Ctrl Pts',(-31.8728616822359,-33.6639042422839,
50.5549765341885));
#25131=CARTESIAN_POINT('Ctrl Pts',(-31.3230382691947,-33.6218924353386,
50.5920197972617));
#25132=CARTESIAN_POINT('Ctrl Pts',(-30.7960978331653,-33.280402994945,50.629063060335));
#25133=CARTESIAN_POINT('Ctrl Pts',(-30.5331654604567,-32.7956996373825,
50.6661063234082));
#25134=CARTESIAN_POINT('Ctrl Pts',(-30.402150834935,-32.5541803895775,50.6845643367355));
#25135=CARTESIAN_POINT('Ctrl Pts',(-30.3366855957013,-32.2771031960785,
50.7030223500629));
#25136=CARTESIAN_POINT('Ctrl Pts',(-30.3367088458252,-32.0000156711401,
50.7214803633902));
#25137=CARTESIAN_POINT('Ctrl Pts',(-30.3343902432864,-31.9984850050443,
50.5285196366098));
#25138=CARTESIAN_POINT('Ctrl Pts',(-30.3380687739757,-32.4098004753368,
50.5010237856321));
#25139=CARTESIAN_POINT('Ctrl Pts',(-30.4920238221381,-32.8235763920677,
50.4735279346544));
#25140=CARTESIAN_POINT('Ctrl Pts',(-30.7681349422019,-33.1257217778669,
50.4460320836768));
#25141=CARTESIAN_POINT('Ctrl Pts',(-31.140120405255,-33.5327814110317,50.4089888206035));
#25142=CARTESIAN_POINT('Ctrl Pts',(-31.733822973692,-33.7372281261045,50.3719455575303));
#25143=CARTESIAN_POINT('Ctrl Pts',(-32.2775675714139,-33.6455082148342,
50.3349022944571));
#25144=CARTESIAN_POINT('Ctrl Pts',(-32.8213121691358,-33.553788303564,50.2978590313838));
#25145=CARTESIAN_POINT('Ctrl Pts',(-33.3150987961427,-33.1659017659506,
50.2608157683106));
#25146=CARTESIAN_POINT('Ctrl Pts',(-33.5329733693628,-32.6593433783788,
50.2237725052373));
#25147=CARTESIAN_POINT('Ctrl Pts',(-33.7508479425829,-32.1527849908071,
50.1867292421641));
#25148=CARTESIAN_POINT('Ctrl Pts',(-33.6928104620162,-31.5275547532769,
50.1496859790908));
#25149=CARTESIAN_POINT('Ctrl Pts',(-33.3854185640749,-31.0697546323123,
50.1126427160176));
#25150=CARTESIAN_POINT('Ctrl Pts',(-33.0780266661335,-30.6119545113477,
50.0755994529444));
#25151=CARTESIAN_POINT('Ctrl Pts',(-32.5212803508175,-30.3215845069488,
50.0385561898711));
#25152=CARTESIAN_POINT('Ctrl Pts',(-31.9699437131843,-30.3315163586626,
50.0015129267979));
#25153=CARTESIAN_POINT('Ctrl Pts',(-31.418607075551,-30.3414482103765,49.9644696637246));
#25154=CARTESIAN_POINT('Ctrl Pts',(-30.8726801156006,-30.6516819182031,
49.9274264006514));
#25155=CARTESIAN_POINT('Ctrl Pts',(-30.5819760500406,-31.1202562196133,
49.8903831375781));
#25156=CARTESIAN_POINT('Ctrl Pts',(-30.4201475127281,-31.3811011915381,
49.8697619705887));
#25157=CARTESIAN_POINT('Ctrl Pts',(-30.3374100791124,-31.6910143802325,
49.8491408035992));
#25158=CARTESIAN_POINT('Ctrl Pts',(-30.3365646054836,-32.0005076073409,
49.8285196366098));
#25159=CARTESIAN_POINT('Origin',(-32.,-32.,48.));
#25160=CARTESIAN_POINT('',(-30.3325307315923,-32.0012453487269,49.1285196366098));
#25161=CARTESIAN_POINT('',(-30.3319159147668,-31.9990590791559,49.3214803633902));
#25162=CARTESIAN_POINT('',(-30.334,-32.,48.));
#25163=CARTESIAN_POINT('Ctrl Pts',(-30.3319159147668,-31.9990590791559,
49.3214803633902));
#25164=CARTESIAN_POINT('Ctrl Pts',(-30.3315442283774,-31.944078547628,49.3251698598506));
#25165=CARTESIAN_POINT('Ctrl Pts',(-30.334026958555,-31.8891319939439,49.3288593563111));
#25166=CARTESIAN_POINT('Ctrl Pts',(-30.3394745019395,-31.8344809690004,
49.3325488527715));
#25167=CARTESIAN_POINT('Ctrl Pts',(-30.3941688985489,-31.285774034079,49.3695921158447));
#25168=CARTESIAN_POINT('Ctrl Pts',(-30.7477328056741,-30.7668580248817,
49.4066353789179));
#25169=CARTESIAN_POINT('Ctrl Pts',(-31.2383772965352,-30.5151860935124,
49.4436786419912));
#25170=CARTESIAN_POINT('Ctrl Pts',(-31.7290217873962,-30.2635141621431,
49.4807219050644));
#25171=CARTESIAN_POINT('Ctrl Pts',(-32.356746861993,-30.2790863086019,49.5177651681377));
#25172=CARTESIAN_POINT('Ctrl Pts',(-32.8343089298875,-30.5547768031055,
49.554808431211));
#25173=CARTESIAN_POINT('Ctrl Pts',(-33.3118709977821,-30.8304672976092,
49.5918516942842));
#25174=CARTESIAN_POINT('Ctrl Pts',(-33.6392700589744,-31.3662761401577,
49.6288949573574));
#25175=CARTESIAN_POINT('Ctrl Pts',(-33.6666900783104,-31.9170201097035,
49.6659382204307));
#25176=CARTESIAN_POINT('Ctrl Pts',(-33.6941100976464,-32.4677640792492,
49.7029814835039));
#25177=CARTESIAN_POINT('Ctrl Pts',(-33.4215510751261,-33.0334431757922,
49.7400247465771));
#25178=CARTESIAN_POINT('Ctrl Pts',(-32.9737345415649,-33.3552057120214,
49.7770680096504));
#25179=CARTESIAN_POINT('Ctrl Pts',(-32.5259180080037,-33.6769682482507,
49.8141112727236));
#25180=CARTESIAN_POINT('Ctrl Pts',(-31.9028439634017,-33.7548142241662,
49.8511545357969));
#25181=CARTESIAN_POINT('Ctrl Pts',(-31.3896277120905,-33.5531217432913,
49.8881977988701));
#25182=CARTESIAN_POINT('Ctrl Pts',(-30.8764114607793,-33.3514292624164,
49.9252410619434));
#25183=CARTESIAN_POINT('Ctrl Pts',(-30.4730530027589,-32.870198324751,49.9622843250166));
#25184=CARTESIAN_POINT('Ctrl Pts',(-30.3641269812991,-32.3296375980049,
49.9993275880898));
#25185=CARTESIAN_POINT('Ctrl Pts',(-30.3424135082988,-32.2218814292955,
50.0067118465233));
#25186=CARTESIAN_POINT('Ctrl Pts',(-30.3323999031507,-32.1117676715239,
50.0140961049567));
#25187=CARTESIAN_POINT('Ctrl Pts',(-30.3334137580317,-32.0014707566408,
50.0214803633902));
#25188=CARTESIAN_POINT('Ctrl Pts',(-30.3365646054836,-32.0005076073409,
49.8285196366098));
#25189=CARTESIAN_POINT('Ctrl Pts',(-30.3358912949394,-32.246978988687,49.812097540526));
#25190=CARTESIAN_POINT('Ctrl Pts',(-30.3871543989708,-32.493184027659,49.7956754444422));
#25191=CARTESIAN_POINT('Ctrl Pts',(-30.4917685280704,-32.7141280479498,
49.7792533483584));
#25192=CARTESIAN_POINT('Ctrl Pts',(-30.7277462428298,-33.2125106798825,
49.7422100852852));
#25193=CARTESIAN_POINT('Ctrl Pts',(-31.2351828435182,-33.582361048754,49.7051668222119));
#25194=CARTESIAN_POINT('Ctrl Pts',(-31.7818780931209,-33.6544376311989,
49.6681235591387));
#25195=CARTESIAN_POINT('Ctrl Pts',(-32.3285733427237,-33.7265142136438,
49.6310802960654));
#25196=CARTESIAN_POINT('Ctrl Pts',(-32.9145272412408,-33.5008170096621,
49.5940370329922));
#25197=CARTESIAN_POINT('Ctrl Pts',(-33.2716104619136,-33.0806238360038,
49.5569937699189));
#25198=CARTESIAN_POINT('Ctrl Pts',(-33.6286936825864,-32.6604306623454,
49.5199505068457));
#25199=CARTESIAN_POINT('Ctrl Pts',(-33.7569062254148,-32.0457415190103,
49.4829072437725));
#25200=CARTESIAN_POINT('Ctrl Pts',(-33.5975787260042,-31.5178348249755,
49.4458639806993));
#25201=CARTESIAN_POINT('Ctrl Pts',(-33.4382512265936,-30.9899281309408,
49.408820717626));
#25202=CARTESIAN_POINT('Ctrl Pts',(-32.9913836849439,-30.5488038862063,
49.3717774545527));
#25203=CARTESIAN_POINT('Ctrl Pts',(-32.4614602650756,-30.3963181532661,
49.3347341914795));
#25204=CARTESIAN_POINT('Ctrl Pts',(-31.9315368452074,-30.2438324203258,
49.2976909284063));
#25205=CARTESIAN_POINT('Ctrl Pts',(-31.3185575471206,-30.3799851991798,
49.260647665333));
#25206=CARTESIAN_POINT('Ctrl Pts',(-30.903018373878,-30.7424737164821,49.2236044022598));
#25207=CARTESIAN_POINT('Ctrl Pts',(-30.5474751375992,-31.0526258004598,
49.1919094803765));
#25208=CARTESIAN_POINT('Ctrl Pts',(-30.3364746524795,-31.5284746512257,
49.1602145584931));
#25209=CARTESIAN_POINT('Ctrl Pts',(-30.3325307315923,-32.0012453487269,
49.1285196366098));
#25210=CARTESIAN_POINT('Origin',(-32.,-32.,48.));
#25211=CARTESIAN_POINT('',(-30.3326865583594,-31.9986999266502,48.4285196366098));
#25212=CARTESIAN_POINT('',(-30.3362532052763,-31.9991286485791,48.6214803633902));
#25213=CARTESIAN_POINT('',(-30.334,-32.,48.));
#25214=CARTESIAN_POINT('Ctrl Pts',(-30.3362532052763,-31.9991286485791,
48.6214803633902));
#25215=CARTESIAN_POINT('Ctrl Pts',(-30.3352028054858,-31.7776576899582,
48.6362436147445));
#25216=CARTESIAN_POINT('Ctrl Pts',(-30.3763004874845,-31.5565607348184,
48.6510068660988));
#25217=CARTESIAN_POINT('Ctrl Pts',(-30.461383908182,-31.3539334389316,48.6657701174531));
#25218=CARTESIAN_POINT('Ctrl Pts',(-30.6748712667882,-30.8455104603333,
48.7028133805264));
#25219=CARTESIAN_POINT('Ctrl Pts',(-31.1652862840003,-30.4533697050991,
48.7398566435996));
#25220=CARTESIAN_POINT('Ctrl Pts',(-31.7082177071069,-30.3569526565293,
48.7768999066728));
#25221=CARTESIAN_POINT('Ctrl Pts',(-32.2511491302134,-30.2605356079596,
48.8139431697461));
#25222=CARTESIAN_POINT('Ctrl Pts',(-32.8465969592144,-30.4598422660544,
48.8509864328193));
#25223=CARTESIAN_POINT('Ctrl Pts',(-33.2220874962403,-30.8636709847649,
48.8880296958926));
#25224=CARTESIAN_POINT('Ctrl Pts',(-33.5975780332662,-31.2674997034754,
48.9250729589658));
#25225=CARTESIAN_POINT('Ctrl Pts',(-33.7531112783172,-31.8758504828017,
48.962116222039));
#25226=CARTESIAN_POINT('Ctrl Pts',(-33.6175160618016,-32.4103453047687,
48.9991594851123));
#25227=CARTESIAN_POINT('Ctrl Pts',(-33.4819208452861,-32.9448401267356,
49.0362027481855));
#25228=CARTESIAN_POINT('Ctrl Pts',(-33.0551971672042,-33.4054789913434,
49.0732460112588));
#25229=CARTESIAN_POINT('Ctrl Pts',(-32.5326114688334,-33.5814760518576,
49.110289274332));
#25230=CARTESIAN_POINT('Ctrl Pts',(-32.0100257704625,-33.7574731123719,
49.1473325374053));
#25231=CARTESIAN_POINT('Ctrl Pts',(-31.3915780518028,-33.6488283687926,
49.1843758004785));
#25232=CARTESIAN_POINT('Ctrl Pts',(-30.9602666355197,-33.3052570666801,
49.2214190635517));
#25233=CARTESIAN_POINT('Ctrl Pts',(-30.5719136902701,-32.9959053499358,
49.2547728301646));
#25234=CARTESIAN_POINT('Ctrl Pts',(-30.3352760321209,-32.4960937928359,
49.2881265967774));
#25235=CARTESIAN_POINT('Ctrl Pts',(-30.3319159147668,-31.9990590791559,
49.3214803633902));
#25236=CARTESIAN_POINT('Ctrl Pts',(-30.3325307315923,-32.0012453487269,
49.1285196366098));
#25237=CARTESIAN_POINT('Ctrl Pts',(-30.3318652169521,-32.0810227655679,
49.1231712954199));
#25238=CARTESIAN_POINT('Ctrl Pts',(-30.337095571527,-32.1607125329826,49.11782295423));
#25239=CARTESIAN_POINT('Ctrl Pts',(-30.3485221706369,-32.239503697069,49.11247461304));
#25240=CARTESIAN_POINT('Ctrl Pts',(-30.4276641890369,-32.7852209046031,
49.0754313499668));
#25241=CARTESIAN_POINT('Ctrl Pts',(-30.8040472742353,-33.2878310639205,
49.0383880868936));
#25242=CARTESIAN_POINT('Ctrl Pts',(-31.3054405672976,-33.5173424914078,
49.0013448238203));
#25243=CARTESIAN_POINT('Ctrl Pts',(-31.8068338603599,-33.7468539188952,
48.9643015607471));
#25244=CARTESIAN_POINT('Ctrl Pts',(-32.4332373612862,-33.7032666145523,
48.9272582976738));
#25245=CARTESIAN_POINT('Ctrl Pts',(-32.8980122245841,-33.4065258925043,
48.8902150346006));
#25246=CARTESIAN_POINT('Ctrl Pts',(-33.3627870878821,-33.1097851704563,
48.8531717715273));
#25247=CARTESIAN_POINT('Ctrl Pts',(-33.6659333135516,-32.5598910307031,
48.8161285084541));
#25248=CARTESIAN_POINT('Ctrl Pts',(-33.6687328324683,-32.008472049919,48.7790852453809));
#25249=CARTESIAN_POINT('Ctrl Pts',(-33.6715323513851,-31.4570530691349,
48.7420419823076));
#25250=CARTESIAN_POINT('Ctrl Pts',(-33.373985163549,-30.9041092473198,48.7049987192344));
#25251=CARTESIAN_POINT('Ctrl Pts',(-32.9122472487315,-30.6026646791234,
48.6679554561611));
#25252=CARTESIAN_POINT('Ctrl Pts',(-32.450509333914,-30.3012201109269,48.6309121930879));
#25253=CARTESIAN_POINT('Ctrl Pts',(-31.824580692115,-30.2512747963491,48.5938689300147));
#25254=CARTESIAN_POINT('Ctrl Pts',(-31.3208828758651,-30.4756834405235,
48.5568256669414));
#25255=CARTESIAN_POINT('Ctrl Pts',(-30.8171850596151,-30.7000920846979,
48.5197824038682));
#25256=CARTESIAN_POINT('Ctrl Pts',(-30.4357180689142,-31.1988546876245,
48.4827391407949));
#25257=CARTESIAN_POINT('Ctrl Pts',(-30.3510391302884,-31.7437401866318,
48.4456958777217));
#25258=CARTESIAN_POINT('Ctrl Pts',(-30.3379511376165,-31.8279577917855,
48.4399704640177));
#25259=CARTESIAN_POINT('Ctrl Pts',(-30.3319530707094,-31.913277219964,48.4342450503138));
#25260=CARTESIAN_POINT('Ctrl Pts',(-30.3326865583594,-31.9986999266502,
48.4285196366098));
#25261=CARTESIAN_POINT('Origin',(-32.,-32.,48.));
#25262=CARTESIAN_POINT('',(-30.3366116224995,-31.9995809948969,47.7285196366098));
#25263=CARTESIAN_POINT('',(-30.3350930889229,-32.0014151418723,47.9214803633902));
#25264=CARTESIAN_POINT('',(-30.334,-32.,48.));
#25265=CARTESIAN_POINT('Ctrl Pts',(-30.3350930889229,-32.0014151418723,
47.9214803633902));
#25266=CARTESIAN_POINT('Ctrl Pts',(-30.3382178115278,-31.6145003654984,
47.9473173696384));
#25267=CARTESIAN_POINT('Ctrl Pts',(-30.4725789758866,-31.2256285393869,
47.9731543758866));
#25268=CARTESIAN_POINT('Ctrl Pts',(-30.719095189131,-30.9304092629306,47.9989913821348));
#25269=CARTESIAN_POINT('Ctrl Pts',(-31.0725326133941,-30.5071448484311,
48.036034645208));
#25270=CARTESIAN_POINT('Ctrl Pts',(-31.6565135579398,-30.2763906124344,
48.0730779082813));
#25271=CARTESIAN_POINT('Ctrl Pts',(-32.2038115090487,-30.3437384421199,
48.1101211713545));
#25272=CARTESIAN_POINT('Ctrl Pts',(-32.7511094601577,-30.4110862718055,
48.1471644344278));
#25273=CARTESIAN_POINT('Ctrl Pts',(-33.2617244178299,-30.7765361671732,
48.184207697501));
#25274=CARTESIAN_POINT('Ctrl Pts',(-33.5020017461289,-31.2728602376724,
48.2212509605742));
#25275=CARTESIAN_POINT('Ctrl Pts',(-33.7422790744279,-31.7691843081716,
48.2582942236475));
#25276=CARTESIAN_POINT('Ctrl Pts',(-33.7122187733536,-32.3963825538023,
48.2953374867207));
#25277=CARTESIAN_POINT('Ctrl Pts',(-33.4255762736826,-32.8674524582047,
48.3323807497939));
#25278=CARTESIAN_POINT('Ctrl Pts',(-33.1389337740115,-33.3385223626072,
48.3694240128672));
#25279=CARTESIAN_POINT('Ctrl Pts',(-32.5957090757435,-33.6534639257813,
48.4064672759404));
#25280=CARTESIAN_POINT('Ctrl Pts',(-32.0444788552928,-33.6681615961183,
48.4435105390136));
#25281=CARTESIAN_POINT('Ctrl Pts',(-31.4932486348422,-33.6828592664552,
48.4805538020869));
#25282=CARTESIAN_POINT('Ctrl Pts',(-30.9340128922089,-33.3973130439549,
48.5175970651602));
#25283=CARTESIAN_POINT('Ctrl Pts',(-30.6226748708923,-32.9421873317236,
48.5546403282334));
#25284=CARTESIAN_POINT('Ctrl Pts',(-30.4354177507577,-32.6684477807004,
48.5769203399523));
#25285=CARTESIAN_POINT('Ctrl Pts',(-30.3378384197443,-32.3333623099221,
48.5992003516713));
#25286=CARTESIAN_POINT('Ctrl Pts',(-30.3362532052763,-31.9991286485791,
48.6214803633902));
#25287=CARTESIAN_POINT('Ctrl Pts',(-30.3326865583594,-31.9986999266502,
48.4285196366098));
#25288=CARTESIAN_POINT('Ctrl Pts',(-30.3366987148472,-32.4659596914531,
48.3972017872405));
#25289=CARTESIAN_POINT('Ctrl Pts',(-30.5421229378924,-32.9363096098717,
48.3658839378713));
#25290=CARTESIAN_POINT('Ctrl Pts',(-30.8903064904358,-33.2463231349127,
48.334566088502));
#25291=CARTESIAN_POINT('Ctrl Pts',(-31.3021436757596,-33.6130121890985,
48.2975228254287));
#25292=CARTESIAN_POINT('Ctrl Pts',(-31.913708932958,-33.7553819023824,48.2604795623555));
#25293=CARTESIAN_POINT('Ctrl Pts',(-32.4451533164113,-33.6082846659331,
48.2234362992822));
#25294=CARTESIAN_POINT('Ctrl Pts',(-32.9765976998647,-33.4611874294839,
48.186393036209));
#25295=CARTESIAN_POINT('Ctrl Pts',(-33.4279212095732,-33.0246232433016,
48.1493497731358));
#25296=CARTESIAN_POINT('Ctrl Pts',(-33.5926006546939,-32.4983615118125,
48.1123065100625));
#25297=CARTESIAN_POINT('Ctrl Pts',(-33.7572800998147,-31.9720997803234,
48.0752632469893));
#25298=CARTESIAN_POINT('Ctrl Pts',(-33.6353154803478,-31.3561405035276,
48.038219983916));
#25299=CARTESIAN_POINT('Ctrl Pts',(-33.2825171448356,-30.9323433065866,
48.0011767208428));
#25300=CARTESIAN_POINT('Ctrl Pts',(-32.9297188093234,-30.5085461096457,
47.9641334577695));
#25301=CARTESIAN_POINT('Ctrl Pts',(-32.346086757766,-30.2769109925596,47.9270901946963));
#25302=CARTESIAN_POINT('Ctrl Pts',(-31.798687852343,-30.343432928918,47.8900469316231));
#25303=CARTESIAN_POINT('Ctrl Pts',(-31.2512889469199,-30.4099548652763,
47.8530036685498));
#25304=CARTESIAN_POINT('Ctrl Pts',(-30.7401231876313,-30.774633855079,47.8159604054766));
#25305=CARTESIAN_POINT('Ctrl Pts',(-30.4990972542467,-31.2705947699818,
47.7789171424033));
#25306=CARTESIAN_POINT('Ctrl Pts',(-30.3897916759726,-31.4955136981799,
47.7621179738055));
#25307=CARTESIAN_POINT('Ctrl Pts',(-30.33604398485,-31.7474325193236,47.7453188052077));
#25308=CARTESIAN_POINT('Ctrl Pts',(-30.3366116224995,-31.9995809948969,
47.7285196366098));
#25309=CARTESIAN_POINT('Origin',(-32.,-32.,48.));
#25310=CARTESIAN_POINT('',(-30.3342224410882,-32.0015218249211,47.0285196366098));
#25311=CARTESIAN_POINT('',(-30.3312461696345,-32.0000368502823,47.2214803633902));
#25312=CARTESIAN_POINT('',(-30.334,-32.,48.));
#25313=CARTESIAN_POINT('Ctrl Pts',(-30.3312465621464,-32.0000368450299,
47.2214803633902));
#25314=CARTESIAN_POINT('Ctrl Pts',(-30.3314253521056,-31.4505822201728,
47.2583911245323));
#25315=CARTESIAN_POINT('Ctrl Pts',(-30.6293231084363,-30.9009614593998,
47.2953018856743));
#25316=CARTESIAN_POINT('Ctrl Pts',(-31.089862141057,-30.601289680795,47.3322126468164));
#25317=CARTESIAN_POINT('Ctrl Pts',(-31.5520544127147,-30.3005421430306,
47.3692559098896));
#25318=CARTESIAN_POINT('Ctrl Pts',(-32.1780577530503,-30.2515413378172,
47.4062991729629));
#25319=CARTESIAN_POINT('Ctrl Pts',(-32.681416427888,-30.4767097679246,47.4433424360361));
#25320=CARTESIAN_POINT('Ctrl Pts',(-33.1847751027257,-30.701878198032,47.4803856991094));
#25321=CARTESIAN_POINT('Ctrl Pts',(-33.5654891120655,-31.2012158634602,
47.5174289621826));
#25322=CARTESIAN_POINT('Ctrl Pts',(-33.6493457895693,-31.7462285560549,
47.5544722252559));
#25323=CARTESIAN_POINT('Ctrl Pts',(-33.7332024670731,-32.2912412486497,
47.5915154883291));
#25324=CARTESIAN_POINT('Ctrl Pts',(-33.5202018127409,-32.8819289684111,
47.6285587514023));
#25325=CARTESIAN_POINT('Ctrl Pts',(-33.1078117710471,-33.2479962176471,
47.6656020144756));
#25326=CARTESIAN_POINT('Ctrl Pts',(-32.6954217293533,-33.6140634668831,
47.7026452775488));
#25327=CARTESIAN_POINT('Ctrl Pts',(-32.083642300298,-33.7555102455937,47.739688540622));
#25328=CARTESIAN_POINT('Ctrl Pts',(-31.552420433381,-33.6076112748041,47.7767318036953));
#25329=CARTESIAN_POINT('Ctrl Pts',(-31.021198566464,-33.4597123040145,47.8137750667685));
#25330=CARTESIAN_POINT('Ctrl Pts',(-30.5705342616853,-33.0224675837247,
47.8508183298418));
#25331=CARTESIAN_POINT('Ctrl Pts',(-30.4066490612863,-32.4959579270787,
47.887861592915));
#25332=CARTESIAN_POINT('Ctrl Pts',(-30.357070825107,-32.3366792366031,47.8990678497401));
#25333=CARTESIAN_POINT('Ctrl Pts',(-30.3337378063611,-32.1692312700957,
47.9102741065651));
#25334=CARTESIAN_POINT('Ctrl Pts',(-30.3350930889229,-32.0014151418723,
47.9214803633902));
#25335=CARTESIAN_POINT('Ctrl Pts',(-30.3366116224995,-31.9995809948969,
47.7285196366098));
#25336=CARTESIAN_POINT('Ctrl Pts',(-30.3372956629111,-32.303436363191,47.7082755421344));
#25337=CARTESIAN_POINT('Ctrl Pts',(-30.4168554613542,-32.6076252315785,
47.688031447659));
#25338=CARTESIAN_POINT('Ctrl Pts',(-30.5731165724514,-32.8653003674879,
47.6677873531836));
#25339=CARTESIAN_POINT('Ctrl Pts',(-30.8590479315214,-33.3368022100883,
47.6307440901104));
#25340=CARTESIAN_POINT('Ctrl Pts',(-31.4017967571419,-33.6525630552862,
47.5937008270371));
#25341=CARTESIAN_POINT('Ctrl Pts',(-31.9530041296421,-33.6680924524609,
47.5566575639639));
#25342=CARTESIAN_POINT('Ctrl Pts',(-32.5042115021423,-33.6836218496355,
47.5196143008906));
#25343=CARTESIAN_POINT('Ctrl Pts',(-33.0638774215221,-33.398919798787,47.4825710378174));
#25344=CARTESIAN_POINT('Ctrl Pts',(-33.3759017977354,-32.944264414651,47.4455277747442));
#25345=CARTESIAN_POINT('Ctrl Pts',(-33.6879261739487,-32.489609030515,47.4084845116709));
#25346=CARTESIAN_POINT('Ctrl Pts',(-33.7523090069954,-31.8650003130914,
47.3714412485976));
#25347=CARTESIAN_POINT('Ctrl Pts',(-33.5395890615749,-31.3562558246737,
47.3343979855244));
#25348=CARTESIAN_POINT('Ctrl Pts',(-33.3268691161543,-30.8475113362559,
47.2973547224511));
#25349=CARTESIAN_POINT('Ctrl Pts',(-32.8370463922665,-30.454631076844,47.2603114593779));
#25350=CARTESIAN_POINT('Ctrl Pts',(-32.2942611124092,-30.3573949228402,
47.2232681963047));
#25351=CARTESIAN_POINT('Ctrl Pts',(-31.751475832552,-30.2601587688364,47.1862249332315));
#25352=CARTESIAN_POINT('Ctrl Pts',(-31.1557279967253,-30.4585667202408,
47.1491816701582));
#25353=CARTESIAN_POINT('Ctrl Pts',(-30.7796285842955,-30.861828374313,47.112138407085));
#25354=CARTESIAN_POINT('Ctrl Pts',(-30.4966354222943,-31.165259559867,47.0842654835932));
#25355=CARTESIAN_POINT('Ctrl Pts',(-30.3380005280478,-31.5846726915372,
47.0563925601015));
#25356=CARTESIAN_POINT('Ctrl Pts',(-30.3342224410882,-32.0015218249211,
47.0285196366098));
#25357=CARTESIAN_POINT('Origin',(-32.,-32.,48.));
#25358=CARTESIAN_POINT('',(-30.3314412753146,-31.9994832045548,46.3285196366098));
#25359=CARTESIAN_POINT('',(-30.3349857214592,-31.9985615244857,46.5214803633902));
#25360=CARTESIAN_POINT('',(-30.334,-32.,48.));
#25361=CARTESIAN_POINT('Ctrl Pts',(-30.3349857214592,-31.9985615244857,
46.5214803633902));
#25362=CARTESIAN_POINT('Ctrl Pts',(-30.3336343248108,-31.8347406191154,
46.5324216163529));
#25363=CARTESIAN_POINT('Ctrl Pts',(-30.3558556414528,-31.6712783220273,
46.5433628693156));
#25364=CARTESIAN_POINT('Ctrl Pts',(-30.4031505005406,-31.5154247680614,
46.5543041222783));
#25365=CARTESIAN_POINT('Ctrl Pts',(-30.5632743833515,-30.987759040915,46.5913473853516));
#25366=CARTESIAN_POINT('Ctrl Pts',(-31.010807058637,-30.547309536914,46.6283906484248));
#25367=CARTESIAN_POINT('Ctrl Pts',(-31.5409600008313,-30.3956235608514,
46.665433911498));
#25368=CARTESIAN_POINT('Ctrl Pts',(-32.0711129430257,-30.2439375847887,
46.7024771745713));
#25369=CARTESIAN_POINT('Ctrl Pts',(-32.6838861521289,-30.3810151366644,
46.7395204376445));
#25370=CARTESIAN_POINT('Ctrl Pts',(-33.0988779302797,-30.7441302720122,
46.7765637007178));
#25371=CARTESIAN_POINT('Ctrl Pts',(-33.5138697084305,-31.10724540736,46.813606963791));
#25372=CARTESIAN_POINT('Ctrl Pts',(-33.7310800556289,-31.6963981261798,
46.8506502268642));
#25373=CARTESIAN_POINT('Ctrl Pts',(-33.651114694771,-32.2419953388874,46.8876934899375));
#25374=CARTESIAN_POINT('Ctrl Pts',(-33.5711493339131,-32.7875925515949,
46.9247367530107));
#25375=CARTESIAN_POINT('Ctrl Pts',(-33.1940082649989,-33.2896342581902,
46.961780016084));
#25376=CARTESIAN_POINT('Ctrl Pts',(-32.6922691962012,-33.518388895943,46.9988232791572));
#25377=CARTESIAN_POINT('Ctrl Pts',(-32.1905301274034,-33.7471435336958,
47.0358665422305));
#25378=CARTESIAN_POINT('Ctrl Pts',(-31.5641930587222,-33.7026111026061,
47.0729098053037));
#25379=CARTESIAN_POINT('Ctrl Pts',(-31.0998664366148,-33.4051694016735,
47.109953068377));
#25380=CARTESIAN_POINT('Ctrl Pts',(-30.6355398145073,-33.1077277007409,
47.1469963314502));
#25381=CARTESIAN_POINT('Ctrl Pts',(-30.3332236389736,-32.5573767299654,
47.1840395945234));
#25382=CARTESIAN_POINT('Ctrl Pts',(-30.3312561526966,-32.00595410942,47.2210828575967));
#25383=CARTESIAN_POINT('Ctrl Pts',(-30.3312491150949,-32.0039816978112,
47.2212153595279));
#25384=CARTESIAN_POINT('Ctrl Pts',(-30.3312459203277,-32.002009272491,47.221347861459));
#25385=CARTESIAN_POINT('Ctrl Pts',(-30.3312465621464,-32.0000368450299,
47.2214803633902));
#25386=CARTESIAN_POINT('Ctrl Pts',(-30.3342224410882,-32.0015218249211,
47.0285196366098));
#25387=CARTESIAN_POINT('Ctrl Pts',(-30.332979430451,-32.1386673994973,47.0193492970283));
#25388=CARTESIAN_POINT('Ctrl Pts',(-30.3484988156394,-32.2755354353916,
47.0101789574467));
#25389=CARTESIAN_POINT('Ctrl Pts',(-30.3818667414576,-32.4079041546572,
47.0010086178652));
#25390=CARTESIAN_POINT('Ctrl Pts',(-30.5166553000827,-32.9426029241892,
46.963965354792));
#25391=CARTESIAN_POINT('Ctrl Pts',(-30.9426834063659,-33.4038851065129,
46.9269220917188));
#25392=CARTESIAN_POINT('Ctrl Pts',(-31.4650029089132,-33.5806704761956,
46.8898788286455));
#25393=CARTESIAN_POINT('Ctrl Pts',(-31.9873224114606,-33.7574558458782,
46.8528355655723));
#25394=CARTESIAN_POINT('Ctrl Pts',(-32.6059333102722,-33.6497444029199,
46.815792302499));
#25395=CARTESIAN_POINT('Ctrl Pts',(-33.0377626123296,-33.3068243195772,
46.7787490394258));
#25396=CARTESIAN_POINT('Ctrl Pts',(-33.4695919143871,-32.9639042362345,
46.7417057763526));
#25397=CARTESIAN_POINT('Ctrl Pts',(-33.7146396196904,-32.3857755125076,
46.7046625132793));
#25398=CARTESIAN_POINT('Ctrl Pts',(-33.6607732270088,-31.8369867176014,
46.6676192502061));
#25399=CARTESIAN_POINT('Ctrl Pts',(-33.6069068343271,-31.2881979226952,
46.6305759871328));
#25400=CARTESIAN_POINT('Ctrl Pts',(-33.2541263436604,-30.7687490566096,
46.5935327240596));
#25401=CARTESIAN_POINT('Ctrl Pts',(-32.7638621946652,-30.5163371038714,
46.5564894609864));
#25402=CARTESIAN_POINT('Ctrl Pts',(-32.27359804567,-30.2639251511331,46.5194461979131));
#25403=CARTESIAN_POINT('Ctrl Pts',(-31.6458502383462,-30.2785501117421,
46.4824029348399));
#25404=CARTESIAN_POINT('Ctrl Pts',(-31.1678727655046,-30.5535196830241,
46.4453596717666));
#25405=CARTESIAN_POINT('Ctrl Pts',(-30.6898952926629,-30.8284892543062,
46.4083164086933));
#25406=CARTESIAN_POINT('Ctrl Pts',(-30.3616881543033,-31.3638034362614,
46.3712731456201));
#25407=CARTESIAN_POINT('Ctrl Pts',(-30.3334371573101,-31.9145053618474,
46.3342298825469));
#25408=CARTESIAN_POINT('Ctrl Pts',(-30.3319855200674,-31.9428023959298,
46.3323264672345));
#25409=CARTESIAN_POINT('Ctrl Pts',(-30.3313258485816,-31.9711400578387,
46.3304230519221));
#25410=CARTESIAN_POINT('Ctrl Pts',(-30.3314412753146,-31.9994832045548,
46.3285196366098));
#25411=CARTESIAN_POINT('Origin',(-32.,-32.,48.));
#25412=CARTESIAN_POINT('',(-30.3357441857247,-31.9988063630956,45.6285196366098));
#25413=CARTESIAN_POINT('',(-30.3363139698042,-32.0008167216185,45.8214803633902));
#25414=CARTESIAN_POINT('',(-30.334,-32.,48.));
#25415=CARTESIAN_POINT('Ctrl Pts',(-30.3363139698042,-32.0008167216185,
45.8214803633902));
#25416=CARTESIAN_POINT('Ctrl Pts',(-30.3377789567259,-31.6705283252898,
45.8434953712468));
#25417=CARTESIAN_POINT('Ctrl Pts',(-30.4328915698991,-31.3394622789351,
45.8655103791034));
#25418=CARTESIAN_POINT('Ctrl Pts',(-30.6159865406001,-31.0676651762742,
45.8875253869599));
#25419=CARTESIAN_POINT('Ctrl Pts',(-30.9240688820304,-30.6103293605433,
45.9245686500332));
#25420=CARTESIAN_POINT('Ctrl Pts',(-31.4812527432153,-30.3207997319075,
45.9616119131064));
#25421=CARTESIAN_POINT('Ctrl Pts',(-32.0325738104803,-30.3315634785216,
45.9986551761797));
#25422=CARTESIAN_POINT('Ctrl Pts',(-32.5838948777453,-30.3423272251357,
46.0356984392529));
#25423=CARTESIAN_POINT('Ctrl Pts',(-33.1293531510904,-30.6533843469997,
46.0727417023262));
#25424=CARTESIAN_POINT('Ctrl Pts',(-33.4193498822572,-31.1223967917855,
46.1097849653994));
#25425=CARTESIAN_POINT('Ctrl Pts',(-33.709346613424,-31.5914092365713,46.1468282284727));
#25426=CARTESIAN_POINT('Ctrl Pts',(-33.7438818024125,-32.218377004279,46.1838714915459));
#25427=CARTESIAN_POINT('Ctrl Pts',(-33.5071523340008,-32.7164030439968,
46.2209147546191));
#25428=CARTESIAN_POINT('Ctrl Pts',(-33.2704228655892,-33.2144290837145,
46.2579580176924));
#25429=CARTESIAN_POINT('Ctrl Pts',(-32.7624287397773,-33.5835133954422,
46.2950012807656));
#25430=CARTESIAN_POINT('Ctrl Pts',(-32.2156253140534,-33.6547649994097,
46.3320445438389));
#25431=CARTESIAN_POINT('Ctrl Pts',(-31.6688218883294,-33.7260166033772,
46.3690878069121));
#25432=CARTESIAN_POINT('Ctrl Pts',(-31.0832091626933,-33.4994354995844,
46.4061310699853));
#25433=CARTESIAN_POINT('Ctrl Pts',(-30.7267603450434,-33.078703972542,46.4431743330586));
#25434=CARTESIAN_POINT('Ctrl Pts',(-30.4755937395586,-32.7822414673095,
46.4692763431691));
#25435=CARTESIAN_POINT('Ctrl Pts',(-30.3382096821063,-32.3893810168113,
46.4953783532797));
#25436=CARTESIAN_POINT('Ctrl Pts',(-30.3349857214592,-31.9985615244857,
46.5214803633902));
#25437=CARTESIAN_POINT('Ctrl Pts',(-30.3314412753146,-31.9994832045548,
46.3285196366098));
#25438=CARTESIAN_POINT('Ctrl Pts',(-30.3335722226689,-32.522739403137,46.2933797888489));
#25439=CARTESIAN_POINT('Ctrl Pts',(-30.5998767445262,-33.0478649663095,
46.258239941088));
#25440=CARTESIAN_POINT('Ctrl Pts',(-31.0242217896239,-33.3537348063572,
46.2231000933272));
#25441=CARTESIAN_POINT('Ctrl Pts',(-31.471552274558,-33.6761726560644,46.1860568302539));
#25442=CARTESIAN_POINT('Ctrl Pts',(-32.0945081000531,-33.7549586862622,
46.1490135671807));
#25443=CARTESIAN_POINT('Ctrl Pts',(-32.6080280581999,-33.5540408367315,
46.1119703041074));
#25444=CARTESIAN_POINT('Ctrl Pts',(-33.1215480163468,-33.3531229872009,
46.0749270410342));
#25445=CARTESIAN_POINT('Ctrl Pts',(-33.5256321071454,-32.8725012579417,
46.0378837779609));
#25446=CARTESIAN_POINT('Ctrl Pts',(-33.6353736417011,-32.3321055462003,
46.0008405148877));
#25447=CARTESIAN_POINT('Ctrl Pts',(-33.7451151762568,-31.7917098344589,
45.9637972518145));
#25448=CARTESIAN_POINT('Ctrl Pts',(-33.5605141545695,-31.1915401402351,
45.9267539887412));
#25449=CARTESIAN_POINT('Ctrl Pts',(-33.166043003206,-30.8062308613212,45.889710725668));
#25450=CARTESIAN_POINT('Ctrl Pts',(-32.7715718518426,-30.4209215824073,
45.8526674625947));
#25451=CARTESIAN_POINT('Ctrl Pts',(-32.1672305708029,-30.2504727188033,
45.8156241995215));
#25452=CARTESIAN_POINT('Ctrl Pts',(-31.6295624533867,-30.3728807462738,
45.7785809364483));
#25453=CARTESIAN_POINT('Ctrl Pts',(-31.0918943359704,-30.4952887737443,
45.741537673375));
#25454=CARTESIAN_POINT('Ctrl Pts',(-30.6208993821775,-30.9105536922893,
45.7044944103018));
#25455=CARTESIAN_POINT('Ctrl Pts',(-30.4321023289999,-31.428652526863,45.6674511472285));
#25456=CARTESIAN_POINT('Ctrl Pts',(-30.3659620570514,-31.6101553482161,
45.6544739770223));
#25457=CARTESIAN_POINT('Ctrl Pts',(-30.3344551994185,-31.8042787086015,
45.641496806816));
#25458=CARTESIAN_POINT('Ctrl Pts',(-30.3357441857247,-31.9988063630956,
45.6285196366098));
#25459=CARTESIAN_POINT('Origin',(-32.,-32.,48.));
#25460=CARTESIAN_POINT('',(-30.3357491875936,-32.001191282378,44.9285196366098));
#25461=CARTESIAN_POINT('',(-30.3320047816524,-32.0009960539197,45.1214803633902));
#25462=CARTESIAN_POINT('',(-30.334,-32.,48.));
#25463=CARTESIAN_POINT('Ctrl Pts',(-30.3320047816524,-32.0009960539197,
45.1214803633902));
#25464=CARTESIAN_POINT('Ctrl Pts',(-30.3354914992898,-31.5078412923967,
45.1545691261407));
#25465=CARTESIAN_POINT('Ctrl Pts',(-30.5679112651413,-31.011830923742,45.1876578888911));
#25466=CARTESIAN_POINT('Ctrl Pts',(-30.9509788634419,-30.7021956486487,
45.2207466516416));
#25467=CARTESIAN_POINT('Ctrl Pts',(-31.3798275915038,-30.35555527897,45.2577899147148));
#25468=CARTESIAN_POINT('Ctrl Pts',(-31.9974842806421,-30.2425000916246,
45.2948331777881));
#25469=CARTESIAN_POINT('Ctrl Pts',(-32.5213125790108,-30.4147635273256,
45.3318764408613));
#25470=CARTESIAN_POINT('Ctrl Pts',(-33.0451408773795,-30.5870269630266,
45.3689197039346));
#25471=CARTESIAN_POINT('Ctrl Pts',(-33.4751407849788,-31.044609021774,45.4059629670078));
#25472=CARTESIAN_POINT('Ctrl Pts',(-33.6145466756685,-31.5781226346204,
45.4430062300811));
#25473=CARTESIAN_POINT('Ctrl Pts',(-33.7539525663583,-32.1116362474668,
45.4800494931543));
#25474=CARTESIAN_POINT('Ctrl Pts',(-33.6027644401386,-32.7210814144121,
45.5170927562275));
#25475=CARTESIAN_POINT('Ctrl Pts',(-33.2301651637841,-33.1275793316411,
45.5541360193008));
#25476=CARTESIAN_POINT('Ctrl Pts',(-32.8575658874295,-33.53407724887,45.591179282374));
#25477=CARTESIAN_POINT('Ctrl Pts',(-32.2635554609402,-33.7376279163826,
45.6282225454473));
#25478=CARTESIAN_POINT('Ctrl Pts',(-31.7199498345901,-33.6450876524325,
45.6652658085205));
#25479=CARTESIAN_POINT('Ctrl Pts',(-31.17634420824,-33.5525473884824,45.7023090715937));
#25480=CARTESIAN_POINT('Ctrl Pts',(-30.6831433820292,-33.1639161930697,
45.739352334667));
#25481=CARTESIAN_POINT('Ctrl Pts',(-30.4660333797617,-32.6570295939504,
45.7763955977402));
#25482=CARTESIAN_POINT('Ctrl Pts',(-30.3779530041826,-32.4513883910573,
45.7914238529569));
#25483=CARTESIAN_POINT('Ctrl Pts',(-30.3353139157731,-32.2262837460894,
45.8064521081735));
#25484=CARTESIAN_POINT('Ctrl Pts',(-30.3363139698042,-32.0008167216185,
45.8214803633902));
#25485=CARTESIAN_POINT('Ctrl Pts',(-30.3357441857247,-31.9988063630956,
45.6285196366098));
#25486=CARTESIAN_POINT('Ctrl Pts',(-30.338134603948,-32.3595568598412,45.6044535437428));
#25487=CARTESIAN_POINT('Ctrl Pts',(-30.4533148635796,-32.7216977848527,
45.5803874508758));
#25488=CARTESIAN_POINT('Ctrl Pts',(-30.6695651499702,-33.0073153188619,
45.5563213580088));
#25489=CARTESIAN_POINT('Ctrl Pts',(-31.0024241766806,-33.4469465256848,
45.5192780949355));
#25490=CARTESIAN_POINT('Ctrl Pts',(-31.5747413826638,-33.7052761887284,
45.4822348318623));
#25491=CARTESIAN_POINT('Ctrl Pts',(-32.1246275177226,-33.6640940549181,
45.4451915687891));
#25492=CARTESIAN_POINT('Ctrl Pts',(-32.6745136527815,-33.6229119211079,
45.4081483057158));
#25493=CARTESIAN_POINT('Ctrl Pts',(-33.2019687169161,-33.2822179904438,
45.3711050426426));
#25494=CARTESIAN_POINT('Ctrl Pts',(-33.4656321327844,-32.7979119582619,
45.3340617795693));
#25495=CARTESIAN_POINT('Ctrl Pts',(-33.7292955486528,-32.3136059260799,
45.2970185164961));
#25496=CARTESIAN_POINT('Ctrl Pts',(-33.7291673162548,-31.6856877923802,
45.2599752534229));
#25497=CARTESIAN_POINT('Ctrl Pts',(-33.4653061140406,-31.2014894903992,
45.2229319903496));
#25498=CARTESIAN_POINT('Ctrl Pts',(-33.2014449118263,-30.7172911884183,
45.1858887272764));
#25499=CARTESIAN_POINT('Ctrl Pts',(-32.6738507397958,-30.3768127181562,
45.1488454642031));
#25500=CARTESIAN_POINT('Ctrl Pts',(-32.1239478303099,-30.3358551814373,
45.1118022011299));
#25501=CARTESIAN_POINT('Ctrl Pts',(-31.5740449208239,-30.2948976447184,
45.0747589380567));
#25502=CARTESIAN_POINT('Ctrl Pts',(-31.0018332738826,-30.5534610415427,
45.0377156749834));
#25503=CARTESIAN_POINT('Ctrl Pts',(-30.6691538364378,-30.993228163525,45.0006724119102));
#25504=CARTESIAN_POINT('Ctrl Pts',(-30.4531564439696,-31.2787539308252,
44.9766214868101));
#25505=CARTESIAN_POINT('Ctrl Pts',(-30.338132925853,-31.6406654260182,44.9525705617099));
#25506=CARTESIAN_POINT('Ctrl Pts',(-30.3357491875936,-32.001191282378,44.9285196366098));
#25507=CARTESIAN_POINT('Origin',(-32.,-32.,48.));
#25508=CARTESIAN_POINT('',(-30.3314442558758,-32.000520718743,44.2285196366098));
#25509=CARTESIAN_POINT('',(-30.3332944489024,-31.9985486373494,44.4214803633902));
#25510=CARTESIAN_POINT('',(-30.334,-32.,48.));
#25511=CARTESIAN_POINT('Ctrl Pts',(-30.3332944489024,-31.9985486373494,
44.4214803633902));
#25512=CARTESIAN_POINT('Ctrl Pts',(-30.3323221970028,-31.8922296275463,
44.4285996179613));
#25513=CARTESIAN_POINT('Ctrl Pts',(-30.3416240090201,-31.786080088522,44.4357188725324));
#25514=CARTESIAN_POINT('Ctrl Pts',(-30.3618163562289,-31.6820442977201,
44.4428381271035));
#25515=CARTESIAN_POINT('Ctrl Pts',(-30.4668821917387,-31.1407200440053,
44.4798813901768));
#25516=CARTESIAN_POINT('Ctrl Pts',(-30.8667963414239,-30.6566230145736,
44.51692465325));
#25517=CARTESIAN_POINT('Ctrl Pts',(-31.3785602588332,-30.4512733851868,
44.5539679163232));
#25518=CARTESIAN_POINT('Ctrl Pts',(-31.8903241762424,-30.2459237557999,
44.5910111793965));
#25519=CARTESIAN_POINT('Ctrl Pts',(-32.5139378613757,-30.3193215264579,
44.6280544424697));
#25520=CARTESIAN_POINT('Ctrl Pts',(-32.9640390733202,-30.6378802752901,
44.665097705543));
#25521=CARTESIAN_POINT('Ctrl Pts',(-33.4141402852647,-30.9564390241223,
44.7021409686162));
#25522=CARTESIAN_POINT('Ctrl Pts',(-33.6907290240204,-31.5201587511287,
44.7391842316894));
#25523=CARTESIAN_POINT('Ctrl Pts',(-33.6672397824729,-32.0710843658744,
44.7762274947627));
#25524=CARTESIAN_POINT('Ctrl Pts',(-33.6437505409253,-32.6220099806201,
44.8132707578359));
#25525=CARTESIAN_POINT('Ctrl Pts',(-33.3201833190745,-33.160141483105,44.8503140209092));
#25526=CARTESIAN_POINT('Ctrl Pts',(-32.844600723169,-33.4392328156884,44.8873572839824));
#25527=CARTESIAN_POINT('Ctrl Pts',(-32.3690181272635,-33.7183241482719,
44.9244005470557));
#25528=CARTESIAN_POINT('Ctrl Pts',(-31.7414201573035,-33.738375310954,44.9614438101289));
#25529=CARTESIAN_POINT('Ctrl Pts',(-31.2489922413343,-33.4902110004143,
44.9984870732021));
#25530=CARTESIAN_POINT('Ctrl Pts',(-30.7565643253651,-33.2420466898746,
45.0355303362754));
#25531=CARTESIAN_POINT('Ctrl Pts',(-30.3993064633867,-32.7256669061132,
45.0725735993486));
#25532=CARTESIAN_POINT('Ctrl Pts',(-30.3406979158904,-32.1773642382264,
45.1096168624219));
#25533=CARTESIAN_POINT('Ctrl Pts',(-30.3344412446157,-32.1188309747596,
45.1135713627446));
#25534=CARTESIAN_POINT('Ctrl Pts',(-30.3315880774641,-32.0599339077866,
45.1175258630674));
#25535=CARTESIAN_POINT('Ctrl Pts',(-30.3320047816524,-32.0009960539197,
45.1214803633902));
#25536=CARTESIAN_POINT('Ctrl Pts',(-30.3357491875936,-32.001191282378,44.9285196366098));
#25537=CARTESIAN_POINT('Ctrl Pts',(-30.3344614893875,-32.1959477732146,
44.9155272986367));
#25538=CARTESIAN_POINT('Ctrl Pts',(-30.3660440285482,-32.3902999106566,
44.9025349606636));
#25539=CARTESIAN_POINT('Ctrl Pts',(-30.4323358190322,-32.5719878123685,
44.8895426226904));
#25540=CARTESIAN_POINT('Ctrl Pts',(-30.6213444670197,-33.0900094920897,
44.8524993596172));
#25541=CARTESIAN_POINT('Ctrl Pts',(-31.0925089909431,-33.5050820043918,
44.8154560965439));
#25542=CARTESIAN_POINT('Ctrl Pts',(-31.6302270594382,-33.6272704182821,
44.7784128334707));
#25543=CARTESIAN_POINT('Ctrl Pts',(-32.1679451279333,-33.7494588321725,
44.7413695703975));
#25544=CARTESIAN_POINT('Ctrl Pts',(-32.7722167410002,-33.5787631476509,
44.7043263073243));
#25545=CARTESIAN_POINT('Ctrl Pts',(-33.1665304850258,-33.1932927843964,
44.667283044251));
#25546=CARTESIAN_POINT('Ctrl Pts',(-33.5608442290514,-32.807822421142,44.6302397811778));
#25547=CARTESIAN_POINT('Ctrl Pts',(-33.7452001040358,-32.2075773791546,
44.5931965181045));
#25548=CARTESIAN_POINT('Ctrl Pts',(-33.6352378612141,-31.6672265349532,
44.5561532550313));
#25549=CARTESIAN_POINT('Ctrl Pts',(-33.5252756183925,-31.1268756907518,
44.519109991958));
#25550=CARTESIAN_POINT('Ctrl Pts',(-33.1209952577648,-30.6464190443362,
44.4820667288848));
#25551=CARTESIAN_POINT('Ctrl Pts',(-32.6073932802354,-30.4457109519414,
44.4450234658115));
#25552=CARTESIAN_POINT('Ctrl Pts',(-32.093791302706,-30.2450028595466,44.4079802027383));
#25553=CARTESIAN_POINT('Ctrl Pts',(-31.470867708275,-30.3240433211725,44.370936939665));
#25554=CARTESIAN_POINT('Ctrl Pts',(-31.0236689560912,-30.6466638501528,
44.3338936765918));
#25555=CARTESIAN_POINT('Ctrl Pts',(-30.5996319852359,-30.9525748822755,
44.2987689965978));
#25556=CARTESIAN_POINT('Ctrl Pts',(-30.3335885954286,-31.4774878871477,
44.2636443166038));
#25557=CARTESIAN_POINT('Ctrl Pts',(-30.3314442558758,-32.000520718743,44.2285196366098));
#25558=CARTESIAN_POINT('Origin',(-32.,-32.,48.));
#25559=CARTESIAN_POINT('',(-30.3342156502641,-31.9984780271966,43.5285196366098));
#25560=CARTESIAN_POINT('',(-30.3367054145197,-31.9999190856858,43.7214803633902));
#25561=CARTESIAN_POINT('',(-30.334,-32.,48.));
#25562=CARTESIAN_POINT('Ctrl Pts',(-30.3367054145197,-31.9999190856858,
43.7214803633902));
#25563=CARTESIAN_POINT('Ctrl Pts',(-30.3365870778148,-31.7268111441588,
43.7396733728552));
#25564=CARTESIAN_POINT('Ctrl Pts',(-30.4000931167448,-31.4537550325403,
43.7578663823202));
#25565=CARTESIAN_POINT('Ctrl Pts',(-30.5275247375743,-31.2147878752588,
43.7760593917852));
#25566=CARTESIAN_POINT('Ctrl Pts',(-30.7869915983661,-30.7282205874178,
43.8131026548584));
#25567=CARTESIAN_POINT('Ctrl Pts',(-31.3114817673872,-30.3829796228422,
43.8501459179316));
#25568=CARTESIAN_POINT('Ctrl Pts',(-31.8609913872482,-30.3370453749637,
43.8871891810049));
#25569=CARTESIAN_POINT('Ctrl Pts',(-32.4105010071092,-30.2911111270853,
43.9242324440781));
#25570=CARTESIAN_POINT('Ctrl Pts',(-32.9850300778102,-30.544483595904,43.9612757071514));
#25571=CARTESIAN_POINT('Ctrl Pts',(-33.3216772118398,-30.9812209135267,
43.9983189702246));
#25572=CARTESIAN_POINT('Ctrl Pts',(-33.6583243458694,-31.4179582311494,
44.0353622332979));
#25573=CARTESIAN_POINT('Ctrl Pts',(-33.7570895432276,-32.0380603975761,
44.0724054963711));
#25574=CARTESIAN_POINT('Ctrl Pts',(-33.5727783851417,-32.5577720238224,
44.1094487594443));
#25575=CARTESIAN_POINT('Ctrl Pts',(-33.3884672270558,-33.0774836500687,
44.1464920225176));
#25576=CARTESIAN_POINT('Ctrl Pts',(-32.9210797135258,-33.4968047361345,
44.1835352855908));
#25577=CARTESIAN_POINT('Ctrl Pts',(-32.3844898364365,-33.6238562267059,
44.2205785486641));
#25578=CARTESIAN_POINT('Ctrl Pts',(-31.8478999593472,-33.7509077172772,
44.2576218117373));
#25579=CARTESIAN_POINT('Ctrl Pts',(-31.2421077186987,-33.585689612354,44.2946650748106));
#25580=CARTESIAN_POINT('Ctrl Pts',(-30.8443203590416,-33.2038048208934,
44.3317083378838));
#25581=CARTESIAN_POINT('Ctrl Pts',(-30.5229827838695,-32.895313538041,44.3616323463859));
#25582=CARTESIAN_POINT('Ctrl Pts',(-30.3373810669353,-32.4454340410825,
44.3915563548881));
#25583=CARTESIAN_POINT('Ctrl Pts',(-30.3332944489024,-31.9985486373494,
44.4214803633902));
#25584=CARTESIAN_POINT('Ctrl Pts',(-30.3314442558758,-32.000520718743,44.2285196366098));
#25585=CARTESIAN_POINT('Ctrl Pts',(-30.3313271275893,-32.0290898598927,
44.2266010535306));
#25586=CARTESIAN_POINT('Ctrl Pts',(-30.3319973610194,-32.0576533914107,
44.2246824704513));
#25587=CARTESIAN_POINT('Ctrl Pts',(-30.3334722154628,-32.0861753163795,
44.2227638873721));
#25588=CARTESIAN_POINT('Ctrl Pts',(-30.3619481369549,-32.6368656572913,
44.1857206242989));
#25589=CARTESIAN_POINT('Ctrl Pts',(-30.6903738898756,-33.1720457427803,
44.1486773612256));
#25590=CARTESIAN_POINT('Ctrl Pts',(-31.1684636305021,-33.4468200675988,
44.1116340981523));
#25591=CARTESIAN_POINT('Ctrl Pts',(-31.6465533711285,-33.7215943924173,
44.0745908350791));
#25592=CARTESIAN_POINT('Ctrl Pts',(-32.2743070994606,-33.7359629565652,
44.0375475720059));
#25593=CARTESIAN_POINT('Ctrl Pts',(-32.7644681132684,-33.4833507830407,
44.0005043089326));
#25594=CARTESIAN_POINT('Ctrl Pts',(-33.2546291270762,-33.2307386095162,
43.9634610458594));
#25595=CARTESIAN_POINT('Ctrl Pts',(-33.6071974263597,-32.7111456983192,
43.9264177827861));
#25596=CARTESIAN_POINT('Ctrl Pts',(-33.6608396690849,-32.1623349481554,
43.8893745197129));
#25597=CARTESIAN_POINT('Ctrl Pts',(-33.7144819118102,-31.6135241979915,
43.8523312566396));
#25598=CARTESIAN_POINT('Ctrl Pts',(-33.4691980979772,-31.0354956088606,
43.8152879935664));
#25599=CARTESIAN_POINT('Ctrl Pts',(-33.0372287708073,-30.6927519290839,
43.7782447304932));
#25600=CARTESIAN_POINT('Ctrl Pts',(-32.6052594436374,-30.3500082493071,
43.7412014674199));
#25601=CARTESIAN_POINT('Ctrl Pts',(-31.9866046031307,-30.2425494788845,
43.7041582043467));
#25602=CARTESIAN_POINT('Ctrl Pts',(-31.464357349772,-30.4195481681652,43.6671149412734));
#25603=CARTESIAN_POINT('Ctrl Pts',(-30.9421100964133,-30.596546857446,43.6300716782002));
#25604=CARTESIAN_POINT('Ctrl Pts',(-30.5162704302025,-31.0580030064301,
43.593028415127));
#25605=CARTESIAN_POINT('Ctrl Pts',(-30.3817002734078,-31.5927567841279,
43.5559851520537));
#25606=CARTESIAN_POINT('Ctrl Pts',(-30.3484415158263,-31.7249201603314,
43.5468299802391));
#25607=CARTESIAN_POINT('Ctrl Pts',(-30.3329741347624,-31.8615607154642,
43.5376748084244));
#25608=CARTESIAN_POINT('Ctrl Pts',(-30.3342156502641,-31.9984780271966,
43.5285196366098));
#25609=CARTESIAN_POINT('Origin',(-32.,-32.,48.));
#25610=CARTESIAN_POINT('',(-30.3366133246983,-32.0004154269571,42.8285196366098));
#25611=CARTESIAN_POINT('',(-30.3335913899458,-32.0014938639798,43.0214803633902));
#25612=CARTESIAN_POINT('',(-30.334,-32.,48.));
#25613=CARTESIAN_POINT('Ctrl Pts',(-30.3335913899458,-32.0014938639798,
43.0214803633902));
#25614=CARTESIAN_POINT('Ctrl Pts',(-30.3376271579769,-31.5642233339688,
43.050747127749));
#25615=CARTESIAN_POINT('Ctrl Pts',(-30.5143062321943,-31.1240664255995,
43.0800138921079));
#25616=CARTESIAN_POINT('Ctrl Pts',(-30.8231972488936,-30.8168361220973,
43.1092806564668));
#25617=CARTESIAN_POINT('Ctrl Pts',(-31.2141639800378,-30.4279713737721,
43.14632391954));
#25618=CARTESIAN_POINT('Ctrl Pts',(-31.816937431779,-30.2520582524214,43.1833671826133));
#25619=CARTESIAN_POINT('Ctrl Pts',(-32.355691742528,-30.3695936505264,43.2204104456865));
#25620=CARTESIAN_POINT('Ctrl Pts',(-32.8944460532771,-30.4871290486314,
43.2574537087598));
#25621=CARTESIAN_POINT('Ctrl Pts',(-33.3691812230342,-30.8981129661922,
43.294496971833));
#25622=CARTESIAN_POINT('Ctrl Pts',(-33.5626610114924,-31.4144813899901,
43.3315402349062));
#25623=CARTESIAN_POINT('Ctrl Pts',(-33.7561407999506,-31.930849813788,43.3685834979795));
#25624=CARTESIAN_POINT('Ctrl Pts',(-33.6683652071101,-32.552602743823,43.4056267610527));
#25625=CARTESIAN_POINT('Ctrl Pts',(-33.3394998687003,-32.9952294111363,
43.442670024126));
#25626=CARTESIAN_POINT('Ctrl Pts',(-33.0106345302905,-33.4378560784496,
43.4797132871992));
#25627=CARTESIAN_POINT('Ctrl Pts',(-32.4406794463115,-33.7013564830411,
43.5167565502725));
#25628=CARTESIAN_POINT('Ctrl Pts',(-31.8904429725427,-33.6651542682835,
43.5537998133457));
#25629=CARTESIAN_POINT('Ctrl Pts',(-31.340206498774,-33.628952053526,43.5908430764189));
#25630=CARTESIAN_POINT('Ctrl Pts',(-30.8096886352155,-33.2930472194193,
43.6278863394922));
#25631=CARTESIAN_POINT('Ctrl Pts',(-30.5416514797176,-32.8111479968127,
43.6649296025654));
#25632=CARTESIAN_POINT('Ctrl Pts',(-30.405255062707,-32.5659233106992,43.6837798561737));
#25633=CARTESIAN_POINT('Ctrl Pts',(-30.3368280262791,-32.2828933769994,
43.7026301097819));
#25634=CARTESIAN_POINT('Ctrl Pts',(-30.3367054145197,-31.9999190856858,
43.7214803633902));
#25635=CARTESIAN_POINT('Ctrl Pts',(-30.3342156502641,-31.9984780271966,
43.5285196366098));
#25636=CARTESIAN_POINT('Ctrl Pts',(-30.3379975014744,-32.4155496629652,
43.5006315453512));
#25637=CARTESIAN_POINT('Ctrl Pts',(-30.4968224208937,-32.8351893433793,
43.4727434540926));
#25638=CARTESIAN_POINT('Ctrl Pts',(-30.7800935571206,-33.1386699755361,
43.444855362834));
#25639=CARTESIAN_POINT('Ctrl Pts',(-31.156357645007,-33.5417779828347,43.4078120997607));
#25640=CARTESIAN_POINT('Ctrl Pts',(-31.7521864681585,-33.7399425910204,
43.3707688366875));
#25641=CARTESIAN_POINT('Ctrl Pts',(-32.2949319879635,-33.6424847524125,
43.3337255736143));
#25642=CARTESIAN_POINT('Ctrl Pts',(-32.8376775077686,-33.5450269138045,
43.296682310541));
#25643=CARTESIAN_POINT('Ctrl Pts',(-33.3273397242272,-33.151946628403,43.2596390474678));
#25644=CARTESIAN_POINT('Ctrl Pts',(-33.5398518619426,-32.6431152984257,
43.2225957843945));
#25645=CARTESIAN_POINT('Ctrl Pts',(-33.7523639996579,-32.1342839684484,
43.1855525213213));
#25646=CARTESIAN_POINT('Ctrl Pts',(-33.6877260586298,-31.5097015938952,
43.1485092582481));
#25647=CARTESIAN_POINT('Ctrl Pts',(-33.37551601064,-31.0551736925882,43.1114659951748));
#25648=CARTESIAN_POINT('Ctrl Pts',(-33.0633059626503,-30.6006457912812,
43.0744227321016));
#25649=CARTESIAN_POINT('Ctrl Pts',(-32.5035238076987,-30.3161723632205,
43.0373794690283));
#25650=CARTESIAN_POINT('Ctrl Pts',(-31.9523228237046,-30.3319268870294,
43.0003362059551));
#25651=CARTESIAN_POINT('Ctrl Pts',(-31.4011218397105,-30.3476814108382,
42.9632929428818));
#25652=CARTESIAN_POINT('Ctrl Pts',(-30.8585020266738,-30.6636638865167,
42.9262496798086));
#25653=CARTESIAN_POINT('Ctrl Pts',(-30.5727632705769,-31.1352824852655,
42.8892064167354));
#25654=CARTESIAN_POINT('Ctrl Pts',(-30.4167244155916,-31.3928283188926,
42.8689774900268));
#25655=CARTESIAN_POINT('Ctrl Pts',(-30.3372909438258,-31.6967869359013,
42.8487485633183));
#25656=CARTESIAN_POINT('Ctrl Pts',(-30.3366133246983,-32.0004154269571,
42.8285196366098));
#25657=CARTESIAN_POINT('Origin',(-32.,-32.,48.));
#25658=CARTESIAN_POINT('',(-30.3326929969897,-32.0013037885424,42.1285196366098));
#25659=CARTESIAN_POINT('',(-30.3317921677919,-31.9991447210974,42.3214803633902));
#25660=CARTESIAN_POINT('',(-30.334,-32.,48.));
#25661=CARTESIAN_POINT('Ctrl Pts',(-30.3317921677919,-31.9991447210974,
42.3214803633902));
#25662=CARTESIAN_POINT('Ctrl Pts',(-30.3314846178305,-31.9500189154433,
42.3247776195697));
#25663=CARTESIAN_POINT('Ctrl Pts',(-30.3334665928779,-31.9009182758191,
42.3280748757492));
#25664=CARTESIAN_POINT('Ctrl Pts',(-30.3378188581809,-31.8520286465018,
42.3313721319287));
#25665=CARTESIAN_POINT('Ctrl Pts',(-30.3867146975717,-31.3027745692444,
42.368415395002));
#25666=CARTESIAN_POINT('Ctrl Pts',(-30.7347781808911,-30.7801532877911,
42.4054586580752));
#25667=CARTESIAN_POINT('Ctrl Pts',(-31.2227371636538,-30.5233132282111,
42.4425019211484));
#25668=CARTESIAN_POINT('Ctrl Pts',(-31.7106961464166,-30.266473168631,42.4795451842217));
#25669=CARTESIAN_POINT('Ctrl Pts',(-32.3385506286227,-30.2754143309243,
42.5165884472949));
#25670=CARTESIAN_POINT('Ctrl Pts',(-32.8189978954459,-30.5460454081846,
42.5536317103682));
#25671=CARTESIAN_POINT('Ctrl Pts',(-33.2994451622691,-30.8166764854448,
42.5906749734414));
#25672=CARTESIAN_POINT('Ctrl Pts',(-33.6324852137093,-31.348997477672,42.6277182365146));
#25673=CARTESIAN_POINT('Ctrl Pts',(-33.6657206816788,-31.8994211243615,
42.6647614995879));
#25674=CARTESIAN_POINT('Ctrl Pts',(-33.6989561496482,-32.4498447710511,
42.7018047626611));
#25675=CARTESIAN_POINT('Ctrl Pts',(-33.4323870341469,-33.018371072203,42.7388480257344));
#25676=CARTESIAN_POINT('Ctrl Pts',(-32.987993940445,-33.3448455058512,42.7758912888076));
#25677=CARTESIAN_POINT('Ctrl Pts',(-32.5436008467431,-33.6713199394994,
42.8129345518808));
#25678=CARTESIAN_POINT('Ctrl Pts',(-31.9213837748406,-33.7557425056438,
42.8499778149541));
#25679=CARTESIAN_POINT('Ctrl Pts',(-31.4060658711755,-33.559481880255,42.8870210780273));
#25680=CARTESIAN_POINT('Ctrl Pts',(-30.8907479675104,-33.3632212548662,
42.9240643411006));
#25681=CARTESIAN_POINT('Ctrl Pts',(-30.4823292320827,-32.8862774379442,
42.9611076041738));
#25682=CARTESIAN_POINT('Ctrl Pts',(-30.3676998696425,-32.3468973418332,
42.9981508672471));
#25683=CARTESIAN_POINT('Ctrl Pts',(-30.3436357074793,-32.2336651836491,
43.0059273659614));
#25684=CARTESIAN_POINT('Ctrl Pts',(-30.3325190423327,-32.1176814162753,
43.0137038646758));
#25685=CARTESIAN_POINT('Ctrl Pts',(-30.3335913899458,-32.0014938639798,
43.0214803633902));
#25686=CARTESIAN_POINT('Ctrl Pts',(-30.3366133246983,-32.0004154269571,
42.8285196366098));
#25687=CARTESIAN_POINT('Ctrl Pts',(-30.3360500859214,-32.2527922164965,
42.8117053002451));
#25688=CARTESIAN_POINT('Ctrl Pts',(-30.3898990887803,-32.5049409227568,
42.7948909638803));
#25689=CARTESIAN_POINT('Ctrl Pts',(-30.4993952962616,-32.7300182145042,
42.7780766275156));
#25690=CARTESIAN_POINT('Ctrl Pts',(-30.7406237772002,-33.2258806231749,
42.7410333644424));
#25691=CARTESIAN_POINT('Ctrl Pts',(-31.2519384382344,-33.5903507186974,
42.7039901013692));
#25692=CARTESIAN_POINT('Ctrl Pts',(-31.7993644698996,-33.6566491133687,
42.6669468382959));
#25693=CARTESIAN_POINT('Ctrl Pts',(-32.3467905015648,-33.7229475080399,
42.6299035752227));
#25694=CARTESIAN_POINT('Ctrl Pts',(-32.9303279038609,-33.4910742018599,
42.5928603121494));
#25695=CARTESIAN_POINT('Ctrl Pts',(-33.2829531118668,-33.0671328620635,
42.5558170490762));
#25696=CARTESIAN_POINT('Ctrl Pts',(-33.6355783198726,-32.6431915222671,
42.5187737860029));
#25697=CARTESIAN_POINT('Ctrl Pts',(-33.7572913335882,-32.0271821488543,
42.4817305229297));
#25698=CARTESIAN_POINT('Ctrl Pts',(-33.5923969650778,-31.5009878855554,
42.4446872598564));
#25699=CARTESIAN_POINT('Ctrl Pts',(-33.4275025965674,-30.9747936222564,
42.4076439967832));
#25700=CARTESIAN_POINT('Ctrl Pts',(-32.9760008458309,-30.5384144690715,
42.3706007337099));
#25701=CARTESIAN_POINT('Ctrl Pts',(-32.4444964120379,-30.3915339832607,
42.3335574706367));
#25702=CARTESIAN_POINT('Ctrl Pts',(-31.9129919782449,-30.24465349745,42.2965142075635));
#25703=CARTESIAN_POINT('Ctrl Pts',(-31.3014848613954,-30.3872716790136,
42.2594709444902));
#25704=CARTESIAN_POINT('Ctrl Pts',(-30.8897975089001,-30.7541295513978,
42.222427681417));
#25705=CARTESIAN_POINT('Ctrl Pts',(-30.5419092008583,-31.0641355881196,
42.1911249998146));
#25706=CARTESIAN_POINT('Ctrl Pts',(-30.3367074496864,-31.5342658723109,
42.1598223182122));
#25707=CARTESIAN_POINT('Ctrl Pts',(-30.3326929969897,-32.0013037885424,
42.1285196366098));
#25708=CARTESIAN_POINT('Origin',(-32.,-32.,48.));
#25709=CARTESIAN_POINT('',(-30.3325261502749,-31.9987897978733,41.4285196366098));
#25710=CARTESIAN_POINT('',(-30.336158884875,-31.9990545752999,41.6214803633902));
#25711=CARTESIAN_POINT('',(-30.334,-32.,48.));
#25712=CARTESIAN_POINT('',(-33.2690708798524,-30.9206413469515,41.));
#25713=CARTESIAN_POINT('Ctrl Pts',(-30.3325261502749,-31.9987897978733,
41.4285196366098));
#25714=CARTESIAN_POINT('Ctrl Pts',(-30.3364618898858,-32.4716719965804,
41.3968095469596));
#25715=CARTESIAN_POINT('Ctrl Pts',(-30.547679155389,-32.9475346897789,41.3650994573094));
#25716=CARTESIAN_POINT('Ctrl Pts',(-30.903524458539,-33.2578207687041,41.3333893676592));
#25717=CARTESIAN_POINT('Ctrl Pts',(-31.3192177386076,-33.6202924291878,
41.2963461045859));
#25718=CARTESIAN_POINT('Ctrl Pts',(-31.9322786939314,-33.7568087910484,
41.2593028415127));
#25719=CARTESIAN_POINT('Ctrl Pts',(-32.4621353665983,-33.6037827270274,
41.2222595784395));
#25720=CARTESIAN_POINT('Ctrl Pts',(-32.9919920392653,-33.4507566630064,
41.1852163153662));
#25721=CARTESIAN_POINT('Ctrl Pts',(-33.4386444292754,-33.0081881731037,
41.148173052293));
#25722=CARTESIAN_POINT('Ctrl Pts',(-33.5976357065192,-32.4811507187836,
41.1111297892197));
#25723=CARTESIAN_POINT('Ctrl Pts',(-33.7566269837631,-31.9541132644636,
41.0740865261465));
#25724=CARTESIAN_POINT('Ctrl Pts',(-33.6279571482407,-31.3426068457263,
41.0370432630732));
#25725=CARTESIAN_POINT('Ctrl Pts',(-33.2690708798524,-30.9206413469515,
41.));
#25726=CARTESIAN_POINT('',(-30.7285328693903,-30.9187901141545,41.));
#25727=CARTESIAN_POINT('Origin',(-32.,-32.,41.));
#25728=CARTESIAN_POINT('Ctrl Pts',(-30.7285315473809,-30.918789092831,41.));
#25729=CARTESIAN_POINT('Ctrl Pts',(-31.0793196250029,-30.5073509960358,
41.0363148168372));
#25730=CARTESIAN_POINT('Ctrl Pts',(-31.6491071295587,-30.2813272422374,
41.0726296336745));
#25731=CARTESIAN_POINT('Ctrl Pts',(-32.1864002131136,-30.3417998878807,
41.1089444505117));
#25732=CARTESIAN_POINT('Ctrl Pts',(-32.7344709670091,-30.403485566521,41.1459877135849));
#25733=CARTESIAN_POINT('Ctrl Pts',(-33.2487306007817,-30.7632767007414,
41.1830309766582));
#25734=CARTESIAN_POINT('Ctrl Pts',(-33.4941904839029,-31.2569744981691,
41.2200742397314));
#25735=CARTESIAN_POINT('Ctrl Pts',(-33.739650367024,-31.7506722955968,41.2571175028047));
#25736=CARTESIAN_POINT('Ctrl Pts',(-33.7163104994937,-32.378276756232,41.2941607658779));
#25737=CARTESIAN_POINT('Ctrl Pts',(-33.4346827711206,-32.8523785277167,
41.3312040289511));
#25738=CARTESIAN_POINT('Ctrl Pts',(-33.1530550427475,-33.3264802992015,
41.3682472920244));
#25739=CARTESIAN_POINT('Ctrl Pts',(-32.6131394535318,-33.6470793815359,
41.4052905550977));
#25740=CARTESIAN_POINT('Ctrl Pts',(-32.0620834355512,-33.6675828812401,
41.4423338181709));
#25741=CARTESIAN_POINT('Ctrl Pts',(-31.5110274175706,-33.6880863809443,
41.4793770812442));
#25742=CARTESIAN_POINT('Ctrl Pts',(-30.9488309708251,-33.4084942980185,
41.5164203443174));
#25743=CARTESIAN_POINT('Ctrl Pts',(-30.6327092175202,-32.9566901398629,
41.5534636073906));
#25744=CARTESIAN_POINT('Ctrl Pts',(-30.4392275569172,-32.6801643460085,
41.5761358593905));
#25745=CARTESIAN_POINT('Ctrl Pts',(-30.3379261292159,-32.3391274519624,
41.5988081113903));
#25746=CARTESIAN_POINT('Ctrl Pts',(-30.336158884875,-31.9990545752999,41.6214803633902));
#25747=CARTESIAN_POINT('Origin',(-32.,-32.,39.4540747194623));
#25748=CARTESIAN_POINT('',(-29.946715297465,-31.9981685983364,53.7459252805377));
#25749=CARTESIAN_POINT('',(-29.9453611647571,-32.0018310237742,53.8040747194623));
#25750=CARTESIAN_POINT('',(-29.94525,-31.9999999999998,39.4540747194623));
#25751=CARTESIAN_POINT('',(-32.3836679988468,-29.9813874990081,54.));
#25752=CARTESIAN_POINT('Ctrl Pts',(-29.9453611647571,-32.0018310237742,
53.8040747194623));
#25753=CARTESIAN_POINT('Ctrl Pts',(-29.950627974885,-31.4803614070367,53.832339883235));
#25754=CARTESIAN_POINT('Ctrl Pts',(-30.4182836665071,-30.2677806430719,
53.8976483100809));
#25755=CARTESIAN_POINT('Ctrl Pts',(-31.7124802469751,-29.853818061345,53.9629567369268));
#25756=CARTESIAN_POINT('Ctrl Pts',(-32.3836679988468,-29.9813874990081,
54.));
#25757=CARTESIAN_POINT('',(-33.3415658621448,-30.43873672012,54.));
#25758=CARTESIAN_POINT('Origin',(-32.,-32.,54.));
#25759=CARTESIAN_POINT('Ctrl Pts',(-29.946715297465,-31.9981685983364,53.7459252805377));
#25760=CARTESIAN_POINT('Ctrl Pts',(-29.9450488863716,-31.7888166485938,
53.7572587737813));
#25761=CARTESIAN_POINT('Ctrl Pts',(-30.0707451223458,-30.8972175670589,
53.8056355300982));
#25762=CARTESIAN_POINT('Ctrl Pts',(-31.3453228233254,-29.6694106382552,
53.8903271032523));
#25763=CARTESIAN_POINT('Ctrl Pts',(-32.8352372258873,-30.0047894254256,
53.9636851831628));
#25764=CARTESIAN_POINT('Ctrl Pts',(-33.3415672767799,-30.4387352221184,
54.));
#25765=CARTESIAN_POINT('Origin',(-32.,-32.,39.4540747194623));
#25766=CARTESIAN_POINT('',(-29.9479916133119,-32.0011056334653,53.0459252805377));
#25767=CARTESIAN_POINT('',(-29.94219064225,-31.9992426220948,53.1040747194623));
#25768=CARTESIAN_POINT('',(-29.94525,-31.9999999999998,39.4540747194623));
#25769=CARTESIAN_POINT('Ctrl Pts',(-29.94219064225,-31.9992426220948,53.1040747194623));
#25770=CARTESIAN_POINT('Ctrl Pts',(-29.9419903899876,-31.957076450319,53.1063703750556));
#25771=CARTESIAN_POINT('Ctrl Pts',(-29.9622810278528,-31.2347025931292,
53.1457092937222));
#25772=CARTESIAN_POINT('Ctrl Pts',(-30.811328806025,-29.8822030832705,53.2220914754619));
#25773=CARTESIAN_POINT('Ctrl Pts',(-33.1343255681424,-29.8526923031888,
53.3332212646816));
#25774=CARTESIAN_POINT('Ctrl Pts',(-34.4195104145668,-31.7882159864216,
53.4443510539014));
#25775=CARTESIAN_POINT('Ctrl Pts',(-33.4897707765082,-33.9178754505755,
53.555480843121));
#25776=CARTESIAN_POINT('Ctrl Pts',(-31.1978269047507,-34.2916948256168,
53.6666106323409));
#25777=CARTESIAN_POINT('Ctrl Pts',(-30.0344356552593,-33.0074711411215,
53.7494752577879));
#25778=CARTESIAN_POINT('Ctrl Pts',(-29.9437254911529,-32.1637799201182,
53.7952966201617));
#25779=CARTESIAN_POINT('Ctrl Pts',(-29.9453611647571,-32.0018310237742,
53.8040747194623));
#25780=CARTESIAN_POINT('Ctrl Pts',(-29.9479916133119,-32.0011056334653,
53.0459252805377));
#25781=CARTESIAN_POINT('Ctrl Pts',(-29.9500185021419,-31.5865449050144,
53.0683325286752));
#25782=CARTESIAN_POINT('Ctrl Pts',(-30.2732452755414,-30.4837342237769,
53.127783039886));
#25783=CARTESIAN_POINT('Ctrl Pts',(-32.0730427793273,-29.5725272947448,
53.2242768141699));
#25784=CARTESIAN_POINT('Ctrl Pts',(-34.0790039218848,-30.7446672388737,
53.3354066033898));
#25785=CARTESIAN_POINT('Ctrl Pts',(-34.1822410279863,-33.0657522628949,
53.4465363926093));
#25786=CARTESIAN_POINT('Ctrl Pts',(-32.2883983467057,-34.4113176464284,
53.5576661818292));
#25787=CARTESIAN_POINT('Ctrl Pts',(-30.3505279516326,-33.6381799778053,
53.6574624778052));
#25788=CARTESIAN_POINT('Ctrl Pts',(-29.9504955128613,-32.4730787011233,
53.7202155107081));
#25789=CARTESIAN_POINT('Ctrl Pts',(-29.946715297465,-31.9981685983364,53.7459252805377));
#25790=CARTESIAN_POINT('Origin',(-32.,-32.,39.4540747194623));
#25791=CARTESIAN_POINT('',(-29.942628805933,-32.0011268474386,52.3459252805377));
#25792=CARTESIAN_POINT('',(-29.9475562677021,-31.9986057848623,52.4040747194623));
#25793=CARTESIAN_POINT('',(-29.94525,-31.9999999999998,39.4540747194623));
#25794=CARTESIAN_POINT('Ctrl Pts',(-29.9475562677021,-31.9986057848623,
52.4040747194624));
#25795=CARTESIAN_POINT('Ctrl Pts',(-29.9460125514017,-31.7513877791255,
52.4174441299495));
#25796=CARTESIAN_POINT('Ctrl Pts',(-30.1017872484456,-30.8210709304397,
52.46785680351));
#25797=CARTESIAN_POINT('Ctrl Pts',(-31.4859339874079,-29.6264478597178,
52.5553127401435));
#25798=CARTESIAN_POINT('Ctrl Pts',(-33.7152268510116,-30.2806972438647,
52.6664425293633));
#25799=CARTESIAN_POINT('Ctrl Pts',(-34.3747678628917,-32.5084312351377,
52.777572318583));
#25800=CARTESIAN_POINT('Ctrl Pts',(-32.8609368628007,-34.2708596802663,
52.8887021078028));
#25801=CARTESIAN_POINT('Ctrl Pts',(-30.6067538461013,-33.961536273617,52.9975362414292));
#25802=CARTESIAN_POINT('Ctrl Pts',(-29.9452217097288,-32.6374801652532,
53.0693271119824));
#25803=CARTESIAN_POINT('Ctrl Pts',(-29.94219064225,-31.9992426220948,53.1040747194623));
#25804=CARTESIAN_POINT('Ctrl Pts',(-29.942628805933,-32.0011268474386,52.3459252805377));
#25805=CARTESIAN_POINT('Ctrl Pts',(-29.9466920764506,-31.3858139005692,
52.3794062835691));
#25806=CARTESIAN_POINT('Ctrl Pts',(-30.5667600036778,-30.0826171398043,
52.4499305496737));
#25807=CARTESIAN_POINT('Ctrl Pts',(-32.7830045778855,-29.7011054025381,
52.5574980788515));
#25808=CARTESIAN_POINT('Ctrl Pts',(-34.3560464702414,-31.4108820816923,
52.6686278680714));
#25809=CARTESIAN_POINT('Ctrl Pts',(-33.7728594827364,-33.6598143885419,
52.779757657291));
#25810=CARTESIAN_POINT('Ctrl Pts',(-31.5671721094895,-34.389699997922,52.8908874465108));
#25811=CARTESIAN_POINT('Ctrl Pts',(-30.1224675495405,-33.2263676194101,
52.979609987593));
#25812=CARTESIAN_POINT('Ctrl Pts',(-29.94666768567,-32.2718893091822,53.031289265602));
#25813=CARTESIAN_POINT('Ctrl Pts',(-29.9479916133119,-32.0011056334653,
53.0459252805377));
#25814=CARTESIAN_POINT('Origin',(-32.,-32.,39.4540747194623));
#25815=CARTESIAN_POINT('',(-29.9445978953396,-31.9981759025628,51.6459252805377));
#25816=CARTESIAN_POINT('',(-29.9472436367207,-32.0015414516679,51.7040747194623));
#25817=CARTESIAN_POINT('',(-29.94525,-31.9999999999998,39.4540747194623));
#25818=CARTESIAN_POINT('Ctrl Pts',(-29.9472436367207,-32.0015414516679,
51.7040747194623));
#25819=CARTESIAN_POINT('Ctrl Pts',(-29.9503946641538,-31.549728231468,51.7285178848434));
#25820=CARTESIAN_POINT('Ctrl Pts',(-30.3199519211819,-30.4085132585972,
51.7900043132977));
#25821=CARTESIAN_POINT('Ctrl Pts',(-32.2059544087099,-29.5801662395198,
51.8885340048252));
#25822=CARTESIAN_POINT('Ctrl Pts',(-34.1446539207691,-30.8604948262468,
51.9996637940449));
#25823=CARTESIAN_POINT('Ctrl Pts',(-34.1205895081331,-33.1836861468564,
52.1107935832646));
#25824=CARTESIAN_POINT('Ctrl Pts',(-32.1557844046688,-34.4235808289435,
52.2219233724844));
#25825=CARTESIAN_POINT('Ctrl Pts',(-30.3019343102738,-33.5631151086926,
52.3196837512169));
#25826=CARTESIAN_POINT('Ctrl Pts',(-29.9502897997577,-32.4363664946596,
52.3804008668763));
#25827=CARTESIAN_POINT('Ctrl Pts',(-29.9475562677021,-31.9986057848623,
52.4040747194624));
#25828=CARTESIAN_POINT('Ctrl Pts',(-29.9445978953396,-31.9981759025628,
51.6459252805377));
#25829=CARTESIAN_POINT('Ctrl Pts',(-29.943323539856,-31.8597856808618,51.6534367753897));
#25830=CARTESIAN_POINT('Ctrl Pts',(-30.0191495440249,-31.0403066328242,
51.697991533315));
#25831=CARTESIAN_POINT('Ctrl Pts',(-31.119458497007,-29.7366705485938,51.7795895543135));
#25832=CARTESIAN_POINT('Ctrl Pts',(-33.4238507688844,-30.0326000635722,
51.8907193435332));
#25833=CARTESIAN_POINT('Ctrl Pts',(-34.4251502639725,-32.1290726539236,
52.001849132753));
#25834=CARTESIAN_POINT('Ctrl Pts',(-33.2069785255006,-34.1074193726832,
52.1129789219726));
#25835=CARTESIAN_POINT('Ctrl Pts',(-30.8841931526569,-34.1570786929198,
52.2241087111924));
#25836=CARTESIAN_POINT('Ctrl Pts',(-29.9747293436638,-32.8124059711623,
52.3017574973807));
#25837=CARTESIAN_POINT('Ctrl Pts',(-29.942196488353,-32.0665939638752,52.3423630204958));
#25838=CARTESIAN_POINT('Ctrl Pts',(-29.942628805933,-32.0011268474386,52.3459252805377));
#25839=CARTESIAN_POINT('Origin',(-32.,-32.,39.4540747194623));
#25840=CARTESIAN_POINT('',(-29.9485909369504,-32.000019327896,50.9459252805377));
#25841=CARTESIAN_POINT('',(-29.9420109978713,-32.0005154328236,51.0040747194623));
#25842=CARTESIAN_POINT('',(-29.94525,-31.9999999999998,39.4540747194623));
#25843=CARTESIAN_POINT('Ctrl Pts',(-29.9420109978713,-32.0005154328236,
51.0040747194623));
#25844=CARTESIAN_POINT('Ctrl Pts',(-29.944207079629,-31.3483062578826,51.0395916397372));
#25845=CARTESIAN_POINT('Ctrl Pts',(-30.6316982652924,-30.0118743248253,
51.1121518230855));
#25846=CARTESIAN_POINT('Ctrl Pts',(-32.9077975170184,-29.7474644773485,
51.2217552695068));
#25847=CARTESIAN_POINT('Ctrl Pts',(-34.3847873913407,-31.54086852875,51.3328850587266));
#25848=CARTESIAN_POINT('Ctrl Pts',(-33.6792457084763,-33.7544647228394,
51.4440148479463));
#25849=CARTESIAN_POINT('Ctrl Pts',(-31.4368765610531,-34.3623938304022,
51.5551446371661));
#25850=CARTESIAN_POINT('Ctrl Pts',(-30.0897291770567,-33.150114152176,51.6418312610047));
#25851=CARTESIAN_POINT('Ctrl Pts',(-29.9456193277218,-32.2344446221205,
51.6914746217701));
#25852=CARTESIAN_POINT('Ctrl Pts',(-29.9472436367207,-32.0015414516679,
51.7040747194623));
#25853=CARTESIAN_POINT('Ctrl Pts',(-29.9485909369504,-32.000019327896,50.9459252805377));
#25854=CARTESIAN_POINT('Ctrl Pts',(-29.9486198100036,-31.6559195346657,
50.9645105302836));
#25855=CARTESIAN_POINT('Ctrl Pts',(-30.1938071310638,-30.6259372284373,
51.0201390431027));
#25856=CARTESIAN_POINT('Ctrl Pts',(-31.8232699653508,-29.5778563144268,
51.1128108189952));
#25857=CARTESIAN_POINT('Ctrl Pts',(-33.9390244464751,-30.5377422476497,
51.2239406082148));
#25858=CARTESIAN_POINT('Ctrl Pts',(-34.2802047821274,-32.8358706181179,
51.3350703974346));
#25859=CARTESIAN_POINT('Ctrl Pts',(-32.5345664287748,-34.3690192638818,
51.4462001866543));
#25860=CARTESIAN_POINT('Ctrl Pts',(-30.4507580622789,-33.7769849094658,
51.549818481022));
#25861=CARTESIAN_POINT('Ctrl Pts',(-29.9496080792662,-32.5422630692145,
51.6163935123165));
#25862=CARTESIAN_POINT('Ctrl Pts',(-29.9445978953396,-31.9981759025628,
51.6459252805377));
#25863=CARTESIAN_POINT('Origin',(-32.,-32.,39.4540747194623));
#25864=CARTESIAN_POINT('',(-29.9445269623743,-32.0018139479035,50.2459252805377));
#25865=CARTESIAN_POINT('',(-29.9457313039573,-31.9981314910653,50.3040747194623));
#25866=CARTESIAN_POINT('',(-29.94525,-31.9999999999998,39.4540747194623));
#25867=CARTESIAN_POINT('Ctrl Pts',(-29.9457313039573,-31.9981314910653,
50.3040747194623));
#25868=CARTESIAN_POINT('Ctrl Pts',(-29.9441559546048,-31.8219835628476,
50.3136221315579));
#25869=CARTESIAN_POINT('Ctrl Pts',(-30.04551831087,-30.9641799638719,50.3602128067267));
#25870=CARTESIAN_POINT('Ctrl Pts',(-31.2448019668464,-29.6918213798318,
50.4438467449688));
#25871=CARTESIAN_POINT('Ctrl Pts',(-33.5295162933197,-30.1135767918179,
50.5549765341885));
#25872=CARTESIAN_POINT('Ctrl Pts',(-34.4144338950484,-32.2617662665304,
50.6661063234082));
#25873=CARTESIAN_POINT('Ctrl Pts',(-33.0896877794978,-34.1703900928393,
50.7772361126279));
#25874=CARTESIAN_POINT('Ctrl Pts',(-30.7676712252758,-34.0926964431059,
50.8883659018477));
#25875=CARTESIAN_POINT('Ctrl Pts',(-29.9551340369839,-32.736719821345,50.9639787707924));
#25876=CARTESIAN_POINT('Ctrl Pts',(-29.9419166210631,-32.0285441799519,
51.002548376664));
#25877=CARTESIAN_POINT('Ctrl Pts',(-29.9420109978713,-32.0005154328236,
51.0040747194623));
#25878=CARTESIAN_POINT('Ctrl Pts',(-29.9445269623743,-32.0018139479035,
50.2459252805377));
#25879=CARTESIAN_POINT('Ctrl Pts',(-29.9495493412608,-31.4554311203763,
50.2755842851775));
#25880=CARTESIAN_POINT('Ctrl Pts',(-30.4542942197084,-30.2184357035796,
50.3422865528905));
#25881=CARTESIAN_POINT('Ctrl Pts',(-32.5426800429829,-29.6328261767372,
50.4460320836768));
#25882=CARTESIAN_POINT('Ctrl Pts',(-34.2830552647223,-31.1719467427689,
50.5571618728965));
#25883=CARTESIAN_POINT('Ctrl Pts',(-33.9340030668927,-33.4688926699519,
50.6682916621162));
#25884=CARTESIAN_POINT('Ctrl Pts',(-31.8149722356298,-34.4215239550785,
50.7794214513359));
#25885=CARTESIAN_POINT('Ctrl Pts',(-30.1913421833166,-33.3693129648789,
50.8719659908098));
#25886=CARTESIAN_POINT('Ctrl Pts',(-29.9485622615649,-32.3417633806376,
50.9274672672104));
#25887=CARTESIAN_POINT('Ctrl Pts',(-29.9485909369504,-32.000019327896,50.9459252805377));
#25888=CARTESIAN_POINT('Origin',(-32.,-32.,39.4540747194623));
#25889=CARTESIAN_POINT('',(-29.9426796073631,-31.9988395215457,49.5459252805377));
#25890=CARTESIAN_POINT('',(-29.9484130390861,-32.0006260541318,49.6040747194623));
#25891=CARTESIAN_POINT('',(-29.94525,-31.9999999999998,39.4540747194623));
#25892=CARTESIAN_POINT('Ctrl Pts',(-29.9484130390861,-32.0006260541318,
49.6040747194623));
#25893=CARTESIAN_POINT('Ctrl Pts',(-29.949455798353,-31.6189146445274,49.6246958864518));
#25894=CARTESIAN_POINT('Ctrl Pts',(-30.2348077206026,-30.5500595899322,
49.6823603165144));
#25895=CARTESIAN_POINT('Ctrl Pts',(-31.9562582889836,-29.5718115240782,
49.7770680096504));
#25896=CARTESIAN_POINT('Ctrl Pts',(-34.0162363647259,-30.6461892549403,
49.8881977988701));
#25897=CARTESIAN_POINT('Ctrl Pts',(-34.2309767846438,-32.9595598982149,
49.9993275880899));
#25898=CARTESIAN_POINT('Ctrl Pts',(-32.4039514451918,-34.3947517286369,
50.1104573773095));
#25899=CARTESIAN_POINT('Ctrl Pts',(-30.3959590882678,-33.7032818528283,
50.2120397544337));
#25900=CARTESIAN_POINT('Ctrl Pts',(-29.9502681952741,-32.5054246858934,
50.2765788684846));
#25901=CARTESIAN_POINT('Ctrl Pts',(-29.9457313039573,-31.9981314910653,
50.3040747194623));
#25902=CARTESIAN_POINT('Ctrl Pts',(-29.9426796073631,-31.9988395215457,
49.5459252805377));
#25903=CARTESIAN_POINT('Ctrl Pts',(-29.9422211904312,-31.9310296493027,
49.5496147769981));
#25904=CARTESIAN_POINT('Ctrl Pts',(-29.9760269151363,-31.1828581065124,
49.5903475365317));
#25905=CARTESIAN_POINT('Ctrl Pts',(-30.8915902884901,-29.8391109584199,
49.6681235591387));
#25906=CARTESIAN_POINT('Ctrl Pts',(-33.2141919037862,-29.8967283676685,
49.7792533483584));
#25907=CARTESIAN_POINT('Ctrl Pts',(-34.4255782561001,-31.8792371657958,
49.8903831375781));
#25908=CARTESIAN_POINT('Ctrl Pts',(-33.417101692732,-33.9722668001683,50.0015129267978));
#25909=CARTESIAN_POINT('Ctrl Pts',(-31.1117090280035,-34.2602992473698,
50.1126427160177));
#25910=CARTESIAN_POINT('Ctrl Pts',(-30.0175818073808,-32.9549395658362,
50.1941135005975));
#25911=CARTESIAN_POINT('Ctrl Pts',(-29.9432765312118,-32.1378479130034,
50.2385410221042));
#25912=CARTESIAN_POINT('Ctrl Pts',(-29.9445269623743,-32.0018139479035,
50.2459252805377));
#25913=CARTESIAN_POINT('Origin',(-32.,-32.,39.4540747194623));
#25914=CARTESIAN_POINT('',(-29.9480289757152,-31.9989253245302,48.8459252805377));
#25915=CARTESIAN_POINT('',(-29.9434378875985,-32.001535942555,48.9040747194623));
#25916=CARTESIAN_POINT('',(-29.94525,-31.9999999999998,39.4540747194623));
#25917=CARTESIAN_POINT('Ctrl Pts',(-29.9434378875985,-32.001535942555,48.9040747194623));
#25918=CARTESIAN_POINT('Ctrl Pts',(-29.9483020961478,-31.4184473527047,
48.9357696413456));
#25919=CARTESIAN_POINT('Ctrl Pts',(-30.5126875610296,-30.1456437631745,
49.0045078263023));
#25920=CARTESIAN_POINT('Ctrl Pts',(-32.6715753574031,-29.6661192937061,
49.110289274332));
#25921=CARTESIAN_POINT('Ctrl Pts',(-34.3249986728979,-31.2982922382464,
49.2214190635518));
#25922=CARTESIAN_POINT('Ctrl Pts',(-33.8506084165172,-33.5726605166398,
49.3325488527714));
#25923=CARTESIAN_POINT('Ctrl Pts',(-31.6825614063526,-34.4077469449976,
49.4436786419912));
#25924=CARTESIAN_POINT('Ctrl Pts',(-30.1534240465415,-33.2932195029209,
49.5341872642215));
#25925=CARTESIAN_POINT('Ctrl Pts',(-29.9475826160125,-32.3046098901588,
49.5876526233785));
#25926=CARTESIAN_POINT('Ctrl Pts',(-29.9484130390861,-32.0006260541318,
49.6040747194623));
#25927=CARTESIAN_POINT('Ctrl Pts',(-29.9480289757152,-31.9989253245302,
48.8459252805377));
#25928=CARTESIAN_POINT('Ctrl Pts',(-29.946733472132,-31.725775593302,48.860688531892));
#25929=CARTESIAN_POINT('Ctrl Pts',(-30.124603871078,-30.7688699552255,48.9124950463195));
#25930=CARTESIAN_POINT('Ctrl Pts',(-31.5753614937973,-29.6088296426979,
49.0013448238204));
#25931=CARTESIAN_POINT('Ctrl Pts',(-33.7785363316839,-30.346270259241,49.11247461304));
#25932=CARTESIAN_POINT('Ctrl Pts',(-34.3540140062368,-32.5971864005746,
49.2236044022598));
#25933=CARTESIAN_POINT('Ctrl Pts',(-32.7751235905007,-34.3015640243191,
49.3347341914795));
#25934=CARTESIAN_POINT('Ctrl Pts',(-30.5628189463383,-33.9129211956171,
49.4421744842388));
#25935=CARTESIAN_POINT('Ctrl Pts',(-29.9468237857144,-32.6118539740871,
49.5125715139248));
#25936=CARTESIAN_POINT('Ctrl Pts',(-29.9426796073631,-31.9988395215457,
49.5459252805377));
#25937=CARTESIAN_POINT('Origin',(-32.,-32.,39.4540747194623));
#25938=CARTESIAN_POINT('',(-29.9465981539402,-32.0017453557993,48.1459252805377));
#25939=CARTESIAN_POINT('',(-29.9436300755036,-31.998396563196,48.2040747194623));
#25940=CARTESIAN_POINT('',(-29.94525,-31.9999999999998,39.4540747194623));
#25941=CARTESIAN_POINT('Ctrl Pts',(-29.9436300755036,-31.998396563196,48.2040747194623));
#25942=CARTESIAN_POINT('Ctrl Pts',(-29.9427254333975,-31.8930410370475,
48.2098001331663));
#25943=CARTESIAN_POINT('Ctrl Pts',(-29.9979858606748,-31.1069897759954,
48.2525688099435));
#25944=CARTESIAN_POINT('Ctrl Pts',(-31.0116628453703,-29.7816217002818,
48.3323807497939));
#25945=CARTESIAN_POINT('Ctrl Pts',(-33.3276176053999,-29.9664208631788,
48.4435105390137));
#25946=CARTESIAN_POINT('Ctrl Pts',(-34.4285511303809,-32.0123295988471,
48.5546403282334));
#25947=CARTESIAN_POINT('Ctrl Pts',(-33.3069009973776,-34.0469544193595,
48.6657701174531));
#25948=CARTESIAN_POINT('Ctrl Pts',(-30.9891892443255,-34.2082287535704,
48.7768999066729));
#25949=CARTESIAN_POINT('Ctrl Pts',(-29.9937470887763,-32.8789465406671,
48.8563347740092));
#25950=CARTESIAN_POINT('Ctrl Pts',(-29.9426170795512,-32.0999288880857,
48.8987263782724));
#25951=CARTESIAN_POINT('Ctrl Pts',(-29.9434378875985,-32.001535942555,48.9040747194623));
#25952=CARTESIAN_POINT('Ctrl Pts',(-29.9465981539402,-32.0017453557993,
48.1459252805377));
#25953=CARTESIAN_POINT('Ctrl Pts',(-29.9504520097461,-31.5245465942421,
48.1717622867859));
#25954=CARTESIAN_POINT('Ctrl Pts',(-30.3537536178561,-30.3572998412992,
48.2346425561073));
#25955=CARTESIAN_POINT('Ctrl Pts',(-32.2966122923061,-29.5895986461497,
48.334566088502));
#25956=CARTESIAN_POINT('Ctrl Pts',(-34.1859029602719,-30.9417742268944,
48.4456958777216));
#25957=CARTESIAN_POINT('Ctrl Pts',(-34.0746789441273,-33.2624265592047,
48.5568256669415));
#25958=CARTESIAN_POINT('Ctrl Pts',(-32.0647312572736,-34.4277197949768,
48.6679554561611));
#25959=CARTESIAN_POINT('Ctrl Pts',(-30.2704276366367,-33.5115469150408,
48.7643219940266));
#25960=CARTESIAN_POINT('Ctrl Pts',(-29.9499840894175,-32.4111501838608,
48.8236452688188));
#25961=CARTESIAN_POINT('Ctrl Pts',(-29.9480289757152,-31.9989253245302,
48.8459252805377));
#25962=CARTESIAN_POINT('Origin',(-32.,-32.,39.4540747194623));
#25963=CARTESIAN_POINT('',(-29.9418535816666,-32.0000454490499,47.4459252805377));
#25964=CARTESIAN_POINT('',(-29.9484710272094,-31.9994832228478,47.5040747194623));
#25965=CARTESIAN_POINT('',(-29.94525,-31.9999999999998,39.4540747194623));
#25966=CARTESIAN_POINT('Ctrl Pts',(-29.9484710272094,-31.9994832228478,
47.5040747194623));
#25967=CARTESIAN_POINT('Ctrl Pts',(-29.9477709350964,-31.6884975804803,
47.5208738880602));
#25968=CARTESIAN_POINT('Ctrl Pts',(-30.1602326495066,-30.6926761132785,
47.5747163197313));
#25969=CARTESIAN_POINT('Ctrl Pts',(-31.707025094587,-29.5891540246876,47.6656020144756));
#25970=CARTESIAN_POINT('Ctrl Pts',(-33.8664812013175,-30.44621090974,47.7767318036953));
#25971=CARTESIAN_POINT('Ctrl Pts',(-34.3177539537478,-32.7252787200575,
47.887861592915));
#25972=CARTESIAN_POINT('Ctrl Pts',(-32.6478434227033,-34.3405793110984,
47.9989913821348));
#25973=CARTESIAN_POINT('Ctrl Pts',(-30.5016137197587,-33.840946436515,48.1043957576505));
#25974=CARTESIAN_POINT('Ctrl Pts',(-29.9485784419762,-32.5746882809203,
48.1727568700931));
#25975=CARTESIAN_POINT('Ctrl Pts',(-29.9436300755036,-31.998396563196,48.2040747194623));
#25976=CARTESIAN_POINT('Ctrl Pts',(-29.9418540657684,-32.0000454425719,
47.4459252805377));
#25977=CARTESIAN_POINT('Ctrl Pts',(-29.9420745751735,-31.3223792418367,
47.4828360416797));
#25978=CARTESIAN_POINT('Ctrl Pts',(-30.678213927134,-29.9642036192908,47.556790065895));
#25979=CARTESIAN_POINT('Ctrl Pts',(-32.9916833923377,-29.7831153417573,
47.6677873531836));
#25980=CARTESIAN_POINT('Ctrl Pts',(-34.4003366528858,-31.6306796899659,
47.7789171424033));
#25981=CARTESIAN_POINT('Ctrl Pts',(-33.6122278392798,-33.8162419808058,
47.890046931623));
#25982=CARTESIAN_POINT('Ctrl Pts',(-31.3486255910479,-34.3395993071363,
48.0011767208428));
#25983=CARTESIAN_POINT('Ctrl Pts',(-30.068831201512,-33.0979137910051,48.0864695038143));
#25984=CARTESIAN_POINT('Ctrl Pts',(-29.9449266252224,-32.208720259441,48.1347190237126));
#25985=CARTESIAN_POINT('Ctrl Pts',(-29.9465981539402,-32.0017453557993,
48.1459252805377));
#25986=CARTESIAN_POINT('Origin',(-32.,-32.,39.4540747194623));
#25987=CARTESIAN_POINT('',(-29.9464657329942,-31.9982258658083,46.7459252805377));
#25988=CARTESIAN_POINT('',(-29.945524346234,-32.001876932627,46.8040747194623));
#25989=CARTESIAN_POINT('',(-29.94525,-31.9999999999998,39.4540747194623));
#25990=CARTESIAN_POINT('Ctrl Pts',(-29.945524346234,-32.001876932627,46.8040747194623));
#25991=CARTESIAN_POINT('Ctrl Pts',(-29.9501840246136,-31.4877588312942,
46.831947642954));
#25992=CARTESIAN_POINT('Ctrl Pts',(-30.4058569158982,-30.2830100573331,
46.896863829519));
#25993=CARTESIAN_POINT('Ctrl Pts',(-32.4282459979597,-29.6094732845848,
46.9988232791572));
#25994=CARTESIAN_POINT('Ctrl Pts',(-34.2406047769068,-31.0631420355334,
47.109953068377));
#25995=CARTESIAN_POINT('Ctrl Pts',(-34.0023863623759,-33.3742130357603,
47.2210828575967));
#25996=CARTESIAN_POINT('Ctrl Pts',(-31.9316056639743,-34.4276191683791,
47.3322126468164));
#25997=CARTESIAN_POINT('Ctrl Pts',(-30.2269905282735,-33.4359068134596,
47.4265432674383));
#25998=CARTESIAN_POINT('Ctrl Pts',(-29.9493146838935,-32.3742412168468,
47.4838306249869));
#25999=CARTESIAN_POINT('Ctrl Pts',(-29.9484710272094,-31.9994832228478,
47.5040747194623));
#26000=CARTESIAN_POINT('Ctrl Pts',(-29.9464657329942,-31.9982258658082,
46.7459252805377));
#26001=CARTESIAN_POINT('Ctrl Pts',(-29.9447989969418,-31.7961784436538,
46.7568665335004));
#26002=CARTESIAN_POINT('Ctrl Pts',(-30.0649943949212,-30.9120086993632,
46.8048510495363));
#26003=CARTESIAN_POINT('Ctrl Pts',(-31.3319469197342,-29.6651084349508,
46.8898788286455));
#26004=CARTESIAN_POINT('Ctrl Pts',(-33.5992261839687,-30.172299490863,47.0010086178653));
#26005=CARTESIAN_POINT('Ctrl Pts',(-34.4029109875207,-32.3521822321507,
47.1121384070849));
#26006=CARTESIAN_POINT('Ctrl Pts',(-33.0074777137784,-34.2097516138314,
47.2232681963047));
#26007=CARTESIAN_POINT('Ctrl Pts',(-30.6900117620269,-34.0449802822919,
47.3343979855244));
#26008=CARTESIAN_POINT('Ctrl Pts',(-29.942958779693,-32.6850089432713,47.4086170136021));
#26009=CARTESIAN_POINT('Ctrl Pts',(-29.9418532741857,-32.0024781228395,
47.4457927786065));
#26010=CARTESIAN_POINT('Ctrl Pts',(-29.9418540657684,-32.0000454425719,
47.4459252805377));
#26011=CARTESIAN_POINT('Origin',(-32.,-32.,39.4540747194623));
#26012=CARTESIAN_POINT('',(-29.9481039192408,-32.0010072981663,46.0459252805377));
#26013=CARTESIAN_POINT('',(-29.9420942139572,-31.999362613781,46.1040747194623));
#26014=CARTESIAN_POINT('',(-29.94525,-31.9999999999998,39.4540747194623));
#26015=CARTESIAN_POINT('Ctrl Pts',(-29.9420942139572,-31.999362613781,46.1040747194623));
#26016=CARTESIAN_POINT('Ctrl Pts',(-29.9419518531651,-31.9644057826194,
46.1059781347747));
#26017=CARTESIAN_POINT('Ctrl Pts',(-29.9585993357687,-31.2492759887623,
46.1449248131603));
#26018=CARTESIAN_POINT('Ctrl Pts',(-30.7889831753562,-29.8948988474869,
46.2209147546191));
#26019=CARTESIAN_POINT('Ctrl Pts',(-33.1116689024243,-29.8407860543094,
46.3320445438389));
#26020=CARTESIAN_POINT('Ctrl Pts',(-34.4169673055408,-31.7627624485277,
46.4431743330586));
#26021=CARTESIAN_POINT('Ctrl Pts',(-33.5102834415455,-33.9018560771194,
46.5543041222783));
#26022=CARTESIAN_POINT('Ctrl Pts',(-31.2214045501895,-34.3003916487017,
46.665433911498));
#26023=CARTESIAN_POINT('Ctrl Pts',(-30.0404503222317,-33.0217127646971,
46.748690777226));
#26024=CARTESIAN_POINT('Ctrl Pts',(-29.9439912873465,-32.1710245132755,
46.7949043798808));
#26025=CARTESIAN_POINT('Ctrl Pts',(-29.945524346234,-32.001876932627,46.8040747194623));
#26026=CARTESIAN_POINT('Ctrl Pts',(-29.9481039192408,-32.0010072981663,
46.0459252805377));
#26027=CARTESIAN_POINT('Ctrl Pts',(-29.9499107511001,-31.5936483051554,
46.0679402883943));
#26028=CARTESIAN_POINT('Ctrl Pts',(-30.2646015094173,-30.498279124301,46.1269985593241));
#26029=CARTESIAN_POINT('Ctrl Pts',(-32.0474055299468,-29.5718800988582,
46.2231000933271));
#26030=CARTESIAN_POINT('Ctrl Pts',(-34.06561751162,-30.7228007852025,46.3342298825469));
#26031=CARTESIAN_POINT('Ctrl Pts',(-34.1933987473477,-33.0426003422808,
46.4453596717667));
#26032=CARTESIAN_POINT('Ctrl Pts',(-32.3138052359217,-34.4082233726336,
46.5564894609863));
#26033=CARTESIAN_POINT('Ctrl Pts',(-30.360350765969,-33.6524066858803,46.6566779972433));
#26034=CARTESIAN_POINT('Ctrl Pts',(-29.950441983378,-32.4802404827688,46.7198232704271));
#26035=CARTESIAN_POINT('Ctrl Pts',(-29.9464657329942,-31.9982258658082,
46.7459252805377));
#26036=CARTESIAN_POINT('Origin',(-32.,-32.,39.4540747194623));
#26037=CARTESIAN_POINT('',(-29.9427892107444,-32.0012284764652,45.3459252805377));
#26038=CARTESIAN_POINT('',(-29.9474011798426,-31.9985278358768,45.4040747194623));
#26039=CARTESIAN_POINT('',(-29.94525,-31.9999999999998,39.4540747194623));
#26040=CARTESIAN_POINT('Ctrl Pts',(-29.9474011798426,-31.9985278358768,
45.4040747194623));
#26041=CARTESIAN_POINT('Ctrl Pts',(-29.94581141717,-31.758608449279,45.4170518896686));
#26042=CARTESIAN_POINT('Ctrl Pts',(-30.0955923500213,-30.8357624344355,
45.4670723229481));
#26043=CARTESIAN_POINT('Ctrl Pts',(-31.4608924178518,-29.6320102139679,
45.5541360193008));
#26044=CARTESIAN_POINT('Ctrl Pts',(-33.6969732951919,-30.2626761248151,
45.6652658085205));
#26045=CARTESIAN_POINT('Ctrl Pts',(-34.3800026156816,-32.4833220057386,
45.7763955977402));
#26046=CARTESIAN_POINT('Ctrl Pts',(-32.8848793523529,-34.2616368284191,
45.88752538696));
#26047=CARTESIAN_POINT('Ctrl Pts',(-30.6194030494022,-33.9751191057943,
45.9967517608673));
#26048=CARTESIAN_POINT('Ctrl Pts',(-29.9447224036788,-32.6447171600214,
46.0689348717014));
#26049=CARTESIAN_POINT('Ctrl Pts',(-29.9420942139572,-31.999362613781,46.1040747194623));
#26050=CARTESIAN_POINT('Ctrl Pts',(-29.9427892107444,-32.0012284764652,
45.3459252805377));
#26051=CARTESIAN_POINT('Ctrl Pts',(-29.9470895307118,-31.3929993370659,
45.3790140432881));
#26052=CARTESIAN_POINT('Ctrl Pts',(-30.5546547538757,-30.0963856466631,
45.4491460691119));
#26053=CARTESIAN_POINT('Ctrl Pts',(-32.7586800166002,-29.6929633355749,
45.5563213580088));
#26054=CARTESIAN_POINT('Ctrl Pts',(-34.3496925798768,-31.3860306858952,
45.6674511472285));
#26055=CARTESIAN_POINT('Ctrl Pts',(-33.7902919754051,-33.6409960942643,
45.7785809364483));
#26056=CARTESIAN_POINT('Ctrl Pts',(-31.5924355699507,-34.3941396730243,
45.889710725668));
#26057=CARTESIAN_POINT('Ctrl Pts',(-30.1290852814386,-33.2410524482903,
45.9788255070311));
#26058=CARTESIAN_POINT('Ctrl Pts',(-29.9468705092646,-32.2790855505863,
46.030897025321));
#26059=CARTESIAN_POINT('Ctrl Pts',(-29.9481039192408,-32.0010072981663,
46.0459252805377));
#26060=CARTESIAN_POINT('Origin',(-32.,-32.,39.4540747194623));
#26061=CARTESIAN_POINT('',(-29.9443798132546,-31.9982099715446,44.6459252805377));
#26062=CARTESIAN_POINT('',(-29.9474073488643,-32.0014692601838,44.7040747194623));
#26063=CARTESIAN_POINT('',(-29.94525,-31.9999999999998,39.4540747194623));
#26064=CARTESIAN_POINT('Ctrl Pts',(-29.9474073488643,-32.0014692601838,
44.7040747194623));
#26065=CARTESIAN_POINT('Ctrl Pts',(-29.9503473165645,-31.5568170973055,
44.7281256445624));
#26066=CARTESIAN_POINT('Ctrl Pts',(-30.3107091196527,-30.4229700275786,
44.7892198327358));
#26067=CARTESIAN_POINT('Ctrl Pts',(-32.1803845633948,-29.5781259278874,
44.8873572839824));
#26068=CARTESIAN_POINT('Ctrl Pts',(-34.1324988340666,-30.8379064862986,
44.9984870732022));
#26069=CARTESIAN_POINT('Ctrl Pts',(-34.1329732977875,-33.1612224260699,
45.1096168624218));
#26070=CARTESIAN_POINT('Ctrl Pts',(-32.1813737305056,-34.4218001944348,
45.2207466516416));
#26071=CARTESIAN_POINT('Ctrl Pts',(-30.3110643538795,-33.5775893512171,
45.3188992706551));
#26072=CARTESIAN_POINT('Ctrl Pts',(-29.9503493862318,-32.4434570574783,
45.3800086265953));
#26073=CARTESIAN_POINT('Ctrl Pts',(-29.9474011798426,-31.9985278358768,
45.4040747194623));
#26074=CARTESIAN_POINT('Ctrl Pts',(-29.9443798132547,-31.9982099715446,
44.6459252805377));
#26075=CARTESIAN_POINT('Ctrl Pts',(-29.943180692852,-31.867082129172,44.6530445351088));
#26076=CARTESIAN_POINT('Ctrl Pts',(-30.014346413535,-31.0549598855982,44.6972070527531));
#26077=CARTESIAN_POINT('Ctrl Pts',(-31.0956022698719,-29.7460970996221,
44.7784128334707));
#26078=CARTESIAN_POINT('Ctrl Pts',(-33.4029916207618,-30.0176710538707,
44.8895426226904));
#26079=CARTESIAN_POINT('Ctrl Pts',(-34.4263782551407,-32.1034509621539,
45.0006724119102));
#26080=CARTESIAN_POINT('Ctrl Pts',(-33.2291698233915,-34.0945536717531,
45.1118022011298));
#26081=CARTESIAN_POINT('Ctrl Pts',(-30.907038499066,-34.1687435754524,45.2229319903497));
#26082=CARTESIAN_POINT('Ctrl Pts',(-29.9787573653101,-32.8270079213671,
45.3009730168189));
#26083=CARTESIAN_POINT('Ctrl Pts',(-29.9422752714102,-32.0739190858488,
45.3419707802149));
#26084=CARTESIAN_POINT('Ctrl Pts',(-29.9427892107444,-32.0012284764652,
45.3459252805377));
#26085=CARTESIAN_POINT('Origin',(-32.,-32.,39.4540747194623));
#26086=CARTESIAN_POINT('',(-29.9485867049726,-31.9999002048695,43.9459252805377));
#26087=CARTESIAN_POINT('',(-29.9420978900125,-32.0006422249924,44.0040747194623));
#26088=CARTESIAN_POINT('',(-29.94525,-31.9999999999998,39.4540747194623));
#26089=CARTESIAN_POINT('Ctrl Pts',(-29.9420978900125,-32.0006422249924,
44.0040747194623));
#26090=CARTESIAN_POINT('Ctrl Pts',(-29.9447425969129,-31.3555631669369,
44.0391993994563));
#26091=CARTESIAN_POINT('Ctrl Pts',(-30.6189110335615,-30.0254050294705,
44.1113673425236));
#26092=CARTESIAN_POINT('Ctrl Pts',(-32.8839555431527,-29.7380019430538,
44.2205785486641));
#26093=CARTESIAN_POINT('Ctrl Pts',(-34.3798050107393,-31.5157059542584,
44.3317083378838));
#26094=CARTESIAN_POINT('Ctrl Pts',(-33.6976827404077,-33.7366306241687,
44.4428381271036));
#26095=CARTESIAN_POINT('Ctrl Pts',(-31.4618596366578,-34.3682097798181,
44.5539679163232));
#26096=CARTESIAN_POINT('Ctrl Pts',(-30.0958300853345,-33.1648056843117,
44.6410467804429));
#26097=CARTESIAN_POINT('Ctrl Pts',(-29.9458191748613,-32.2416708805599,
44.6910823814892));
#26098=CARTESIAN_POINT('Ctrl Pts',(-29.9474073488643,-32.0014692601838,
44.7040747194623));
#26099=CARTESIAN_POINT('Ctrl Pts',(-29.9485867049726,-31.9999002048695,
43.9459252805377));
#26100=CARTESIAN_POINT('Ctrl Pts',(-29.948440755186,-31.6630643448139,43.9641182900027));
#26101=CARTESIAN_POINT('Ctrl Pts',(-30.1862445800855,-30.6405822494248,
44.0193545625409));
#26102=CARTESIAN_POINT('Ctrl Pts',(-31.7976970806331,-29.5798580480631,
44.1116340981523));
#26103=CARTESIAN_POINT('Ctrl Pts',(-33.923471884996,-30.5173437869082,44.2227638873721));
#26104=CARTESIAN_POINT('Ctrl Pts',(-34.2889060793629,-32.8117404131962,
44.3338936765918));
#26105=CARTESIAN_POINT('Ctrl Pts',(-32.5595582520656,-34.3632410163062,
44.4450234658115));
#26106=CARTESIAN_POINT('Ctrl Pts',(-30.4617016867902,-33.7910912546249,
44.5490340004601));
#26107=CARTESIAN_POINT('Ctrl Pts',(-29.9494200163777,-32.5493731067912,
44.6160012720355));
#26108=CARTESIAN_POINT('Ctrl Pts',(-29.9443798132547,-31.9982099715446,
44.6459252805377));
#26109=CARTESIAN_POINT('Origin',(-32.,-32.,39.4540747194623));
#26110=CARTESIAN_POINT('',(-29.9447460435121,-32.001842447186,43.2459252805377));
#26111=CARTESIAN_POINT('',(-29.9455159708164,-31.9981228849833,43.3040747194623));
#26112=CARTESIAN_POINT('',(-29.94525,-31.9999999999998,39.4540747194623));
#26113=CARTESIAN_POINT('Ctrl Pts',(-29.9455159708164,-31.9981228849833,
43.3040747194623));
#26114=CARTESIAN_POINT('Ctrl Pts',(-29.9439847559442,-31.8292568307923,
43.3132298912769));
#26115=CARTESIAN_POINT('Ctrl Pts',(-30.0402482322227,-30.9788546338471,
43.3594283261648));
#26116=CARTESIAN_POINT('Ctrl Pts',(-31.2204650508714,-29.6999265505474,
43.442670024126));
#26117=CARTESIAN_POINT('Ctrl Pts',(-33.5095065278182,-30.0975272261643,
43.5537998133457));
#26118=CARTESIAN_POINT('Ctrl Pts',(-34.4170640004594,-32.2362503537452,
43.6649296025654));
#26119=CARTESIAN_POINT('Ctrl Pts',(-33.1125507118291,-34.1587597191989,
43.7760593917852));
#26120=CARTESIAN_POINT('Ctrl Pts',(-30.7898430768523,-34.1055956006222,
43.8871891810049));
#26121=CARTESIAN_POINT('Ctrl Pts',(-29.9587402723266,-32.7512874624185,
43.9631942902306));
#26122=CARTESIAN_POINT('Ctrl Pts',(-29.9419534306207,-32.0358777848827,
44.0021561363831));
#26123=CARTESIAN_POINT('Ctrl Pts',(-29.9420978900125,-32.0006422249924,
44.0040747194623));
#26124=CARTESIAN_POINT('Ctrl Pts',(-29.9447460435121,-32.001842447186,43.2459252805377));
#26125=CARTESIAN_POINT('Ctrl Pts',(-29.9497235311244,-31.4625377523841,
43.2751920448965));
#26126=CARTESIAN_POINT('Ctrl Pts',(-30.4434354407804,-30.2325635251486,
43.3415020723286));
#26127=CARTESIAN_POINT('Ctrl Pts',(-32.5176476217965,-29.6272264154066,
43.444855362834));
#26128=CARTESIAN_POINT('Ctrl Pts',(-34.2741819976516,-31.1478792448328,
43.5559851520537));
#26129=CARTESIAN_POINT('Ctrl Pts',(-33.9494096698203,-33.4483837460143,
43.6671149412734));
#26130=CARTESIAN_POINT('Ctrl Pts',(-31.8405587536029,-34.4233431511784,
43.7782447304932));
#26131=CARTESIAN_POINT('Ctrl Pts',(-30.1989774834058,-33.3839529211499,
43.8711815102479));
#26132=CARTESIAN_POINT('Ctrl Pts',(-29.9487379273691,-32.3489046616982,
43.9270750269294));
#26133=CARTESIAN_POINT('Ctrl Pts',(-29.9485867049726,-31.9999002048695,
43.9459252805377));
#26134=CARTESIAN_POINT('Origin',(-32.,-32.,39.4540747194623));
#26135=CARTESIAN_POINT('',(-29.9425269848562,-31.9989451474637,42.5459252805377));
#26136=CARTESIAN_POINT('',(-29.9484731266049,-32.0005123640697,42.6040747194623));
#26137=CARTESIAN_POINT('',(-29.94525,-31.9999999999998,39.4540747194623));
#26138=CARTESIAN_POINT('Ctrl Pts',(-29.9484731266049,-32.0005123640697,
42.6040747194623));
#26139=CARTESIAN_POINT('Ctrl Pts',(-29.9493088636411,-31.6260341876009,
42.6243036461708));
#26140=CARTESIAN_POINT('Ctrl Pts',(-30.2266782234694,-30.5646578541764,
42.6815758359526));
#26141=CARTESIAN_POINT('Ctrl Pts',(-31.9306141422462,-29.57240899581,42.7758912888076));
#26142=CARTESIAN_POINT('Ctrl Pts',(-34.0018249157517,-30.6249692172527,
42.8870210780274));
#26143=CARTESIAN_POINT('Ctrl Pts',(-34.2409872374696,-32.9359427480687,
42.9981508672471));
#26144=CARTESIAN_POINT('Ctrl Pts',(-32.4292223408278,-34.3903516011817,
43.1092806564668));
#26145=CARTESIAN_POINT('Ctrl Pts',(-30.406257433528,-33.7175408329679,43.2112552738719));
#26146=CARTESIAN_POINT('Ctrl Pts',(-29.9501802918094,-32.5125154081499,
43.2761866282037));
#26147=CARTESIAN_POINT('Ctrl Pts',(-29.9455159708164,-31.9981228849833,
43.3040747194623));
#26148=CARTESIAN_POINT('Ctrl Pts',(-29.9425269848562,-31.9989451474637,
42.5459252805377));
#26149=CARTESIAN_POINT('Ctrl Pts',(-29.9421476701604,-31.9383561623691,
42.5492225367172));
#26150=CARTESIAN_POINT('Ctrl Pts',(-29.9720545404929,-31.1974555822032,
42.5895630559699));
#26151=CARTESIAN_POINT('Ctrl Pts',(-30.8688288772728,-29.8509387094972,
42.6669468382958));
#26152=CARTESIAN_POINT('Ctrl Pts',(-33.1919093046072,-29.8840212783247,
42.7780766275157));
#26153=CARTESIAN_POINT('Ctrl Pts',(-34.4241674901357,-31.8536249255854,
42.8892064167353));
#26154=CARTESIAN_POINT('Ctrl Pts',(-33.4378537625072,-33.9571893024616,
43.0003362059551));
#26155=CARTESIAN_POINT('Ctrl Pts',(-31.1356319224862,-34.2695553308866,
43.1114659951748));
#26156=CARTESIAN_POINT('Ctrl Pts',(-30.0224447317067,-32.9695959958596,
43.1933290200357));
#26157=CARTESIAN_POINT('Ctrl Pts',(-29.9434234707281,-32.145141590691,43.2381487818233));
#26158=CARTESIAN_POINT('Ctrl Pts',(-29.9447460435121,-32.001842447186,43.2459252805377));
#26159=CARTESIAN_POINT('Origin',(-32.,-32.,39.4540747194623));
#26160=CARTESIAN_POINT('',(-29.9479126462767,-31.9988339667449,41.8459252805377));
#26161=CARTESIAN_POINT('',(-29.9436380165453,-32.001608018912,41.9040747194623));
#26162=CARTESIAN_POINT('',(-29.94525,-31.9999999999998,39.4540747194623));
#26163=CARTESIAN_POINT('Ctrl Pts',(-29.9436380165453,-32.001608018912,41.9040747194623));
#26164=CARTESIAN_POINT('Ctrl Pts',(-29.9485892150319,-31.4255899166451,
41.9353774010647));
#26165=CARTESIAN_POINT('Ctrl Pts',(-30.5011706140803,-30.1595907295533,
42.0037233457405));
#26166=CARTESIAN_POINT('Ctrl Pts',(-32.646887464373,-29.6591579023516,42.1091125534892));
#26167=CARTESIAN_POINT('Ctrl Pts',(-34.3174574925706,-31.2737738657493,
42.220242342709));
#26168=CARTESIAN_POINT('Ctrl Pts',(-33.8671156889712,-33.553027035053,42.3313721319286));
#26169=CARTESIAN_POINT('Ctrl Pts',(-31.7080097873483,-34.4109652269018,
42.4425019211485));
#26170=CARTESIAN_POINT('Ctrl Pts',(-30.1605085472801,-33.3078911948606,
42.5334027836596));
#26171=CARTESIAN_POINT('Ctrl Pts',(-29.9477784598121,-32.3117795959461,
42.5872603830976));
#26172=CARTESIAN_POINT('Ctrl Pts',(-29.9484731266049,-32.0005123640697,
42.6040747194623));
#26173=CARTESIAN_POINT('Ctrl Pts',(-29.9479126462767,-31.9988339667449,
41.8459252805377));
#26174=CARTESIAN_POINT('Ctrl Pts',(-29.9465310751269,-31.7329766292276,
41.8602962916111));
#26175=CARTESIAN_POINT('Ctrl Pts',(-30.1180449363604,-30.783544371031,41.9117105657577));
#26176=CARTESIAN_POINT('Ctrl Pts',(-31.5501371962138,-29.6134580581644,
42.0001681029775));
#26177=CARTESIAN_POINT('Ctrl Pts',(-33.7609665425501,-30.3275725104634,
42.1112978921973));
#26178=CARTESIAN_POINT('Ctrl Pts',(-34.3601921411462,-32.5722924840244,
42.2224276814169));
#26179=CARTESIAN_POINT('Ctrl Pts',(-32.7993885499411,-34.2932474809962,
42.3335574706367));
#26180=CARTESIAN_POINT('Ctrl Pts',(-30.5750127249874,-33.9266611661355,
42.4413900036769));
#26181=CARTESIAN_POINT('Ctrl Pts',(-29.9464091085501,-32.6190474984427,
42.512179273644));
#26182=CARTESIAN_POINT('Ctrl Pts',(-29.9425269848562,-31.9989451474637,
42.5459252805377));
#26183=CARTESIAN_POINT('Origin',(-32.,-32.,39.4540747194623));
#26184=CARTESIAN_POINT('',(-29.9473238289665,-32.0023603893952,41.1459252805377));
#26185=CARTESIAN_POINT('',(-29.9434322372613,-31.9985074052702,41.2040747194623));
#26186=CARTESIAN_POINT('',(-29.94525,-31.9999999999998,39.4540747194623));
#26187=CARTESIAN_POINT('',(-31.4698297828114,-33.9851743256717,41.));
#26188=CARTESIAN_POINT('Ctrl Pts',(-31.4698297828114,-33.9851743256717,
41.));
#26189=CARTESIAN_POINT('Ctrl Pts',(-30.8097602092473,-33.8088929660699,
41.0370432630732));
#26190=CARTESIAN_POINT('Ctrl Pts',(-30.0750747845072,-33.1128764409483,
41.0856850232525));
#26191=CARTESIAN_POINT('Ctrl Pts',(-29.9457054770538,-32.216656490295,41.1343267834317));
#26192=CARTESIAN_POINT('Ctrl Pts',(-29.9473238289665,-32.0023603893952,
41.1459252805377));
#26193=CARTESIAN_POINT('',(-32.5313020899646,-33.98873329687,41.));
#26194=CARTESIAN_POINT('Origin',(-32.,-32.,41.));
#26195=CARTESIAN_POINT('Ctrl Pts',(-32.5313027126548,-33.9887352548077,
41.));
#26196=CARTESIAN_POINT('Ctrl Pts',(-31.886832910374,-34.1600186848657,41.0363148168372));
#26197=CARTESIAN_POINT('Ctrl Pts',(-30.5071217326733,-33.8407636746777,
41.1043397233247));
#26198=CARTESIAN_POINT('Ctrl Pts',(-29.9482863554879,-32.5817335143899,
41.1723646298121));
#26199=CARTESIAN_POINT('Ctrl Pts',(-29.9434322372613,-31.9985074052702,
41.2040747194623));
#26200=CARTESIAN_POINT('Origin',(32.,-32.,172.));
#26201=CARTESIAN_POINT('',(30.3314948688693,-31.9993848803471,166.67148036339));
#26202=CARTESIAN_POINT('',(30.3351640391491,-31.9985292345028,166.47851963661));
#26203=CARTESIAN_POINT('',(30.334,-32.,172.));
#26204=CARTESIAN_POINT('',(32.6750771856746,-33.5230977622535,166.));
#26205=CARTESIAN_POINT('Ctrl Pts',(30.3351640391491,-31.9985292345028,166.47851963661));
#26206=CARTESIAN_POINT('Ctrl Pts',(30.3338126585907,-31.8287852696714,166.467186143366));
#26207=CARTESIAN_POINT('Ctrl Pts',(30.3576887735277,-31.6594223554909,166.455852650123));
#26208=CARTESIAN_POINT('Ctrl Pts',(30.4083704460928,-31.4985231798901,166.444519156879));
#26209=CARTESIAN_POINT('Ctrl Pts',(30.5740223320084,-30.9726279098336,166.407475893806));
#26210=CARTESIAN_POINT('Ctrl Pts',(31.0260364492964,-30.5371502725322,166.370432630732));
#26211=CARTESIAN_POINT('Ctrl Pts',(31.5578489866309,-30.390951172157,166.333389367659));
#26212=CARTESIAN_POINT('Ctrl Pts',(32.0896615239654,-30.2447520717818,166.296346104586));
#26213=CARTESIAN_POINT('Ctrl Pts',(32.7012724813464,-30.3878315083329,166.259302841513));
#26214=CARTESIAN_POINT('Ctrl Pts',(33.1122475059105,-30.7555629775481,166.222259578439));
#26215=CARTESIAN_POINT('Ctrl Pts',(33.5232225304745,-31.1232944467632,166.185216315366));
#26216=CARTESIAN_POINT('Ctrl Pts',(33.7335616222216,-31.7156779486424,166.148173052293));
#26217=CARTESIAN_POINT('Ctrl Pts',(33.6481326168522,-32.2595130620954,166.11112978922));
#26218=CARTESIAN_POINT('Ctrl Pts',(33.5627036114828,-32.8033481755483,166.074086526146));
#26219=CARTESIAN_POINT('Ctrl Pts',(33.181506508997,-33.298634900575,166.037043263073));
#26220=CARTESIAN_POINT('Ctrl Pts',(32.6750771856746,-33.5230977622535,166.));
#26221=CARTESIAN_POINT('',(30.334,-32.,166.));
#26222=CARTESIAN_POINT('Origin',(32.,-32.,166.));
#26223=CARTESIAN_POINT('',(30.334,-32.,165.));
#26224=CARTESIAN_POINT('',(30.334,-32.,172.));
#26225=CARTESIAN_POINT('Origin',(32.,-32.,165.));
#26226=CARTESIAN_POINT('',(30.38531543383,-32.4224457855202,166.));
#26227=CARTESIAN_POINT('Origin',(32.,-32.,166.));
#26228=CARTESIAN_POINT('Ctrl Pts',(30.385313195272,-32.4224462418485,166.));
#26229=CARTESIAN_POINT('Ctrl Pts',(30.5228540811707,-32.9453078801577,166.036314816837));
#26230=CARTESIAN_POINT('Ctrl Pts',(30.9381273047563,-33.3962489804972,166.072629633675));
#26231=CARTESIAN_POINT('Ctrl Pts',(31.4484542466326,-33.5749075296435,166.108944450512));
#26232=CARTESIAN_POINT('Ctrl Pts',(31.9690179395742,-33.7571498266643,166.145987713585));
#26233=CARTESIAN_POINT('Ctrl Pts',(32.5884870011376,-33.6560764725003,166.183030976658));
#26234=CARTESIAN_POINT('Ctrl Pts',(33.0238560671702,-33.3177567300594,166.220074239731));
#26235=CARTESIAN_POINT('Ctrl Pts',(33.4592251332029,-32.9794369876186,166.257117502805));
#26236=CARTESIAN_POINT('Ctrl Pts',(33.7104942037048,-32.4038708569011,166.294160765878));
#26237=CARTESIAN_POINT('Ctrl Pts',(33.6624581941067,-31.8545228213468,166.331204028951));
#26238=CARTESIAN_POINT('Ctrl Pts',(33.6144221845086,-31.3051747857925,166.368247292024));
#26239=CARTESIAN_POINT('Ctrl Pts',(33.2670810948105,-30.7820448454015,166.405290555098));
#26240=CARTESIAN_POINT('Ctrl Pts',(32.7794871658154,-30.524470954864,166.442333818171));
#26241=CARTESIAN_POINT('Ctrl Pts',(32.2918932368204,-30.2668970643265,166.479377081244));
#26242=CARTESIAN_POINT('Ctrl Pts',(31.6640464685286,-30.2748792236425,166.516420344317));
#26243=CARTESIAN_POINT('Ctrl Pts',(31.1831917006873,-30.5447861876656,166.553463607391));
#26244=CARTESIAN_POINT('Ctrl Pts',(30.702336932846,-30.8146931516887,166.590506870464));
#26245=CARTESIAN_POINT('Ctrl Pts',(30.3684741654553,-31.3465249204188,166.627550133537));
#26246=CARTESIAN_POINT('Ctrl Pts',(30.3344039265837,-31.896907675664,166.66459339661));
#26247=CARTESIAN_POINT('Ctrl Pts',(30.3322925160885,-31.9310161516919,166.666889052204));
#26248=CARTESIAN_POINT('Ctrl Pts',(30.3313324779548,-31.9651958739689,166.669184707797));
#26249=CARTESIAN_POINT('Ctrl Pts',(30.3314948688693,-31.9993848803471,166.67148036339));
#26250=CARTESIAN_POINT('Origin',(32.,-32.,172.));
#26251=CARTESIAN_POINT('',(30.3358443822319,-31.9988695272148,167.37148036339));
#26252=CARTESIAN_POINT('',(30.3361975811458,-32.0008966207542,167.17851963661));
#26253=CARTESIAN_POINT('',(30.334,-32.,172.));
#26254=CARTESIAN_POINT('Ctrl Pts',(30.3361975811458,-32.0008966207542,167.17851963661));
#26255=CARTESIAN_POINT('Ctrl Pts',(30.3378409630666,-31.6647641269526,167.156112388472));
#26256=CARTESIAN_POINT('Ctrl Pts',(30.4366195132904,-31.3277436672723,167.133705140335));
#26257=CARTESIAN_POINT('Ctrl Pts',(30.6258907070991,-31.0530840229842,167.111297892197));
#26258=CARTESIAN_POINT('Ctrl Pts',(30.9387904697746,-30.5990215965532,167.074254629124));
#26259=CARTESIAN_POINT('Ctrl Pts',(31.4990076484233,-30.3153919822247,167.037211366051));
#26260=CARTESIAN_POINT('Ctrl Pts',(32.0501937676499,-30.3319767966563,167.000168102978));
#26261=CARTESIAN_POINT('Ctrl Pts',(32.6013798868764,-30.3485616110878,166.963124839904));
#26262=CARTESIAN_POINT('Ctrl Pts',(33.1435349466808,-30.6653608542793,166.926081576831));
#26263=CARTESIAN_POINT('Ctrl Pts',(33.4285638569807,-31.1374206305279,166.889038313758));
#26264=CARTESIAN_POINT('Ctrl Pts',(33.7135927672805,-31.6094804067765,166.851995050685));
#26265=CARTESIAN_POINT('Ctrl Pts',(33.7414955280759,-32.2368007160821,166.814951787611));
#26266=CARTESIAN_POINT('Ctrl Pts',(33.4995200183968,-32.7322993259295,166.777908524538));
#26267=CARTESIAN_POINT('Ctrl Pts',(33.2575445087177,-33.227797935777,166.740865261465));
#26268=CARTESIAN_POINT('Ctrl Pts',(32.7456907285641,-33.5914748461662,166.703821998392));
#26269=CARTESIAN_POINT('Ctrl Pts',(32.1981475556008,-33.6569620511966,166.666778735318));
#26270=CARTESIAN_POINT('Ctrl Pts',(31.6506043826374,-33.7224492562269,166.629735472245));
#26271=CARTESIAN_POINT('Ctrl Pts',(31.0673718168642,-33.4897467558983,166.592692209172));
#26272=CARTESIAN_POINT('Ctrl Pts',(30.7154003612491,-33.0652390543282,166.555648946099));
#26273=CARTESIAN_POINT('Ctrl Pts',(30.4711155882646,-32.7706107091773,166.529939176269));
#26274=CARTESIAN_POINT('Ctrl Pts',(30.3382296149924,-32.3835895307383,166.504229406439));
#26275=CARTESIAN_POINT('Ctrl Pts',(30.3351640391491,-31.9985292345028,166.47851963661));
#26276=CARTESIAN_POINT('Ctrl Pts',(30.3314948688693,-31.9993848803471,166.67148036339));
#26277=CARTESIAN_POINT('Ctrl Pts',(30.333952857677,-32.5168780867464,166.70622797087));
#26278=CARTESIAN_POINT('Ctrl Pts',(30.5935660073833,-33.0364983358831,166.74097557835));
#26279=CARTESIAN_POINT('Ctrl Pts',(31.0099645855531,-33.3433730549829,166.77572318583));
#26280=CARTESIAN_POINT('Ctrl Pts',(31.4538731937464,-33.6705219372966,166.812766448903));
#26281=CARTESIAN_POINT('Ctrl Pts',(32.0759681204853,-33.7558859601639,166.849809711977));
#26282=CARTESIAN_POINT('Ctrl Pts',(32.5915885496141,-33.5604004805478,166.88685297505));
#26283=CARTESIAN_POINT('Ctrl Pts',(33.107208978743,-33.3649150009316,166.923896238123));
#26284=CARTESIAN_POINT('Ctrl Pts',(33.5163549102618,-32.8885800188319,166.960939501196));
#26285=CARTESIAN_POINT('Ctrl Pts',(33.6318002169891,-32.3493650813451,166.997982764269));
#26286=CARTESIAN_POINT('Ctrl Pts',(33.7472455237165,-31.8101501438584,167.035026027343));
#26287=CARTESIAN_POINT('Ctrl Pts',(33.5689902056525,-31.2080552509844,167.072069290416));
#26288=CARTESIAN_POINT('Ctrl Pts',(33.1786044854326,-30.8185951509338,167.109112553489));
#26289=CARTESIAN_POINT('Ctrl Pts',(32.7882187652126,-30.4291350508832,167.146155816562));
#26290=CARTESIAN_POINT('Ctrl Pts',(32.1857026428369,-30.2523097436559,167.183199079636));
#26291=CARTESIAN_POINT('Ctrl Pts',(31.6467634648643,-30.3690338306598,167.220242342709));
#26292=CARTESIAN_POINT('Ctrl Pts',(31.1078242868917,-30.4857579176637,167.257285605782));
#26293=CARTESIAN_POINT('Ctrl Pts',(30.6324620533223,-30.8960313988988,167.294328868856));
#26294=CARTESIAN_POINT('Ctrl Pts',(30.438200319938,-31.4121152068147,167.331372131929));
#26295=CARTESIAN_POINT('Ctrl Pts',(30.3680886548174,-31.5983767750833,167.344741542416));
#26296=CARTESIAN_POINT('Ctrl Pts',(30.3345927167679,-31.7984210368744,167.358110952903));
#26297=CARTESIAN_POINT('Ctrl Pts',(30.3358443822319,-31.9988695272148,167.37148036339));
#26298=CARTESIAN_POINT('Origin',(32.,-32.,172.));
#26299=CARTESIAN_POINT('',(30.3355908703268,-32.0012498346338,168.07148036339));
#26300=CARTESIAN_POINT('',(30.3318493573046,-32.0009136636957,167.87851963661));
#26301=CARTESIAN_POINT('',(30.334,-32.,172.));
#26302=CARTESIAN_POINT('Ctrl Pts',(30.3318493573046,-32.0009136636957,167.87851963661));
#26303=CARTESIAN_POINT('Ctrl Pts',(30.3351439225427,-31.5020077390951,167.845038633578));
#26304=CARTESIAN_POINT('Ctrl Pts',(30.5738270707978,-31.0003673701955,167.811557630547));
#26305=CARTESIAN_POINT('Ctrl Pts',(30.9647290831503,-30.6911683371181,167.778076627516));
#26306=CARTESIAN_POINT('Ctrl Pts',(31.3972216839798,-30.3490716229446,167.741033364442));
#26307=CARTESIAN_POINT('Ctrl Pts',(32.0160473928934,-30.2425448720619,167.703990101369));
#26308=CARTESIAN_POINT('Ctrl Pts',(32.5380349752617,-30.4203340671972,167.666946838296));
#26309=CARTESIAN_POINT('Ctrl Pts',(33.0600225576301,-30.5981232623325,167.629903575223));
#26310=CARTESIAN_POINT('Ctrl Pts',(33.4851720134531,-31.0602284034857,167.592860312149));
#26311=CARTESIAN_POINT('Ctrl Pts',(33.6189371464225,-31.595192848343,167.555817049076));
#26312=CARTESIAN_POINT('Ctrl Pts',(33.7527022793919,-32.1301572932002,167.518773786003));
#26313=CARTESIAN_POINT('Ctrl Pts',(33.5950830895075,-32.7379810417613,167.48173052293));
#26314=CARTESIAN_POINT('Ctrl Pts',(33.2182054885714,-33.1405269073384,167.444687259856));
#26315=CARTESIAN_POINT('Ctrl Pts',(32.8413278876354,-33.5430727729154,167.407643996783));
#26316=CARTESIAN_POINT('Ctrl Pts',(32.2451918756475,-33.7403407555083,167.37060073371));
#26317=CARTESIAN_POINT('Ctrl Pts',(31.7025856008802,-33.6420627782017,167.333557470637));
#26318=CARTESIAN_POINT('Ctrl Pts',(31.1599793261128,-33.543784800895,167.296514207563));
#26319=CARTESIAN_POINT('Ctrl Pts',(30.6709027885658,-33.1499608636888,167.25947094449));
#26320=CARTESIAN_POINT('Ctrl Pts',(30.4591556931435,-32.6408012758188,167.222427681417));
#26321=CARTESIAN_POINT('Ctrl Pts',(30.3754931484841,-32.4396292754474,167.207791666481));
#26322=CARTESIAN_POINT('Ctrl Pts',(30.3351241533785,-32.2204523720658,167.193155651546));
#26323=CARTESIAN_POINT('Ctrl Pts',(30.3361975811458,-32.0008966207542,167.17851963661));
#26324=CARTESIAN_POINT('Ctrl Pts',(30.3358443822319,-31.9988695272148,167.37148036339));
#26325=CARTESIAN_POINT('Ctrl Pts',(30.3380607659467,-32.3538132261889,167.395154215976));
#26326=CARTESIAN_POINT('Ctrl Pts',(30.4492299054888,-32.7100244029166,167.418828068562));
#26327=CARTESIAN_POINT('Ctrl Pts',(30.6589794872193,-32.9932222989656,167.442501921148));
#26328=CARTESIAN_POINT('Ctrl Pts',(30.987181621084,-33.4363514486041,167.479545184222));
#26329=CARTESIAN_POINT('Ctrl Pts',(31.5567471220124,-33.7007156132847,167.516588447295));
#26330=CARTESIAN_POINT('Ctrl Pts',(32.1070459956353,-33.6653431492089,167.553631710368));
#26331=CARTESIAN_POINT('Ctrl Pts',(32.6573448692581,-33.6299706851331,167.590674973441));
#26332=CARTESIAN_POINT('Ctrl Pts',(33.1883771155753,-33.2948615923009,167.627718236515));
#26333=CARTESIAN_POINT('Ctrl Pts',(33.4571452136192,-32.8133599919722,167.664761499588));
#26334=CARTESIAN_POINT('Ctrl Pts',(33.7259133116631,-32.3318583916434,167.701804762661));
#26335=CARTESIAN_POINT('Ctrl Pts',(33.7324172614337,-31.7039642838181,167.738848025734));
#26336=CARTESIAN_POINT('Ctrl Pts',(33.4736809126159,-31.2169985990609,167.775891288808));
#26337=CARTESIAN_POINT('Ctrl Pts',(33.214944563798,-30.7300329143038,167.812934551881));
#26338=CARTESIAN_POINT('Ctrl Pts',(32.6909679163918,-30.3839956526149,167.849977814954));
#26339=CARTESIAN_POINT('Ctrl Pts',(32.1415198323818,-30.3372315928392,167.887021078027));
#26340=CARTESIAN_POINT('Ctrl Pts',(31.5920717483718,-30.2904675330635,167.924064341101));
#26341=CARTESIAN_POINT('Ctrl Pts',(31.0171522277581,-30.5429766752011,167.961107604174));
#26342=CARTESIAN_POINT('Ctrl Pts',(30.6798413310688,-30.9792122029183,167.998150867247));
#26343=CARTESIAN_POINT('Ctrl Pts',(30.4572652038981,-31.2670641971662,168.022594032628));
#26344=CARTESIAN_POINT('Ctrl Pts',(30.3381457763264,-31.6349121325016,168.047037198009));
#26345=CARTESIAN_POINT('Ctrl Pts',(30.3355908703268,-32.0012498346338,168.07148036339));
#26346=CARTESIAN_POINT('Origin',(32.,-32.,172.));
#26347=CARTESIAN_POINT('',(30.331348159225,-32.0004179215413,168.77148036339));
#26348=CARTESIAN_POINT('',(30.3334459265416,-31.9985209914786,168.57851963661));
#26349=CARTESIAN_POINT('',(30.334,-32.,172.));
#26350=CARTESIAN_POINT('Ctrl Pts',(30.3334459265416,-31.9985209914786,168.57851963661));
#26351=CARTESIAN_POINT('Ctrl Pts',(30.3324126580069,-31.8863119073345,168.571008141758));
#26352=CARTESIAN_POINT('Ctrl Pts',(30.3427777477924,-31.7742926336736,168.563496646906));
#26353=CARTESIAN_POINT('Ctrl Pts',(30.3652411290288,-31.6647543980759,168.555985152054));
#26354=CARTESIAN_POINT('Ctrl Pts',(30.4760202691391,-31.1245618321822,168.518941888981));
#26355=CARTESIAN_POINT('Ctrl Pts',(30.8810313161917,-30.6447084111596,168.481898625907));
#26356=CARTESIAN_POINT('Ctrl Pts',(31.3949434107614,-30.444772459129,168.444855362834));
#26357=CARTESIAN_POINT('Ctrl Pts',(31.908855505331,-30.2448365070984,168.407812099761));
#26358=CARTESIAN_POINT('Ctrl Pts',(32.5316686474178,-30.3248180240599,168.370768836687));
#26359=CARTESIAN_POINT('Ctrl Pts',(32.9783869210295,-30.6481179003979,168.333725573614));
#26360=CARTESIAN_POINT('Ctrl Pts',(33.4251051946411,-30.9714177767359,168.296682310541));
#26361=CARTESIAN_POINT('Ctrl Pts',(33.6957285997776,-31.5380360124503,168.259639047468));
#26362=CARTESIAN_POINT('Ctrl Pts',(33.6664213320894,-32.0886911775499,168.222595784395));
#26363=CARTESIAN_POINT('Ctrl Pts',(33.6371140644012,-32.6393463426495,168.185552521321));
#26364=CARTESIAN_POINT('Ctrl Pts',(33.3078761238883,-33.1740384371342,168.148509258248));
#26365=CARTESIAN_POINT('Ctrl Pts',(32.8293650100735,-33.4480952531079,168.111465995175));
#26366=CARTESIAN_POINT('Ctrl Pts',(32.3508538962588,-33.7221520690815,168.074422732102));
#26367=CARTESIAN_POINT('Ctrl Pts',(31.7230696091422,-33.7355736065441,168.037379469028));
#26368=CARTESIAN_POINT('Ctrl Pts',(31.2332828280513,-33.482218252311,168.000336205955));
#26369=CARTESIAN_POINT('Ctrl Pts',(30.7434960469603,-33.2288628980779,167.963292942882));
#26370=CARTESIAN_POINT('Ctrl Pts',(30.3917067718951,-32.7087306521491,167.926249679809));
#26371=CARTESIAN_POINT('Ctrl Pts',(30.3388918807352,-32.1598311904525,167.889206416735));
#26372=CARTESIAN_POINT('Ctrl Pts',(30.3338129443569,-32.1070463530174,167.885644156694));
#26373=CARTESIAN_POINT('Ctrl Pts',(30.3314988272416,-32.0539954855925,167.882081896652));
#26374=CARTESIAN_POINT('Ctrl Pts',(30.3318493573046,-32.0009136636957,167.87851963661));
#26375=CARTESIAN_POINT('Ctrl Pts',(30.3355908703268,-32.0012498346338,168.07148036339));
#26376=CARTESIAN_POINT('Ctrl Pts',(30.334273853292,-32.1900916136439,168.084080461082));
#26377=CARTESIAN_POINT('Ctrl Pts',(30.3639309805944,-32.3785320854588,168.096680558775));
#26378=CARTESIAN_POINT('Ctrl Pts',(30.4263577295918,-32.5554067339021,168.109280656467));
#26379=CARTESIAN_POINT('Ctrl Pts',(30.6098872975689,-33.0754038238718,168.14632391954));
#26380=CARTESIAN_POINT('Ctrl Pts',(31.076648706288,-33.4954360905143,168.183367182613));
#26381=CARTESIAN_POINT('Ctrl Pts',(31.6130544672979,-33.6232990456459,168.220410445686));
#26382=CARTESIAN_POINT('Ctrl Pts',(32.1494602283077,-33.7511620007776,168.25745370876));
#26383=CARTESIAN_POINT('Ctrl Pts',(32.7555103416085,-33.5868556443984,168.294496971833));
#26384=CARTESIAN_POINT('Ctrl Pts',(33.1538795608996,-33.205565674518,168.331540234906));
#26385=CARTESIAN_POINT('Ctrl Pts',(33.5522487801907,-32.8242757046377,168.36858349798));
#26386=CARTESIAN_POINT('Ctrl Pts',(33.7429371054722,-32.2260021212562,168.405626761053));
#26387=CARTESIAN_POINT('Ctrl Pts',(33.6386865933661,-31.6845116720053,168.442670024126));
#26388=CARTESIAN_POINT('Ctrl Pts',(33.53443608126,-31.1430212227544,168.479713287199));
#26389=CARTESIAN_POINT('Ctrl Pts',(33.1352467317664,-30.6583139076341,168.516756550272));
#26390=CARTESIAN_POINT('Ctrl Pts',(32.6237854265488,-30.4521891658866,168.553799813346));
#26391=CARTESIAN_POINT('Ctrl Pts',(32.1123241213312,-30.246064424139,168.590843076419));
#26392=CARTESIAN_POINT('Ctrl Pts',(31.4885908603897,-30.3185222557641,168.627886339492));
#26393=CARTESIAN_POINT('Ctrl Pts',(31.0380026019522,-30.6364063498675,168.664929602565));
#26394=CARTESIAN_POINT('Ctrl Pts',(30.6059805303517,-30.9411922431787,168.70044652284));
#26395=CARTESIAN_POINT('Ctrl Pts',(30.3331287789836,-31.4715958339525,168.735963443115));
#26396=CARTESIAN_POINT('Ctrl Pts',(30.331348159225,-32.0004179215413,168.77148036339));
#26397=CARTESIAN_POINT('Origin',(32.,-32.,172.));
#26398=CARTESIAN_POINT('',(30.3343646455143,-31.9984849817613,169.47148036339));
#26399=CARTESIAN_POINT('',(30.3366835507802,-32.0000156713773,169.27851963661));
#26400=CARTESIAN_POINT('',(30.334,-32.,172.));
#26401=CARTESIAN_POINT('Ctrl Pts',(30.3366835507802,-32.0000156713773,169.27851963661));
#26402=CARTESIAN_POINT('Ctrl Pts',(30.3367069615302,-31.7210138591281,169.259934386864));
#26403=CARTESIAN_POINT('Ctrl Pts',(30.4031258453532,-31.4420015723541,169.241349137118));
#26404=CARTESIAN_POINT('Ctrl Pts',(30.5358780363316,-31.1992671761327,169.222763887372));
#26405=CARTESIAN_POINT('Ctrl Pts',(30.8004735839401,-30.7154601668603,169.185720624299));
#26406=CARTESIAN_POINT('Ctrl Pts',(31.3285889721842,-30.3757729723078,169.148677361226));
#26407=CARTESIAN_POINT('Ctrl Pts',(31.8785614629847,-30.3356446108332,169.111634098152));
#26408=CARTESIAN_POINT('Ctrl Pts',(32.4285339537853,-30.2955162493585,169.074590835079));
#26409=CARTESIAN_POINT('Ctrl Pts',(33.0003635471422,-30.5549467209617,169.037547572006));
#26410=CARTESIAN_POINT('Ctrl Pts',(33.3323841217629,-30.9952220485243,169.000504308933));
#26411=CARTESIAN_POINT('Ctrl Pts',(33.6644046963836,-31.4354973760869,168.963461045859));
#26412=CARTESIAN_POINT('Ctrl Pts',(33.7566162522682,-32.0566175596089,168.926417782786));
#26413=CARTESIAN_POINT('Ctrl Pts',(33.5668232814184,-32.574361371027,168.889374519713));
#26414=CARTESIAN_POINT('Ctrl Pts',(33.3770303105685,-33.0921051824452,168.85233125664));
#26415=CARTESIAN_POINT('Ctrl Pts',(32.9052328129843,-33.5064726217596,168.815287993567));
#26416=CARTESIAN_POINT('Ctrl Pts',(32.3673227653892,-33.6278513954876,168.778244730493));
#26417=CARTESIAN_POINT('Ctrl Pts',(31.829412717794,-33.7492301692157,168.74120146742));
#26418=CARTESIAN_POINT('Ctrl Pts',(31.2253901201881,-33.5776202773574,168.704158204347));
#26419=CARTESIAN_POINT('Ctrl Pts',(30.8316524379692,-33.1915494760459,168.667114941273));
#26420=CARTESIAN_POINT('Ctrl Pts',(30.5177554157697,-32.8837646732125,168.637583173052));
#26421=CARTESIAN_POINT('Ctrl Pts',(30.3375082666587,-32.4396758788251,168.608051404831));
#26422=CARTESIAN_POINT('Ctrl Pts',(30.3334459265416,-31.9985209914786,168.57851963661));
#26423=CARTESIAN_POINT('Ctrl Pts',(30.331348159225,-32.0004179215413,168.77148036339));
#26424=CARTESIAN_POINT('Ctrl Pts',(30.331271636933,-32.0231440976491,168.773006706189));
#26425=CARTESIAN_POINT('Ctrl Pts',(30.3316957445959,-32.0458673529448,168.774533048987));
#26426=CARTESIAN_POINT('Ctrl Pts',(30.3326293636575,-32.0685696548783,168.776059391785));
#26427=CARTESIAN_POINT('Ctrl Pts',(30.3552876397336,-32.6195385092039,168.813102654858));
#26428=CARTESIAN_POINT('Ctrl Pts',(30.6780474478191,-33.1581658612735,168.850145917932));
#26429=CARTESIAN_POINT('Ctrl Pts',(31.1532156498442,-33.4379787553583,168.887189181005));
#26430=CARTESIAN_POINT('Ctrl Pts',(31.6283838518693,-33.717791649443,168.924232444078));
#26431=CARTESIAN_POINT('Ctrl Pts',(32.2559604478339,-33.7387900855429,168.961275707151));
#26432=CARTESIAN_POINT('Ctrl Pts',(32.7487697903083,-33.4913652931613,168.998318970225));
#26433=CARTESIAN_POINT('Ctrl Pts',(33.2415791327826,-33.2439405007796,169.035362233298));
#26434=CARTESIAN_POINT('Ctrl Pts',(33.5996212217667,-32.7280924799166,169.072405496371));
#26435=CARTESIAN_POINT('Ctrl Pts',(33.6590579387482,-32.1798704878478,169.109448759444));
#26436=CARTESIAN_POINT('Ctrl Pts',(33.7184946557296,-31.6316484957791,169.146492022518));
#26437=CARTESIAN_POINT('Ctrl Pts',(33.4793260007084,-31.0510525325048,169.183535285591));
#26438=CARTESIAN_POINT('Ctrl Pts',(33.050994253382,-30.7037601626695,169.220578548664));
#26439=CARTESIAN_POINT('Ctrl Pts',(32.6226625060557,-30.3564677928342,169.257621811737));
#26440=CARTESIAN_POINT('Ctrl Pts',(32.0051676664242,-30.2424790164378,169.29466507481));
#26441=CARTESIAN_POINT('Ctrl Pts',(31.4810720248777,-30.4139544794807,169.331708337884));
#26442=CARTESIAN_POINT('Ctrl Pts',(30.9569763833312,-30.5854299425236,169.368751600957));
#26443=CARTESIAN_POINT('Ctrl Pts',(30.5262799398696,-31.0423696450056,169.40579486403));
#26444=CARTESIAN_POINT('Ctrl Pts',(30.3860670516662,-31.5756804567236,169.442838127103));
#26445=CARTESIAN_POINT('Ctrl Pts',(30.3499290305059,-31.7131342788782,169.452385539199));
#26446=CARTESIAN_POINT('Ctrl Pts',(30.3330873259591,-31.8556613007967,169.461932951295));
#26447=CARTESIAN_POINT('Ctrl Pts',(30.3343646455143,-31.9984849817613,169.47148036339));
#26448=CARTESIAN_POINT('Origin',(32.,-32.,172.));
#26449=CARTESIAN_POINT('',(30.3365390411281,-32.0005076151419,170.17148036339));
#26450=CARTESIAN_POINT('',(30.333388412875,-32.0014707790079,169.97851963661));
#26451=CARTESIAN_POINT('',(30.334,-32.,172.));
#26452=CARTESIAN_POINT('Ctrl Pts',(30.333388412875,-32.0014707790079,169.97851963661));
#26453=CARTESIAN_POINT('Ctrl Pts',(30.3374606408701,-31.5584545318011,169.94886063197));
#26454=CARTESIAN_POINT('Ctrl Pts',(30.5194351289634,-31.1124834732387,169.91920162733));
#26455=CARTESIAN_POINT('Ctrl Pts',(30.8357417913499,-30.8044545164215,169.88954262269));
#26456=CARTESIAN_POINT('Ctrl Pts',(31.2307999212129,-30.4197350081262,169.852499359617));
#26457=CARTESIAN_POINT('Ctrl Pts',(31.8354069446881,-30.2501956303943,169.815456096544));
#26458=CARTESIAN_POINT('Ctrl Pts',(32.3728979661781,-30.3734166831869,169.778412833471));
#26459=CARTESIAN_POINT('Ctrl Pts',(32.9103889876682,-30.4966377359796,169.741369570397));
#26460=CARTESIAN_POINT('Ctrl Pts',(33.3807640071732,-30.9126192192969,169.704326307324));
#26461=CARTESIAN_POINT('Ctrl Pts',(33.5687819662701,-31.4310102619383,169.667283044251));
#26462=CARTESIAN_POINT('Ctrl Pts',(33.7567999253671,-31.9494013045796,169.630239781178));
#26463=CARTESIAN_POINT('Ctrl Pts',(33.6624608240559,-32.570201906545,169.593196518104));
#26464=CARTESIAN_POINT('Ctrl Pts',(33.3289337235639,-33.0093370785267,169.556153255031));
#26465=CARTESIAN_POINT('Ctrl Pts',(32.9954066230718,-33.4484722505083,169.519109991958));
#26466=CARTESIAN_POINT('Ctrl Pts',(32.4226915233989,-33.7059419925063,169.482066728885));
#26467=CARTESIAN_POINT('Ctrl Pts',(31.8728597487378,-33.6639295466528,169.445023465811));
#26468=CARTESIAN_POINT('Ctrl Pts',(31.3230279740766,-33.6219171007993,169.407980202738));
#26469=CARTESIAN_POINT('Ctrl Pts',(30.7960795244272,-33.2804224670944,169.370936939665));
#26470=CARTESIAN_POINT('Ctrl Pts',(30.5331431530888,-32.7957117382458,169.333893676592));
#26471=CARTESIAN_POINT('Ctrl Pts',(30.4021265351196,-32.5541888174575,169.315435663264));
#26472=CARTESIAN_POINT('Ctrl Pts',(30.3366603003024,-32.2771074102156,169.296977649937));
#26473=CARTESIAN_POINT('Ctrl Pts',(30.3366835507802,-32.0000156713773,169.27851963661));
#26474=CARTESIAN_POINT('Ctrl Pts',(30.3343646455143,-31.9984849817613,169.47148036339));
#26475=CARTESIAN_POINT('Ctrl Pts',(30.3380432327368,-32.4098067733181,169.498976214368));
#26476=CARTESIAN_POINT('Ctrl Pts',(30.4920006469433,-32.8235890491262,169.526472065346));
#26477=CARTESIAN_POINT('Ctrl Pts',(30.7681160103956,-33.1257390784193,169.553967916323));
#26478=CARTESIAN_POINT('Ctrl Pts',(31.1401071902734,-33.5328049674431,169.591011179396));
#26479=CARTESIAN_POINT('Ctrl Pts',(31.7338188829742,-33.7372548245368,169.62805444247));
#26480=CARTESIAN_POINT('Ctrl Pts',(32.2775718371854,-33.6455335036776,169.665097705543));
#26481=CARTESIAN_POINT('Ctrl Pts',(32.8213247913967,-33.5538121828183,169.702140968616));
#26482=CARTESIAN_POINT('Ctrl Pts',(33.3151190071186,-33.1659196840061,169.739184231689));
#26483=CARTESIAN_POINT('Ctrl Pts',(33.5329969287243,-32.6593535114379,169.776227494763));
#26484=CARTESIAN_POINT('Ctrl Pts',(33.7508748503301,-32.1527873388697,169.813270757836));
#26485=CARTESIAN_POINT('Ctrl Pts',(33.6928364778198,-31.5275474925455,169.850314020909));
#26486=CARTESIAN_POINT('Ctrl Pts',(33.3854398557542,-31.0697403359214,169.887357283982));
#26487=CARTESIAN_POINT('Ctrl Pts',(33.0780432336886,-30.6119331792972,169.924400547056));
#26488=CARTESIAN_POINT('Ctrl Pts',(32.5212883620675,-30.3215587123731,169.961443810129));
#26489=CARTESIAN_POINT('Ctrl Pts',(31.9699432512674,-30.3314907167236,169.998487073202));
#26490=CARTESIAN_POINT('Ctrl Pts',(31.4185981404672,-30.3414227210741,170.035530336275));
#26491=CARTESIAN_POINT('Ctrl Pts',(30.8726627904879,-30.6516611966991,170.072573599349));
#26492=CARTESIAN_POINT('Ctrl Pts',(30.5819542572688,-31.1202426993507,170.109616862422));
#26493=CARTESIAN_POINT('Ctrl Pts',(30.420123232909,-31.3810916800477,170.130238029411));
#26494=CARTESIAN_POINT('Ctrl Pts',(30.3373845277505,-31.6910096316149,170.150859196401));
#26495=CARTESIAN_POINT('Ctrl Pts',(30.3365390411281,-32.0005076151419,170.17148036339));
#26496=CARTESIAN_POINT('Origin',(32.,-32.,172.));
#26497=CARTESIAN_POINT('',(30.3325051052426,-32.0012453678659,170.87148036339));
#26498=CARTESIAN_POINT('',(30.3318905468311,-31.9990590648467,170.67851963661));
#26499=CARTESIAN_POINT('',(30.334,-32.,172.));
#26500=CARTESIAN_POINT('Ctrl Pts',(30.3318905468311,-31.9990590648467,170.67851963661));
#26501=CARTESIAN_POINT('Ctrl Pts',(30.3315188547892,-31.9440776971841,170.674830140149));
#26502=CARTESIAN_POINT('Ctrl Pts',(30.3340016227238,-31.889130307882,170.671140643689));
#26503=CARTESIAN_POINT('Ctrl Pts',(30.3394492489536,-31.8344784518149,170.667451147228));
#26504=CARTESIAN_POINT('Ctrl Pts',(30.3941444773462,-31.2857631722528,170.630407884155));
#26505=CARTESIAN_POINT('Ctrl Pts',(30.7477137614107,-30.7668392714703,170.593364621082));
#26506=CARTESIAN_POINT('Ctrl Pts',(31.2383657139088,-30.5151635127178,170.556321358009));
#26507=CARTESIAN_POINT('Ctrl Pts',(31.7290176664068,-30.2634877539653,170.519278094935));
#26508=CARTESIAN_POINT('Ctrl Pts',(32.3567522873385,-30.2790601372428,170.482234831862));
#26509=CARTESIAN_POINT('Ctrl Pts',(32.8343216179147,-30.5547548244002,170.445191568789));
#26510=CARTESIAN_POINT('Ctrl Pts',(33.3118909484909,-30.8304495115576,170.408148305716));
#26511=CARTESIAN_POINT('Ctrl Pts',(33.6392949887116,-31.366266502595,170.371105042643));
#26512=CARTESIAN_POINT('Ctrl Pts',(33.6667154250463,-31.9170188477602,170.334061779569));
#26513=CARTESIAN_POINT('Ctrl Pts',(33.694135861381,-32.4677711929255,170.297018516496));
#26514=CARTESIAN_POINT('Ctrl Pts',(33.4215726938297,-33.0334588922186,170.259975253423));
#26515=CARTESIAN_POINT('Ctrl Pts',(32.9737493499516,-33.355226321757,170.22293199035));
#26516=CARTESIAN_POINT('Ctrl Pts',(32.5259260060736,-33.6769937512953,170.185888727276));
#26517=CARTESIAN_POINT('Ctrl Pts',(31.9028424858688,-33.7548409110788,170.148845464203));
#26518=CARTESIAN_POINT('Ctrl Pts',(31.3896184296533,-33.5531453628992,170.11180220113));
#26519=CARTESIAN_POINT('Ctrl Pts',(30.8763943734377,-33.3514498147196,170.074758938057));
#26520=CARTESIAN_POINT('Ctrl Pts',(30.4730297812114,-32.8702115585768,170.037715674983));
#26521=CARTESIAN_POINT('Ctrl Pts',(30.3641021032237,-32.3296426110762,170.00067241191));
#26522=CARTESIAN_POINT('Ctrl Pts',(30.3423883000087,-32.2218848036297,169.993288153477));
#26523=CARTESIAN_POINT('Ctrl Pts',(30.3323745425755,-32.1117693712673,169.985903895043));
#26524=CARTESIAN_POINT('Ctrl Pts',(30.333388412875,-32.0014707790079,169.97851963661));
#26525=CARTESIAN_POINT('Ctrl Pts',(30.3365390411281,-32.0005076151419,170.17148036339));
#26526=CARTESIAN_POINT('Ctrl Pts',(30.3358657202362,-32.2469827843609,170.187902459474));
#26527=CARTESIAN_POINT('Ctrl Pts',(30.3871296120999,-32.4931916071125,170.204324555558));
#26528=CARTESIAN_POINT('Ctrl Pts',(30.4917453489521,-32.7141390229613,170.220746651642));
#26529=CARTESIAN_POINT('Ctrl Pts',(30.7277266903134,-33.2125293142421,170.257789914715));
#26530=CARTESIAN_POINT('Ctrl Pts',(31.2351710894949,-33.5823853671255,170.294833177788));
#26531=CARTESIAN_POINT('Ctrl Pts',(31.7818747409338,-33.654463057273,170.331876440861));
#26532=CARTESIAN_POINT('Ctrl Pts',(32.3285783923727,-33.7265407474205,170.368919703935));
#26533=CARTESIAN_POINT('Ctrl Pts',(32.9145412960691,-33.500840074832,170.405962967008));
#26534=CARTESIAN_POINT('Ctrl Pts',(33.271630004543,-33.0806404434732,170.443006230081));
#26535=CARTESIAN_POINT('Ctrl Pts',(33.6287187130169,-32.6604408121143,170.480049493154));
#26536=CARTESIAN_POINT('Ctrl Pts',(33.7569332262683,-32.0457422219851,170.517092756228));
#26537=CARTESIAN_POINT('Ctrl Pts',(33.5976032782476,-31.5178274148643,170.554136019301));
#26538=CARTESIAN_POINT('Ctrl Pts',(33.4382733302269,-30.9899126077435,170.591179282374));
#26539=CARTESIAN_POINT('Ctrl Pts',(32.9913989209342,-30.5487815836311,170.628222545447));
#26540=CARTESIAN_POINT('Ctrl Pts',(32.4614673569861,-30.3962935072277,170.665265808521));
#26541=CARTESIAN_POINT('Ctrl Pts',(31.9315357930381,-30.2438054308242,170.702309071594));
#26542=CARTESIAN_POINT('Ctrl Pts',(31.3185470744347,-30.3799603021296,170.739352334667));
#26543=CARTESIAN_POINT('Ctrl Pts',(30.9030015150161,-30.7424543903036,170.77639559774));
#26544=CARTESIAN_POINT('Ctrl Pts',(30.5474528146032,-31.0526112408253,170.808090519624));
#26545=CARTESIAN_POINT('Ctrl Pts',(30.3364490867416,-31.5284674046311,170.839785441507));
#26546=CARTESIAN_POINT('Ctrl Pts',(30.3325051052426,-32.0012453678659,170.87148036339));
#26547=CARTESIAN_POINT('Origin',(32.,-32.,172.));
#26548=CARTESIAN_POINT('',(30.3326609344046,-31.9986999066702,171.57148036339));
#26549=CARTESIAN_POINT('',(30.3362279033014,-31.9991286353279,171.37851963661));
#26550=CARTESIAN_POINT('',(30.334,-32.,172.));
#26551=CARTESIAN_POINT('Ctrl Pts',(30.3362279033014,-31.9991286353279,171.37851963661));
#26552=CARTESIAN_POINT('Ctrl Pts',(30.3351774875366,-31.7776543086145,171.363756385256));
#26553=CARTESIAN_POINT('Ctrl Pts',(30.3762757945419,-31.55655399107,171.348993133901));
#26554=CARTESIAN_POINT('Ctrl Pts',(30.4613605091736,-31.3539236136619,171.334229882547));
#26555=CARTESIAN_POINT('Ctrl Pts',(30.674851114459,-30.8454929030546,171.297186619474));
#26556=CARTESIAN_POINT('Ctrl Pts',(31.1652735898184,-30.4533461842114,171.2601433564));
#26557=CARTESIAN_POINT('Ctrl Pts',(31.7082132697327,-30.356927669348,171.223100093327));
#26558=CARTESIAN_POINT('Ctrl Pts',(32.2511529496469,-30.2605091544846,171.186056830254));
#26559=CARTESIAN_POINT('Ctrl Pts',(32.8466098341158,-30.4598188436011,171.149013567181));
#26560=CARTESIAN_POINT('Ctrl Pts',(33.222106081537,-30.8636537036694,171.111970304107));
#26561=CARTESIAN_POINT('Ctrl Pts',(33.5976023289583,-31.2674885637377,171.074927041034));
#26562=CARTESIAN_POINT('Ctrl Pts',(33.7531379393318,-31.8758485947579,171.037883777961));
#26563=CARTESIAN_POINT('Ctrl Pts',(33.6175406607073,-32.41035154523,171.000840514888));
#26564=CARTESIAN_POINT('Ctrl Pts',(33.4819433820829,-32.9448544957022,170.963797251814));
#26565=CARTESIAN_POINT('Ctrl Pts',(33.0552132144606,-33.4055003656264,170.926753988741));
#26566=CARTESIAN_POINT('Ctrl Pts',(32.5326195686963,-33.5815001026734,170.889710725668));
#26567=CARTESIAN_POINT('Ctrl Pts',(32.010025922932,-33.7574998397204,170.852667462595));
#26568=CARTESIAN_POINT('Ctrl Pts',(31.3915687990259,-33.6488534438904,170.815624199522));
#26569=CARTESIAN_POINT('Ctrl Pts',(30.9602508234331,-33.3052769168045,170.778580936448));
#26570=CARTESIAN_POINT('Ctrl Pts',(30.5718919721791,-32.9959204954925,170.745227169836));
#26571=CARTESIAN_POINT('Ctrl Pts',(30.3352507152854,-32.4961013373448,170.711873403223));
#26572=CARTESIAN_POINT('Ctrl Pts',(30.3318905468311,-31.9990590648467,170.67851963661));
#26573=CARTESIAN_POINT('Ctrl Pts',(30.3325051052426,-32.0012453678659,170.87148036339));
#26574=CARTESIAN_POINT('Ctrl Pts',(30.3318395803745,-32.0810240107588,170.87682870458));
#26575=CARTESIAN_POINT('Ctrl Pts',(30.3370700153316,-32.1607150028783,170.88217704577));
#26576=CARTESIAN_POINT('Ctrl Pts',(30.3484967900501,-32.2395073778593,170.88752538696));
#26577=CARTESIAN_POINT('Ctrl Pts',(30.4276400247368,-32.7852329721987,170.924568650033));
#26578=CARTESIAN_POINT('Ctrl Pts',(30.8040288943443,-33.2878508558347,170.961611913106));
#26579=CARTESIAN_POINT('Ctrl Pts',(31.3054298930238,-33.5173658105477,170.99865517618));
#26580=CARTESIAN_POINT('Ctrl Pts',(31.8068308917033,-33.7468807652606,171.035698439253));
#26581=CARTESIAN_POINT('Ctrl Pts',(32.4332440194548,-33.7032927910504,171.072741702326));
#26582=CARTESIAN_POINT('Ctrl Pts',(32.8980260256029,-33.4065475085697,171.109784965399));
#26583=CARTESIAN_POINT('Ctrl Pts',(33.3628080317511,-33.109802226089,171.146828228473));
#26584=CARTESIAN_POINT('Ctrl Pts',(33.665958916296,-32.5598996353379,171.183871491546));
#26585=CARTESIAN_POINT('Ctrl Pts',(33.668758478237,-32.0084721801214,171.220914754619));
#26586=CARTESIAN_POINT('Ctrl Pts',(33.671558040178,-31.4570447249048,171.257958017692));
#26587=CARTESIAN_POINT('Ctrl Pts',(33.3740062795152,-30.9040924052229,171.295001280766));
#26588=CARTESIAN_POINT('Ctrl Pts',(32.9122612685207,-30.6026432043029,171.332044543839));
#26589=CARTESIAN_POINT('Ctrl Pts',(32.4505162575261,-30.3011940033829,171.369087806912));
#26590=CARTESIAN_POINT('Ctrl Pts',(31.8245779961998,-30.2512479212249,171.406131069985));
#26591=CARTESIAN_POINT('Ctrl Pts',(31.3208724389158,-30.475660014203,171.443174333059));
#26592=CARTESIAN_POINT('Ctrl Pts',(30.8171668816317,-30.7000721071811,171.480217596132));
#26593=CARTESIAN_POINT('Ctrl Pts',(30.4356940283899,-31.1988423752953,171.517260859205));
#26594=CARTESIAN_POINT('Ctrl Pts',(30.3510137883834,-31.7437362483257,171.554304122278));
#26595=CARTESIAN_POINT('Ctrl Pts',(30.3379255945698,-31.8279551477702,171.560029535982));
#26596=CARTESIAN_POINT('Ctrl Pts',(30.331927435482,-31.9132758871728,171.565754949686));
#26597=CARTESIAN_POINT('Ctrl Pts',(30.3326609344046,-31.9986999066702,171.57148036339));
#26598=CARTESIAN_POINT('Origin',(32.,-32.,172.));
#26599=CARTESIAN_POINT('',(30.3365860588666,-31.9995809884575,172.27148036339));
#26600=CARTESIAN_POINT('',(30.3350677693052,-32.0014151633937,172.07851963661));
#26601=CARTESIAN_POINT('',(30.334,-32.,172.));
#26602=CARTESIAN_POINT('Ctrl Pts',(30.3350677693052,-32.0014151633937,172.07851963661));
#26603=CARTESIAN_POINT('Ctrl Pts',(30.3381925394303,-31.6144945028862,172.052682630362));
#26604=CARTESIAN_POINT('Ctrl Pts',(30.4725557471307,-31.2256167628786,172.026845624113));
#26605=CARTESIAN_POINT('Ctrl Pts',(30.7190757093515,-30.9303929967783,172.001008617865));
#26606=CARTESIAN_POINT('Ctrl Pts',(31.0725185086303,-30.5071221453465,171.963965354792));
#26607=CARTESIAN_POINT('Ctrl Pts',(31.6565083342578,-30.2763644000794,171.926922091719));
#26608=CARTESIAN_POINT('Ctrl Pts',(32.2038146085797,-30.3437132539793,171.889878828646));
#26609=CARTESIAN_POINT('Ctrl Pts',(32.7511208829017,-30.4110621078793,171.852835565572));
#26610=CARTESIAN_POINT('Ctrl Pts',(33.2617436059181,-30.7765175609463,171.815792302499));
#26611=CARTESIAN_POINT('Ctrl Pts',(33.5020245883132,-31.2728491794567,171.778749039426));
#26612=CARTESIAN_POINT('Ctrl Pts',(33.7423055707082,-31.769180797967,171.741705776352));
#26613=CARTESIAN_POINT('Ctrl Pts',(33.7122448124818,-32.3963885819206,171.704662513279));
#26614=CARTESIAN_POINT('Ctrl Pts',(33.4255979536008,-32.867465650273,171.667619250206));
#26615=CARTESIAN_POINT('Ctrl Pts',(33.1389510947197,-33.3385427186253,171.630575987133));
#26616=CARTESIAN_POINT('Ctrl Pts',(32.595718135184,-33.6534890713764,171.59353272406));
#26617=CARTESIAN_POINT('Ctrl Pts',(32.044479531719,-33.6681869652327,171.556489460986));
#26618=CARTESIAN_POINT('Ctrl Pts',(31.493240928254,-33.6828848590891,171.519446197913));
#26619=CARTESIAN_POINT('Ctrl Pts',(30.9339966808599,-33.3973342940507,171.48240293484));
#26620=CARTESIAN_POINT('Ctrl Pts',(30.6226539247684,-32.9422016603458,171.445359671767));
#26621=CARTESIAN_POINT('Ctrl Pts',(30.43539395686,-32.6684579463388,171.423079660048));
#26622=CARTESIAN_POINT('Ctrl Pts',(30.3378131418771,-32.3333673796386,171.400799648329));
#26623=CARTESIAN_POINT('Ctrl Pts',(30.3362279033014,-31.9991286353279,171.37851963661));
#26624=CARTESIAN_POINT('Ctrl Pts',(30.3326609344046,-31.9986999066702,171.57148036339));
#26625=CARTESIAN_POINT('Ctrl Pts',(30.3366731525528,-32.4659668525121,171.60279821276));
#26626=CARTESIAN_POINT('Ctrl Pts',(30.5421005326414,-32.9363239994605,171.634116062129));
#26627=CARTESIAN_POINT('Ctrl Pts',(30.8902894362117,-33.2463422889161,171.665433911498));
#26628=CARTESIAN_POINT('Ctrl Pts',(31.3021329508178,-33.6130369785294,171.702477174571));
#26629=CARTESIAN_POINT('Ctrl Pts',(31.9137076068011,-33.7554088798094,171.739520437644));
#26630=CARTESIAN_POINT('Ctrl Pts',(32.4451601577091,-33.6083093827098,171.776563700718));
#26631=CARTESIAN_POINT('Ctrl Pts',(32.9766127086172,-33.4612098856102,171.813606963791));
#26632=CARTESIAN_POINT('Ctrl Pts',(33.42794315445,-33.024638990131,171.850650226864));
#26633=CARTESIAN_POINT('Ctrl Pts',(33.592625130432,-32.4983691708365,171.887693489937));
#26634=CARTESIAN_POINT('Ctrl Pts',(33.757307106414,-31.9720993515419,171.924736753011));
#26635=CARTESIAN_POINT('Ctrl Pts',(33.6353406125451,-31.3561306084319,171.961780016084));
#26636=CARTESIAN_POINT('Ctrl Pts',(33.2825368550839,-30.9323268984023,171.998823279157));
#26637=CARTESIAN_POINT('Ctrl Pts',(32.9297330976227,-30.5085231883726,172.035866542231));
#26638=CARTESIAN_POINT('Ctrl Pts',(32.3460920765693,-30.2768845114231,172.072909805304));
#26639=CARTESIAN_POINT('Ctrl Pts',(31.798684758496,-30.3434074701176,172.109953068377));
#26640=CARTESIAN_POINT('Ctrl Pts',(31.2512774404227,-30.4099304288121,172.14699633145));
#26641=CARTESIAN_POINT('Ctrl Pts',(30.7401038253296,-30.7746150231505,172.184039594523));
#26642=CARTESIAN_POINT('Ctrl Pts',(30.4990741877597,-31.2705835601835,172.221082857597));
#26643=CARTESIAN_POINT('Ctrl Pts',(30.3897669296326,-31.4955059450278,172.237882026195));
#26644=CARTESIAN_POINT('Ctrl Pts',(30.3360184124935,-31.7474286377632,172.254681194792));
#26645=CARTESIAN_POINT('Ctrl Pts',(30.3365860588666,-31.9995809884575,172.27148036339));
#26646=CARTESIAN_POINT('Origin',(32.,-32.,172.));
#26647=CARTESIAN_POINT('',(30.3341968407374,-32.0015218483092,172.97148036339));
#26648=CARTESIAN_POINT('',(30.3312207903893,-32.00003685081,172.77851963661));
#26649=CARTESIAN_POINT('',(30.334,-32.,172.));
#26650=CARTESIAN_POINT('Ctrl Pts',(30.3312211840313,-32.0000368455905,172.77851963661));
#26651=CARTESIAN_POINT('Ctrl Pts',(30.3313999767094,-31.4505738647218,172.741608875468));
#26652=CARTESIAN_POINT('Ctrl Pts',(30.6293022634182,-30.9009447454105,172.704698114326));
#26653=CARTESIAN_POINT('Ctrl Pts',(31.0898482998377,-30.6012684094488,172.667787353184));
#26654=CARTESIAN_POINT('Ctrl Pts',(31.552047600436,-30.3005162979679,172.63074409011));
#26655=CARTESIAN_POINT('Ctrl Pts',(32.1780604609226,-30.2515147475589,172.593700827037));
#26656=CARTESIAN_POINT('Ctrl Pts',(32.6814267907523,-30.4766866019892,172.556657563964));
#26657=CARTESIAN_POINT('Ctrl Pts',(33.184793120582,-30.7018584564195,172.519614300891));
#26658=CARTESIAN_POINT('Ctrl Pts',(33.5655129197548,-31.2012037156891,172.482571037817));
#26659=CARTESIAN_POINT('Ctrl Pts',(33.6493708725363,-31.7462246967432,172.445527774744));
#26660=CARTESIAN_POINT('Ctrl Pts',(33.7332288253178,-32.2912456777972,172.408484511671));
#26661=CARTESIAN_POINT('Ctrl Pts',(33.520224931708,-32.8819423806357,172.371441248598));
#26662=CARTESIAN_POINT('Ctrl Pts',(33.1078286184573,-33.2480151969592,172.334397985524));
#26663=CARTESIAN_POINT('Ctrl Pts',(32.6954323052066,-33.6140880132827,172.297354722451));
#26664=CARTESIAN_POINT('Ctrl Pts',(32.083643572315,-33.7555369430913,172.260311459378));
#26665=CARTESIAN_POINT('Ctrl Pts',(31.5524136266673,-33.6076357230794,172.223268196305));
#26666=CARTESIAN_POINT('Ctrl Pts',(31.0211836810197,-33.4597345030675,172.186224933231));
#26667=CARTESIAN_POINT('Ctrl Pts',(30.570512522616,-33.0224831332352,172.149181670158));
#26668=CARTESIAN_POINT('Ctrl Pts',(30.4066248298793,-32.4959654695208,172.112138407085));
#26669=CARTESIAN_POINT('Ctrl Pts',(30.3570458397229,-32.3366843567626,172.10093215026));
#26670=CARTESIAN_POINT('Ctrl Pts',(30.3337124661325,-32.1692338437356,172.089725893435));
#26671=CARTESIAN_POINT('Ctrl Pts',(30.3350677693052,-32.0014151633937,172.07851963661));
#26672=CARTESIAN_POINT('Ctrl Pts',(30.3365860588666,-31.9995809884575,172.27148036339));
#26673=CARTESIAN_POINT('Ctrl Pts',(30.3372701097908,-32.303441026525,172.291724457866));
#26674=CARTESIAN_POINT('Ctrl Pts',(30.4168311309414,-32.6076345698113,172.311968552341));
#26675=CARTESIAN_POINT('Ctrl Pts',(30.573094643523,-32.8653136657775,172.332212646816));
#26676=CARTESIAN_POINT('Ctrl Pts',(30.8590303969029,-33.3368227546111,172.36925590989));
#26677=CARTESIAN_POINT('Ctrl Pts',(31.4017875637094,-33.6525884525509,172.406299172963));
#26678=CARTESIAN_POINT('Ctrl Pts',(31.9530034073899,-33.6681180883879,172.443342436036));
#26679=CARTESIAN_POINT('Ctrl Pts',(32.5042192510704,-33.6836477242249,172.480385699109));
#26680=CARTESIAN_POINT('Ctrl Pts',(33.063893771625,-33.3989412979589,172.517428962183));
#26681=CARTESIAN_POINT('Ctrl Pts',(33.3759229431567,-32.9442789264931,172.554472225256));
#26682=CARTESIAN_POINT('Ctrl Pts',(33.6879521146883,-32.4896165550273,172.591515488329));
#26683=CARTESIAN_POINT('Ctrl Pts',(33.752335937197,-31.8649982383616,172.628558751402));
#26684=CARTESIAN_POINT('Ctrl Pts',(33.5396127226094,-31.3562459313504,172.665602014476));
#26685=CARTESIAN_POINT('Ctrl Pts',(33.3268895080219,-30.8474936243392,172.702645277549));
#26686=CARTESIAN_POINT('Ctrl Pts',(32.8370592563382,-30.4546073269825,172.739688540622));
#26687=CARTESIAN_POINT('Ctrl Pts',(32.2942656347348,-30.3573696786136,172.776731803695));
#26688=CARTESIAN_POINT('Ctrl Pts',(31.7514720131314,-30.2601320302447,172.813775066769));
#26689=CARTESIAN_POINT('Ctrl Pts',(31.1557150216083,-30.4585430308634,172.850818329842));
#26690=CARTESIAN_POINT('Ctrl Pts',(30.7796098291288,-30.8618108824256,172.887861592915));
#26691=CARTESIAN_POINT('Ctrl Pts',(30.4966123179727,-31.1652467312342,172.915734516407));
#26692=CARTESIAN_POINT('Ctrl Pts',(30.3379749857601,-31.5846663086172,172.943607439899));
#26693=CARTESIAN_POINT('Ctrl Pts',(30.3341968407374,-32.0015218483092,172.97148036339));
#26694=CARTESIAN_POINT('Origin',(32.,-32.,172.));
#26695=CARTESIAN_POINT('',(30.3314156322217,-31.9994831966126,173.67148036339));
#26696=CARTESIAN_POINT('',(30.3349604002087,-31.9985615026093,173.47851963661));
#26697=CARTESIAN_POINT('',(30.334,-32.,172.));
#26698=CARTESIAN_POINT('Ctrl Pts',(30.3349604002087,-31.9985615026093,173.47851963661));
#26699=CARTESIAN_POINT('Ctrl Pts',(30.3336089830085,-31.8347381058788,173.467578383647));
#26700=CARTESIAN_POINT('Ctrl Pts',(30.3558306375885,-31.6712733228841,173.456637130684));
#26701=CARTESIAN_POINT('Ctrl Pts',(30.4031262159285,-31.515417398724,173.445695877722));
#26702=CARTESIAN_POINT('Ctrl Pts',(30.5632525338761,-30.9877436469281,173.408652614648));
#26703=CARTESIAN_POINT('Ctrl Pts',(31.0107920151616,-30.5472874446471,173.371609351575));
#26704=CARTESIAN_POINT('Ctrl Pts',(31.5409530198307,-30.3955991617705,173.334566088502));
#26705=CARTESIAN_POINT('Ctrl Pts',(32.0711140244998,-30.2439108788938,173.297522825429));
#26706=CARTESIAN_POINT('Ctrl Pts',(32.6838965525525,-30.3809905154216,173.260479562355));
#26707=CARTESIAN_POINT('Ctrl Pts',(33.0988946418266,-30.744111172962,173.223436299282));
#26708=CARTESIAN_POINT('Ctrl Pts',(33.5138927311008,-31.1072318305024,173.186393036209));
#26709=CARTESIAN_POINT('Ctrl Pts',(33.7311063815966,-31.6963935090555,173.149349773136));
#26710=CARTESIAN_POINT('Ctrl Pts',(33.651139804639,-32.2419990191115,173.112306510063));
#26711=CARTESIAN_POINT('Ctrl Pts',(33.5711732276814,-32.7876045291676,173.075263246989));
#26712=CARTESIAN_POINT('Ctrl Pts',(33.1940264232705,-33.2896538707265,173.038219983916));
#26713=CARTESIAN_POINT('Ctrl Pts',(32.6922797241113,-33.5184119873403,173.001176720843));
#26714=CARTESIAN_POINT('Ctrl Pts',(32.1905330249521,-33.747170103954,172.964133457769));
#26715=CARTESIAN_POINT('Ctrl Pts',(31.5641864310446,-33.7026369956225,172.927090194696));
#26716=CARTESIAN_POINT('Ctrl Pts',(31.0998527475379,-33.4051907712475,172.890046931623));
#26717=CARTESIAN_POINT('Ctrl Pts',(30.6355190640312,-33.1077445468725,172.85300366855));
#26718=CARTESIAN_POINT('Ctrl Pts',(30.3331982909253,-32.5573852064541,172.815960405477));
#26719=CARTESIAN_POINT('Ctrl Pts',(30.3312307747274,-32.0059541999684,172.778917142403));
#26720=CARTESIAN_POINT('Ctrl Pts',(30.3312237370187,-32.0039817583638,172.778784640472));
#26721=CARTESIAN_POINT('Ctrl Pts',(30.3312205422029,-32.0020093030476,172.778652138541));
#26722=CARTESIAN_POINT('Ctrl Pts',(30.3312211840313,-32.0000368455905,172.77851963661));
#26723=CARTESIAN_POINT('Ctrl Pts',(30.3341968407374,-32.0015218483092,172.97148036339));
#26724=CARTESIAN_POINT('Ctrl Pts',(30.3329538109971,-32.1386695305945,172.980650702972));
#26725=CARTESIAN_POINT('Ctrl Pts',(30.3484734346937,-32.2755396699326,172.989821042553));
#26726=CARTESIAN_POINT('Ctrl Pts',(30.3818418733238,-32.4079104234947,172.998991382135));
#26727=CARTESIAN_POINT('Ctrl Pts',(30.5166325034344,-32.942617410496,173.036034645208));
#26728=CARTESIAN_POINT('Ctrl Pts',(30.9426671570916,-33.4039066819931,173.073077908281));
#26729=CARTESIAN_POINT('Ctrl Pts',(31.4649946868587,-33.5806947685858,173.110121171354));
#26730=CARTESIAN_POINT('Ctrl Pts',(31.9873222166257,-33.7574828551785,173.147164434428));
#26731=CARTESIAN_POINT('Ctrl Pts',(32.6059426225026,-33.6497697568668,173.184207697501));
#26732=CARTESIAN_POINT('Ctrl Pts',(33.0377785610895,-33.3068444033881,173.221250960574));
#26733=CARTESIAN_POINT('Ctrl Pts',(33.4696144996764,-32.9639190499095,173.258294223647));
#26734=CARTESIAN_POINT('Ctrl Pts',(33.7146659709733,-32.3857814412639,173.295337486721));
#26735=CARTESIAN_POINT('Ctrl Pts',(33.660798750451,-31.8369842123471,173.332380749794));
#26736=CARTESIAN_POINT('Ctrl Pts',(33.6069315299288,-31.2881869834302,173.369424012867));
#26737=CARTESIAN_POINT('Ctrl Pts',(33.2541456175874,-30.7687301342419,173.40646727594));
#26738=CARTESIAN_POINT('Ctrl Pts',(32.7638739340123,-30.5163143023334,173.443510539014));
#26739=CARTESIAN_POINT('Ctrl Pts',(32.2736022504372,-30.2638984704248,173.480553802087));
#26740=CARTESIAN_POINT('Ctrl Pts',(31.6458447956283,-30.278523655796,173.51759706516));
#26741=CARTESIAN_POINT('Ctrl Pts',(31.1678599770333,-30.5534974529228,173.554640328233));
#26742=CARTESIAN_POINT('Ctrl Pts',(30.6898751584383,-30.8284712500496,173.591683591307));
#26743=CARTESIAN_POINT('Ctrl Pts',(30.361662976057,-31.363793658932,173.62872685438));
#26744=CARTESIAN_POINT('Ctrl Pts',(30.3334115448907,-31.9145040479303,173.665770117453));
#26745=CARTESIAN_POINT('Ctrl Pts',(30.3319598853387,-31.9428015168934,173.667673532765));
#26746=CARTESIAN_POINT('Ctrl Pts',(30.3313002037148,-31.9711396143072,173.669576948078));
#26747=CARTESIAN_POINT('Ctrl Pts',(30.3314156322217,-31.9994831966126,173.67148036339));
#26748=CARTESIAN_POINT('Origin',(32.,-32.,172.));
#26749=CARTESIAN_POINT('',(30.3357186087607,-31.9988063447514,174.37148036339));
#26750=CARTESIAN_POINT('',(30.3362886687534,-32.0008167340388,174.17851963661));
#26751=CARTESIAN_POINT('',(30.334,-32.,172.));
#26752=CARTESIAN_POINT('Ctrl Pts',(30.3362886687534,-32.0008167340388,174.17851963661));
#26753=CARTESIAN_POINT('Ctrl Pts',(30.3377536779545,-31.6705233147409,174.156504628753));
#26754=CARTESIAN_POINT('Ctrl Pts',(30.4328677375841,-31.3394522335906,174.134489620897));
#26755=CARTESIAN_POINT('Ctrl Pts',(30.6159654927621,-31.067650997486,174.11247461304));
#26756=CARTESIAN_POINT('Ctrl Pts',(30.9240525194557,-30.6103082266709,174.075431349967));
#26757=CARTESIAN_POINT('Ctrl Pts',(31.481244854197,-30.3207741949187,174.038388086894));
#26758=CARTESIAN_POINT('Ctrl Pts',(32.0325743058579,-30.3315381052262,174.00134482382));
#26759=CARTESIAN_POINT('Ctrl Pts',(32.5839037575188,-30.3423020155338,173.964301560747));
#26760=CARTESIAN_POINT('Ctrl Pts',(33.1293703260993,-30.6533638679011,173.927258297674));
#26761=CARTESIAN_POINT('Ctrl Pts',(33.4193714674863,-31.1223834453475,173.8902150346));
#26762=CARTESIAN_POINT('Ctrl Pts',(33.7093726088733,-31.591403022794,173.853171771527));
#26763=CARTESIAN_POINT('Ctrl Pts',(33.7439083230667,-32.2183803253196,173.816128508454));
#26764=CARTESIAN_POINT('Ctrl Pts',(33.5071752545138,-32.7164139389316,173.779085245381));
#26765=CARTESIAN_POINT('Ctrl Pts',(33.2704421859609,-33.2144475525435,173.742041982308));
#26766=CARTESIAN_POINT('Ctrl Pts',(32.7624403346617,-33.5835374772417,173.704998719234));
#26767=CARTESIAN_POINT('Ctrl Pts',(32.2156285932453,-33.6547901647911,173.667955456161));
#26768=CARTESIAN_POINT('Ctrl Pts',(31.668816851829,-33.7260428523404,173.630912193088));
#26769=CARTESIAN_POINT('Ctrl Pts',(31.0831952202954,-33.499458302741,173.593868930015));
#26770=CARTESIAN_POINT('Ctrl Pts',(30.7267409818334,-33.0787203772859,173.556825666941));
#26771=CARTESIAN_POINT('Ctrl Pts',(30.4755705566504,-32.7822533635026,173.530723656831));
#26772=CARTESIAN_POINT('Ctrl Pts',(30.3381844098851,-32.3893869384504,173.50462164672));
#26773=CARTESIAN_POINT('Ctrl Pts',(30.3349604002087,-31.9985615026093,173.47851963661));
#26774=CARTESIAN_POINT('Ctrl Pts',(30.3314156322217,-31.9994831966126,173.67148036339));
#26775=CARTESIAN_POINT('Ctrl Pts',(30.3335466123253,-32.5227474368098,173.706620211151));
#26776=CARTESIAN_POINT('Ctrl Pts',(30.5998552268592,-33.0478810703266,173.741760058912));
#26777=CARTESIAN_POINT('Ctrl Pts',(31.0242067934649,-33.353755611107,173.776899906673));
#26778=CARTESIAN_POINT('Ctrl Pts',(31.4715441531567,-33.6761984161711,173.813943169746));
#26779=CARTESIAN_POINT('Ctrl Pts',(32.0945095524917,-33.7549856571851,173.850986432819));
#26780=CARTESIAN_POINT('Ctrl Pts',(32.6080374026233,-33.5540647198669,173.888029695893));
#26781=CARTESIAN_POINT('Ctrl Pts',(33.121565252755,-33.3531437825487,173.925072958966));
#26782=CARTESIAN_POINT('Ctrl Pts',(33.5256555536833,-32.8725146668984,173.962116222039));
#26783=CARTESIAN_POINT('Ctrl Pts',(33.6353987747919,-32.3321106501347,173.999159485112));
#26784=CARTESIAN_POINT('Ctrl Pts',(33.7451419959006,-31.7917066333709,174.036202748186));
#26785=CARTESIAN_POINT('Ctrl Pts',(33.5605381371895,-31.1915277154938,174.073246011259));
#26786=CARTESIAN_POINT('Ctrl Pts',(33.1660609234322,-30.8062125149892,174.110289274332));
#26787=CARTESIAN_POINT('Ctrl Pts',(32.7715837096748,-30.4208973144846,174.147332537405));
#26788=CARTESIAN_POINT('Ctrl Pts',(32.1672331408712,-30.2504458313525,174.184375800479));
#26789=CARTESIAN_POINT('Ctrl Pts',(31.6295567603514,-30.3728557400395,174.221419063552));
#26790=CARTESIAN_POINT('Ctrl Pts',(31.0918803798316,-30.4952656487264,174.258462326625));
#26791=CARTESIAN_POINT('Ctrl Pts',(30.6208781875955,-30.9105369492325,174.295505589698));
#26792=CARTESIAN_POINT('Ctrl Pts',(30.4320782329074,-31.4286437461609,174.332548852772));
#26793=CARTESIAN_POINT('Ctrl Pts',(30.365936944488,-31.6101493569238,174.345526022978));
#26794=CARTESIAN_POINT('Ctrl Pts',(30.3344296026448,-31.8042757006765,174.358503193184));
#26795=CARTESIAN_POINT('Ctrl Pts',(30.3357186087607,-31.9988063447514,174.37148036339));
#26796=CARTESIAN_POINT('Origin',(32.,-32.,172.));
#26797=CARTESIAN_POINT('',(30.3357236107064,-32.0011913006864,175.07148036339));
#26798=CARTESIAN_POINT('',(30.3319794150682,-32.0009960690673,174.87851963661));
#26799=CARTESIAN_POINT('',(30.334,-32.,172.));
#26800=CARTESIAN_POINT('Ctrl Pts',(30.3319794150682,-32.0009960690673,174.87851963661));
#26801=CARTESIAN_POINT('Ctrl Pts',(30.3354661857311,-31.5078338077314,174.845430873859));
#26802=CARTESIAN_POINT('Ctrl Pts',(30.5678894861827,-31.0118158958362,174.812342111109));
#26803=CARTESIAN_POINT('Ctrl Pts',(30.9509629101096,-30.7021759118631,174.779253348358));
#26804=CARTESIAN_POINT('Ctrl Pts',(31.3798181600293,-30.3555302705375,174.742210085285));
#26805=CARTESIAN_POINT('Ctrl Pts',(31.9974842423841,-30.2424733638685,174.705166822212));
#26806=CARTESIAN_POINT('Ctrl Pts',(32.5213205070434,-30.4147394193224,174.668123559139));
#26807=CARTESIAN_POINT('Ctrl Pts',(33.0451567717027,-30.5870054747763,174.631080296065));
#26808=CARTESIAN_POINT('Ctrl Pts',(33.4751632186663,-31.0445944923531,174.594037032992));
#26809=CARTESIAN_POINT('Ctrl Pts',(33.6145712294167,-31.5781162187827,174.556993769919));
#26810=CARTESIAN_POINT('Ctrl Pts',(33.753979240167,-32.1116379452123,174.519950506846));
#26811=CARTESIAN_POINT('Ctrl Pts',(33.602788814704,-32.7210923804948,174.482907243772));
#26812=CARTESIAN_POINT('Ctrl Pts',(33.2301838719237,-33.127596479674,174.445863980699));
#26813=CARTESIAN_POINT('Ctrl Pts',(32.8575789291433,-33.5341005788531,174.408820717626));
#26814=CARTESIAN_POINT('Ctrl Pts',(32.2635594690455,-33.7376543419289,174.371777454553));
#26815=CARTESIAN_POINT('Ctrl Pts',(31.7199455756347,-33.6451126706422,174.334734191479));
#26816=CARTESIAN_POINT('Ctrl Pts',(31.1763316822239,-33.5525709993555,174.297690928406));
#26817=CARTESIAN_POINT('Ctrl Pts',(30.6831233555,-33.1639338937063,174.260647665333));
#26818=CARTESIAN_POINT('Ctrl Pts',(30.4660100514611,-32.6570395859427,174.22360440226));
#26819=CARTESIAN_POINT('Ctrl Pts',(30.377928336371,-32.4513952556937,174.208576147043));
#26820=CARTESIAN_POINT('Ctrl Pts',(30.3352885995137,-32.2262871873733,174.193547891827));
#26821=CARTESIAN_POINT('Ctrl Pts',(30.3362886687534,-32.0008167340388,174.17851963661));
#26822=CARTESIAN_POINT('Ctrl Pts',(30.3357186087607,-31.9988063447514,174.37148036339));
#26823=CARTESIAN_POINT('Ctrl Pts',(30.3381090637209,-32.359562385658,174.395546456257));
#26824=CARTESIAN_POINT('Ctrl Pts',(30.4532910934898,-32.7217088761992,174.419612549124));
#26825=CARTESIAN_POINT('Ctrl Pts',(30.669544703303,-33.0073307996953,174.443678641991));
#26826=CARTESIAN_POINT('Ctrl Pts',(31.0024088455269,-33.4469687629505,174.480721905064));
#26827=CARTESIAN_POINT('Ctrl Pts',(31.5747348471149,-33.7053023961102,174.517765168138));
#26828=CARTESIAN_POINT('Ctrl Pts',(32.1246294330488,-33.6641196293962,174.554808431211));
#26829=CARTESIAN_POINT('Ctrl Pts',(32.6745240189827,-33.6229368626822,174.591851694284));
#26830=CARTESIAN_POINT('Ctrl Pts',(33.2019871892626,-33.2822376960947,174.628894957357));
#26831=CARTESIAN_POINT('Ctrl Pts',(33.4656546572183,-32.7979242208996,174.665938220431));
#26832=CARTESIAN_POINT('Ctrl Pts',(33.7293221251739,-32.3136107457046,174.702981483504));
#26833=CARTESIAN_POINT('Ctrl Pts',(33.7291938908055,-31.6856829619021,174.740024746577));
#26834=CARTESIAN_POINT('Ctrl Pts',(33.4653286334645,-31.2014772185636,174.77706800965));
#26835=CARTESIAN_POINT('Ctrl Pts',(33.2014633761235,-30.717271475225,174.814111272724));
#26836=CARTESIAN_POINT('Ctrl Pts',(32.6738610958101,-30.3767877723504,174.851154535797));
#26837=CARTESIAN_POINT('Ctrl Pts',(32.1239497351913,-30.3358296061791,174.88819779887));
#26838=CARTESIAN_POINT('Ctrl Pts',(31.5740383745726,-30.2948714400079,174.925241061943));
#26839=CARTESIAN_POINT('Ctrl Pts',(31.0018179336486,-30.55343881054,174.962284325017));
#26840=CARTESIAN_POINT('Ctrl Pts',(30.66913338345,-30.9932126910432,174.99932758809));
#26841=CARTESIAN_POINT('Ctrl Pts',(30.4531326714452,-31.2787428464203,175.02337851319));
#26842=CARTESIAN_POINT('Ctrl Pts',(30.3381073856001,-31.6406599036176,175.04742943829));
#26843=CARTESIAN_POINT('Ctrl Pts',(30.3357236107064,-32.0011913006864,175.07148036339));
#26844=CARTESIAN_POINT('Origin',(32.,-32.,172.));
#26845=CARTESIAN_POINT('',(30.3314186128286,-32.0005207267479,175.77148036339));
#26846=CARTESIAN_POINT('',(30.3332691019313,-31.9985486152772,175.57851963661));
#26847=CARTESIAN_POINT('',(30.334,-32.,172.));
#26848=CARTESIAN_POINT('Ctrl Pts',(30.3332691019313,-31.9985486152772,175.57851963661));
#26849=CARTESIAN_POINT('Ctrl Pts',(30.3322968352458,-31.8922279885927,175.571400382039));
#26850=CARTESIAN_POINT('Ctrl Pts',(30.3415987887235,-31.7860768352642,175.564281127468));
#26851=CARTESIAN_POINT('Ctrl Pts',(30.3617914430141,-31.6820394623037,175.557161872896));
#26852=CARTESIAN_POINT('Ctrl Pts',(30.4668588763472,-31.1407069762228,175.520118609823));
#26853=CARTESIAN_POINT('Ctrl Pts',(30.8667791078583,-30.6566025847272,175.48307534675));
#26854=CARTESIAN_POINT('Ctrl Pts',(31.3785508080852,-30.4512498324188,175.446032083677));
#26855=CARTESIAN_POINT('Ctrl Pts',(31.8903225083122,-30.2458970801104,175.408988820603));
#26856=CARTESIAN_POINT('Ctrl Pts',(32.5139456772549,-30.3192959669891,175.37194555753));
#26857=CARTESIAN_POINT('Ctrl Pts',(32.964053734261,-30.6378595604081,175.334902294457));
#26858=CARTESIAN_POINT('Ctrl Pts',(33.4141617912671,-30.9564231538271,175.297859031384));
#26859=CARTESIAN_POINT('Ctrl Pts',(33.6907547363366,-31.5201514537863,175.26081576831));
#26860=CARTESIAN_POINT('Ctrl Pts',(33.6672651375685,-32.0710854469139,175.223772505237));
#26861=CARTESIAN_POINT('Ctrl Pts',(33.6437755388003,-32.6220194400415,175.186729242164));
#26862=CARTESIAN_POINT('Ctrl Pts',(33.3202033961946,-33.1601591263375,175.149685979091));
#26863=CARTESIAN_POINT('Ctrl Pts',(32.8446135677108,-33.4392547032937,175.112642716018));
#26864=CARTESIAN_POINT('Ctrl Pts',(32.369023739227,-33.7183502802499,175.075599452944));
#26865=CARTESIAN_POINT('Ctrl Pts',(31.741416224865,-33.7384017478664,175.038556189871));
#26866=CARTESIAN_POINT('Ctrl Pts',(31.2489808201369,-33.4902336632864,175.001512926798));
#26867=CARTESIAN_POINT('Ctrl Pts',(30.7565454154088,-33.2420655787064,174.964469663725));
#26868=CARTESIAN_POINT('Ctrl Pts',(30.3992821203146,-32.7256779419299,174.927426400651));
#26869=CARTESIAN_POINT('Ctrl Pts',(30.3406726815099,-32.1773669355505,174.890383137578));
#26870=CARTESIAN_POINT('Ctrl Pts',(30.3344159150848,-32.11883278192,174.886428637255));
#26871=CARTESIAN_POINT('Ctrl Pts',(30.3315627045428,-32.0599348192507,174.882474136933));
#26872=CARTESIAN_POINT('Ctrl Pts',(30.3319794150682,-32.0009960690673,174.87851963661));
#26873=CARTESIAN_POINT('Ctrl Pts',(30.3357236107064,-32.0011913006864,175.07148036339));
#26874=CARTESIAN_POINT('Ctrl Pts',(30.3344358927105,-32.1959507846202,175.084472701363));
#26875=CARTESIAN_POINT('Ctrl Pts',(30.3660189172445,-32.3903059089451,175.097465039337));
#26876=CARTESIAN_POINT('Ctrl Pts',(30.4323117265277,-32.5719966029107,175.11045737731));
#26877=CARTESIAN_POINT('Ctrl Pts',(30.6213232792773,-33.090026243801,175.147500640383));
#26878=CARTESIAN_POINT('Ctrl Pts',(31.0924950442497,-33.5051051351073,175.184543903456));
#26879=CARTESIAN_POINT('Ctrl Pts',(31.6302213766159,-33.6272954268393,175.221587166529));
#26880=CARTESIAN_POINT('Ctrl Pts',(32.1679477089822,-33.7494857185713,175.258630429603));
#26881=CARTESIAN_POINT('Ctrl Pts',(32.7722286087424,-33.5787874107291,175.295673692676));
#26882=CARTESIAN_POINT('Ctrl Pts',(33.166548412743,-33.1933111234085,175.332716955749));
#26883=CARTESIAN_POINT('Ctrl Pts',(33.5608682167436,-32.8078348360878,175.369760218822));
#26884=CARTESIAN_POINT('Ctrl Pts',(33.7452269249847,-32.2075805692888,175.406803481895));
#26885=CARTESIAN_POINT('Ctrl Pts',(33.6352629922185,-31.6672214207547,175.443846744969));
#26886=CARTESIAN_POINT('Ctrl Pts',(33.5252990594523,-31.1268622722207,175.480890008042));
#26887=CARTESIAN_POINT('Ctrl Pts',(33.1210124856788,-30.6463982419517,175.517933271115));
#26888=CARTESIAN_POINT('Ctrl Pts',(32.6074026149042,-30.4456870649923,175.554976534189));
#26889=CARTESIAN_POINT('Ctrl Pts',(32.0937927441297,-30.2449758880328,175.592019797262));
#26890=CARTESIAN_POINT('Ctrl Pts',(31.4708595763541,-30.3240175643829,175.629063060335));
#26891=CARTESIAN_POINT('Ctrl Pts',(31.0236539514369,-30.6466430515281,175.666106323408));
#26892=CARTESIAN_POINT('Ctrl Pts',(30.5996104638076,-30.9525587850175,175.701231003402));
#26893=CARTESIAN_POINT('Ctrl Pts',(30.3335629853364,-31.4774798569709,175.736355683396));
#26894=CARTESIAN_POINT('Ctrl Pts',(30.3314186128286,-32.0005207267479,175.77148036339));
#26895=CARTESIAN_POINT('Origin',(32.,-32.,172.));
#26896=CARTESIAN_POINT('',(30.3341900498104,-31.9984780038006,176.47148036339));
#26897=CARTESIAN_POINT('',(30.3366801194269,-31.9999190844631,176.27851963661));
#26898=CARTESIAN_POINT('',(30.334,-32.,172.));
#26899=CARTESIAN_POINT('Ctrl Pts',(30.3366801194269,-31.9999190844631,176.27851963661));
#26900=CARTESIAN_POINT('Ctrl Pts',(30.3365617809194,-31.7268069895527,176.260326627145));
#26901=CARTESIAN_POINT('Ctrl Pts',(30.4000687856344,-31.4537467253374,176.24213361768));
#26902=CARTESIAN_POINT('Ctrl Pts',(30.5275023444207,-31.2147759338819,176.223940608215));
#26903=CARTESIAN_POINT('Ctrl Pts',(30.7869731511369,-30.7282012464043,176.186897345142));
#26904=CARTESIAN_POINT('Ctrl Pts',(31.3114712965213,-30.3829550314745,176.149854082068));
#26905=CARTESIAN_POINT('Ctrl Pts',(31.8609892732317,-30.3370200850388,176.112810818995));
#26906=CARTESIAN_POINT('Ctrl Pts',(32.4105072499422,-30.2910851386031,176.075767555922));
#26907=CARTESIAN_POINT('Ctrl Pts',(32.9850450579787,-30.5444614606614,176.038724292849));
#26908=CARTESIAN_POINT('Ctrl Pts',(33.3216973116788,-30.9812054201089,176.001681029775));
#26909=CARTESIAN_POINT('Ctrl Pts',(33.658349565379,-31.4179493795564,175.964637766702));
#26910=CARTESIAN_POINT('Ctrl Pts',(33.7571162647429,-32.0380609763929,175.927594503629));
#26911=CARTESIAN_POINT('Ctrl Pts',(33.5728023036849,-32.5577805063248,175.890551240556));
#26912=CARTESIAN_POINT('Ctrl Pts',(33.3884883426268,-33.0775000362566,175.853507977482));
#26913=CARTESIAN_POINT('Ctrl Pts',(32.9210937211468,-33.4968274992837,175.816464714409));
#26914=CARTESIAN_POINT('Ctrl Pts',(32.3844956836908,-33.6238809220316,175.779421451336));
#26915=CARTESIAN_POINT('Ctrl Pts',(31.8478976462348,-33.7509343447796,175.742378188263));
#26916=CARTESIAN_POINT('Ctrl Pts',(31.2420961928027,-33.5857137272483,175.705334925189));
#26917=CARTESIAN_POINT('Ctrl Pts',(30.8443027836642,-33.2038231281496,175.668291662116));
#26918=CARTESIAN_POINT('Ctrl Pts',(30.5229603216459,-32.895327153815,175.638367653614));
#26919=CARTESIAN_POINT('Ctrl Pts',(30.3373557821128,-32.4454408151666,175.608443645112));
#26920=CARTESIAN_POINT('Ctrl Pts',(30.3332691019313,-31.9985486152772,175.57851963661));
#26921=CARTESIAN_POINT('Ctrl Pts',(30.3314186128286,-32.0005207267479,175.77148036339));
#26922=CARTESIAN_POINT('Ctrl Pts',(30.331301482742,-32.0290903069594,175.77339894647));
#26923=CARTESIAN_POINT('Ctrl Pts',(30.3319717264726,-32.0576542774531,175.775317529549));
#26924=CARTESIAN_POINT('Ctrl Pts',(30.3334466035821,-32.0861766407582,175.777236112628));
#26925=CARTESIAN_POINT('Ctrl Pts',(30.3619229627037,-32.6368754449028,175.814279375701));
#26926=CARTESIAN_POINT('Ctrl Pts',(30.6903537630058,-33.1720637552517,175.851322638774));
#26927=CARTESIAN_POINT('Ctrl Pts',(31.1684508511107,-33.4468423029177,175.888365901848));
#26928=CARTESIAN_POINT('Ctrl Pts',(31.6465479392156,-33.7216208505837,175.925409164921));
#26929=CARTESIAN_POINT('Ctrl Pts',(32.2743113151233,-33.7359896355667,175.962452427994));
#26930=CARTESIAN_POINT('Ctrl Pts',(32.7644798619264,-33.4833735797891,175.999495691067));
#26931=CARTESIAN_POINT('Ctrl Pts',(33.2546484087295,-33.2307575240115,176.036538954141));
#26932=CARTESIAN_POINT('Ctrl Pts',(33.6072221264279,-32.7111566274731,176.073582217214));
#26933=CARTESIAN_POINT('Ctrl Pts',(33.6608651935486,-32.1623374429729,176.110625480287));
#26934=CARTESIAN_POINT('Ctrl Pts',(33.7145082606694,-31.6135182584726,176.14766874336));
#26935=CARTESIAN_POINT('Ctrl Pts',(33.4692206772125,-31.0354807860105,176.184712006434));
#26936=CARTESIAN_POINT('Ctrl Pts',(33.0372447113627,-30.6927318387861,176.221755269507));
#26937=CARTESIAN_POINT('Ctrl Pts',(32.6052687455129,-30.3499828915616,176.25879853258));
#26938=CARTESIAN_POINT('Ctrl Pts',(31.98660439727,-30.2425224695748,176.295841795653));
#26939=CARTESIAN_POINT('Ctrl Pts',(31.4643491177993,-30.4195238790869,176.332885058727));
#26940=CARTESIAN_POINT('Ctrl Pts',(30.9420938383286,-30.5965252885991,176.3699283218));
#26941=CARTESIAN_POINT('Ctrl Pts',(30.51624762763,-31.0579885296102,176.406971584873));
#26942=CARTESIAN_POINT('Ctrl Pts',(30.3816754027113,-31.5927505255396,176.444014847946));
#26943=CARTESIAN_POINT('Ctrl Pts',(30.3484161339968,-31.7249159328636,176.453170019761));
#26944=CARTESIAN_POINT('Ctrl Pts',(30.3329485152262,-31.8615585879079,176.462325191576));
#26945=CARTESIAN_POINT('Ctrl Pts',(30.3341900498104,-31.9984780038006,176.47148036339));
#26946=CARTESIAN_POINT('Origin',(32.,-32.,172.));
#26947=CARTESIAN_POINT('',(30.3365877619741,-32.0004154259877,177.17148036339));
#26948=CARTESIAN_POINT('',(30.3335660478939,-32.0014938873844,176.97851963661));
#26949=CARTESIAN_POINT('',(30.334,-32.,172.));
#26950=CARTESIAN_POINT('Ctrl Pts',(30.3335660478939,-32.0014938873844,176.97851963661));
#26951=CARTESIAN_POINT('Ctrl Pts',(30.3376018772674,-31.5642167073913,176.949252872251));
#26952=CARTESIAN_POINT('Ctrl Pts',(30.5142836379638,-31.1240531044688,176.919986107892));
#26953=CARTESIAN_POINT('Ctrl Pts',(30.823179352105,-30.8168181284545,176.890719343533));
#26954=CARTESIAN_POINT('Ctrl Pts',(31.2141520288524,-30.4279474660799,176.85367608046));
#26955=CARTESIAN_POINT('Ctrl Pts',(31.8169346478076,-30.2520316700382,176.816632817387));
#26956=CARTESIAN_POINT('Ctrl Pts',(32.3556971519197,-30.3695688557376,176.779589554313));
#26957=CARTESIAN_POINT('Ctrl Pts',(32.8944596560319,-30.487106041437,176.74254629124));
#26958=CARTESIAN_POINT('Ctrl Pts',(33.3692020453011,-30.8980962088774,176.705503028167));
#26959=CARTESIAN_POINT('Ctrl Pts',(33.562684776124,-31.4144724854469,176.668459765094));
#26960=CARTESIAN_POINT('Ctrl Pts',(33.756167506947,-31.9308487620163,176.63141650202));
#26961=CARTESIAN_POINT('Ctrl Pts',(33.6683905793237,-32.5526111477147,176.594373238947));
#26962=CARTESIAN_POINT('Ctrl Pts',(33.3395202396086,-32.9952445464546,176.557329975874));
#26963=CARTESIAN_POINT('Ctrl Pts',(33.0106498998934,-33.4378779451946,176.520286712801));
#26964=CARTESIAN_POINT('Ctrl Pts',(32.4406861480864,-33.7013823569761,176.483243449727));
#26965=CARTESIAN_POINT('Ctrl Pts',(31.8904413064044,-33.6651795916422,176.446200186654));
#26966=CARTESIAN_POINT('Ctrl Pts',(31.3401964647224,-33.6289768263084,176.409156923581));
#26967=CARTESIAN_POINT('Ctrl Pts',(30.8096705331653,-33.2930668838592,176.372113660508));
#26968=CARTESIAN_POINT('Ctrl Pts',(30.5416293014109,-32.8111603326219,176.335070397435));
#26969=CARTESIAN_POINT('Ctrl Pts',(30.4052308101104,-32.5659319171787,176.316220143826));
#26970=CARTESIAN_POINT('Ctrl Pts',(30.336802733054,-32.2828976792056,176.297369890218));
#26971=CARTESIAN_POINT('Ctrl Pts',(30.3366801194269,-31.9999190844631,176.27851963661));
#26972=CARTESIAN_POINT('Ctrl Pts',(30.3341900498104,-31.9984780038006,176.47148036339));
#26973=CARTESIAN_POINT('Ctrl Pts',(30.3379719591493,-32.4155560491711,176.499368454649));
#26974=CARTESIAN_POINT('Ctrl Pts',(30.4967993194642,-32.8352021786124,176.527256545907));
#26975=CARTESIAN_POINT('Ctrl Pts',(30.7800748091088,-33.1386874749035,176.555144637166));
#26976=CARTESIAN_POINT('Ctrl Pts',(31.156344679564,-33.5418016774904,176.592187900239));
#26977=CARTESIAN_POINT('Ctrl Pts',(31.7521826596132,-33.7399693318165,176.629231163313));
#26978=CARTESIAN_POINT('Ctrl Pts',(32.2949365205777,-33.6425099951321,176.666274426386));
#26979=CARTESIAN_POINT('Ctrl Pts',(32.8376903815422,-33.5450506584477,176.703317689459));
#26980=CARTESIAN_POINT('Ctrl Pts',(33.3273601234219,-33.1519643307528,176.740360952532));
#26981=CARTESIAN_POINT('Ctrl Pts',(33.5398755270596,-32.6431251814289,176.777404215605));
#26982=CARTESIAN_POINT('Ctrl Pts',(33.7523909306974,-32.1342860321049,176.814447478679));
#26983=CARTESIAN_POINT('Ctrl Pts',(33.6877519960932,-31.5096940611519,176.851490741752));
#26984=CARTESIAN_POINT('Ctrl Pts',(33.3755371500396,-31.0551591733681,176.888534004825));
#26985=CARTESIAN_POINT('Ctrl Pts',(33.0633223039859,-30.6006242855842,176.925577267898));
#26986=CARTESIAN_POINT('Ctrl Pts',(32.5035315464827,-30.3161464809697,176.962620530972));
#26987=CARTESIAN_POINT('Ctrl Pts',(31.9523220911802,-30.3319012489989,176.999663794045));
#26988=CARTESIAN_POINT('Ctrl Pts',(31.4011126358776,-30.3476560170281,177.036707057118));
#26989=CARTESIAN_POINT('Ctrl Pts',(30.8584844827757,-30.6636433577011,177.073750320191));
#26990=CARTESIAN_POINT('Ctrl Pts',(30.5727413358032,-31.1352692005083,177.110793583265));
#26991=CARTESIAN_POINT('Ctrl Pts',(30.416700083008,-31.3928189900376,177.131022509973));
#26992=CARTESIAN_POINT('Ctrl Pts',(30.3372653911337,-31.6967822724175,177.151251436682));
#26993=CARTESIAN_POINT('Ctrl Pts',(30.3365877619741,-32.0004154259877,177.17148036339));
#26994=CARTESIAN_POINT('Origin',(32.,-32.,172.));
#26995=CARTESIAN_POINT('',(30.3326674689016,-32.0013033567452,177.87148036339));
#26996=CARTESIAN_POINT('',(30.3317668085256,-31.999144727569,177.67851963661));
#26997=CARTESIAN_POINT('',(30.334,-32.,172.));
#26998=CARTESIAN_POINT('Ctrl Pts',(30.3317668085256,-31.999144727569,177.67851963661));
#26999=CARTESIAN_POINT('Ctrl Pts',(30.3314592554189,-31.9500181779958,177.67522238043));
#27000=CARTESIAN_POINT('Ctrl Pts',(30.3334412619116,-31.9009167943827,177.671925124251));
#27001=CARTESIAN_POINT('Ctrl Pts',(30.3377935944025,-31.8520264236762,177.668627868071));
#27002=CARTESIAN_POINT('Ctrl Pts',(30.3866901886209,-31.3027640172314,177.631584604998));
#27003=CARTESIAN_POINT('Ctrl Pts',(30.7347589380456,-30.7801347347176,177.594541341925));
#27004=CARTESIAN_POINT('Ctrl Pts',(31.2227253353964,-30.5232907565712,177.557498078852));
#27005=CARTESIAN_POINT('Ctrl Pts',(31.7106917327472,-30.2664467784248,177.520454815778));
#27006=CARTESIAN_POINT('Ctrl Pts',(32.3385557780241,-30.2753881046458,177.483411552705));
#27007=CARTESIAN_POINT('Ctrl Pts',(32.8190103548061,-30.5460233042592,177.446368289632));
#27008=CARTESIAN_POINT('Ctrl Pts',(33.2994649315881,-30.8166585038727,177.409325026559));
#27009=CARTESIAN_POINT('Ctrl Pts',(33.6325100398753,-31.3489875768786,177.372281763485));
#27010=CARTESIAN_POINT('Ctrl Pts',(33.6657460114371,-31.8994195908216,177.335238500412));
#27011=CARTESIAN_POINT('Ctrl Pts',(33.6989819829988,-32.4498516047646,177.298195237339));
#27012=CARTESIAN_POINT('Ctrl Pts',(33.4324088178351,-33.0183865596447,177.261151974266));
#27013=CARTESIAN_POINT('Ctrl Pts',(32.9880089668758,-33.3448659600934,177.224108711192));
#27014=CARTESIAN_POINT('Ctrl Pts',(32.5436091159166,-33.6713453605421,177.187065448119));
#27015=CARTESIAN_POINT('Ctrl Pts',(31.9213825791617,-33.7557692065595,177.150022185046));
#27016=CARTESIAN_POINT('Ctrl Pts',(31.4060568380961,-33.5595055955127,177.112978921973));
#27017=CARTESIAN_POINT('Ctrl Pts',(30.8907310970306,-33.3632419844659,177.075935658899));
#27018=CARTESIAN_POINT('Ctrl Pts',(30.4823061516544,-32.8862909163551,177.038892395826));
#27019=CARTESIAN_POINT('Ctrl Pts',(30.3676750462361,-32.3469026179459,177.001849132753));
#27020=CARTESIAN_POINT('Ctrl Pts',(30.3436105181693,-32.233668737852,176.994072634039));
#27021=CARTESIAN_POINT('Ctrl Pts',(30.3324936839814,-32.1176832066525,176.986296135324));
#27022=CARTESIAN_POINT('Ctrl Pts',(30.3335660478939,-32.0014938873844,176.97851963661));
#27023=CARTESIAN_POINT('Ctrl Pts',(30.3365877619741,-32.0004154259877,177.17148036339));
#27024=CARTESIAN_POINT('Ctrl Pts',(30.3360245148585,-32.2527960910209,177.188294699755));
#27025=CARTESIAN_POINT('Ctrl Pts',(30.3898743454176,-32.5049486708014,177.20510903612));
#27026=CARTESIAN_POINT('Ctrl Pts',(30.4993722352302,-32.7300294250239,177.221923372484));
#27027=CARTESIAN_POINT('Ctrl Pts',(30.7406044224728,-33.2258994617911,177.258966635558));
#27028=CARTESIAN_POINT('Ctrl Pts',(31.2519269378011,-33.5903751903842,177.296009898631));
#27029=CARTESIAN_POINT('Ctrl Pts',(31.7993613846112,-33.6566745899168,177.333053161704));
#27030=CARTESIAN_POINT('Ctrl Pts',(32.3467958314214,-33.7229739894494,177.370096424777));
#27031=CARTESIAN_POINT('Ctrl Pts',(32.9303422097134,-33.4910970599214,177.407139687851));
#27032=CARTESIAN_POINT('Ctrl Pts',(33.2829728326695,-33.0671492310509,177.444182950924));
#27033=CARTESIAN_POINT('Ctrl Pts',(33.6356034556255,-32.6432014021804,177.481226213997));
#27034=CARTESIAN_POINT('Ctrl Pts',(33.7573183232455,-32.0271826739674,177.51826947707));
#27035=CARTESIAN_POINT('Ctrl Pts',(33.5924214296177,-31.5009802751582,177.555312740144));
#27036=CARTESIAN_POINT('Ctrl Pts',(33.4275245359899,-30.974777876349,177.592356003217));
#27037=CARTESIAN_POINT('Ctrl Pts',(32.9760158811143,-30.5383918069435,177.62939926629));
#27038=CARTESIAN_POINT('Ctrl Pts',(32.4445032601022,-30.3915091538223,177.666442529363));
#27039=CARTESIAN_POINT('Ctrl Pts',(31.9129906390901,-30.2446265007011,177.703485792437));
#27040=CARTESIAN_POINT('Ctrl Pts',(31.3014740519416,-30.3872472638642,177.74052905551));
#27041=CARTESIAN_POINT('Ctrl Pts',(30.8897804116652,-30.7541106092808,177.777572318583));
#27042=CARTESIAN_POINT('Ctrl Pts',(30.5418867902575,-31.064121270881,177.808875000185));
#27043=CARTESIAN_POINT('Ctrl Pts',(30.3366819982801,-31.5342582446545,177.840177681788));
#27044=CARTESIAN_POINT('Ctrl Pts',(30.3326674689016,-32.0013033567452,177.87148036339));
#27045=CARTESIAN_POINT('Origin',(32.,-32.,172.));
#27046=CARTESIAN_POINT('',(30.3325025779359,-31.9987820654682,178.57148036339));
#27047=CARTESIAN_POINT('',(30.3361334267378,-31.9990537049732,178.37851963661));
#27048=CARTESIAN_POINT('',(30.334,-32.,172.));
#27049=CARTESIAN_POINT('',(33.2690708798529,-30.9206413469521,179.));
#27050=CARTESIAN_POINT('Ctrl Pts',(30.3325025779359,-31.9987820654682,178.57148036339));
#27051=CARTESIAN_POINT('Ctrl Pts',(30.336429253093,-32.4716839315359,178.60319045304));
#27052=CARTESIAN_POINT('Ctrl Pts',(30.547633069383,-32.9475800416084,178.634900542691));
#27053=CARTESIAN_POINT('Ctrl Pts',(30.9034954394858,-33.2578609596282,178.666610632341));
#27054=CARTESIAN_POINT('Ctrl Pts',(31.3192086569192,-33.6203265912177,178.703653895414));
#27055=CARTESIAN_POINT('Ctrl Pts',(31.9323311937098,-33.7567842787443,178.740697158487));
#27056=CARTESIAN_POINT('Ctrl Pts',(32.4621594616056,-33.6037851887319,178.777740421561));
#27057=CARTESIAN_POINT('Ctrl Pts',(32.9919877295014,-33.4507860987195,178.814783684634));
#27058=CARTESIAN_POINT('Ctrl Pts',(33.4385217285025,-33.008330231168,178.851826947707));
#27059=CARTESIAN_POINT('Ctrl Pts',(33.5975140831873,-32.4812854179199,178.88887021078));
#27060=CARTESIAN_POINT('Ctrl Pts',(33.7565064378722,-31.9542406046717,178.925913473854));
#27061=CARTESIAN_POINT('Ctrl Pts',(33.6279571482409,-31.3426068457268,178.962956736927));
#27062=CARTESIAN_POINT('Ctrl Pts',(33.2690708798528,-30.920641346952,179.));
#27063=CARTESIAN_POINT('',(30.7285119307802,-30.9188041231383,179.));
#27064=CARTESIAN_POINT('Origin',(32.,-32.,179.));
#27065=CARTESIAN_POINT('Ctrl Pts',(30.7285101132668,-30.918802741708,179.));
#27066=CARTESIAN_POINT('Ctrl Pts',(31.0792913649319,-30.5073972709685,178.963685183163));
#27067=CARTESIAN_POINT('Ctrl Pts',(31.6490955450374,-30.2812940154422,178.927370366325));
#27068=CARTESIAN_POINT('Ctrl Pts',(32.1864012091873,-30.3417508515848,178.891055549488));
#27069=CARTESIAN_POINT('Ctrl Pts',(32.7344847960344,-30.4034204035983,178.854012286415));
#27070=CARTESIAN_POINT('Ctrl Pts',(33.2487530018731,-30.7632616842773,178.816969023342));
#27071=CARTESIAN_POINT('Ctrl Pts',(33.4942155254316,-31.2569767153464,178.779925760268));
#27072=CARTESIAN_POINT('Ctrl Pts',(33.7396780489901,-31.7506917464154,178.742882497195));
#27073=CARTESIAN_POINT('Ctrl Pts',(33.7163348902683,-32.3782805278743,178.705839234122));
#27074=CARTESIAN_POINT('Ctrl Pts',(33.4347027853158,-32.8523839466767,178.668795971049));
#27075=CARTESIAN_POINT('Ctrl Pts',(33.1530706803632,-33.326487365479,178.631752707976));
#27076=CARTESIAN_POINT('Ctrl Pts',(32.6131496291799,-33.6471054216247,178.594709444902));
#27077=CARTESIAN_POINT('Ctrl Pts',(32.0620855996171,-33.6676123863825,178.557666181829));
#27078=CARTESIAN_POINT('Ctrl Pts',(31.5110215700544,-33.6881193511403,178.520622918756));
#27079=CARTESIAN_POINT('Ctrl Pts',(30.9488145621123,-33.4085152245102,178.483579655683));
#27080=CARTESIAN_POINT('Ctrl Pts',(30.6326876565862,-32.9567024322525,178.446536392609));
#27081=CARTESIAN_POINT('Ctrl Pts',(30.4392028425771,-32.680171353914,178.423864140609));
#27082=CARTESIAN_POINT('Ctrl Pts',(30.3379002876861,-32.33913045263,178.40119188861));
#27083=CARTESIAN_POINT('Ctrl Pts',(30.3361334267378,-31.9990537049732,178.37851963661));
#27084=CARTESIAN_POINT('Origin',(32.,-32.,180.545925280538));
#27085=CARTESIAN_POINT('',(29.9466856599289,-31.9981860411733,166.254074719462));
#27086=CARTESIAN_POINT('',(29.9453305924909,-32.0018604224553,166.195925280538));
#27087=CARTESIAN_POINT('',(29.94525,-31.9999999999998,180.545925280538));
#27088=CARTESIAN_POINT('',(32.3836679988472,-29.9813874990082,166.));
#27089=CARTESIAN_POINT('Ctrl Pts',(29.9453305924909,-32.0018604224553,166.195925280538));
#27090=CARTESIAN_POINT('Ctrl Pts',(29.9505791509393,-31.480465367446,166.167660116765));
#27091=CARTESIAN_POINT('Ctrl Pts',(30.4181725087355,-30.2681453601149,166.102351689919));
#27092=CARTESIAN_POINT('Ctrl Pts',(31.7124802469756,-29.853818061345,166.037043263073));
#27093=CARTESIAN_POINT('Ctrl Pts',(32.3836679988472,-29.9813874990082,166.));
#27094=CARTESIAN_POINT('',(33.341594060514,-30.4387497693343,166.));
#27095=CARTESIAN_POINT('Origin',(32.,-32.,166.));
#27096=CARTESIAN_POINT('Ctrl Pts',(29.9466856599289,-31.9981860411733,166.254074719462));
#27097=CARTESIAN_POINT('Ctrl Pts',(29.945018943721,-31.7888334530956,166.242741226219));
#27098=CARTESIAN_POINT('Ctrl Pts',(30.070714697938,-30.8972227664145,166.194364469902));
#27099=CARTESIAN_POINT('Ctrl Pts',(31.3452942740116,-29.6692723969184,166.109672896747));
#27100=CARTESIAN_POINT('Ctrl Pts',(32.8352805361695,-30.004840379919,166.036314816837));
#27101=CARTESIAN_POINT('Ctrl Pts',(33.3415960097258,-30.4387477375165,166.));
#27102=CARTESIAN_POINT('Origin',(32.,-32.,180.545925280538));
#27103=CARTESIAN_POINT('',(29.9479603720644,-32.0011058412333,166.954074719462));
#27104=CARTESIAN_POINT('',(29.9421603132108,-31.9992413462749,166.895925280538));
#27105=CARTESIAN_POINT('',(29.94525,-31.9999999999998,180.545925280538));
#27106=CARTESIAN_POINT('Ctrl Pts',(29.9421603132107,-31.9992413462749,166.895925280538));
#27107=CARTESIAN_POINT('Ctrl Pts',(29.9419600294583,-31.9570745630481,166.893629624944));
#27108=CARTESIAN_POINT('Ctrl Pts',(29.9622503150868,-31.2346904166825,166.854290706278));
#27109=CARTESIAN_POINT('Ctrl Pts',(30.8113033217656,-29.8821785273914,166.777908524538));
#27110=CARTESIAN_POINT('Ctrl Pts',(33.1343552073857,-29.8526442983615,166.666778735318));
#27111=CARTESIAN_POINT('Ctrl Pts',(34.4195276636713,-31.7882407779865,166.555648946099));
#27112=CARTESIAN_POINT('Ctrl Pts',(33.4898245617256,-33.917852735535,166.444519156879));
#27113=CARTESIAN_POINT('Ctrl Pts',(31.1977704424326,-34.291827179356,166.333389367659));
#27114=CARTESIAN_POINT('Ctrl Pts',(30.0344359462898,-33.0073757885885,166.250524742212));
#27115=CARTESIAN_POINT('Ctrl Pts',(29.9437005871736,-32.163786162724,166.204703379838));
#27116=CARTESIAN_POINT('Ctrl Pts',(29.9453305924909,-32.0018604224553,166.195925280538));
#27117=CARTESIAN_POINT('Ctrl Pts',(29.9479603720644,-32.0011058412333,166.954074719462));
#27118=CARTESIAN_POINT('Ctrl Pts',(29.9499872262071,-31.5865390695413,166.931667471325));
#27119=CARTESIAN_POINT('Ctrl Pts',(30.2732187500398,-30.4837122260773,166.872216960114));
#27120=CARTESIAN_POINT('Ctrl Pts',(32.0730445458741,-29.572487230153,166.77572318583));
#27121=CARTESIAN_POINT('Ctrl Pts',(34.0790345383106,-30.7446539377421,166.66459339661));
#27122=CARTESIAN_POINT('Ctrl Pts',(34.1822755906712,-33.0657579093129,166.55346360739));
#27123=CARTESIAN_POINT('Ctrl Pts',(32.2884012423449,-34.4113733924264,166.442333818171));
#27124=CARTESIAN_POINT('Ctrl Pts',(30.3505031103998,-33.638176271501,166.342537522195));
#27125=CARTESIAN_POINT('Ctrl Pts',(29.9504665674704,-32.4730975920075,166.279784489292));
#27126=CARTESIAN_POINT('Ctrl Pts',(29.9466856599289,-31.9981860411733,166.254074719462));
#27127=CARTESIAN_POINT('Origin',(32.,-32.,180.545925280538));
#27128=CARTESIAN_POINT('',(29.9425975191606,-32.001126861031,167.654074719462));
#27129=CARTESIAN_POINT('',(29.9475247565372,-31.9986057389228,167.595925280538));
#27130=CARTESIAN_POINT('',(29.94525,-31.9999999999998,180.545925280538));
#27131=CARTESIAN_POINT('Ctrl Pts',(29.9475247565372,-31.9986057389228,167.595925280538));
#27132=CARTESIAN_POINT('Ctrl Pts',(29.9459810232766,-31.7513839288824,167.582555870051));
#27133=CARTESIAN_POINT('Ctrl Pts',(30.1017581212936,-30.8210527785577,167.53214319649));
#27134=CARTESIAN_POINT('Ctrl Pts',(31.4859258720994,-29.6264115520718,167.444687259857));
#27135=CARTESIAN_POINT('Ctrl Pts',(33.7152536076064,-30.2806704956948,167.333557470637));
#27136=CARTESIAN_POINT('Ctrl Pts',(34.3748036342428,-32.5084396694031,167.222427681417));
#27137=CARTESIAN_POINT('Ctrl Pts',(32.8609514083336,-34.2708933989397,167.111297892197));
#27138=CARTESIAN_POINT('Ctrl Pts',(30.6067301545083,-33.9615685895118,167.002463758571));
#27139=CARTESIAN_POINT('Ctrl Pts',(29.9451918573301,-32.6374881445034,166.930672888018));
#27140=CARTESIAN_POINT('Ctrl Pts',(29.9421603132107,-31.9992413462749,166.895925280538));
#27141=CARTESIAN_POINT('Ctrl Pts',(29.9425975191606,-32.001126861031,167.654074719462));
#27142=CARTESIAN_POINT('Ctrl Pts',(29.9466608492467,-31.3858045629682,167.620593716431));
#27143=CARTESIAN_POINT('Ctrl Pts',(30.5667381950234,-30.0825880151908,167.550069450326));
#27144=CARTESIAN_POINT('Ctrl Pts',(32.7830165101667,-29.7010703688433,167.442501921148));
#27145=CARTESIAN_POINT('Ctrl Pts',(34.3560822562997,-31.4108732598121,167.331372131929));
#27146=CARTESIAN_POINT('Ctrl Pts',(33.7728865232597,-33.6598393714977,167.220242342709));
#27147=CARTESIAN_POINT('Ctrl Pts',(31.567165387668,-34.3897368274991,167.10911255349));
#27148=CARTESIAN_POINT('Ctrl Pts',(30.1224391605011,-33.22638563952,167.020390012407));
#27149=CARTESIAN_POINT('Ctrl Pts',(29.9466364670795,-32.271893464287,166.968710734398));
#27150=CARTESIAN_POINT('Ctrl Pts',(29.9479603720644,-32.0011058412333,166.954074719462));
#27151=CARTESIAN_POINT('Origin',(32.,-32.,180.545925280538));
#27152=CARTESIAN_POINT('',(29.9445666371917,-31.9981758746936,168.354074719462));
#27153=CARTESIAN_POINT('',(29.9472120893181,-32.0015414752182,168.295925280538));
#27154=CARTESIAN_POINT('',(29.94525,-31.9999999999998,180.545925280538));
#27155=CARTESIAN_POINT('Ctrl Pts',(29.9472120893181,-32.0015414752182,168.295925280538));
#27156=CARTESIAN_POINT('Ctrl Pts',(29.9503631656104,-31.5497213110789,168.271482115157));
#27157=CARTESIAN_POINT('Ctrl Pts',(30.3199261032473,-30.4084887988219,168.209995686702));
#27158=CARTESIAN_POINT('Ctrl Pts',(32.2059575689964,-29.5801290538745,168.111465995175));
#27159=CARTESIAN_POINT('Ctrl Pts',(34.1446868899892,-30.8604773073957,168.000336205955));
#27160=CARTESIAN_POINT('Ctrl Pts',(34.1206220806415,-33.1837043507103,167.889206416735));
#27161=CARTESIAN_POINT('Ctrl Pts',(32.1557868319255,-34.4236180514851,167.778076627515));
#27162=CARTESIAN_POINT('Ctrl Pts',(30.301908163091,-33.5631391690622,167.680316248783));
#27163=CARTESIAN_POINT('Ctrl Pts',(29.9502583186249,-32.4363731851813,167.619599133124));
#27164=CARTESIAN_POINT('Ctrl Pts',(29.9475247565372,-31.9986057389228,167.595925280538));
#27165=CARTESIAN_POINT('Ctrl Pts',(29.9445666371917,-31.9981758746936,168.354074719462));
#27166=CARTESIAN_POINT('Ctrl Pts',(29.9432922623288,-31.8597835483762,168.34656322461));
#27167=CARTESIAN_POINT('Ctrl Pts',(30.0191194196309,-31.0402920378829,168.302008466685));
#27168=CARTESIAN_POINT('Ctrl Pts',(31.1194451055679,-29.7366361290419,168.220410445686));
#27169=CARTESIAN_POINT('Ctrl Pts',(33.42387242316,-30.0325701422052,168.109280656467));
#27170=CARTESIAN_POINT('Ctrl Pts',(34.4251871441161,-32.1290746196978,167.998150867247));
#27171=CARTESIAN_POINT('Ctrl Pts',(33.2069968831276,-34.107451416473,167.887021078027));
#27172=CARTESIAN_POINT('Ctrl Pts',(30.8841761797311,-34.1571115078919,167.775891288808));
#27173=CARTESIAN_POINT('Ctrl Pts',(29.9746985475988,-32.8124183152547,167.698242502619));
#27174=CARTESIAN_POINT('Ctrl Pts',(29.9421651952428,-32.0665949724013,167.657636979504));
#27175=CARTESIAN_POINT('Ctrl Pts',(29.9425975191606,-32.001126861031,167.654074719462));
#27176=CARTESIAN_POINT('Origin',(32.,-32.,180.545925280538));
#27177=CARTESIAN_POINT('',(29.9485597394751,-32.0000193281882,169.054074719462));
#27178=CARTESIAN_POINT('',(29.9419793698485,-32.0005154407483,168.995925280538));
#27179=CARTESIAN_POINT('',(29.94525,-31.9999999999998,180.545925280538));
#27180=CARTESIAN_POINT('Ctrl Pts',(29.9419793698485,-32.0005154407483,168.995925280538));
#27181=CARTESIAN_POINT('Ctrl Pts',(29.9441754853642,-31.3482962423852,168.960408360263));
#27182=CARTESIAN_POINT('Ctrl Pts',(30.6316772367222,-30.0118437704654,168.887848176914));
#27183=CARTESIAN_POINT('Ctrl Pts',(32.9078114683222,-29.7474298595245,168.778244730493));
#27184=CARTESIAN_POINT('Ctrl Pts',(34.3848240419215,-31.5408614725078,168.667114941273));
#27185=CARTESIAN_POINT('Ctrl Pts',(33.679271515441,-33.7544916864091,168.555985152054));
#27186=CARTESIAN_POINT('Ctrl Pts',(31.4368679074494,-34.3624301361752,168.444855362834));
#27187=CARTESIAN_POINT('Ctrl Pts',(30.0896998183334,-33.1501318281965,168.358168738995));
#27188=CARTESIAN_POINT('Ctrl Pts',(29.9455877551331,-32.2344482251709,168.30852537823));
#27189=CARTESIAN_POINT('Ctrl Pts',(29.9472120893181,-32.0015414752182,168.295925280538));
#27190=CARTESIAN_POINT('Ctrl Pts',(29.9485597394751,-32.0000193281882,169.054074719462));
#27191=CARTESIAN_POINT('Ctrl Pts',(29.9485886129679,-31.6559143019464,169.035489469716));
#27192=CARTESIAN_POINT('Ctrl Pts',(30.1937796627957,-30.6259163319228,168.979860956897));
#27193=CARTESIAN_POINT('Ctrl Pts',(31.8232672776651,-29.5778194788973,168.887189181005));
#27194=CARTESIAN_POINT('Ctrl Pts',(33.9390539348382,-30.5377200098576,168.776059391785));
#27195=CARTESIAN_POINT('Ctrl Pts',(34.2802394590648,-32.8358833299508,168.664929602565));
#27196=CARTESIAN_POINT('Ctrl Pts',(32.5345745584143,-34.3690552914116,168.553799813346));
#27197=CARTESIAN_POINT('Ctrl Pts',(30.4507345015949,-33.7770119337325,168.450181518978));
#27198=CARTESIAN_POINT('Ctrl Pts',(29.949576897309,-32.5422713157353,168.383606487684));
#27199=CARTESIAN_POINT('Ctrl Pts',(29.9445666371917,-31.9981758746936,168.354074719462));
#27200=CARTESIAN_POINT('Origin',(32.,-32.,180.545925280538));
#27201=CARTESIAN_POINT('',(29.9444957030941,-32.0018139754894,169.754074719462));
#27202=CARTESIAN_POINT('',(29.9456997331156,-31.9981314623491,169.695925280538));
#27203=CARTESIAN_POINT('',(29.94525,-31.9999999999998,180.545925280538));
#27204=CARTESIAN_POINT('Ctrl Pts',(29.9456997331156,-31.9981314623491,169.695925280538));
#27205=CARTESIAN_POINT('Ctrl Pts',(29.9441243595525,-31.8219808270179,169.686377868442));
#27206=CARTESIAN_POINT('Ctrl Pts',(30.0454882735961,-30.9641640449656,169.639787193273));
#27207=CARTESIAN_POINT('Ctrl Pts',(31.2447903606557,-29.6917859067979,169.556153255031));
#27208=CARTESIAN_POINT('Ctrl Pts',(33.5295397995502,-30.113547800496,169.445023465812));
#27209=CARTESIAN_POINT('Ctrl Pts',(34.4144710010597,-32.2617702894598,169.333893676592));
#27210=CARTESIAN_POINT('Ctrl Pts',(33.0897045262574,-34.1704234482866,169.222763887372));
#27211=CARTESIAN_POINT('Ctrl Pts',(30.7676522863566,-34.092728604512,169.111634098152));
#27212=CARTESIAN_POINT('Ctrl Pts',(29.9551026106334,-32.7367311435647,169.036021229208));
#27213=CARTESIAN_POINT('Ctrl Pts',(29.9418849915895,-32.028544618634,168.997451623336));
#27214=CARTESIAN_POINT('Ctrl Pts',(29.9419793698485,-32.0005154407483,168.995925280538));
#27215=CARTESIAN_POINT('Ctrl Pts',(29.9444957030942,-32.0018139754894,169.754074719462));
#27216=CARTESIAN_POINT('Ctrl Pts',(29.9495181583603,-31.455422838666,169.724415714822));
#27217=CARTESIAN_POINT('Ctrl Pts',(30.4542707128816,-30.2184086098558,169.65771344711));
#27218=CARTESIAN_POINT('Ctrl Pts',(32.5426882959684,-29.6327901771656,169.553967916323));
#27219=CARTESIAN_POINT('Ctrl Pts',(34.2830899850343,-31.1719341498779,169.442838127104));
#27220=CARTESIAN_POINT('Ctrl Pts',(33.9340324788774,-33.4689150086206,169.331708337884));
#27221=CARTESIAN_POINT('Ctrl Pts',(31.8149694217593,-34.4215607811959,169.220578548664));
#27222=CARTESIAN_POINT('Ctrl Pts',(30.1913146775582,-33.3693337891571,169.12803400919));
#27223=CARTESIAN_POINT('Ctrl Pts',(29.9485310636531,-32.3417685781152,169.07253273279));
#27224=CARTESIAN_POINT('Ctrl Pts',(29.9485597394751,-32.0000193281882,169.054074719462));
#27225=CARTESIAN_POINT('Origin',(32.,-32.,180.545925280538));
#27226=CARTESIAN_POINT('',(29.9426483199887,-31.9988395038972,170.454074719462));
#27227=CARTESIAN_POINT('',(29.9483815094586,-32.0006260637531,170.395925280538));
#27228=CARTESIAN_POINT('',(29.94525,-31.9999999999998,180.545925280538));
#27229=CARTESIAN_POINT('Ctrl Pts',(29.9483815094586,-32.0006260637531,170.395925280538));
#27230=CARTESIAN_POINT('Ctrl Pts',(29.9494242847511,-31.6189087878515,170.375304113548));
#27231=CARTESIAN_POINT('Ctrl Pts',(30.2347805924059,-30.5500373066546,170.317639683485));
#27232=CARTESIAN_POINT('Ctrl Pts',(31.9562576167437,-29.5717742066846,170.22293199035));
#27233=CARTESIAN_POINT('Ctrl Pts',(34.0162673510713,-30.6461684490236,170.11180220113));
#27234=CARTESIAN_POINT('Ctrl Pts',(34.2310110712073,-32.9595746451244,170.00067241191));
#27235=CARTESIAN_POINT('Ctrl Pts',(32.4039576532821,-34.394788532161,169.88954262269));
#27236=CARTESIAN_POINT('Ctrl Pts',(30.3959344367109,-33.7033080295599,169.787960245566));
#27237=CARTESIAN_POINT('Ctrl Pts',(29.9502366941572,-32.5054324534664,169.723421131515));
#27238=CARTESIAN_POINT('Ctrl Pts',(29.9456997331156,-31.9981314623491,169.695925280538));
#27239=CARTESIAN_POINT('Ctrl Pts',(29.9426483199887,-31.9988395038972,170.454074719462));
#27240=CARTESIAN_POINT('Ctrl Pts',(29.9421898960853,-31.9310286004131,170.450385223002));
#27241=CARTESIAN_POINT('Ctrl Pts',(29.9759961349022,-31.1828456795586,170.409652463468));
#27242=CARTESIAN_POINT('Ctrl Pts',(30.8915734319869,-29.8390780959909,170.331876440861));
#27243=CARTESIAN_POINT('Ctrl Pts',(33.2142103690085,-29.896696381476,170.220746651642));
#27244=CARTESIAN_POINT('Ctrl Pts',(34.4256151438767,-31.8792353292564,170.109616862422));
#27245=CARTESIAN_POINT('Ctrl Pts',(33.4171232437699,-33.9722967940629,169.998487073202));
#27246=CARTESIAN_POINT('Ctrl Pts',(31.1116955190265,-34.2603336216113,169.887357283983));
#27247=CARTESIAN_POINT('Ctrl Pts',(30.0175516591059,-32.9549540883922,169.805886499402));
#27248=CARTESIAN_POINT('Ctrl Pts',(29.9432452529153,-32.1378500093702,169.761458977896));
#27249=CARTESIAN_POINT('Ctrl Pts',(29.9444957030942,-32.0018139754894,169.754074719462));
#27250=CARTESIAN_POINT('Origin',(32.,-32.,180.545925280538));
#27251=CARTESIAN_POINT('',(29.947997769693,-31.9989253081866,171.154074719462));
#27252=CARTESIAN_POINT('',(29.9434062815109,-32.0015359661597,171.095925280538));
#27253=CARTESIAN_POINT('',(29.94525,-31.9999999999998,180.545925280538));
#27254=CARTESIAN_POINT('Ctrl Pts',(29.9434062815109,-32.0015359661597,171.095925280538));
#27255=CARTESIAN_POINT('Ctrl Pts',(29.9482705648154,-31.4184384151654,171.064230358654));
#27256=CARTESIAN_POINT('Ctrl Pts',(30.5126647034041,-30.1456152646691,170.995492173698));
#27257=CARTESIAN_POINT('Ctrl Pts',(32.6715856784485,-29.666083425673,170.889710725668));
#27258=CARTESIAN_POINT('Ctrl Pts',(34.3250344044286,-31.2982814541151,170.778580936448));
#27259=CARTESIAN_POINT('Ctrl Pts',(33.8506368574238,-33.5726846859303,170.667451147228));
#27260=CARTESIAN_POINT('Ctrl Pts',(31.6825565278258,-34.4077839482373,170.556321358009));
#27261=CARTESIAN_POINT('Ctrl Pts',(30.1533956676068,-33.2932393776467,170.465812735779));
#27262=CARTESIAN_POINT('Ctrl Pts',(29.9475510736226,-32.3046145715278,170.412347376622));
#27263=CARTESIAN_POINT('Ctrl Pts',(29.9483815094586,-32.0006260637531,170.395925280538));
#27264=CARTESIAN_POINT('Ctrl Pts',(29.947997769693,-31.9989253081866,171.154074719462));
#27265=CARTESIAN_POINT('Ctrl Pts',(29.9467022464081,-31.7257714229441,171.139311468108));
#27266=CARTESIAN_POINT('Ctrl Pts',(30.1245753503767,-30.7688512324111,171.087504953681));
#27267=CARTESIAN_POINT('Ctrl Pts',(31.5753550359689,-29.6087932781905,170.99865517618));
#27268=CARTESIAN_POINT('Ctrl Pts',(33.778563379359,-30.3462451096045,170.88752538696));
#27269=CARTESIAN_POINT('Ctrl Pts',(34.3540498056764,-32.5971954824835,170.77639559774));
#27270=CARTESIAN_POINT('Ctrl Pts',(32.7751353784459,-34.3015990261089,170.665265808521));
#27271=CARTESIAN_POINT('Ctrl Pts',(30.5627970899358,-33.9129502869929,170.557825515761));
#27272=CARTESIAN_POINT('Ctrl Pts',(29.9467925613639,-32.6118632790567,170.487428486075));
#27273=CARTESIAN_POINT('Ctrl Pts',(29.9426483199887,-31.9988395038972,170.454074719462));
#27274=CARTESIAN_POINT('Origin',(32.,-32.,180.545925280538));
#27275=CARTESIAN_POINT('',(29.9465669261584,-32.0017453823422,171.854074719462));
#27276=CARTESIAN_POINT('',(29.9435984723696,-31.9983965385536,171.795925280538));
#27277=CARTESIAN_POINT('',(29.94525,-31.9999999999998,180.545925280538));
#27278=CARTESIAN_POINT('Ctrl Pts',(29.9435984723696,-31.9983965385536,171.795925280538));
#27279=CARTESIAN_POINT('Ctrl Pts',(29.9426938163605,-31.8930393932581,171.790199866834));
#27280=CARTESIAN_POINT('Ctrl Pts',(29.9979550929028,-31.1069760518487,171.747431190057));
#27281=CARTESIAN_POINT('Ctrl Pts',(31.0116476562013,-29.7815876073365,171.667619250206));
#27282=CARTESIAN_POINT('Ctrl Pts',(33.3276380087708,-29.9663896103033,171.556489460986));
#27283=CARTESIAN_POINT('Ctrl Pts',(34.4285884533479,-32.0123297883341,171.445359671767));
#27284=CARTESIAN_POINT('Ctrl Pts',(33.3069210823662,-34.0469858777925,171.334229882547));
#27285=CARTESIAN_POINT('Ctrl Pts',(30.9891737097718,-34.2082626905328,171.223100093327));
#27286=CARTESIAN_POINT('Ctrl Pts',(29.9937162558609,-32.8789600486766,171.143665225991));
#27287=CARTESIAN_POINT('Ctrl Pts',(29.9425854608491,-32.0999304238333,171.101273621728));
#27288=CARTESIAN_POINT('Ctrl Pts',(29.9434062815109,-32.0015359661597,171.095925280538));
#27289=CARTESIAN_POINT('Ctrl Pts',(29.9465669261584,-32.0017453823422,171.854074719462));
#27290=CARTESIAN_POINT('Ctrl Pts',(29.950420840573,-31.5245393636282,171.828237713214));
#27291=CARTESIAN_POINT('Ctrl Pts',(30.3537285820249,-30.3572748593973,171.765357443893));
#27292=CARTESIAN_POINT('Ctrl Pts',(32.2966168031358,-29.589561989181,171.665433911498));
#27293=CARTESIAN_POINT('Ctrl Pts',(34.1859362031082,-30.9417581335798,171.554304122278));
#27294=CARTESIAN_POINT('Ctrl Pts',(34.0747104954871,-33.2624457579713,171.443174333059));
#27295=CARTESIAN_POINT('Ctrl Pts',(32.0647322416946,-34.4277567153216,171.332044543839));
#27296=CARTESIAN_POINT('Ctrl Pts',(30.2704013335975,-33.5115699023856,171.235678005973));
#27297=CARTESIAN_POINT('Ctrl Pts',(29.9499529131283,-32.4111564365617,171.176354731181));
#27298=CARTESIAN_POINT('Ctrl Pts',(29.947997769693,-31.9989253081866,171.154074719462));
#27299=CARTESIAN_POINT('Origin',(32.,-32.,180.545925280538));
#27300=CARTESIAN_POINT('',(29.9418222803435,-32.0000454497003,172.554074719462));
#27301=CARTESIAN_POINT('',(29.948439498473,-31.9994832149056,172.495925280538));
#27302=CARTESIAN_POINT('',(29.94525,-31.9999999999998,180.545925280538));
#27303=CARTESIAN_POINT('Ctrl Pts',(29.948439498473,-31.9994832149056,172.495925280538));
#27304=CARTESIAN_POINT('Ctrl Pts',(29.9477393956008,-31.6884927931834,172.47912611194));
#27305=CARTESIAN_POINT('Ctrl Pts',(30.1602043752097,-30.6926560217899,172.425283680269));
#27306=CARTESIAN_POINT('Ctrl Pts',(31.7070205920295,-29.5891169738205,172.334397985525));
#27307=CARTESIAN_POINT('Ctrl Pts',(33.8665098861644,-30.4461870304743,172.223268196305));
#27308=CARTESIAN_POINT('Ctrl Pts',(34.3177895739383,-32.7252898664381,172.112138407085));
#27309=CARTESIAN_POINT('Ctrl Pts',(32.6478533790253,-34.3406152820788,172.001008617865));
#27310=CARTESIAN_POINT('Ctrl Pts',(30.5015906919452,-33.8409747289323,171.895604242349));
#27311=CARTESIAN_POINT('Ctrl Pts',(29.9485469148907,-32.5746971129646,171.827243129907));
#27312=CARTESIAN_POINT('Ctrl Pts',(29.9435984723696,-31.9983965385536,171.795925280538));
#27313=CARTESIAN_POINT('Ctrl Pts',(29.9418227658393,-32.0000454432629,172.554074719462));
#27314=CARTESIAN_POINT('Ctrl Pts',(29.9420432785979,-31.3223689366965,172.51716395832));
#27315=CARTESIAN_POINT('Ctrl Pts',(30.6781938256394,-29.9641726592493,172.443209934105));
#27316=CARTESIAN_POINT('Ctrl Pts',(32.9916984736889,-29.7830816277574,172.332212646816));
#27317=CARTESIAN_POINT('Ctrl Pts',(34.4003731567925,-31.6306740734072,172.221082857597));
#27318=CARTESIAN_POINT('Ctrl Pts',(33.6122523577626,-33.8162696019019,172.109953068377));
#27319=CARTESIAN_POINT('Ctrl Pts',(31.3486156850571,-34.3396348873596,171.998823279157));
#27320=CARTESIAN_POINT('Ctrl Pts',(30.0688018326291,-33.0979304878885,171.913530496186));
#27321=CARTESIAN_POINT('Ctrl Pts',(29.9448953720202,-32.2087234336225,171.865280976287));
#27322=CARTESIAN_POINT('Ctrl Pts',(29.9465669261584,-32.0017453823422,171.854074719462));
#27323=CARTESIAN_POINT('Origin',(32.,-32.,180.545925280538));
#27324=CARTESIAN_POINT('',(29.9464345031986,-31.9982258388275,173.254074719462));
#27325=CARTESIAN_POINT('',(29.9454927722119,-32.0018769614724,173.195925280538));
#27326=CARTESIAN_POINT('',(29.94525,-31.9999999999998,180.545925280538));
#27327=CARTESIAN_POINT('Ctrl Pts',(29.9454927722119,-32.0018769614724,173.195925280538));
#27328=CARTESIAN_POINT('Ctrl Pts',(29.9501525222033,-31.4877509589622,173.168052357046));
#27329=CARTESIAN_POINT('Ctrl Pts',(30.4058324164555,-30.282983669929,173.103136170481));
#27330=CARTESIAN_POINT('Ctrl Pts',(32.4282525794201,-29.6094365459927,173.001176720843));
#27331=CARTESIAN_POINT('Ctrl Pts',(34.2406392114377,-31.0631276375177,172.890046931623));
#27332=CARTESIAN_POINT('Ctrl Pts',(34.002417135868,-33.3742341552288,172.778917142403));
#27333=CARTESIAN_POINT('Ctrl Pts',(31.9316046128615,-34.4276564770234,172.667787353183));
#27334=CARTESIAN_POINT('Ctrl Pts',(30.2269632799385,-33.4359288810624,172.573456732562));
#27335=CARTESIAN_POINT('Ctrl Pts',(29.9492831681228,-32.3742469683386,172.516169375013));
#27336=CARTESIAN_POINT('Ctrl Pts',(29.948439498473,-31.9994832149056,172.495925280538));
#27337=CARTESIAN_POINT('Ctrl Pts',(29.9464345031986,-31.9982258388275,173.254074719462));
#27338=CARTESIAN_POINT('Ctrl Pts',(29.9447677417987,-31.7961753439703,173.2431334665));
#27339=CARTESIAN_POINT('Ctrl Pts',(30.0649649676893,-30.9119921533782,173.195148950464));
#27340=CARTESIAN_POINT('Ctrl Pts',(31.331936760099,-29.6650729263216,173.110121171355));
#27341=CARTESIAN_POINT('Ctrl Pts',(33.5992505047259,-30.1722716955089,172.998991382135));
#27342=CARTESIAN_POINT('Ctrl Pts',(34.4029475305773,-32.3521875880785,172.887861592915));
#27343=CARTESIAN_POINT('Ctrl Pts',(33.0074930353251,-34.2097852193539,172.776731803695));
#27344=CARTESIAN_POINT('Ctrl Pts',(30.6899918399505,-34.0450113819995,172.665602014476));
#27345=CARTESIAN_POINT('Ctrl Pts',(29.942927496564,-32.6850193607688,172.591382986398));
#27346=CARTESIAN_POINT('Ctrl Pts',(29.9418219742446,-32.002478160526,172.554207221393));
#27347=CARTESIAN_POINT('Ctrl Pts',(29.9418227658393,-32.0000454432629,172.554074719462));
#27348=CARTESIAN_POINT('Origin',(32.,-32.,180.545925280538));
#27349=CARTESIAN_POINT('',(29.9480727143584,-32.0010073134852,173.954074719462));
#27350=CARTESIAN_POINT('',(29.9420625872194,-31.9993626039853,173.895925280538));
#27351=CARTESIAN_POINT('',(29.94525,-31.9999999999998,180.545925280538));
#27352=CARTESIAN_POINT('Ctrl Pts',(29.9420625872194,-31.9993626039853,173.895925280538));
#27353=CARTESIAN_POINT('Ctrl Pts',(29.9419202242395,-31.9644052355927,173.894021865225));
#27354=CARTESIAN_POINT('Ctrl Pts',(29.9585679626885,-31.2492644513283,173.85507518684));
#27355=CARTESIAN_POINT('Ctrl Pts',(30.788964563955,-29.8948664954311,173.779085245381));
#27356=CARTESIAN_POINT('Ctrl Pts',(33.1116859870073,-29.8407528706267,173.667955456161));
#27357=CARTESIAN_POINT('Ctrl Pts',(34.417004450483,-31.7627588025647,173.556825666941));
#27358=CARTESIAN_POINT('Ctrl Pts',(33.5103066521985,-33.9018853056218,173.445695877722));
#27359=CARTESIAN_POINT('Ctrl Pts',(31.2213925844155,-34.3004270020612,173.334566088502));
#27360=CARTESIAN_POINT('Ctrl Pts',(30.0404202070706,-33.0217284667963,173.251309222774));
#27361=CARTESIAN_POINT('Ctrl Pts',(29.9439596897637,-32.17102714165,173.205095620119));
#27362=CARTESIAN_POINT('Ctrl Pts',(29.9454927722119,-32.0018769614724,173.195925280538));
#27363=CARTESIAN_POINT('Ctrl Pts',(29.9480727143584,-32.0010073134852,173.954074719462));
#27364=CARTESIAN_POINT('Ctrl Pts',(29.9498795736957,-31.5936421254285,173.932059711606));
#27365=CARTESIAN_POINT('Ctrl Pts',(30.2645751177761,-30.4982562863879,173.873001440676));
#27366=CARTESIAN_POINT('Ctrl Pts',(32.0474062508829,-29.5718431724288,173.776899906673));
#27367=CARTESIAN_POINT('Ctrl Pts',(34.0656489251761,-30.7227813617776,173.665770117453));
#27368=CARTESIAN_POINT('Ctrl Pts',(34.1934321041778,-33.0426161979683,173.554640328233));
#27369=CARTESIAN_POINT('Ctrl Pts',(32.3138100082167,-34.4082599964802,173.443510539014));
#27370=CARTESIAN_POINT('Ctrl Pts',(30.3603258304653,-33.6524318153962,173.343322002757));
#27371=CARTESIAN_POINT('Ctrl Pts',(29.9504108140525,-32.4802477861831,173.280176729573));
#27372=CARTESIAN_POINT('Ctrl Pts',(29.9464345031986,-31.9982258388275,173.254074719462));
#27373=CARTESIAN_POINT('Origin',(32.,-32.,180.545925280538));
#27374=CARTESIAN_POINT('',(29.9427579250369,-32.0012284951477,174.654074719462));
#27375=CARTESIAN_POINT('',(29.9473696346645,-31.9985278132519,174.595925280538));
#27376=CARTESIAN_POINT('',(29.94525,-31.9999999999998,180.545925280538));
#27377=CARTESIAN_POINT('Ctrl Pts',(29.9473696346645,-31.9985278132519,174.595925280538));
#27378=CARTESIAN_POINT('Ctrl Pts',(29.9457798475597,-31.7586047394747,174.582948110332));
#27379=CARTESIAN_POINT('Ctrl Pts',(30.0955630823059,-30.835744541956,174.532927677052));
#27380=CARTESIAN_POINT('Ctrl Pts',(31.4608841326267,-29.6319738217322,174.445863980699));
#27381=CARTESIAN_POINT('Ctrl Pts',(33.6969993749721,-30.2626494249117,174.33473419148));
#27382=CARTESIAN_POINT('Ctrl Pts',(34.380039192535,-32.4833294336296,174.22360440226));
#27383=CARTESIAN_POINT('Ctrl Pts',(32.8848929515401,-34.2616715861791,174.11247461304));
#27384=CARTESIAN_POINT('Ctrl Pts',(30.6193818318231,-33.9751494602321,174.003248239133));
#27385=CARTESIAN_POINT('Ctrl Pts',(29.9446908173321,-32.6447270682982,173.931065128299));
#27386=CARTESIAN_POINT('Ctrl Pts',(29.9420625872194,-31.9993626039853,173.895925280538));
#27387=CARTESIAN_POINT('Ctrl Pts',(29.9427579250369,-32.0012284951477,174.654074719462));
#27388=CARTESIAN_POINT('Ctrl Pts',(29.9470583104027,-31.3929901059041,174.620985956712));
#27389=CARTESIAN_POINT('Ctrl Pts',(30.5546327733145,-30.0963566968232,174.550853930888));
#27390=CARTESIAN_POINT('Ctrl Pts',(32.7586915544763,-29.6929282505587,174.443678641991));
#27391=CARTESIAN_POINT('Ctrl Pts',(34.3497283135974,-31.3860213487566,174.332548852772));
#27392=CARTESIAN_POINT('Ctrl Pts',(33.7903192018566,-33.6410210502512,174.221419063552));
#27393=CARTESIAN_POINT('Ctrl Pts',(31.5924293717799,-34.3941760826881,174.110289274332));
#27394=CARTESIAN_POINT('Ctrl Pts',(30.1290568288894,-33.2410713220018,174.021174492969));
#27395=CARTESIAN_POINT('Ctrl Pts',(29.9468392856247,-32.2790897948711,173.969102974679));
#27396=CARTESIAN_POINT('Ctrl Pts',(29.9480727143584,-32.0010073134852,173.954074719462));
#27397=CARTESIAN_POINT('Origin',(32.,-32.,180.545925280538));
#27398=CARTESIAN_POINT('',(29.9443485517367,-31.9982099443222,175.354074719462));
#27399=CARTESIAN_POINT('',(29.9473758037809,-32.0014692827641,175.295925280538));
#27400=CARTESIAN_POINT('',(29.94525,-31.9999999999998,180.545925280538));
#27401=CARTESIAN_POINT('Ctrl Pts',(29.9473758037809,-32.0014692827641,175.295925280538));
#27402=CARTESIAN_POINT('Ctrl Pts',(29.9503158166638,-31.5568102862893,175.271874355438));
#27403=CARTESIAN_POINT('Ctrl Pts',(30.3106831579398,-30.4229457911365,175.210780167264));
#27404=CARTESIAN_POINT('Ctrl Pts',(32.1803873356192,-29.5780887075362,175.112642716017));
#27405=CARTESIAN_POINT('Ctrl Pts',(34.1325316071812,-30.8378886267708,175.001512926798));
#27406=CARTESIAN_POINT('Ctrl Pts',(34.1330060781932,-33.1612402722117,174.890383137578));
#27407=CARTESIAN_POINT('Ctrl Pts',(32.1813765179305,-34.4218374136508,174.779253348358));
#27408=CARTESIAN_POINT('Ctrl Pts',(30.3110383976255,-33.5776135962551,174.681100729345));
#27409=CARTESIAN_POINT('Ctrl Pts',(29.9503178863629,-32.4434638727074,174.619991373405));
#27410=CARTESIAN_POINT('Ctrl Pts',(29.9473696346645,-31.9985278132519,174.595925280538));
#27411=CARTESIAN_POINT('Ctrl Pts',(29.9443485517367,-31.9982099443222,175.354074719462));
#27412=CARTESIAN_POINT('Ctrl Pts',(29.943149413098,-31.8670801077796,175.346955464891));
#27413=CARTESIAN_POINT('Ctrl Pts',(30.014316216057,-31.05494551359,175.302792947247));
#27414=CARTESIAN_POINT('Ctrl Pts',(31.095588515948,-29.7460628226547,175.221587166529));
#27415=CARTESIAN_POINT('Ctrl Pts',(33.4030129572177,-30.0176409069538,175.110457377309));
#27416=CARTESIAN_POINT('Ctrl Pts',(34.4264151550835,-32.1034525354194,174.99932758809));
#27417=CARTESIAN_POINT('Ctrl Pts',(33.2291885163936,-34.0945855253653,174.88819779887));
#27418=CARTESIAN_POINT('Ctrl Pts',(30.9070218774947,-34.168776557331,174.777068009651));
#27419=CARTESIAN_POINT('Ctrl Pts',(29.9787266265999,-32.8270204983606,174.699026983181));
#27420=CARTESIAN_POINT('Ctrl Pts',(29.9422439778867,-32.0739202099972,174.658029219785));
#27421=CARTESIAN_POINT('Ctrl Pts',(29.9427579250369,-32.0012284951477,174.654074719462));
#27422=CARTESIAN_POINT('Origin',(32.,-32.,180.545925280538));
#27423=CARTESIAN_POINT('',(29.9485555074385,-31.9999002033617,176.054074719462));
#27424=CARTESIAN_POINT('',(29.9420662633311,-32.0006422348648,175.995925280538));
#27425=CARTESIAN_POINT('',(29.94525,-31.9999999999998,180.545925280538));
#27426=CARTESIAN_POINT('Ctrl Pts',(29.9420662633311,-32.0006422348648,175.995925280538));
#27427=CARTESIAN_POINT('Ctrl Pts',(29.9447110108764,-31.3555532629716,175.960800600544));
#27428=CARTESIAN_POINT('Ctrl Pts',(30.6188898084219,-30.0253746830828,175.888632657476));
#27429=CARTESIAN_POINT('Ctrl Pts',(32.8839691281437,-29.737967179745,175.779421451336));
#27430=CARTESIAN_POINT('Ctrl Pts',(34.3798415845562,-31.515698511429,175.668291662116));
#27431=CARTESIAN_POINT('Ctrl Pts',(33.6977088310898,-33.7366573134195,175.557161872896));
#27432=CARTESIAN_POINT('Ctrl Pts',(31.4618513662959,-34.3682461754341,175.446032083677));
#27433=CARTESIAN_POINT('Ctrl Pts',(30.0958008212723,-33.1648235855215,175.358953219557));
#27434=CARTESIAN_POINT('Ctrl Pts',(29.9457876053703,-32.2416745946567,175.308917618511));
#27435=CARTESIAN_POINT('Ctrl Pts',(29.9473758037809,-32.0014692827641,175.295925280538));
#27436=CARTESIAN_POINT('Ctrl Pts',(29.9485555074385,-31.9999002033617,176.054074719462));
#27437=CARTESIAN_POINT('Ctrl Pts',(29.9484095554287,-31.6630592207583,176.035881709997));
#27438=CARTESIAN_POINT('Ctrl Pts',(30.186216996793,-30.6405615756134,175.980645437459));
#27439=CARTESIAN_POINT('Ctrl Pts',(31.797694004055,-29.5798212429744,175.888365901848));
#27440=CARTESIAN_POINT('Ctrl Pts',(33.9235011368215,-30.5173212389216,175.777236112628));
#27441=CARTESIAN_POINT('Ctrl Pts',(34.2889408886545,-32.8117527580092,175.666106323408));
#27442=CARTESIAN_POINT('Ctrl Pts',(32.5595667617289,-34.3632769560673,175.554976534188));
#27443=CARTESIAN_POINT('Ctrl Pts',(30.4616782926144,-33.7911184932325,175.45096599954));
#27444=CARTESIAN_POINT('Ctrl Pts',(29.9493888315104,-32.5493814615627,175.383998727965));
#27445=CARTESIAN_POINT('Ctrl Pts',(29.9443485517367,-31.9982099443222,175.354074719462));
#27446=CARTESIAN_POINT('Origin',(32.,-32.,180.545925280538));
#27447=CARTESIAN_POINT('',(29.9447147880612,-32.0018424760523,176.754074719462));
#27448=CARTESIAN_POINT('',(29.9454843966674,-31.9981228561279,176.695925280538));
#27449=CARTESIAN_POINT('',(29.94525,-31.9999999999998,180.545925280538));
#27450=CARTESIAN_POINT('Ctrl Pts',(29.9454843966674,-31.9981228561279,176.695925280538));
#27451=CARTESIAN_POINT('Ctrl Pts',(29.9439531582599,-31.8292542067848,176.686770108723));
#27452=CARTESIAN_POINT('Ctrl Pts',(30.040218113941,-30.9788389407387,176.640571673835));
#27453=CARTESIAN_POINT('Ctrl Pts',(31.2204530706714,-29.6998912018496,176.557329975874));
#27454=CARTESIAN_POINT('Ctrl Pts',(33.5095297265273,-30.0974979883034,176.446200186654));
#27455=CARTESIAN_POINT('Ctrl Pts',(34.4171011468898,-32.2362539844767,176.335070397435));
#27456=CARTESIAN_POINT('Ctrl Pts',(33.1125678099616,-34.1587928959332,176.223940608215));
#27457=CARTESIAN_POINT('Ctrl Pts',(30.7898244786656,-34.1056279602598,176.112810818995));
#27458=CARTESIAN_POINT('Ctrl Pts',(29.9587089014121,-32.7512990085116,176.036805709769));
#27459=CARTESIAN_POINT('Ctrl Pts',(29.9419218017192,-32.0358783362693,175.997843863617));
#27460=CARTESIAN_POINT('Ctrl Pts',(29.9420662633311,-32.0006422348648,175.995925280538));
#27461=CARTESIAN_POINT('Ctrl Pts',(29.9447147880613,-32.0018424760523,176.754074719462));
#27462=CARTESIAN_POINT('Ctrl Pts',(29.9496923513297,-31.4625295795391,176.724807955103));
#27463=CARTESIAN_POINT('Ctrl Pts',(30.443411768081,-30.2325366450479,176.658497927671));
#27464=CARTESIAN_POINT('Ctrl Pts',(32.5176554945262,-29.6271903313891,176.555144637166));
#27465=CARTESIAN_POINT('Ctrl Pts',(34.2742165827931,-31.1478662855577,176.444014847946));
#27466=CARTESIAN_POINT('Ctrl Pts',(33.9494393162254,-33.4484057729775,176.332885058727));
#27467=CARTESIAN_POINT('Ctrl Pts',(31.8405563287846,-34.4233800048647,176.221755269507));
#27468=CARTESIAN_POINT('Ctrl Pts',(30.198950093782,-33.3839739680937,176.128818489752));
#27469=CARTESIAN_POINT('Ctrl Pts',(29.9487067321385,-32.3489099677957,176.072924973071));
#27470=CARTESIAN_POINT('Ctrl Pts',(29.9485555074385,-31.9999002033617,176.054074719462));
#27471=CARTESIAN_POINT('Origin',(32.,-32.,180.545925280538));
#27472=CARTESIAN_POINT('',(29.9424957081741,-31.9989451554456,177.454074719462));
#27473=CARTESIAN_POINT('',(29.9484415989894,-32.0005123628745,177.395925280538));
#27474=CARTESIAN_POINT('',(29.94525,-31.9999999999998,180.545925280538));
#27475=CARTESIAN_POINT('Ctrl Pts',(29.9484415989894,-32.0005123628745,177.395925280538));
#27476=CARTESIAN_POINT('Ctrl Pts',(29.9492773483985,-31.6260284359245,177.375696353829));
#27477=CARTESIAN_POINT('Ctrl Pts',(30.2266509686561,-30.5646358117479,177.318424164048));
#27478=CARTESIAN_POINT('Ctrl Pts',(31.9306130769242,-29.5723716763149,177.224108711192));
#27479=CARTESIAN_POINT('Ctrl Pts',(34.0018556801289,-30.624948091138,177.112978921973));
#27480=CARTESIAN_POINT('Ctrl Pts',(34.2410216781083,-32.9359571289216,177.001849132753));
#27481=CARTESIAN_POINT('Ctrl Pts',(32.4292289371827,-34.3903883387013,176.890719343533));
#27482=CARTESIAN_POINT('Ctrl Pts',(30.4062329402781,-33.7175672281966,176.788744726128));
#27483=CARTESIAN_POINT('Ctrl Pts',(29.9501487893529,-32.5125232845343,176.723813371796));
#27484=CARTESIAN_POINT('Ctrl Pts',(29.9454843966674,-31.9981228561279,176.695925280538));
#27485=CARTESIAN_POINT('Ctrl Pts',(29.9424957081741,-31.9989451554456,177.454074719462));
#27486=CARTESIAN_POINT('Ctrl Pts',(29.942116389599,-31.9383552528433,177.450777463283));
#27487=CARTESIAN_POINT('Ctrl Pts',(29.9720237344228,-31.1974434463136,177.41043694403));
#27488=CARTESIAN_POINT('Ctrl Pts',(30.8688116391535,-29.8509059591332,177.333053161704));
#27489=CARTESIAN_POINT('Ctrl Pts',(33.1919274501366,-29.8839891344978,177.221923372484));
#27490=CARTESIAN_POINT('Ctrl Pts',(34.4242043461506,-31.8536226808824,177.110793583265));
#27491=CARTESIAN_POINT('Ctrl Pts',(33.4378756346499,-33.9572190768126,176.999663794045));
#27492=CARTESIAN_POINT('Ctrl Pts',(31.1356187743909,-34.2695898408057,176.888534004825));
#27493=CARTESIAN_POINT('Ctrl Pts',(30.0224146577596,-32.9696107419196,176.806670979964));
#27494=CARTESIAN_POINT('Ctrl Pts',(29.9433921951746,-32.145143798841,176.761851218177));
#27495=CARTESIAN_POINT('Ctrl Pts',(29.9447147880613,-32.0018424760523,176.754074719462));
#27496=CARTESIAN_POINT('Origin',(32.,-32.,180.545925280538));
#27497=CARTESIAN_POINT('',(29.9478812476528,-31.9988328933335,178.154074719462));
#27498=CARTESIAN_POINT('',(29.943606531648,-32.0016074863584,178.095925280538));
#27499=CARTESIAN_POINT('',(29.94525,-31.9999999999998,180.545925280538));
#27500=CARTESIAN_POINT('Ctrl Pts',(29.943606531648,-32.0016074863584,178.095925280538));
#27501=CARTESIAN_POINT('Ctrl Pts',(29.9485578247094,-31.4255805091263,178.064622598935));
#27502=CARTESIAN_POINT('Ctrl Pts',(30.5011474122479,-30.159563307867,177.99627665426));
#27503=CARTESIAN_POINT('Ctrl Pts',(32.6468974928654,-29.6591214220926,177.890887446511));
#27504=CARTESIAN_POINT('Ctrl Pts',(34.3174930665853,-31.2737629757136,177.779757657291));
#27505=CARTESIAN_POINT('Ctrl Pts',(33.8671444034839,-33.5530507580587,177.668627868071));
#27506=CARTESIAN_POINT('Ctrl Pts',(31.7080052904067,-34.4110023564038,177.557498078852));
#27507=CARTESIAN_POINT('Ctrl Pts',(30.1604802792039,-33.3079112757927,177.46659721634));
#27508=CARTESIAN_POINT('Ctrl Pts',(29.9477469219122,-32.3117843745653,177.412739616902));
#27509=CARTESIAN_POINT('Ctrl Pts',(29.9484415989894,-32.0005123628745,177.395925280538));
#27510=CARTESIAN_POINT('Ctrl Pts',(29.9478812476528,-31.9988328933335,178.154074719462));
#27511=CARTESIAN_POINT('Ctrl Pts',(29.9464999762263,-31.7329725296047,178.139703708389));
#27512=CARTESIAN_POINT('Ctrl Pts',(30.1180175877586,-30.7835296862564,178.088289434242));
#27513=CARTESIAN_POINT('Ctrl Pts',(31.5501292172184,-29.6134187564108,177.999831897022));
#27514=CARTESIAN_POINT('Ctrl Pts',(33.7609939876075,-30.3275486926383,177.888702107803));
#27515=CARTESIAN_POINT('Ctrl Pts',(34.3602276546561,-32.5723003233786,177.777572318583));
#27516=CARTESIAN_POINT('Ctrl Pts',(32.7994009204969,-34.2932828161059,177.666442529363));
#27517=CARTESIAN_POINT('Ctrl Pts',(30.5749909453294,-33.9266902436017,177.558609996323));
#27518=CARTESIAN_POINT('Ctrl Pts',(29.9463778715709,-32.6190568967199,177.487820726356));
#27519=CARTESIAN_POINT('Ctrl Pts',(29.9424957081741,-31.9989451554456,177.454074719462));
#27520=CARTESIAN_POINT('Origin',(32.,-32.,180.545925280538));
#27521=CARTESIAN_POINT('',(29.9473399238087,-32.0021821257033,178.854074719462));
#27522=CARTESIAN_POINT('',(29.9434031644741,-31.9984978685597,178.795925280538));
#27523=CARTESIAN_POINT('',(29.94525,-31.9999999999998,180.545925280538));
#27524=CARTESIAN_POINT('',(31.4698297828105,-33.9851743256715,179.));
#27525=CARTESIAN_POINT('Ctrl Pts',(31.4698297828105,-33.9851743256715,179.));
#27526=CARTESIAN_POINT('Ctrl Pts',(30.8097602092464,-33.8088929660693,178.962956736927));
#27527=CARTESIAN_POINT('Ctrl Pts',(30.0751175985078,-33.1125987294256,178.914314976747));
#27528=CARTESIAN_POINT('Ctrl Pts',(29.945727943022,-32.2164517005945,178.865673216568));
#27529=CARTESIAN_POINT('Ctrl Pts',(29.9473399238087,-32.0021821257033,178.854074719462));
#27530=CARTESIAN_POINT('',(32.5313334939852,-33.9887337712632,179.));
#27531=CARTESIAN_POINT('Origin',(32.,-32.,179.));
#27532=CARTESIAN_POINT('Ctrl Pts',(32.5313343692877,-33.9887364495514,179.));
#27533=CARTESIAN_POINT('Ctrl Pts',(31.8868946933699,-34.159991273772,178.963685183163));
#27534=CARTESIAN_POINT('Ctrl Pts',(30.5070458965819,-33.8408668084245,178.895660276675));
#27535=CARTESIAN_POINT('Ctrl Pts',(29.9482461031169,-32.5817482342877,178.827635370188));
#27536=CARTESIAN_POINT('Ctrl Pts',(29.9434031644741,-31.9984978685597,178.795925280538));
#27537=CARTESIAN_POINT('Origin',(-32.,32.,172.));
#27538=CARTESIAN_POINT('',(-33.6685050626317,32.0006151176758,166.67148036339));
#27539=CARTESIAN_POINT('',(-33.6648360378126,32.0014707311122,166.47851963661));
#27540=CARTESIAN_POINT('',(-33.666,32.,172.));
#27541=CARTESIAN_POINT('',(-31.3249228143254,30.4769022377465,166.));
#27542=CARTESIAN_POINT('Ctrl Pts',(-33.6648360378126,32.0014707311122,166.47851963661));
#27543=CARTESIAN_POINT('Ctrl Pts',(-33.6661874191336,32.1712146992289,166.467186143366));
#27544=CARTESIAN_POINT('Ctrl Pts',(-33.6423113042436,32.3405776208252,166.455852650123));
#27545=CARTESIAN_POINT('Ctrl Pts',(-33.5916296311322,32.5014768113726,166.444519156879));
#27546=CARTESIAN_POINT('Ctrl Pts',(-33.4259777434308,33.0273721302816,166.407475893806));
#27547=CARTESIAN_POINT('Ctrl Pts',(-32.9739636180178,33.4628498968862,166.370432630732));
#27548=CARTESIAN_POINT('Ctrl Pts',(-32.4421510381962,33.6090489648024,166.333389367659));
#27549=CARTESIAN_POINT('Ctrl Pts',(-31.9103384583745,33.7552480327186,166.296346104586));
#27550=CARTESIAN_POINT('Ctrl Pts',(-31.2987274241441,33.6121684019463,166.259302841513));
#27551=CARTESIAN_POINT('Ctrl Pts',(-30.8877524385943,33.2444370387197,166.222259578439));
#27552=CARTESIAN_POINT('Ctrl Pts',(-30.4767774530445,32.876705675493,166.185216315366));
#27553=CARTESIAN_POINT('Ctrl Pts',(-30.2664385161753,32.2843225798121,166.148173052293));
#27554=CARTESIAN_POINT('Ctrl Pts',(-30.3518675256649,31.740487435795,166.11112978922));
#27555=CARTESIAN_POINT('Ctrl Pts',(-30.4372965351546,31.1966522917781,166.074086526147));
#27556=CARTESIAN_POINT('Ctrl Pts',(-30.818493491003,30.701365099425,166.037043263073));
#27557=CARTESIAN_POINT('Ctrl Pts',(-31.3249228143254,30.4769022377465,166.));
#27558=CARTESIAN_POINT('',(-33.666,32.,166.));
#27559=CARTESIAN_POINT('Origin',(-32.,32.,166.));
#27560=CARTESIAN_POINT('',(-33.666,32.,165.));
#27561=CARTESIAN_POINT('',(-33.666,32.,172.));
#27562=CARTESIAN_POINT('Origin',(-32.,32.,165.));
#27563=CARTESIAN_POINT('',(-33.6146845196279,31.5775541929288,166.));
#27564=CARTESIAN_POINT('Origin',(-32.,32.,166.));
#27565=CARTESIAN_POINT('Ctrl Pts',(-33.6146867573337,31.5775537367509,166.));
#27566=CARTESIAN_POINT('Ctrl Pts',(-33.4771458934448,31.0546920138059,166.036314816837));
#27567=CARTESIAN_POINT('Ctrl Pts',(-33.0618726298578,30.6037510878086,166.072629633674));
#27568=CARTESIAN_POINT('Ctrl Pts',(-32.55154570234,30.4250925829005,166.108944450512));
#27569=CARTESIAN_POINT('Ctrl Pts',(-32.0309820240448,30.2428503310052,166.145987713585));
#27570=CARTESIAN_POINT('Ctrl Pts',(-31.4115130336904,30.3439235949188,166.183030976658));
#27571=CARTESIAN_POINT('Ctrl Pts',(-30.9761439936337,30.6822433025976,166.220074239731));
#27572=CARTESIAN_POINT('Ctrl Pts',(-30.540774953577,31.0205630102763,166.257117502805));
#27573=CARTESIAN_POINT('Ctrl Pts',(-30.289505863818,31.5961291617202,166.294160765878));
#27574=CARTESIAN_POINT('Ctrl Pts',(-30.3375418657213,32.145477184728,166.331204028951));
#27575=CARTESIAN_POINT('Ctrl Pts',(-30.3855778676247,32.6948252077357,166.368247292024));
#27576=CARTESIAN_POINT('Ctrl Pts',(-30.7329189611904,33.2179551023072,166.405290555098));
#27577=CARTESIAN_POINT('Ctrl Pts',(-31.2205128733123,33.4755289762921,166.442333818171));
#27578=CARTESIAN_POINT('Ctrl Pts',(-31.7081067854342,33.733102850277,166.479377081244));
#27579=CARTESIAN_POINT('Ctrl Pts',(-32.3359535161123,33.7251207036753,166.516420344317));
#27580=CARTESIAN_POINT('Ctrl Pts',(-32.8168082612591,33.4552137540432,166.553463607391));
#27581=CARTESIAN_POINT('Ctrl Pts',(-33.297663006406,33.1853068044112,166.590506870464));
#27582=CARTESIAN_POINT('Ctrl Pts',(-33.6315257660216,32.6534750517487,166.627550133537));
#27583=CARTESIAN_POINT('Ctrl Pts',(-33.6655960048379,32.1030923182541,166.66459339661));
#27584=CARTESIAN_POINT('Ctrl Pts',(-33.6677074153297,32.0689838435741,166.666889052204));
#27585=CARTESIAN_POINT('Ctrl Pts',(-33.6686674534897,32.0348041226669,166.669184707797));
#27586=CARTESIAN_POINT('Ctrl Pts',(-33.6685050626317,32.0006151176758,166.67148036339));
#27587=CARTESIAN_POINT('Origin',(-32.,32.,172.));
#27588=CARTESIAN_POINT('',(-33.6641555473647,32.0011304727029,167.37148036339));
#27589=CARTESIAN_POINT('',(-33.6638024982419,31.9991033788539,167.17851963661));
#27590=CARTESIAN_POINT('',(-33.666,32.,172.));
#27591=CARTESIAN_POINT('Ctrl Pts',(-33.6638024982419,31.9991033788539,167.17851963661));
#27592=CARTESIAN_POINT('Ctrl Pts',(-33.6621591163747,32.335235888221,167.156112388472));
#27593=CARTESIAN_POINT('Ctrl Pts',(-33.5633805615657,32.6722563635698,167.133705140335));
#27594=CARTESIAN_POINT('Ctrl Pts',(-33.3741093586448,32.9469160213603,167.111297892197));
#27595=CARTESIAN_POINT('Ctrl Pts',(-33.0612095809052,33.4009784701134,167.074254629124));
#27596=CARTESIAN_POINT('Ctrl Pts',(-32.5009923748203,33.6846081008443,167.037211366051));
#27597=CARTESIAN_POINT('Ctrl Pts',(-31.9498062295419,33.6680232843613,167.000168102977));
#27598=CARTESIAN_POINT('Ctrl Pts',(-31.3986200842636,33.6514384678784,166.963124839904));
#27599=CARTESIAN_POINT('Ctrl Pts',(-30.8564649997919,33.3346392041815,166.926081576831));
#27600=CARTESIAN_POINT('Ctrl Pts',(-30.5714360756128,32.862579407757,166.889038313758));
#27601=CARTESIAN_POINT('Ctrl Pts',(-30.2864071514337,32.3905196113324,166.851995050685));
#27602=CARTESIAN_POINT('Ctrl Pts',(-30.2585043875471,31.76319928218,166.814951787611));
#27603=CARTESIAN_POINT('Ctrl Pts',(-30.5004799090271,31.2677006444648,166.777908524538));
#27604=CARTESIAN_POINT('Ctrl Pts',(-30.742455430507,30.7722020067496,166.740865261465));
#27605=CARTESIAN_POINT('Ctrl Pts',(-31.2543092373534,30.4085250604714,166.703821998392));
#27606=CARTESIAN_POINT('Ctrl Pts',(-31.8018524365455,30.3430378599729,166.666778735318));
#27607=CARTESIAN_POINT('Ctrl Pts',(-32.3493956357375,30.2775506594744,166.629735472245));
#27608=CARTESIAN_POINT('Ctrl Pts',(-32.9326282272752,30.5102532047555,166.592692209172));
#27609=CARTESIAN_POINT('Ctrl Pts',(-33.2845996980492,30.9347609130028,166.555648946099));
#27610=CARTESIAN_POINT('Ctrl Pts',(-33.5288844815547,31.229389262788,166.529939176269));
#27611=CARTESIAN_POINT('Ctrl Pts',(-33.6617704602393,31.6164104274241,166.504229406439));
#27612=CARTESIAN_POINT('Ctrl Pts',(-33.6648360378126,32.0014707311122,166.47851963661));
#27613=CARTESIAN_POINT('Ctrl Pts',(-33.6685050626317,32.0006151176758,166.67148036339));
#27614=CARTESIAN_POINT('Ctrl Pts',(-33.6660470746791,31.4831219322734,166.70622797087));
#27615=CARTESIAN_POINT('Ctrl Pts',(-33.4064339327629,30.9635017081271,166.74097557835));
#27616=CARTESIAN_POINT('Ctrl Pts',(-32.990035371472,30.656627002776,166.77572318583));
#27617=CARTESIAN_POINT('Ctrl Pts',(-32.5461267812728,30.3294781351193,166.812766448903));
#27618=CARTESIAN_POINT('Ctrl Pts',(-31.9240318828574,30.2441141141327,166.849809711977));
#27619=CARTESIAN_POINT('Ctrl Pts',(-31.4084114760072,30.4395995850539,166.88685297505));
#27620=CARTESIAN_POINT('Ctrl Pts',(-30.892791069157,30.6350850559752,166.923896238123));
#27621=CARTESIAN_POINT('Ctrl Pts',(-30.4836451538719,31.1114200188042,166.960939501196));
#27622=CARTESIAN_POINT('Ctrl Pts',(-30.3681998517826,31.6506349336804,166.997982764269));
#27623=CARTESIAN_POINT('Ctrl Pts',(-30.2527545496932,32.1898498485566,167.035026027343));
#27624=CARTESIAN_POINT('Ctrl Pts',(-30.4310098607996,32.79194471548,167.072069290416));
#27625=CARTESIAN_POINT('Ctrl Pts',(-30.821395564629,33.1814047989309,167.109112553489));
#27626=CARTESIAN_POINT('Ctrl Pts',(-31.2117812684584,33.5708648823819,167.146155816562));
#27627=CARTESIAN_POINT('Ctrl Pts',(-31.8142973650107,33.7476901823603,167.183199079636));
#27628=CARTESIAN_POINT('Ctrl Pts',(-32.3532365200937,33.6309661003555,167.220242342709));
#27629=CARTESIAN_POINT('Ctrl Pts',(-32.8921756751766,33.5142420183508,167.257285605782));
#27630=CARTESIAN_POINT('Ctrl Pts',(-33.3675378887901,33.1039685543629,167.294328868855));
#27631=CARTESIAN_POINT('Ctrl Pts',(-33.5617996139899,32.5878847682657,167.331372131929));
#27632=CARTESIAN_POINT('Ctrl Pts',(-33.6319112761567,32.4016232078717,167.344741542416));
#27633=CARTESIAN_POINT('Ctrl Pts',(-33.6654072127856,32.2015789545508,167.358110952903));
#27634=CARTESIAN_POINT('Ctrl Pts',(-33.6641555473647,32.0011304727029,167.37148036339));
#27635=CARTESIAN_POINT('Origin',(-32.,32.,172.));
#27636=CARTESIAN_POINT('',(-33.6644090592112,31.9987501654189,168.07148036339));
#27637=CARTESIAN_POINT('',(-33.6681507222124,31.9990863362662,167.87851963661));
#27638=CARTESIAN_POINT('',(-33.666,32.,172.));
#27639=CARTESIAN_POINT('Ctrl Pts',(-33.6681507222124,31.9990863362662,167.87851963661));
#27640=CARTESIAN_POINT('Ctrl Pts',(-33.6648561568213,32.497992284639,167.845038633578));
#27641=CARTESIAN_POINT('Ctrl Pts',(-33.4261729971981,32.9996326774274,167.811557630547));
#27642=CARTESIAN_POINT('Ctrl Pts',(-33.0352709662068,33.308831725257,167.778076627516));
#27643=CARTESIAN_POINT('Ctrl Pts',(-32.6027783447553,33.6509284557524,167.741033364442));
#27644=CARTESIAN_POINT('Ctrl Pts',(-31.9839526063196,33.7574552117728,167.703990101369));
#27645=CARTESIAN_POINT('Ctrl Pts',(-31.4619649990783,33.5796660081348,167.666946838296));
#27646=CARTESIAN_POINT('Ctrl Pts',(-30.9399773918371,33.4018768044968,167.629903575223));
#27647=CARTESIAN_POINT('Ctrl Pts',(-30.5148279157903,32.9397716412004,167.592860312149));
#27648=CARTESIAN_POINT('Ctrl Pts',(-30.3810627764268,32.4048071708948,167.555817049076));
#27649=CARTESIAN_POINT('Ctrl Pts',(-30.2472976370633,31.8698427005891,167.518773786003));
#27650=CARTESIAN_POINT('Ctrl Pts',(-30.404916834383,31.2620189232743,167.48173052293));
#27651=CARTESIAN_POINT('Ctrl Pts',(-30.7817944533159,30.8594730384074,167.444687259856));
#27652=CARTESIAN_POINT('Ctrl Pts',(-31.1586720722489,30.4569271535405,167.407643996783));
#27653=CARTESIAN_POINT('Ctrl Pts',(-31.7548081127951,30.2596591611215,167.37060073371));
#27654=CARTESIAN_POINT('Ctrl Pts',(-32.2974144133735,30.3579371433043,167.333557470637));
#27655=CARTESIAN_POINT('Ctrl Pts',(-32.8400207139519,30.4562151254872,167.296514207563));
#27656=CARTESIAN_POINT('Ctrl Pts',(-33.3290972745624,30.8500390822719,167.25947094449));
#27657=CARTESIAN_POINT('Ctrl Pts',(-33.5408443801705,31.3591986940519,167.222427681417));
#27658=CARTESIAN_POINT('Ctrl Pts',(-33.6245069288544,31.5603707038703,167.207791666481));
#27659=CARTESIAN_POINT('Ctrl Pts',(-33.6648759259742,31.7795476173752,167.193155651546));
#27660=CARTESIAN_POINT('Ctrl Pts',(-33.6638024982419,31.9991033788539,167.17851963661));
#27661=CARTESIAN_POINT('Ctrl Pts',(-33.6641555473647,32.0011304727029,167.37148036339));
#27662=CARTESIAN_POINT('Ctrl Pts',(-33.661939163726,31.6461867887672,167.395154215976));
#27663=CARTESIAN_POINT('Ctrl Pts',(-33.5507700288489,31.2899756271486,167.418828068562));
#27664=CARTESIAN_POINT('Ctrl Pts',(-33.3410204559846,31.0067777430984,167.442501921148));
#27665=CARTESIAN_POINT('Ctrl Pts',(-33.0128183359932,30.5636486122348,167.479545184222));
#27666=CARTESIAN_POINT('Ctrl Pts',(-32.4432528592241,30.2992844587142,167.516588447295));
#27667=CARTESIAN_POINT('Ctrl Pts',(-31.8929540089092,30.3346569212847,167.553631710368));
#27668=CARTESIAN_POINT('Ctrl Pts',(-31.3426551585943,30.3700293838553,167.590674973441));
#27669=CARTESIAN_POINT('Ctrl Pts',(-30.8116229347336,30.7051384625169,167.627718236515));
#27670=CARTESIAN_POINT('Ctrl Pts',(-30.5428548480621,31.1866400424654,167.664761499588));
#27671=CARTESIAN_POINT('Ctrl Pts',(-30.2740867613905,31.6681416224139,167.701804762661));
#27672=CARTESIAN_POINT('Ctrl Pts',(-30.2675828119081,32.2960357036492,167.738848025734));
#27673=CARTESIAN_POINT('Ctrl Pts',(-30.5263191497755,32.7830013677887,167.775891288808));
#27674=CARTESIAN_POINT('Ctrl Pts',(-30.7850554876429,33.2699670319283,167.812934551881));
#27675=CARTESIAN_POINT('Ctrl Pts',(-31.30903211286,33.616004278972,167.849977814954));
#27676=CARTESIAN_POINT('Ctrl Pts',(-31.8584801736076,33.662768336769,167.887021078027));
#27677=CARTESIAN_POINT('Ctrl Pts',(-32.4079282343552,33.709532394566,167.924064341101));
#27678=CARTESIAN_POINT('Ctrl Pts',(-32.9828477306334,33.4570232631162,167.961107604174));
#27679=CARTESIAN_POINT('Ctrl Pts',(-33.3201586130435,33.0207877538663,167.998150867247));
#27680=CARTESIAN_POINT('Ctrl Pts',(-33.5427347307921,32.7329357718042,168.022594032628));
#27681=CARTESIAN_POINT('Ctrl Pts',(-33.6618541533202,32.3650878520419,168.047037198009));
#27682=CARTESIAN_POINT('Ctrl Pts',(-33.6644090592112,31.9987501654189,168.07148036339));
#27683=CARTESIAN_POINT('Origin',(-32.,32.,172.));
#27684=CARTESIAN_POINT('',(-33.668651770133,31.9995820784764,168.77148036339));
#27685=CARTESIAN_POINT('',(-33.6665541529016,32.0014790085921,168.57851963661));
#27686=CARTESIAN_POINT('',(-33.666,32.,172.));
#27687=CARTESIAN_POINT('Ctrl Pts',(-33.6665541529016,32.0014790085921,168.57851963661));
#27688=CARTESIAN_POINT('Ctrl Pts',(-33.6675874214856,32.1136880980852,168.571008141758));
#27689=CARTESIAN_POINT('Ctrl Pts',(-33.6572223312059,32.2257073770859,168.563496646906));
#27690=CARTESIAN_POINT('Ctrl Pts',(-33.6347589488988,32.3352456179051,168.555985152054));
#27691=CARTESIAN_POINT('Ctrl Pts',(-33.5239798035077,32.8754382095492,168.518941888981));
#27692=CARTESIAN_POINT('Ctrl Pts',(-33.1189687371489,33.3552916534455,168.481898625907));
#27693=CARTESIAN_POINT('Ctrl Pts',(-32.6050566180813,33.5552276150071,168.444855362834));
#27694=CARTESIAN_POINT('Ctrl Pts',(-32.0911444990138,33.7551635765688,168.407812099761));
#27695=CARTESIAN_POINT('Ctrl Pts',(-31.4683313272375,33.6751820557957,168.370768836687));
#27696=CARTESIAN_POINT('Ctrl Pts',(-31.0216130323314,33.3518821640458,168.333725573614));
#27697=CARTESIAN_POINT('Ctrl Pts',(-30.5748947374253,33.0285822722958,168.296682310541));
#27698=CARTESIAN_POINT('Ctrl Pts',(-30.3042713193893,32.461964009569,168.259639047468));
#27699=CARTESIAN_POINT('Ctrl Pts',(-30.3335785884741,31.9113088182212,168.222595784395));
#27700=CARTESIAN_POINT('Ctrl Pts',(-30.3628858575589,31.3606536268733,168.185552521321));
#27701=CARTESIAN_POINT('Ctrl Pts',(-30.6921238137645,30.8259615069045,168.148509258248));
#27702=CARTESIAN_POINT('Ctrl Pts',(-31.1706349503903,30.5519046778648,168.111465995175));
#27703=CARTESIAN_POINT('Ctrl Pts',(-31.6491460870161,30.277847848825,168.074422732101));
#27704=CARTESIAN_POINT('Ctrl Pts',(-32.2769304040622,30.2644263107144,168.037379469028));
#27705=CARTESIAN_POINT('Ctrl Pts',(-32.7667172084993,30.5177816770287,168.000336205955));
#27706=CARTESIAN_POINT('Ctrl Pts',(-33.2565040129364,30.7711370433429,167.963292942882));
#27707=CARTESIAN_POINT('Ctrl Pts',(-33.6082933047646,31.2912693140819,167.926249679809));
#27708=CARTESIAN_POINT('Ctrl Pts',(-33.661108198445,31.8401688019366,167.889206416735));
#27709=CARTESIAN_POINT('Ctrl Pts',(-33.6661871350657,31.8929536418872,167.885644156694));
#27710=CARTESIAN_POINT('Ctrl Pts',(-33.6685012522917,31.9460045118401,167.882081896652));
#27711=CARTESIAN_POINT('Ctrl Pts',(-33.6681507222124,31.9990863362662,167.87851963661));
#27712=CARTESIAN_POINT('Ctrl Pts',(-33.6644090592112,31.9987501654189,168.07148036339));
#27713=CARTESIAN_POINT('Ctrl Pts',(-33.6657260761899,31.8099083944035,168.084080461082));
#27714=CARTESIAN_POINT('Ctrl Pts',(-33.6360689501427,31.6214679305664,168.096680558775));
#27715=CARTESIAN_POINT('Ctrl Pts',(-33.573642203788,31.4445932896112,168.109280656467));
#27716=CARTESIAN_POINT('Ctrl Pts',(-33.3901126435801,30.9245962216557,168.14632391954));
#27717=CARTESIAN_POINT('Ctrl Pts',(-32.9233512546222,30.5045639727946,168.183367182613));
#27718=CARTESIAN_POINT('Ctrl Pts',(-32.3869455163211,30.3767010230759,168.220410445686));
#27719=CARTESIAN_POINT('Ctrl Pts',(-31.8505397780201,30.2488380733572,168.25745370876));
#27720=CARTESIAN_POINT('Ctrl Pts',(-31.2444896903759,30.4131444227807,168.294496971833));
#27721=CARTESIAN_POINT('Ctrl Pts',(-30.8461204879495,30.7944343765193,168.331540234906));
#27722=CARTESIAN_POINT('Ctrl Pts',(-30.4477512855231,31.1757243302579,168.36858349798));
#27723=CARTESIAN_POINT('Ctrl Pts',(-30.2570629683146,31.7739978883115,168.405626761053));
#27724=CARTESIAN_POINT('Ctrl Pts',(-30.3613134760073,32.3154883146385,168.442670024126));
#27725=CARTESIAN_POINT('Ctrl Pts',(-30.4655639837,32.8569787409655,168.479713287199));
#27726=CARTESIAN_POINT('Ctrl Pts',(-30.864753316294,33.3416860355659,168.516756550272));
#27727=CARTESIAN_POINT('Ctrl Pts',(-31.376214599859,33.5478107685873,168.553799813346));
#27728=CARTESIAN_POINT('Ctrl Pts',(-31.887675883424,33.7539355016086,168.590843076419));
#27729=CARTESIAN_POINT('Ctrl Pts',(-32.51140911796,33.681477673051,168.627886339492));
#27730=CARTESIAN_POINT('Ctrl Pts',(-32.9619973573219,33.3635935924051,168.664929602565));
#27731=CARTESIAN_POINT('Ctrl Pts',(-33.3940194106328,33.0588077119969,168.70044652284));
#27732=CARTESIAN_POINT('Ctrl Pts',(-33.6668711504497,32.5284041436776,168.735963443115));
#27733=CARTESIAN_POINT('Ctrl Pts',(-33.668651770133,31.9995820784764,168.77148036339));
#27734=CARTESIAN_POINT('Origin',(-32.,32.,172.));
#27735=CARTESIAN_POINT('',(-33.6656352839714,32.0015150181746,169.47148036339));
#27736=CARTESIAN_POINT('',(-33.6633165285087,31.9999843286219,169.27851963661));
#27737=CARTESIAN_POINT('',(-33.666,32.,172.));
#27738=CARTESIAN_POINT('Ctrl Pts',(-33.6633165285087,31.9999843286219,169.27851963661));
#27739=CARTESIAN_POINT('Ctrl Pts',(-33.6632931177575,32.278986154171,169.259934386864));
#27740=CARTESIAN_POINT('Ctrl Pts',(-33.5968742307684,32.5579984542452,169.241349137118));
#27741=CARTESIAN_POINT('Ctrl Pts',(-33.4641220334618,32.8007328620376,169.222763887372));
#27742=CARTESIAN_POINT('Ctrl Pts',(-33.1995264732404,33.2845398943726,169.185720624299));
#27743=CARTESIAN_POINT('Ctrl Pts',(-32.6714110598214,33.6242271051177,169.148677361225));
#27744=CARTESIAN_POINT('Ctrl Pts',(-32.1214385428041,33.6643554685053,169.111634098152));
#27745=CARTESIAN_POINT('Ctrl Pts',(-31.5714660257869,33.7044838318928,169.074590835079));
#27746=CARTESIAN_POINT('Ctrl Pts',(-30.9996364051713,33.4450533479228,169.037547572006));
#27747=CARTESIAN_POINT('Ctrl Pts',(-30.6676158147234,33.0047779993727,169.000504308933));
#27748=CARTESIAN_POINT('Ctrl Pts',(-30.3355952242756,32.5645026508225,168.963461045859));
#27749=CARTESIAN_POINT('Ctrl Pts',(-30.2433836639953,31.9433824376922,168.926417782786));
#27750=CARTESIAN_POINT('Ctrl Pts',(-30.4331766438925,31.4256386015936,168.889374519713));
#27751=CARTESIAN_POINT('Ctrl Pts',(-30.6229696237896,30.907894765495,168.85233125664));
#27752=CARTESIAN_POINT('Ctrl Pts',(-31.094767143864,30.4935273064282,168.815287993566));
#27753=CARTESIAN_POINT('Ctrl Pts',(-31.6326772171009,30.3721485269141,168.778244730493));
#27754=CARTESIAN_POINT('Ctrl Pts',(-32.1705872903377,30.2507697473999,168.74120146742));
#27755=CARTESIAN_POINT('Ctrl Pts',(-32.774609916737,30.4223796474386,168.704158204347));
#27756=CARTESIAN_POINT('Ctrl Pts',(-33.1683476177251,30.8084504671538,168.667114941273));
#27757=CARTESIAN_POINT('Ctrl Pts',(-33.4822446548877,31.1162352846591,168.637583173052));
#27758=CARTESIAN_POINT('Ctrl Pts',(-33.6624918125908,31.5603241002161,168.608051404831));
#27759=CARTESIAN_POINT('Ctrl Pts',(-33.6665541529016,32.0014790085921,168.57851963661));
#27760=CARTESIAN_POINT('Ctrl Pts',(-33.668651770133,31.9995820784764,168.77148036339));
#27761=CARTESIAN_POINT('Ctrl Pts',(-33.6687282924218,31.9768559033307,168.773006706189));
#27762=CARTESIAN_POINT('Ctrl Pts',(-33.6683041847769,31.954132648997,168.774533048987));
#27763=CARTESIAN_POINT('Ctrl Pts',(-33.6673705657548,31.9314303480246,168.776059391785));
#27764=CARTESIAN_POINT('Ctrl Pts',(-33.6447122906379,31.3804615170241,168.813102654858));
#27765=CARTESIAN_POINT('Ctrl Pts',(-33.3219524962164,30.8418341877571,168.850145917932));
#27766=CARTESIAN_POINT('Ctrl Pts',(-32.8467843143074,30.5620213055182,168.887189181005));
#27767=CARTESIAN_POINT('Ctrl Pts',(-32.3716161323985,30.2822084232793,168.924232444078));
#27768=CARTESIAN_POINT('Ctrl Pts',(-31.7440395630021,30.2612099880684,168.961275707151));
#27769=CARTESIAN_POINT('Ctrl Pts',(-31.2512302413907,30.5086347699753,168.998318970225));
#27770=CARTESIAN_POINT('Ctrl Pts',(-30.7584209197793,30.7560595518823,169.035362233298));
#27771=CARTESIAN_POINT('Ctrl Pts',(-30.4003788459528,31.2719075509071,169.072405496371));
#27772=CARTESIAN_POINT('Ctrl Pts',(-30.3409421314876,31.8201295197669,169.109448759444));
#27773=CARTESIAN_POINT('Ctrl Pts',(-30.2815054170224,32.3683514886268,169.146492022518));
#27774=CARTESIAN_POINT('Ctrl Pts',(-30.5206740619185,32.9489474273217,169.183535285591));
#27775=CARTESIAN_POINT('Ctrl Pts',(-30.9490057911116,33.2962397824545,169.220578548664));
#27776=CARTESIAN_POINT('Ctrl Pts',(-31.3773375203046,33.6435321375873,169.257621811737));
#27777=CARTESIAN_POINT('Ctrl Pts',(-31.9948323337946,33.7575209091579,169.294665074811));
#27778=CARTESIAN_POINT('Ctrl Pts',(-32.5189279531536,33.5860454533744,169.331708337884));
#27779=CARTESIAN_POINT('Ctrl Pts',(-33.0430235725127,33.414569997591,169.368751600957));
#27780=CARTESIAN_POINT('Ctrl Pts',(-33.4737199977408,32.9576303144533,169.40579486403));
#27781=CARTESIAN_POINT('Ctrl Pts',(-33.6139328800083,32.4243195253129,169.442838127104));
#27782=CARTESIAN_POINT('Ctrl Pts',(-33.6500708996387,32.2868657089774,169.452385539199));
#27783=CARTESIAN_POINT('Ctrl Pts',(-33.6669126034726,32.1443386930928,169.461932951295));
#27784=CARTESIAN_POINT('Ctrl Pts',(-33.6656352839714,32.0015150181746,169.47148036339));
#27785=CARTESIAN_POINT('Origin',(-32.,32.,172.));
#27786=CARTESIAN_POINT('',(-33.6634608884496,31.9994923848796,170.17148036339));
#27787=CARTESIAN_POINT('',(-33.6666116665711,31.998529220922,169.97851963661));
#27788=CARTESIAN_POINT('',(-33.666,32.,172.));
#27789=CARTESIAN_POINT('Ctrl Pts',(-33.6666116665711,31.998529220922,169.97851963661));
#27790=CARTESIAN_POINT('Ctrl Pts',(-33.6625394383818,32.441545489247,169.94886063197));
#27791=CARTESIAN_POINT('Ctrl Pts',(-33.4805649416139,32.8875165690686,169.91920162733));
#27792=CARTESIAN_POINT('Ctrl Pts',(-33.1642582641494,33.1955455405692,169.88954262269));
#27793=CARTESIAN_POINT('Ctrl Pts',(-32.7692001154543,33.5802650672038,169.852499359617));
#27794=CARTESIAN_POINT('Ctrl Pts',(-32.164593063158,33.7498044530175,169.815456096544));
#27795=CARTESIAN_POINT('Ctrl Pts',(-31.6271020160461,33.6265833943509,169.778412833471));
#27796=CARTESIAN_POINT('Ctrl Pts',(-31.0896109689343,33.5033623356844,169.741369570397));
#27797=CARTESIAN_POINT('Ctrl Pts',(-30.6192359270069,33.0873808325376,169.704326307324));
#27798=CARTESIAN_POINT('Ctrl Pts',(-30.4312179589473,32.568989765185,169.667283044251));
#27799=CARTESIAN_POINT('Ctrl Pts',(-30.2431999908877,32.0505986978324,169.630239781178));
#27800=CARTESIAN_POINT('Ctrl Pts',(-30.3375390966959,31.4297980662739,169.593196518104));
#27801=CARTESIAN_POINT('Ctrl Pts',(-30.6710662130869,30.990662873359,169.556153255031));
#27802=CARTESIAN_POINT('Ctrl Pts',(-31.0045933294779,30.5515276804442,169.519109991958));
#27803=CARTESIAN_POINT('Ctrl Pts',(-31.5773084564517,30.2940579261729,169.482066728885));
#27804=CARTESIAN_POINT('Ctrl Pts',(-32.1271402573229,30.3360703740291,169.445023465812));
#27805=CARTESIAN_POINT('Ctrl Pts',(-32.6769720581941,30.3780828218853,169.407980202738));
#27806=CARTESIAN_POINT('Ctrl Pts',(-33.2039205329627,30.7195774718689,169.370936939665));
#27807=CARTESIAN_POINT('Ctrl Pts',(-33.466856916835,31.2042882238232,169.333893676592));
#27808=CARTESIAN_POINT('Ctrl Pts',(-33.5978735410497,31.4458111561248,169.315435663264));
#27809=CARTESIAN_POINT('Ctrl Pts',(-33.6633397789876,31.7228925765749,169.296977649937));
#27810=CARTESIAN_POINT('Ctrl Pts',(-33.6633165285087,31.9999843286219,169.27851963661));
#27811=CARTESIAN_POINT('Ctrl Pts',(-33.6656352839714,32.0015150181746,169.47148036339));
#27812=CARTESIAN_POINT('Ctrl Pts',(-33.6619566969046,31.590193244031,169.498976214368));
#27813=CARTESIAN_POINT('Ctrl Pts',(-33.5079992892159,31.1764109857402,169.526472065345));
#27814=CARTESIAN_POINT('Ctrl Pts',(-33.2318839374529,30.8742609692386,169.553967916323));
#27815=CARTESIAN_POINT('Ctrl Pts',(-32.8598927733233,30.4671950974478,169.591011179396));
#27816=CARTESIAN_POINT('Ctrl Pts',(-32.2661811057571,30.2627452490095,169.62805444247));
#27817=CARTESIAN_POINT('Ctrl Pts',(-31.7224281745655,30.3544665659857,169.665097705543));
#27818=CARTESIAN_POINT('Ctrl Pts',(-31.1786752433738,30.4461878829619,169.702140968616));
#27819=CARTESIAN_POINT('Ctrl Pts',(-30.6848810485567,30.8340803653528,169.739184231689));
#27820=CARTESIAN_POINT('Ctrl Pts',(-30.4670031361747,31.3406465164756,169.776227494763));
#27821=CARTESIAN_POINT('Ctrl Pts',(-30.2491252237927,31.8472126675985,169.813270757836));
#27822=CARTESIAN_POINT('Ctrl Pts',(-30.307163593846,32.4724524874533,169.850314020909));
#27823=CARTESIAN_POINT('Ctrl Pts',(-30.6145602028981,32.9302596246963,169.887357283982));
#27824=CARTESIAN_POINT('Ctrl Pts',(-30.9219568119501,33.3880667619393,169.924400547056));
#27825=CARTESIAN_POINT('Ctrl Pts',(-31.4787116600011,33.6784412165704,169.961443810129));
#27826=CARTESIAN_POINT('Ctrl Pts',(-32.0300567474602,33.6685092126404,169.998487073202));
#27827=CARTESIAN_POINT('Ctrl Pts',(-32.5814018349192,33.6585772087105,170.035530336275));
#27828=CARTESIAN_POINT('Ctrl Pts',(-33.1273371617865,33.3483387462194,170.072573599349));
#27829=CARTESIAN_POINT('Ctrl Pts',(-33.4180456826985,32.879757263405,170.109616862422));
#27830=CARTESIAN_POINT('Ctrl Pts',(-33.5798767002072,32.6189082937509,170.130238029411));
#27831=CARTESIAN_POINT('Ctrl Pts',(-33.6626154018631,32.308990355304,170.150859196401));
#27832=CARTESIAN_POINT('Ctrl Pts',(-33.6634608884496,31.9994923848796,170.17148036339));
#27833=CARTESIAN_POINT('Origin',(-32.,32.,172.));
#27834=CARTESIAN_POINT('',(-33.6674948241645,31.9987546321869,170.87148036339));
#27835=CARTESIAN_POINT('',(-33.6681095326863,32.0009409351981,170.67851963661));
#27836=CARTESIAN_POINT('',(-33.666,32.,172.));
#27837=CARTESIAN_POINT('Ctrl Pts',(-33.6681095326863,32.0009409351981,170.67851963661));
#27838=CARTESIAN_POINT('Ctrl Pts',(-33.6684812247459,32.0559223054817,170.674830140149));
#27839=CARTESIAN_POINT('Ctrl Pts',(-33.665998456693,32.1108696974031,170.671140643689));
#27840=CARTESIAN_POINT('Ctrl Pts',(-33.6605508302034,32.1655215560754,170.667451147228));
#27841=CARTESIAN_POINT('Ctrl Pts',(-33.6058555992036,32.7142368617943,170.630407884155));
#27842=CARTESIAN_POINT('Ctrl Pts',(-33.2522862982848,33.2331607873135,170.593364621082));
#27843=CARTESIAN_POINT('Ctrl Pts',(-32.7616343223977,33.4848365580631,170.556321358009));
#27844=CARTESIAN_POINT('Ctrl Pts',(-32.2709823465107,33.7365123288128,170.519278094935));
#27845=CARTESIAN_POINT('Ctrl Pts',(-31.6432476956554,33.720939944793,170.482234831862));
#27846=CARTESIAN_POINT('Ctrl Pts',(-31.1656783423139,33.4452452444934,170.445191568789));
#27847=CARTESIAN_POINT('Ctrl Pts',(-30.6881089889724,33.1695505441939,170.408148305716));
#27848=CARTESIAN_POINT('Ctrl Pts',(-30.3607049331446,32.6337335276146,170.371105042642));
#27849=CARTESIAN_POINT('Ctrl Pts',(-30.3332844955028,32.0829811561954,170.334061779569));
#27850=CARTESIAN_POINT('Ctrl Pts',(-30.305864057861,31.5322287847762,170.297018516496));
#27851=CARTESIAN_POINT('Ctrl Pts',(-30.5784272384051,30.9665410585172,170.259975253423));
#27852=CARTESIAN_POINT('Ctrl Pts',(-31.0262506036305,30.6447736136405,170.22293199035));
#27853=CARTESIAN_POINT('Ctrl Pts',(-31.4740739688559,30.3230061687638,170.185888727276));
#27854=CARTESIAN_POINT('Ctrl Pts',(-32.0971575187626,30.2451590052694,170.148845464203));
#27855=CARTESIAN_POINT('Ctrl Pts',(-32.6103815994432,30.4468545630637,170.11180220113));
#27856=CARTESIAN_POINT('Ctrl Pts',(-33.1236056801237,30.6485501208579,170.074758938057));
#27857=CARTESIAN_POINT('Ctrl Pts',(-33.526970291578,31.1297883999409,170.037715674983));
#27858=CARTESIAN_POINT('Ctrl Pts',(-33.6358979747582,31.67035737321,170.00067241191));
#27859=CARTESIAN_POINT('Ctrl Pts',(-33.6576117790083,31.7781151857933,169.993288153477));
#27860=CARTESIAN_POINT('Ctrl Pts',(-33.6676255369189,31.8882306234047,169.985903895043));
#27861=CARTESIAN_POINT('Ctrl Pts',(-33.6666116665711,31.998529220922,169.97851963661));
#27862=CARTESIAN_POINT('Ctrl Pts',(-33.6634608884496,31.9994923848796,170.17148036339));
#27863=CARTESIAN_POINT('Ctrl Pts',(-33.6641342093131,31.7530172260951,170.187902459474));
#27864=CARTESIAN_POINT('Ctrl Pts',(-33.6128703196196,31.5068084137666,170.204324555558));
#27865=CARTESIAN_POINT('Ctrl Pts',(-33.5082545871963,31.2858610072716,170.220746651642));
#27866=CARTESIAN_POINT('Ctrl Pts',(-33.2722732558253,30.78747073709,170.257789914715));
#27867=CARTESIAN_POINT('Ctrl Pts',(-32.7648288781263,30.4176146998644,170.294833177788));
#27868=CARTESIAN_POINT('Ctrl Pts',(-32.2181252498319,30.3455370127683,170.331876440861));
#27869=CARTESIAN_POINT('Ctrl Pts',(-31.6714216215375,30.2734593256722,170.368919703935));
#27870=CARTESIAN_POINT('Ctrl Pts',(-31.0854587426478,30.4991599887057,170.405962967008));
#27871=CARTESIAN_POINT('Ctrl Pts',(-30.7283700492912,30.9193596022755,170.443006230081));
#27872=CARTESIAN_POINT('Ctrl Pts',(-30.3712813559346,31.3395592158453,170.480049493154));
#27873=CARTESIAN_POINT('Ctrl Pts',(-30.2430668481111,31.9542577799514,170.517092756227));
#27874=CARTESIAN_POINT('Ctrl Pts',(-30.4023967893865,32.482172564723,170.554136019301));
#27875=CARTESIAN_POINT('Ctrl Pts',(-30.561726730662,33.0100873494947,170.591179282374));
#27876=CARTESIAN_POINT('Ctrl Pts',(-31.0086011210365,33.4512183549319,170.628222545447));
#27877=CARTESIAN_POINT('Ctrl Pts',(-31.53853266255,33.6037064248798,170.66526580852));
#27878=CARTESIAN_POINT('Ctrl Pts',(-32.0684642040635,33.7561944948277,170.702309071594));
#27879=CARTESIAN_POINT('Ctrl Pts',(-32.6814528967161,33.6200396292864,170.739352334667));
#27880=CARTESIAN_POINT('Ctrl Pts',(-33.0969984385428,33.2575455564586,170.77639559774));
#27881=CARTESIAN_POINT('Ctrl Pts',(-33.4525471239035,32.9473887190672,170.808090519624));
#27882=CARTESIAN_POINT('Ctrl Pts',(-33.6635508428324,32.4715325754067,170.839785441507));
#27883=CARTESIAN_POINT('Ctrl Pts',(-33.6674948241645,31.9987546321869,170.87148036339));
#27884=CARTESIAN_POINT('Origin',(-32.,32.,172.));
#27885=CARTESIAN_POINT('',(-33.6673389950091,32.0013000932747,171.57148036339));
#27886=CARTESIAN_POINT('',(-33.6637721760092,32.0008713647136,171.37851963661));
#27887=CARTESIAN_POINT('',(-33.666,32.,172.));
#27888=CARTESIAN_POINT('Ctrl Pts',(-33.6637721760092,32.0008713647136,171.37851963661));
#27889=CARTESIAN_POINT('Ctrl Pts',(-33.6648225918241,32.2223457019845,171.363756385255));
#27890=CARTESIAN_POINT('Ctrl Pts',(-33.6237242828597,32.4434460300688,171.348993133901));
#27891=CARTESIAN_POINT('Ctrl Pts',(-33.5386395641721,32.646076417136,171.334229882547));
#27892=CARTESIAN_POINT('Ctrl Pts',(-33.3251489487098,33.1545071519798,171.297186619474));
#27893=CARTESIAN_POINT('Ctrl Pts',(-32.8347264499723,33.5466538895163,171.2601433564));
#27894=CARTESIAN_POINT('Ctrl Pts',(-32.2917867441766,33.6430724089759,171.223100093327));
#27895=CARTESIAN_POINT('Ctrl Pts',(-31.7488470383809,33.7394909284354,171.186056830254));
#27896=CARTESIAN_POINT('Ctrl Pts',(-31.153390125527,33.5401812298181,171.149013567181));
#27897=CARTESIAN_POINT('Ctrl Pts',(-30.7778938602062,33.1363463504994,171.111970304107));
#27898=CARTESIAN_POINT('Ctrl Pts',(-30.4023975948853,32.7325114711806,171.074927041034));
#27899=CARTESIAN_POINT('Ctrl Pts',(-30.2468619770976,32.1241514111603,171.037883777961));
#27900=CARTESIAN_POINT('Ctrl Pts',(-30.3824592621858,31.5896484352088,171.000840514888));
#27901=CARTESIAN_POINT('Ctrl Pts',(-30.5180565472741,31.0551454592573,170.963797251814));
#27902=CARTESIAN_POINT('Ctrl Pts',(-30.9447867352383,30.5944995673746,170.926753988741));
#27903=CARTESIAN_POINT('Ctrl Pts',(-31.4673804059142,30.4184998219378,170.889710725668));
#27904=CARTESIAN_POINT('Ctrl Pts',(-31.9899740765901,30.242500076501,170.852667462595));
#27905=CARTESIAN_POINT('Ctrl Pts',(-32.6084312299776,30.3511464775101,170.815624199521));
#27906=CARTESIAN_POINT('Ctrl Pts',(-33.0397492261309,30.694723020974,170.778580936448));
#27907=CARTESIAN_POINT('Ctrl Pts',(-33.4281080958976,31.0040794570328,170.745227169835));
#27908=CARTESIAN_POINT('Ctrl Pts',(-33.6647493640718,31.5038986390065,170.711873403223));
#27909=CARTESIAN_POINT('Ctrl Pts',(-33.6681095326863,32.0009409351981,170.67851963661));
#27910=CARTESIAN_POINT('Ctrl Pts',(-33.6674948241645,31.9987546321869,170.87148036339));
#27911=CARTESIAN_POINT('Ctrl Pts',(-33.6681603490043,31.9189759926714,170.87682870458));
#27912=CARTESIAN_POINT('Ctrl Pts',(-33.6629299142687,31.8392850039256,170.88217704577));
#27913=CARTESIAN_POINT('Ctrl Pts',(-33.6515031400339,31.7604926322801,170.88752538696));
#27914=CARTESIAN_POINT('Ctrl Pts',(-33.5723599086977,31.214767061044,170.924568650033));
#27915=CARTESIAN_POINT('Ctrl Pts',(-33.1959710550246,30.7121491986861,170.961611913106));
#27916=CARTESIAN_POINT('Ctrl Pts',(-32.6945700775718,30.4826342536897,170.99865517618));
#27917=CARTESIAN_POINT('Ctrl Pts',(-32.193169100119,30.2531193086932,171.035698439253));
#27918=CARTESIAN_POINT('Ctrl Pts',(-31.5667559988865,30.2967072810581,171.072741702326));
#27919=CARTESIAN_POINT('Ctrl Pts',(-31.1019740124148,30.5934525509761,171.109784965399));
#27920=CARTESIAN_POINT('Ctrl Pts',(-30.6371920259431,30.8901978208941,171.146828228473));
#27921=CARTESIAN_POINT('Ctrl Pts',(-30.334041154232,31.4401003883653,171.183871491546));
#27922=CARTESIAN_POINT('Ctrl Pts',(-30.3312415924095,31.9915278202373,171.220914754619));
#27923=CARTESIAN_POINT('Ctrl Pts',(-30.328442030587,32.5429552521093,171.257958017692));
#27924=CARTESIAN_POINT('Ctrl Pts',(-30.625993778653,33.0959075483822,171.295001280766));
#27925=CARTESIAN_POINT('Ctrl Pts',(-31.0877387700997,33.3973567365404,171.332044543839));
#27926=CARTESIAN_POINT('Ctrl Pts',(-31.5494837615464,33.6988059246985,171.369087806912));
#27927=CARTESIAN_POINT('Ctrl Pts',(-32.1754219963737,33.7487520047421,171.406131069985));
#27928=CARTESIAN_POINT('Ctrl Pts',(-32.6791275323335,33.5243399212644,171.443174333058));
#27929=CARTESIAN_POINT('Ctrl Pts',(-33.1828330682934,33.2999278377868,171.480217596132));
#27930=CARTESIAN_POINT('Ctrl Pts',(-33.5643059053856,32.8011575907879,171.517260859205));
#27931=CARTESIAN_POINT('Ctrl Pts',(-33.6489861418072,32.2562637408254,171.554304122278));
#27932=CARTESIAN_POINT('Ctrl Pts',(-33.6620743350666,32.1720448449463,171.560029535982));
#27933=CARTESIAN_POINT('Ctrl Pts',(-33.6680724939006,32.0867241091558,171.565754949686));
#27934=CARTESIAN_POINT('Ctrl Pts',(-33.6673389950091,32.0013000932747,171.57148036339));
#27935=CARTESIAN_POINT('Origin',(-32.,32.,172.));
#27936=CARTESIAN_POINT('',(-33.6634138707132,32.0004190115247,172.27148036339));
#27937=CARTESIAN_POINT('',(-33.6649323100607,31.9985848365388,172.07851963661));
#27938=CARTESIAN_POINT('',(-33.666,32.,172.));
#27939=CARTESIAN_POINT('Ctrl Pts',(-33.6649323100607,31.9985848365388,172.07851963661));
#27940=CARTESIAN_POINT('Ctrl Pts',(-33.6618075397867,32.3855055154906,172.052682630362));
#27941=CARTESIAN_POINT('Ctrl Pts',(-33.5274443256813,32.7743832740356,172.026845624113));
#27942=CARTESIAN_POINT('Ctrl Pts',(-33.2809243517091,33.069607054209,172.001008617865));
#27943=CARTESIAN_POINT('Ctrl Pts',(-32.9274815355819,33.4928779258177,171.963965354792));
#27944=CARTESIAN_POINT('Ctrl Pts',(-32.3434916821162,33.7236356820849,171.926922091719));
#27945=CARTESIAN_POINT('Ctrl Pts',(-31.7961853817046,33.6562868249745,171.889878828646));
#27946=CARTESIAN_POINT('Ctrl Pts',(-31.248879081293,33.5889379678641,171.852835565572));
#27947=CARTESIAN_POINT('Ctrl Pts',(-30.7382563339356,33.2234824973761,171.815792302499));
#27948=CARTESIAN_POINT('Ctrl Pts',(-30.4979753400865,32.727150855206,171.778749039426));
#27949=CARTESIAN_POINT('Ctrl Pts',(-30.2576943462375,32.230819213036,171.741705776352));
#27950=CARTESIAN_POINT('Ctrl Pts',(-30.2877551058968,31.6036113991838,171.704662513279));
#27951=CARTESIAN_POINT('Ctrl Pts',(-30.5744019784421,31.1325343083757,171.667619250206));
#27952=CARTESIAN_POINT('Ctrl Pts',(-30.8610488509874,30.6614572175675,171.630575987133));
#27953=CARTESIAN_POINT('Ctrl Pts',(-31.4042818364187,30.3465108498032,171.59353272406));
#27954=CARTESIAN_POINT('Ctrl Pts',(-31.9555204661607,30.3318129552462,171.556489460986));
#27955=CARTESIAN_POINT('Ctrl Pts',(-32.5067590959028,30.3171150606892,171.519446197913));
#27956=CARTESIAN_POINT('Ctrl Pts',(-33.0660033699556,30.6026656393395,171.48240293484));
#27957=CARTESIAN_POINT('Ctrl Pts',(-33.3773461408885,31.0577982947402,171.445359671767));
#27958=CARTESIAN_POINT('Ctrl Pts',(-33.5646061177235,31.3315420217963,171.423079660048));
#27959=CARTESIAN_POINT('Ctrl Pts',(-33.662186937358,31.66663260447,171.400799648329));
#27960=CARTESIAN_POINT('Ctrl Pts',(-33.6637721760092,32.0008713647136,171.37851963661));
#27961=CARTESIAN_POINT('Ctrl Pts',(-33.6673389950091,32.0013000932747,171.57148036339));
#27962=CARTESIAN_POINT('Ctrl Pts',(-33.6633267770306,31.5340331672145,171.60279821276));
#27963=CARTESIAN_POINT('Ctrl Pts',(-33.4578994056388,31.0636760401785,171.634116062129));
#27964=CARTESIAN_POINT('Ctrl Pts',(-33.109710516809,30.7536577638475,171.665433911498));
#27965=CARTESIAN_POINT('Ctrl Pts',(-32.6978670196382,30.3869630897581,171.702477174571));
#27966=CARTESIAN_POINT('Ctrl Pts',(-32.0862923895458,30.2445911945054,171.739520437645));
#27967=CARTESIAN_POINT('Ctrl Pts',(-31.5548398611366,30.3916906853776,171.776563700718));
#27968=CARTESIAN_POINT('Ctrl Pts',(-31.0233873327274,30.5387901762498,171.813606963791));
#27969=CARTESIAN_POINT('Ctrl Pts',(-30.5720569060016,30.9753610532468,171.850650226864));
#27970=CARTESIAN_POINT('Ctrl Pts',(-30.4073749369914,31.5016308502619,171.887693489937));
#27971=CARTESIAN_POINT('Ctrl Pts',(-30.2426929679812,32.0279006472769,171.924736753011));
#27972=CARTESIAN_POINT('Ctrl Pts',(-30.3646594566867,32.64386936431,171.961780016084));
#27973=CARTESIAN_POINT('Ctrl Pts',(-30.717463199212,33.0676730563981,171.998823279157));
#27974=CARTESIAN_POINT('Ctrl Pts',(-31.0702669417373,33.4914767484861,172.03586654223));
#27975=CARTESIAN_POINT('Ctrl Pts',(-31.6539079380824,33.7231154156292,172.072909805304));
#27976=CARTESIAN_POINT('Ctrl Pts',(-32.2013152329814,33.6565924597509,172.109953068377));
#27977=CARTESIAN_POINT('Ctrl Pts',(-32.7487225278803,33.5900695038727,172.14699633145));
#27978=CARTESIAN_POINT('Ctrl Pts',(-33.259896121333,33.2253849249731,172.184039594523));
#27979=CARTESIAN_POINT('Ctrl Pts',(-33.500925748699,32.7294164089369,172.221082857597));
#27980=CARTESIAN_POINT('Ctrl Pts',(-33.6102330021986,32.5044940336146,172.237882026195));
#27981=CARTESIAN_POINT('Ctrl Pts',(-33.6639815170623,32.2525713515443,172.254681194792));
#27982=CARTESIAN_POINT('Ctrl Pts',(-33.6634138707132,32.0004190115247,172.27148036339));
#27983=CARTESIAN_POINT('Origin',(-32.,32.,172.));
#27984=CARTESIAN_POINT('',(-33.6658030887413,31.9984781517552,172.97148036339));
#27985=CARTESIAN_POINT('',(-33.6687792891636,31.9999631491883,172.77851963661));
#27986=CARTESIAN_POINT('',(-33.666,32.,172.));
#27987=CARTESIAN_POINT('Ctrl Pts',(-33.668778895518,31.9999631544077,172.77851963661));
#27988=CARTESIAN_POINT('Ctrl Pts',(-33.6686001028313,32.5494261614689,172.741608875468));
#27989=CARTESIAN_POINT('Ctrl Pts',(-33.3706978019218,33.0990553069806,172.704698114326));
#27990=CARTESIAN_POINT('Ctrl Pts',(-32.9101517435485,33.3987316572276,172.667787353184));
#27991=CARTESIAN_POINT('Ctrl Pts',(-32.4479524209175,33.6994837830451,172.63074409011));
#27992=CARTESIAN_POINT('Ctrl Pts',(-31.8219395305894,33.74848533579,172.593700827037));
#27993=CARTESIAN_POINT('Ctrl Pts',(-31.3185731767646,33.5233134706259,172.556657563964));
#27994=CARTESIAN_POINT('Ctrl Pts',(-30.8152068229398,33.2981416054618,172.519614300891));
#27995=CARTESIAN_POINT('Ctrl Pts',(-30.4344870056185,32.7987963223888,172.482571037817));
#27996=CARTESIAN_POINT('Ctrl Pts',(-30.3506290488396,32.2537753153541,172.445527774744));
#27997=CARTESIAN_POINT('Ctrl Pts',(-30.2667710920606,31.7087543083194,172.408484511671));
#27998=CARTESIAN_POINT('Ctrl Pts',(-30.4797749958241,31.1180575773228,172.371441248598));
#27999=CARTESIAN_POINT('Ctrl Pts',(-30.8921713287334,30.7519847435489,172.334397985524));
#28000=CARTESIAN_POINT('Ctrl Pts',(-31.3045676616427,30.385911909775,172.297354722451));
#28001=CARTESIAN_POINT('Ctrl Pts',(-31.9163564236978,30.2444629732237,172.260311459378));
#28002=CARTESIAN_POINT('Ctrl Pts',(-32.4475863946687,30.3923642002859,172.223268196305));
#28003=CARTESIAN_POINT('Ctrl Pts',(-32.9788163656397,30.5402654273481,172.186224933231));
#28004=CARTESIAN_POINT('Ctrl Pts',(-33.4294875455265,30.9775168180239,172.149181670158));
#28005=CARTESIAN_POINT('Ctrl Pts',(-33.5933752460756,31.5040345068369,172.112138407085));
#28006=CARTESIAN_POINT('Ctrl Pts',(-33.6429542385954,31.6633156271879,172.10093215026));
#28007=CARTESIAN_POINT('Ctrl Pts',(-33.666287613298,31.8307661481971,172.089725893435));
#28008=CARTESIAN_POINT('Ctrl Pts',(-33.6649323100607,31.9985848365388,172.07851963661));
#28009=CARTESIAN_POINT('Ctrl Pts',(-33.6634138707132,32.0004190115247,172.27148036339));
#28010=CARTESIAN_POINT('Ctrl Pts',(-33.6627298198179,31.6965589863211,172.291724457866));
#28011=CARTESIAN_POINT('Ctrl Pts',(-33.5831688020356,31.3923654559128,172.311968552341));
#28012=CARTESIAN_POINT('Ctrl Pts',(-33.4269052960693,31.1346863708554,172.332212646816));
#28013=CARTESIAN_POINT('Ctrl Pts',(-33.1409695547944,30.6631773019829,172.36925590989));
#28014=CARTESIAN_POINT('Ctrl Pts',(-32.5982124109655,30.347411617411,172.406299172963));
#28015=CARTESIAN_POINT('Ctrl Pts',(-32.0469965906205,30.3318819822315,172.443342436036));
#28016=CARTESIAN_POINT('Ctrl Pts',(-31.4957807702756,30.316352347052,172.480385699109));
#28017=CARTESIAN_POINT('Ctrl Pts',(-30.9361062734147,30.6010587612649,172.517428962183));
#28018=CARTESIAN_POINT('Ctrl Pts',(-30.6240771150927,31.0557211134827,172.554472225256));
#28019=CARTESIAN_POINT('Ctrl Pts',(-30.3120479567707,31.5103834657005,172.591515488329));
#28020=CARTESIAN_POINT('Ctrl Pts',(-30.2476641369877,32.1350017559232,172.628558751402));
#28021=CARTESIAN_POINT('Ctrl Pts',(-30.4603873425697,32.6437540413965,172.665602014475));
#28022=CARTESIAN_POINT('Ctrl Pts',(-30.6731105481516,33.1525063268697,172.702645277549));
#28023=CARTESIAN_POINT('Ctrl Pts',(-31.1629407790985,33.5453926075936,172.739688540622));
#28024=CARTESIAN_POINT('Ctrl Pts',(-31.7057343777229,33.642630251846,172.776731803695));
#28025=CARTESIAN_POINT('Ctrl Pts',(-32.2485279763472,33.7398678960985,172.813775066769));
#28026=CARTESIAN_POINT('Ctrl Pts',(-32.844284942649,33.5414569038794,172.850818329842));
#28027=CARTESIAN_POINT('Ctrl Pts',(-33.2203901192063,33.1381890693894,172.887861592915));
#28028=CARTESIAN_POINT('Ctrl Pts',(-33.5033876183818,32.8347532334267,172.915734516407));
#28029=CARTESIAN_POINT('Ctrl Pts',(-33.6620249438784,32.4153336737998,172.943607439899));
#28030=CARTESIAN_POINT('Ctrl Pts',(-33.6658030887413,31.9984781517552,172.97148036339));
#28031=CARTESIAN_POINT('Origin',(-32.,32.,172.));
#28032=CARTESIAN_POINT('',(-33.6685842971392,32.0005168033655,173.67148036339));
#28033=CARTESIAN_POINT('',(-33.6650396791624,32.0014384974592,173.47851963661));
#28034=CARTESIAN_POINT('',(-33.666,32.,172.));
#28035=CARTESIAN_POINT('Ctrl Pts',(-33.6650396791624,32.0014384974592,173.47851963661));
#28036=CARTESIAN_POINT('Ctrl Pts',(-33.666391096427,32.1652619019991,173.467578383647));
#28037=CARTESIAN_POINT('Ctrl Pts',(-33.6441694407878,32.3287266927861,173.456637130684));
#28038=CARTESIAN_POINT('Ctrl Pts',(-33.5968738601931,32.4845826243756,173.445695877722));
#28039=CARTESIAN_POINT('Ctrl Pts',(-33.4367475346125,33.0122564013253,173.408652614648));
#28040=CARTESIAN_POINT('Ctrl Pts',(-32.9892080319931,33.4527126246025,173.371609351575));
#28041=CARTESIAN_POINT('Ctrl Pts',(-32.4590470020517,33.60440091471,173.334566088502));
#28042=CARTESIAN_POINT('Ctrl Pts',(-31.9288859721102,33.7560892048175,173.297522825429));
#28043=CARTESIAN_POINT('Ctrl Pts',(-31.3161034148467,33.6190095617553,173.260479562355));
#28044=CARTESIAN_POINT('Ctrl Pts',(-30.9011053057899,33.2558888869052,173.223436299282));
#28045=CARTESIAN_POINT('Ctrl Pts',(-30.4861071967331,32.8927682120551,173.186393036209));
#28046=CARTESIAN_POINT('Ctrl Pts',(-30.268893535883,32.3036065054172,173.149349773136));
#28047=CARTESIAN_POINT('Ctrl Pts',(-30.3488601166525,31.7580009693526,173.112306510063));
#28048=CARTESIAN_POINT('Ctrl Pts',(-30.4288266974221,31.212395433288,173.075263246989));
#28049=CARTESIAN_POINT('Ctrl Pts',(-30.8059735198113,30.7103460677967,173.038219983916));
#28050=CARTESIAN_POINT('Ctrl Pts',(-31.3077202428883,30.4815879402783,173.001176720843));
#28051=CARTESIAN_POINT('Ctrl Pts',(-31.8094669659654,30.2528298127598,172.96413345777));
#28052=CARTESIAN_POINT('Ctrl Pts',(-32.4358135897303,30.2973629232142,172.927090194696));
#28053=CARTESIAN_POINT('Ctrl Pts',(-32.9001472953714,30.5948091617682,172.890046931623));
#28054=CARTESIAN_POINT('Ctrl Pts',(-33.3644810010125,30.8922554003222,172.85300366855));
#28055=CARTESIAN_POINT('Ctrl Pts',(-33.6668017885297,31.4426147669758,172.815960405477));
#28056=CARTESIAN_POINT('Ctrl Pts',(-33.6687693048215,31.9940457997478,172.778917142403));
#28057=CARTESIAN_POINT('Ctrl Pts',(-33.6687763425305,31.9960182414464,172.778784640472));
#28058=CARTESIAN_POINT('Ctrl Pts',(-33.6687795373464,31.9979906968566,172.778652138541));
#28059=CARTESIAN_POINT('Ctrl Pts',(-33.668778895518,31.9999631544077,172.77851963661));
#28060=CARTESIAN_POINT('Ctrl Pts',(-33.6658030887413,31.9984781517552,172.97148036339));
#28061=CARTESIAN_POINT('Ctrl Pts',(-33.6670461184289,31.8613304752761,172.980650702972));
#28062=CARTESIAN_POINT('Ctrl Pts',(-33.6515264953894,31.7244603417323,172.989821042553));
#28063=CARTESIAN_POINT('Ctrl Pts',(-33.6181580581719,31.5920895937741,172.998991382135));
#28064=CARTESIAN_POINT('Ctrl Pts',(-33.4833674337676,31.0573826294095,173.036034645208));
#28065=CARTESIAN_POINT('Ctrl Pts',(-33.0573327981464,30.596093377441,173.073077908281));
#28066=CARTESIAN_POINT('Ctrl Pts',(-32.535005290492,30.4193052983326,173.110121171354));
#28067=CARTESIAN_POINT('Ctrl Pts',(-32.0126777828375,30.2425172192242,173.147164434428));
#28068=CARTESIAN_POINT('Ctrl Pts',(-31.3940574031498,30.3502303129759,173.184207697501));
#28069=CARTESIAN_POINT('Ctrl Pts',(-30.9622214828446,30.6931556519368,173.221250960574));
#28070=CARTESIAN_POINT('Ctrl Pts',(-30.5303855625394,31.0360809908978,173.258294223647));
#28071=CARTESIAN_POINT('Ctrl Pts',(-30.2853341016167,31.614218575068,173.295337486721));
#28072=CARTESIAN_POINT('Ctrl Pts',(-30.3392013198585,32.1630157807517,173.332380749794));
#28073=CARTESIAN_POINT('Ctrl Pts',(-30.3930685381003,32.7118129864354,173.369424012867));
#28074=CARTESIAN_POINT('Ctrl Pts',(-30.7458544355066,33.2312698136326,173.40646727594));
#28075=CARTESIAN_POINT('Ctrl Pts',(-31.2361260983262,33.4836856348551,173.443510539014));
#28076=CARTESIAN_POINT('Ctrl Pts',(-31.7263977611457,33.7361014560777,173.480553802087));
#28077=CARTESIAN_POINT('Ctrl Pts',(-32.3541551893786,33.7214762713257,173.51759706516));
#28078=CARTESIAN_POINT('Ctrl Pts',(-32.8321399877382,33.4465024858399,173.554640328233));
#28079=CARTESIAN_POINT('Ctrl Pts',(-33.3101247860979,33.171528700354,173.591683591307));
#28080=CARTESIAN_POINT('Ctrl Pts',(-33.6383369545844,32.6362063141344,173.62872685438));
#28081=CARTESIAN_POINT('Ctrl Pts',(-33.6665883845547,32.0854959484502,173.665770117453));
#28082=CARTESIAN_POINT('Ctrl Pts',(-33.6680400440452,32.0571984806852,173.667673532765));
#28083=CARTESIAN_POINT('Ctrl Pts',(-33.6686997256412,32.028860384471,173.669576948078));
#28084=CARTESIAN_POINT('Ctrl Pts',(-33.6685842971392,32.0005168033655,173.67148036339));
#28085=CARTESIAN_POINT('Origin',(-32.,32.,172.));
#28086=CARTESIAN_POINT('',(-33.6642813207824,32.0011936551981,174.37148036339));
#28087=CARTESIAN_POINT('',(-33.6637114105544,31.9991832659222,174.17851963661));
#28088=CARTESIAN_POINT('',(-33.666,32.,172.));
#28089=CARTESIAN_POINT('Ctrl Pts',(-33.6637114105544,31.9991832659222,174.17851963661));
#28090=CARTESIAN_POINT('Ctrl Pts',(-33.6622464012834,32.329476700965,174.156504628753));
#28091=CARTESIAN_POINT('Ctrl Pts',(-33.5671323371198,32.6605477978972,174.134489620897));
#28092=CARTESIAN_POINT('Ctrl Pts',(-33.3840345732138,32.9323490469583,174.11247461304));
#28093=CARTESIAN_POINT('Ctrl Pts',(-33.0759475318338,33.3896918395745,174.075431349967));
#28094=CARTESIAN_POINT('Ctrl Pts',(-32.5187551705316,33.6792258851286,174.038388086894));
#28095=CARTESIAN_POINT('Ctrl Pts',(-31.9674256925893,33.668461974308,174.00134482382));
#28096=CARTESIAN_POINT('Ctrl Pts',(-31.416096214647,33.6576980634873,173.964301560747));
#28097=CARTESIAN_POINT('Ctrl Pts',(-30.8706296200645,33.346636196292,173.927258297674));
#28098=CARTESIAN_POINT('Ctrl Pts',(-30.5806284648534,32.8776165964877,173.890215034601));
#28099=CARTESIAN_POINT('Ctrl Pts',(-30.2906273096424,32.4085969966835,173.853171771527));
#28100=CARTESIAN_POINT('Ctrl Pts',(-30.2560915938026,31.7816196642703,173.816128508454));
#28101=CARTESIAN_POINT('Ctrl Pts',(-30.4928246736404,31.2835860269176,173.779085245381));
#28102=CARTESIAN_POINT('Ctrl Pts',(-30.7295577534781,30.7855523895648,173.742041982308));
#28103=CARTESIAN_POINT('Ctrl Pts',(-31.2375596289934,30.4164624472723,173.704998719234));
#28104=CARTESIAN_POINT('Ctrl Pts',(-31.7843713964759,30.3452097563264,173.667955456161));
#28105=CARTESIAN_POINT('Ctrl Pts',(-32.3311831639583,30.2739570653805,173.630912193088));
#28106=CARTESIAN_POINT('Ctrl Pts',(-32.9168048234079,30.5005416257811,173.593868930015));
#28107=CARTESIAN_POINT('Ctrl Pts',(-33.2732590788618,30.9212795712924,173.556825666941));
#28108=CARTESIAN_POINT('Ctrl Pts',(-33.5244295160179,31.217746599208,173.530723656831));
#28109=CARTESIAN_POINT('Ctrl Pts',(-33.6618156693323,31.6106130429878,173.50462164672));
#28110=CARTESIAN_POINT('Ctrl Pts',(-33.6650396791624,32.0014384974592,173.47851963661));
#28111=CARTESIAN_POINT('Ctrl Pts',(-33.6685842971392,32.0005168033655,173.67148036339));
#28112=CARTESIAN_POINT('Ctrl Pts',(-33.6664533171258,31.4772525853206,173.706620211151));
#28113=CARTESIAN_POINT('Ctrl Pts',(-33.400144713866,30.9521189740352,173.741760058912));
#28114=CARTESIAN_POINT('Ctrl Pts',(-32.9757931652251,30.6462444462039,173.776899906673));
#28115=CARTESIAN_POINT('Ctrl Pts',(-32.5284558244712,30.3238016547903,173.813943169746));
#28116=CARTESIAN_POINT('Ctrl Pts',(-31.9054904515093,30.2450144171118,173.850986432819));
#28117=CARTESIAN_POINT('Ctrl Pts',(-31.3919626231178,30.4459353459241,173.888029695893));
#28118=CARTESIAN_POINT('Ctrl Pts',(-30.8784347947262,30.6468562747363,173.925072958966));
#28119=CARTESIAN_POINT('Ctrl Pts',(-30.4743445109049,31.1274853700393,173.962116222039));
#28120=CARTESIAN_POINT('Ctrl Pts',(-30.3646012944423,31.6678893639252,173.999159485112));
#28121=CARTESIAN_POINT('Ctrl Pts',(-30.2548580779796,32.208293357811,174.036202748185));
#28122=CARTESIAN_POINT('Ctrl Pts',(-30.4394619288755,32.8084722502797,174.073246011259));
#28123=CARTESIAN_POINT('Ctrl Pts',(-30.8339391259327,33.1937874344721,174.110289274332));
#28124=CARTESIAN_POINT('Ctrl Pts',(-31.22841632299,33.5791026186644,174.147332537405));
#28125=CARTESIAN_POINT('Ctrl Pts',(-31.8327668662085,33.7495540945805,174.184375800478));
#28126=CARTESIAN_POINT('Ctrl Pts',(-32.3704432239659,33.6271441910758,174.221419063552));
#28127=CARTESIAN_POINT('Ctrl Pts',(-32.9081195817234,33.504734287571,174.258462326625));
#28128=CARTESIAN_POINT('Ctrl Pts',(-33.3791217540197,33.0894630046454,174.295505589698));
#28129=CARTESIAN_POINT('Ctrl Pts',(-33.567921700715,32.5713562296509,174.332548852771));
#28130=CARTESIAN_POINT('Ctrl Pts',(-33.6340629863343,32.389850626572,174.345526022978));
#28131=CARTESIAN_POINT('Ctrl Pts',(-33.6655703268436,32.1957242910376,174.358503193184));
#28132=CARTESIAN_POINT('Ctrl Pts',(-33.6642813207824,32.0011936551981,174.37148036339));
#28133=CARTESIAN_POINT('Origin',(-32.,32.,172.));
#28134=CARTESIAN_POINT('',(-33.6642763188368,31.998808699364,175.07148036339));
#28135=CARTESIAN_POINT('',(-33.668020664445,31.9990039308852,174.87851963661));
#28136=CARTESIAN_POINT('',(-33.666,32.,172.));
#28137=CARTESIAN_POINT('Ctrl Pts',(-33.668020664445,31.9990039308852,174.87851963661));
#28138=CARTESIAN_POINT('Ctrl Pts',(-33.6645338936159,32.4921662157297,174.845430873859));
#28139=CARTESIAN_POINT('Ctrl Pts',(-33.4321105820849,32.9881841512697,174.812342111109));
#28140=CARTESIAN_POINT('Ctrl Pts',(-33.0490371398972,33.2978241500031,174.779253348358));
#28141=CARTESIAN_POINT('Ctrl Pts',(-32.6201818695343,33.6444698078531,174.742210085285));
#28142=CARTESIAN_POINT('Ctrl Pts',(-32.0025157577357,33.7575267199113,174.705166822212));
#28143=CARTESIAN_POINT('Ctrl Pts',(-31.4786794681056,33.5852606562456,174.668123559139));
#28144=CARTESIAN_POINT('Ctrl Pts',(-30.9548431784755,33.4129945925799,174.631080296066));
#28145=CARTESIAN_POINT('Ctrl Pts',(-30.5248367110139,32.9554055531903,174.594037032992));
#28146=CARTESIAN_POINT('Ctrl Pts',(-30.3854286936181,32.4218838013281,174.556993769919));
#28147=CARTESIAN_POINT('Ctrl Pts',(-30.2460206762223,31.888362049466,174.519950506846));
#28148=CARTESIAN_POINT('Ctrl Pts',(-30.3972111088923,31.2789075851313,174.482907243773));
#28149=CARTESIAN_POINT('Ctrl Pts',(-30.7698160694345,30.8724034665744,174.445863980699));
#28150=CARTESIAN_POINT('Ctrl Pts',(-31.1424210299766,30.4658993480176,174.408820717626));
#28151=CARTESIAN_POINT('Ctrl Pts',(-31.7364405183908,30.2623455752385,174.371777454553));
#28152=CARTESIAN_POINT('Ctrl Pts',(-32.2800544377153,30.3548872509366,174.334734191479));
#28153=CARTESIAN_POINT('Ctrl Pts',(-32.8236683570397,30.4474289266347,174.297690928406));
#28154=CARTESIAN_POINT('Ctrl Pts',(-33.3168767072744,30.8360660508099,174.260647665333));
#28155=CARTESIAN_POINT('Ctrl Pts',(-33.5339900216629,31.3429603827367,174.22360440226));
#28156=CARTESIAN_POINT('Ctrl Pts',(-33.6220717409518,31.5486047227887,174.208576147043));
#28157=CARTESIAN_POINT('Ctrl Pts',(-33.6647114798417,31.7737128018398,174.193547891827));
#28158=CARTESIAN_POINT('Ctrl Pts',(-33.6637114105544,31.9991832659222,174.17851963661));
#28159=CARTESIAN_POINT('Ctrl Pts',(-33.6642813207824,32.0011936551981,174.37148036339));
#28160=CARTESIAN_POINT('Ctrl Pts',(-33.6618908659233,31.640437629564,174.395546456257));
#28161=CARTESIAN_POINT('Ctrl Pts',(-33.5467088410307,31.2782911543542,174.419612549124));
#28162=CARTESIAN_POINT('Ctrl Pts',(-33.3304552403725,30.9926692429498,174.443678641991));
#28163=CARTESIAN_POINT('Ctrl Pts',(-32.9975911122403,30.5530312983066,174.480721905064));
#28164=CARTESIAN_POINT('Ctrl Pts',(-32.4252651348816,30.2946976760834,174.517765168138));
#28165=CARTESIAN_POINT('Ctrl Pts',(-31.8753705722274,30.3358804410539,174.554808431211));
#28166=CARTESIAN_POINT('Ctrl Pts',(-31.3254760095731,30.3770632060244,174.591851694284));
#28167=CARTESIAN_POINT('Ctrl Pts',(-30.7980128616233,30.7177623581885,174.628894957357));
#28168=CARTESIAN_POINT('Ctrl Pts',(-30.5343454048299,31.2020758128803,174.665938220431));
#28169=CARTESIAN_POINT('Ctrl Pts',(-30.2706779480365,31.686389267572,174.702981483504));
#28170=CARTESIAN_POINT('Ctrl Pts',(-30.2708061823995,32.3143170247913,174.740024746577));
#28171=CARTESIAN_POINT('Ctrl Pts',(-30.5346714285698,32.7985227476312,174.77706800965));
#28172=CARTESIAN_POINT('Ctrl Pts',(-30.7985366747401,33.282728470471,174.814111272724));
#28173=CARTESIAN_POINT('Ctrl Pts',(-31.3261389327177,33.6232121589313,174.851154535797));
#28174=CARTESIAN_POINT('Ctrl Pts',(-31.876050270056,33.6641703233686,174.88819779887));
#28175=CARTESIAN_POINT('Ctrl Pts',(-32.4259616073944,33.7051284878059,174.925241061943));
#28176=CARTESIAN_POINT('Ctrl Pts',(-32.9981820240936,33.4465611282202,174.962284325017));
#28177=CARTESIAN_POINT('Ctrl Pts',(-33.3308665602081,33.0067872663347,174.99932758809));
#28178=CARTESIAN_POINT('Ctrl Pts',(-33.5468672630685,32.7212571230455,175.02337851319));
#28179=CARTESIAN_POINT('Ctrl Pts',(-33.6618925440441,32.3593400811699,175.04742943829));
#28180=CARTESIAN_POINT('Ctrl Pts',(-33.6642763188368,31.998808699364,175.07148036339));
#28181=CARTESIAN_POINT('Origin',(-32.,32.,172.));
#28182=CARTESIAN_POINT('',(-33.6685813165324,31.9994792732742,175.77148036339));
#28183=CARTESIAN_POINT('',(-33.6667309775204,32.001451384792,175.57851963661));
#28184=CARTESIAN_POINT('',(-33.666,32.,172.));
#28185=CARTESIAN_POINT('Ctrl Pts',(-33.6667309775204,32.001451384792,175.57851963661));
#28186=CARTESIAN_POINT('Ctrl Pts',(-33.6677032442523,32.1077720165447,175.571400382039));
#28187=CARTESIAN_POINT('Ctrl Pts',(-33.6584012903311,32.2139231749333,175.564281127468));
#28188=CARTESIAN_POINT('Ctrl Pts',(-33.638208635078,32.3179605528532,175.557161872896));
#28189=CARTESIAN_POINT('Ctrl Pts',(-33.5331411967364,32.859293064739,175.520118609823));
#28190=CARTESIAN_POINT('Ctrl Pts',(-33.1332209461614,33.3433974793115,175.48307534675));
#28191=CARTESIAN_POINT('Ctrl Pts',(-32.6214492215387,33.5487502414089,175.446032083677));
#28192=CARTESIAN_POINT('Ctrl Pts',(-32.1096774969161,33.7541030035063,175.408988820604));
#28193=CARTESIAN_POINT('Ctrl Pts',(-31.4860542982457,33.6807041131287,175.37194555753));
#28194=CARTESIAN_POINT('Ctrl Pts',(-31.0359462197833,33.362140504524,175.334902294457));
#28195=CARTESIAN_POINT('Ctrl Pts',(-30.5858381413209,33.0435768959193,175.297859031384));
#28196=CARTESIAN_POINT('Ctrl Pts',(-30.3092451830665,32.4798485690876,175.26081576831));
#28197=CARTESIAN_POINT('Ctrl Pts',(-30.3327347829544,31.9289145496975,175.223772505237));
#28198=CARTESIAN_POINT('Ctrl Pts',(-30.3562243828422,31.3779805303073,175.186729242164));
#28199=CARTESIAN_POINT('Ctrl Pts',(-30.6797965408723,30.8398408183586,175.149685979091));
#28200=CARTESIAN_POINT('Ctrl Pts',(-31.1553863920272,30.5607452280982,175.112642716018));
#28201=CARTESIAN_POINT('Ctrl Pts',(-31.630976243182,30.2816496378377,175.075599452944));
#28202=CARTESIAN_POINT('Ctrl Pts',(-32.2585837874615,30.2615981692654,175.038556189871));
#28203=CARTESIAN_POINT('Ctrl Pts',(-32.7510192156636,30.5097662656754,175.001512926798));
#28204=CARTESIAN_POINT('Ctrl Pts',(-33.2434546438656,30.7579343620854,174.964469663725));
#28205=CARTESIAN_POINT('Ctrl Pts',(-33.6007179559903,31.2743220234776,174.927426400651));
#28206=CARTESIAN_POINT('Ctrl Pts',(-33.6593273975889,31.8226330559946,174.890383137578));
#28207=CARTESIAN_POINT('Ctrl Pts',(-33.6655841643122,31.8811672124153,174.886428637255));
#28208=CARTESIAN_POINT('Ctrl Pts',(-33.6684373749903,31.9400651778922,174.882474136933));
#28209=CARTESIAN_POINT('Ctrl Pts',(-33.668020664445,31.9990039308852,174.87851963661));
#28210=CARTESIAN_POINT('Ctrl Pts',(-33.6642763188368,31.998808699364,175.07148036339));
#28211=CARTESIAN_POINT('Ctrl Pts',(-33.6655640367782,31.8040492236754,175.084472701363));
#28212=CARTESIAN_POINT('Ctrl Pts',(-33.6339810135813,31.6096941075785,175.097465039336));
#28213=CARTESIAN_POINT('Ctrl Pts',(-33.5676882071046,31.4280034213046,175.11045737731));
#28214=CARTESIAN_POINT('Ctrl Pts',(-33.3786766623567,30.909973802345,175.147500640383));
#28215=CARTESIAN_POINT('Ctrl Pts',(-32.9075049173313,30.494894928611,175.184543903456));
#28216=CARTESIAN_POINT('Ctrl Pts',(-32.3697786077296,30.3727046420518,175.221587166529));
#28217=CARTESIAN_POINT('Ctrl Pts',(-31.8320522981278,30.2505143554927,175.258630429603));
#28218=CARTESIAN_POINT('Ctrl Pts',(-31.2277714239497,30.4212126561084,175.295673692676));
#28219=CARTESIAN_POINT('Ctrl Pts',(-30.8334516366425,30.80668892711,175.332716955749));
#28220=CARTESIAN_POINT('Ctrl Pts',(-30.4391318493354,31.1921651981116,175.369760218822));
#28221=CARTESIAN_POINT('Ctrl Pts',(-30.2547731488991,31.7924194394991,175.406803481895));
#28222=CARTESIAN_POINT('Ctrl Pts',(-30.36473707701,32.3327785651572,175.443846744969));
#28223=CARTESIAN_POINT('Ctrl Pts',(-30.4747010051209,32.8731376908152,175.480890008042));
#28224=CARTESIAN_POINT('Ctrl Pts',(-30.878987561779,33.3536017007438,175.517933271115));
#28225=CARTESIAN_POINT('Ctrl Pts',(-31.39259741081,33.5543128692062,175.554976534188));
#28226=CARTESIAN_POINT('Ctrl Pts',(-31.906207259841,33.7550240376686,175.592019797262));
#28227=CARTESIAN_POINT('Ctrl Pts',(-32.5291404012448,33.6759823646648,175.629063060335));
#28228=CARTESIAN_POINT('Ctrl Pts',(-32.9763460072298,33.3533568911779,175.666106323408));
#28229=CARTESIAN_POINT('Ctrl Pts',(-33.4003894769072,33.0474411706394,175.701231003402));
#28230=CARTESIAN_POINT('Ctrl Pts',(-33.6664369441154,32.5225201209083,175.736355683396));
#28231=CARTESIAN_POINT('Ctrl Pts',(-33.6685813165324,31.9994792732742,175.77148036339));
#28232=CARTESIAN_POINT('Origin',(-32.,32.,172.));
#28233=CARTESIAN_POINT('',(-33.665809879668,32.0015219961349,176.47148036339));
#28234=CARTESIAN_POINT('',(-33.6633199598622,32.0000809155407,176.27851963661));
#28235=CARTESIAN_POINT('',(-33.666,32.,172.));
#28236=CARTESIAN_POINT('Ctrl Pts',(-33.6633199598622,32.0000809155407,176.27851963661));
#28237=CARTESIAN_POINT('Ctrl Pts',(-33.6634382983753,32.2731930234702,176.260326627145));
#28238=CARTESIAN_POINT('Ctrl Pts',(-33.599931290633,32.5462533007021,176.24213361768));
#28239=CARTESIAN_POINT('Ctrl Pts',(-33.472497725772,32.7852241035491,176.223940608215));
#28240=CARTESIAN_POINT('Ctrl Pts',(-33.2130269066871,33.2717988142213,176.186897345141));
#28241=CARTESIAN_POINT('Ctrl Pts',(-32.6885287363003,33.6170450456087,176.149854082068));
#28242=CARTESIAN_POINT('Ctrl Pts',(-32.1390107333948,33.6629799942341,176.112810818995));
#28243=CARTESIAN_POINT('Ctrl Pts',(-31.5894927304893,33.7089149428595,176.075767555922));
#28244=CARTESIAN_POINT('Ctrl Pts',(-31.0149548950651,33.4555386087229,176.038724292849));
#28245=CARTESIAN_POINT('Ctrl Pts',(-30.6783026253169,33.0187946284562,176.001681029775));
#28246=CARTESIAN_POINT('Ctrl Pts',(-30.3416503555688,32.5820506481895,175.964637766702));
#28247=CARTESIAN_POINT('Ctrl Pts',(-30.2428836514968,31.9619390217927,175.927594503629));
#28248=CARTESIAN_POINT('Ctrl Pts',(-30.4271976213409,31.4422194670863,175.890551240556));
#28249=CARTESIAN_POINT('Ctrl Pts',(-30.6115115911851,30.9224999123798,175.853507977482));
#28250=CARTESIAN_POINT('Ctrl Pts',(-31.0789062349454,30.5031724293638,175.816464714409));
#28251=CARTESIAN_POINT('Ctrl Pts',(-31.6155042979806,30.3761190005593,175.779421451336));
#28252=CARTESIAN_POINT('Ctrl Pts',(-32.1521023610158,30.2490655717549,175.742378188263));
#28253=CARTESIAN_POINT('Ctrl Pts',(-32.757903843326,30.414286197162,175.705334925189));
#28254=CARTESIAN_POINT('Ctrl Pts',(-33.1556972714269,30.7961768144651,175.668291662116));
#28255=CARTESIAN_POINT('Ctrl Pts',(-33.4770397487634,31.1046728035055,175.638367653614));
#28256=CARTESIAN_POINT('Ctrl Pts',(-33.6626442971441,31.5545591635997,175.608443645112));
#28257=CARTESIAN_POINT('Ctrl Pts',(-33.6667309775204,32.001451384792,175.57851963661));
#28258=CARTESIAN_POINT('Ctrl Pts',(-33.6685813165324,31.9994792732742,175.77148036339));
#28259=CARTESIAN_POINT('Ctrl Pts',(-33.668698446614,31.9709096942721,175.773398946469));
#28260=CARTESIAN_POINT('Ctrl Pts',(-33.6680282029118,31.9423457249876,175.775317529549));
#28261=CARTESIAN_POINT('Ctrl Pts',(-33.6665533258647,31.9138233628901,175.777236112628));
#28262=CARTESIAN_POINT('Ctrl Pts',(-33.6380769679487,31.3631245820592,175.814279375701));
#28263=CARTESIAN_POINT('Ctrl Pts',(-33.3096461815507,30.8279362943673,175.851322638774));
#28264=CARTESIAN_POINT('Ctrl Pts',(-32.8315491136859,30.553157758334,175.888365901848));
#28265=CARTESIAN_POINT('Ctrl Pts',(-32.3534520458211,30.2783792223007,175.925409164921));
#28266=CARTESIAN_POINT('Ctrl Pts',(-31.7256886964896,30.264010437926,175.962452427994));
#28267=CARTESIAN_POINT('Ctrl Pts',(-31.2355201704377,30.5166264830092,175.999495691067));
#28268=CARTESIAN_POINT('Ctrl Pts',(-30.7453516443858,30.7692425280923,176.036538954141));
#28269=CARTESIAN_POINT('Ctrl Pts',(-30.3927779416135,31.2888434026335,176.073582217214));
#28270=CARTESIAN_POINT('Ctrl Pts',(-30.3391348767637,31.8376625638996,176.110625480287));
#28271=CARTESIAN_POINT('Ctrl Pts',(-30.2854918119139,32.3864817251657,176.14766874336));
#28272=CARTESIAN_POINT('Ctrl Pts',(-30.5307793849866,32.9645191731569,176.184712006434));
#28273=CARTESIAN_POINT('Ctrl Pts',(-30.9627553325488,33.3072681058711,176.221755269507));
#28274=CARTESIAN_POINT('Ctrl Pts',(-31.3947312801111,33.6500170385854,176.25879853258));
#28275=CARTESIAN_POINT('Ctrl Pts',(-32.0133956021629,33.7574774560227,176.295841795653));
#28276=CARTESIAN_POINT('Ctrl Pts',(-32.535650859524,33.5804760540039,176.332885058727));
#28277=CARTESIAN_POINT('Ctrl Pts',(-33.0579061168852,33.4034746519851,176.3699283218));
#28278=CARTESIAN_POINT('Ctrl Pts',(-33.4837523095557,32.9420114305103,176.406971584873));
#28279=CARTESIAN_POINT('Ctrl Pts',(-33.6183245287774,32.4072494572197,176.444014847946));
#28280=CARTESIAN_POINT('Ctrl Pts',(-33.6515837960838,32.2750840554909,176.453170019761));
#28281=CARTESIAN_POINT('Ctrl Pts',(-33.6670514141996,32.1384414062313,176.462325191576));
#28282=CARTESIAN_POINT('Ctrl Pts',(-33.665809879668,32.0015219961349,176.47148036339));
#28283=CARTESIAN_POINT('Origin',(-32.,32.,172.));
#28284=CARTESIAN_POINT('',(-33.6634121676067,31.9995845740168,177.17148036339));
#28285=CARTESIAN_POINT('',(-33.6664340315428,31.9985061125431,176.97851963661));
#28286=CARTESIAN_POINT('',(-33.666,32.,172.));
#28287=CARTESIAN_POINT('Ctrl Pts',(-33.6664340315428,31.9985061125431,176.97851963661));
#28288=CARTESIAN_POINT('Ctrl Pts',(-33.662398201977,32.435783313381,176.949252872251));
#28289=CARTESIAN_POINT('Ctrl Pts',(-33.4857164328592,32.875946937287,176.919986107892));
#28290=CARTESIAN_POINT('Ctrl Pts',(-33.1768207039935,33.1831819279473,176.890719343533));
#28291=CARTESIAN_POINT('Ctrl Pts',(-32.785848008609,33.5720526088596,176.85367608046));
#28292=CARTESIAN_POINT('Ctrl Pts',(-32.183065360919,33.747968413286,176.816632817387));
#28293=CARTESIAN_POINT('Ctrl Pts',(-31.6443028311243,33.6304312219835,176.779589554314));
#28294=CARTESIAN_POINT('Ctrl Pts',(-31.1055403013296,33.512894030681,176.74254629124));
#28295=CARTESIAN_POINT('Ctrl Pts',(-30.6307978894302,33.1019038436494,176.705503028167));
#28296=CARTESIAN_POINT('Ctrl Pts',(-30.4373151493842,32.5855275424649,176.668459765094));
#28297=CARTESIAN_POINT('Ctrl Pts',(-30.2438324093381,32.0691512412803,176.63141650202));
#28298=CARTESIAN_POINT('Ctrl Pts',(-30.3316093411455,31.4473888259428,176.594373238947));
#28299=CARTESIAN_POINT('Ctrl Pts',(-30.6604796965375,31.0047554061028,176.557329975874));
#28300=CARTESIAN_POINT('Ctrl Pts',(-30.9893500519296,30.5621219862628,176.520286712801));
#28301=CARTESIAN_POINT('Ctrl Pts',(-31.5593138309064,30.2986175619204,176.483243449727));
#28302=CARTESIAN_POINT('Ctrl Pts',(-32.1095586988182,30.3348203289801,176.446200186654));
#28303=CARTESIAN_POINT('Ctrl Pts',(-32.65980356673,30.3710230960397,176.409156923581));
#28304=CARTESIAN_POINT('Ctrl Pts',(-33.1903295235767,30.7069330545014,176.372113660508));
#28305=CARTESIAN_POINT('Ctrl Pts',(-33.4583707681085,31.1888396287107,176.335070397435));
#28306=CARTESIAN_POINT('Ctrl Pts',(-33.594769265911,31.4340680558438,176.316220143826));
#28307=CARTESIAN_POINT('Ctrl Pts',(-33.6631973462292,31.7171023073089,176.297369890218));
#28308=CARTESIAN_POINT('Ctrl Pts',(-33.6633199598622,32.0000809155407,176.27851963661));
#28309=CARTESIAN_POINT('Ctrl Pts',(-33.665809879668,32.0015219961349,176.47148036339));
#28310=CARTESIAN_POINT('Ctrl Pts',(-33.6620279704892,31.5844439684211,176.499368454649));
#28311=CARTESIAN_POINT('Ctrl Pts',(-33.5032006168982,31.1647978567452,176.527256545907));
#28312=CARTESIAN_POINT('Ctrl Pts',(-33.2199251392459,30.8613125733022,176.555144637166));
#28313=CARTESIAN_POINT('Ctrl Pts',(-32.8436552847201,30.4581983877814,176.592187900239));
#28314=CARTESIAN_POINT('Ctrl Pts',(-32.2478173298955,30.2600307418458,176.629231163313));
#28315=CARTESIAN_POINT('Ctrl Pts',(-31.7050634919084,30.3574900744037,176.666274426386));
#28316=CARTESIAN_POINT('Ctrl Pts',(-31.1623096539213,30.4549494069617,176.703317689459));
#28317=CARTESIAN_POINT('Ctrl Pts',(-30.6726399327717,30.8480357180132,176.740360952532));
#28318=CARTESIAN_POINT('Ctrl Pts',(-30.4601245381307,31.3568748457966,176.777404215605));
#28319=CARTESIAN_POINT('Ctrl Pts',(-30.2476091434896,31.86571397358,176.814447478679));
#28320=CARTESIAN_POINT('Ctrl Pts',(-30.3122480753572,32.4903059180951,176.851490741752));
#28321=CARTESIAN_POINT('Ctrl Pts',(-30.6244629081934,32.9448407866344,176.888534004825));
#28322=CARTESIAN_POINT('Ctrl Pts',(-30.9366777410296,33.3993756551737,176.925577267898));
#28323=CARTESIAN_POINT('Ctrl Pts',(-31.4964684748346,33.6838534477371,176.962620530972));
#28324=CARTESIAN_POINT('Ctrl Pts',(-32.0476779068016,33.6680986803785,176.999663794045));
#28325=CARTESIAN_POINT('Ctrl Pts',(-32.5988873387685,33.6523439130199,177.036707057118));
#28326=CARTESIAN_POINT('Ctrl Pts',(-33.1415154688975,33.3363565857395,177.073750320191));
#28327=CARTESIAN_POINT('Ctrl Pts',(-33.4272586037737,32.8647307628914,177.110793583265));
#28328=CARTESIAN_POINT('Ctrl Pts',(-33.5832998499633,32.6071809842615,177.131022509973));
#28329=CARTESIAN_POINT('Ctrl Pts',(-33.6627345384754,32.3032177147393,177.151251436682));
#28330=CARTESIAN_POINT('Ctrl Pts',(-33.6634121676067,31.9995845740168,177.17148036339));
#28331=CARTESIAN_POINT('Origin',(-32.,32.,172.));
#28332=CARTESIAN_POINT('',(-33.6673324606655,31.9986966424362,177.87148036339));
#28333=CARTESIAN_POINT('',(-33.6682332709748,32.0008552724336,177.67851963661));
#28334=CARTESIAN_POINT('',(-33.666,32.,172.));
#28335=CARTESIAN_POINT('Ctrl Pts',(-33.6682332709748,32.0008552724336,177.67851963661));
#28336=CARTESIAN_POINT('Ctrl Pts',(-33.6685408240927,32.049981824342,177.67522238043));
#28337=CARTESIAN_POINT('Ctrl Pts',(-33.6665588175026,32.0990832102901,177.671925124251));
#28338=CARTESIAN_POINT('Ctrl Pts',(-33.6622064848019,32.1479735833227,177.668627868071));
#28339=CARTESIAN_POINT('Ctrl Pts',(-33.613309888227,32.6972360159009,177.631584604998));
#28340=CARTESIAN_POINT('Ctrl Pts',(-33.2652411222702,33.2198653234349,177.594541341925));
#28341=CARTESIAN_POINT('Ctrl Pts',(-32.7772747016725,33.4767093138507,177.557498078852));
#28342=CARTESIAN_POINT('Ctrl Pts',(-32.2893082810747,33.7335533042664,177.520454815778));
#28343=CARTESIAN_POINT('Ctrl Pts',(-31.6614442058359,33.7246119775639,177.483411552705));
#28344=CARTESIAN_POINT('Ctrl Pts',(-31.1809896061435,33.4539767650361,177.446368289632));
#28345=CARTESIAN_POINT('Ctrl Pts',(-30.700535006451,33.1833415525083,177.409325026559));
#28346=CARTESIAN_POINT('Ctrl Pts',(-30.3674898823049,32.6510124541552,177.372281763485));
#28347=CARTESIAN_POINT('Ctrl Pts',(-30.3342539091629,32.1005804139805,177.335238500412));
#28348=CARTESIAN_POINT('Ctrl Pts',(-30.3010179360208,31.5501483738058,177.298195237339));
#28349=CARTESIAN_POINT('Ctrl Pts',(-30.5675911138828,30.9816133918094,177.261151974266));
#28350=CARTESIAN_POINT('Ctrl Pts',(-31.0119909860241,30.6551339757941,177.224108711192));
#28351=CARTESIAN_POINT('Ctrl Pts',(-31.4563908581654,30.3286545597788,177.187065448119));
#28352=CARTESIAN_POINT('Ctrl Pts',(-32.0786174245861,30.2442307097446,177.150022185046));
#28353=CARTESIAN_POINT('Ctrl Pts',(-32.593943190218,30.4404943301489,177.112978921973));
#28354=CARTESIAN_POINT('Ctrl Pts',(-33.1092689558498,30.6367579505533,177.075935658899));
#28355=CARTESIAN_POINT('Ctrl Pts',(-33.5176939206928,31.1137090413961,177.038892395826));
#28356=CARTESIAN_POINT('Ctrl Pts',(-33.6323250315748,31.6530973655166,177.001849132753));
#28357=CARTESIAN_POINT('Ctrl Pts',(-33.6563895607886,31.766331251008,176.994072634039));
#28358=CARTESIAN_POINT('Ctrl Pts',(-33.6675063955064,31.8823167877364,176.986296135324));
#28359=CARTESIAN_POINT('Ctrl Pts',(-33.6664340315428,31.9985061125431,176.97851963661));
#28360=CARTESIAN_POINT('Ctrl Pts',(-33.6634121676067,31.9995845740168,177.17148036339));
#28361=CARTESIAN_POINT('Ctrl Pts',(-33.6639754146988,31.7472039196625,177.188294699755));
#28362=CARTESIAN_POINT('Ctrl Pts',(-33.6101255864195,31.4950513505542,177.20510903612));
#28363=CARTESIAN_POINT('Ctrl Pts',(-33.500627701242,31.2699706058666,177.221923372484));
#28364=CARTESIAN_POINT('Ctrl Pts',(-33.2593955242106,30.7741005901055,177.258966635558));
#28365=CARTESIAN_POINT('Ctrl Pts',(-32.7480730305246,30.4096248769989,177.296009898631));
#28366=CARTESIAN_POINT('Ctrl Pts',(-32.2006386068928,30.3433254802472,177.333053161704));
#28367=CARTESIAN_POINT('Ctrl Pts',(-31.6532041832609,30.2770260834956,177.370096424777));
#28368=CARTESIAN_POINT('Ctrl Pts',(-31.0696578296832,30.5089030030988,177.407139687851));
#28369=CARTESIAN_POINT('Ctrl Pts',(-30.7170272216495,30.9328508140707,177.444182950924));
#28370=CARTESIAN_POINT('Ctrl Pts',(-30.3643966136158,31.3567986250425,177.481226213997));
#28371=CARTESIAN_POINT('Ctrl Pts',(-30.2426817511261,31.972817327383,177.51826947707));
#28372=CARTESIAN_POINT('Ctrl Pts',(-30.4075786377867,32.4990197038229,177.555312740144));
#28373=CARTESIAN_POINT('Ctrl Pts',(-30.5724755244473,33.0252220802628,177.592356003217));
#28374=CARTESIAN_POINT('Ctrl Pts',(-31.0239841602582,33.4616081308021,177.62939926629));
#28375=CARTESIAN_POINT('Ctrl Pts',(-31.5554967587389,33.608490777879,177.666442529363));
#28376=CARTESIAN_POINT('Ctrl Pts',(-32.0870093572195,33.7553734249558,177.703485792437));
#28377=CARTESIAN_POINT('Ctrl Pts',(-32.6985259183698,33.6127526685702,177.74052905551));
#28378=CARTESIAN_POINT('Ctrl Pts',(-33.1102195412827,33.2458893383607,177.777572318583));
#28379=CARTESIAN_POINT('Ctrl Pts',(-33.4581131480177,32.9358786896109,177.808875000185));
#28380=CARTESIAN_POINT('Ctrl Pts',(-33.663317931488,32.4657417347074,177.840177681788));
#28381=CARTESIAN_POINT('Ctrl Pts',(-33.6673324606655,31.9986966424362,177.87148036339));
#28382=CARTESIAN_POINT('Origin',(-32.,32.,172.));
#28383=CARTESIAN_POINT('',(-33.6674973548511,32.0012179185931,178.57148036339));
#28384=CARTESIAN_POINT('',(-33.6638666530066,32.0009462971081,178.37851963661));
#28385=CARTESIAN_POINT('',(-33.666,32.,172.));
#28386=CARTESIAN_POINT('',(-30.7309291201471,33.0793586530479,179.));
#28387=CARTESIAN_POINT('Ctrl Pts',(-33.6674973548511,32.0012179185931,178.57148036339));
#28388=CARTESIAN_POINT('Ctrl Pts',(-33.6635706604874,31.5283160997714,178.60319045304));
#28389=CARTESIAN_POINT('Ctrl Pts',(-33.4523668182224,31.0524200665679,178.634900542691));
#28390=CARTESIAN_POINT('Ctrl Pts',(-33.0965044878972,30.7421391403554,178.666610632341));
#28391=CARTESIAN_POINT('Ctrl Pts',(-32.6807913169313,30.3796734991954,178.703653895414));
#28392=CARTESIAN_POINT('Ctrl Pts',(-32.067668916338,30.2432156860183,178.740697158487));
#28393=CARTESIAN_POINT('Ctrl Pts',(-31.5378405764127,30.3962148457825,178.777740421561));
#28394=CARTESIAN_POINT('Ctrl Pts',(-31.0080122364874,30.5492140055468,178.814783684634));
#28395=CARTESIAN_POINT('Ctrl Pts',(-30.5614779572301,30.9916701382525,178.851826947707));
#28396=CARTESIAN_POINT('Ctrl Pts',(-30.402485611048,31.5187149254341,178.88887021078));
#28397=CARTESIAN_POINT('Ctrl Pts',(-30.243493264866,32.0457597126157,178.925913473853));
#28398=CARTESIAN_POINT('Ctrl Pts',(-30.3720428517591,32.6573931542732,178.962956736927));
#28399=CARTESIAN_POINT('Ctrl Pts',(-30.7309291201472,33.079358653048,179.));
#28400=CARTESIAN_POINT('',(-33.2714881269984,33.0811958775516,179.));
#28401=CARTESIAN_POINT('Origin',(-32.,32.,179.));
#28402=CARTESIAN_POINT('Ctrl Pts',(-33.2714899453064,33.0811972595532,179.));
#28403=CARTESIAN_POINT('Ctrl Pts',(-32.9207087126724,33.49260263365,178.963685183163));
#28404=CARTESIAN_POINT('Ctrl Pts',(-32.3509044879416,33.7187060857981,178.927370366326));
#28405=CARTESIAN_POINT('Ctrl Pts',(-31.8135987875986,33.6582492875696,178.891055549488));
#28406=CARTESIAN_POINT('Ctrl Pts',(-31.2655151638324,33.5965797742307,178.854012286415));
#28407=CARTESIAN_POINT('Ctrl Pts',(-30.7512469298483,33.2367383670875,178.816969023342));
#28408=CARTESIAN_POINT('Ctrl Pts',(-30.5057843969245,32.7430232880388,178.779925760268));
#28409=CARTESIAN_POINT('Ctrl Pts',(-30.2603218640006,32.2493082089901,178.742882497195));
#28410=CARTESIAN_POINT('Ctrl Pts',(-30.283665032137,31.6217194580359,178.705839234122));
#28411=CARTESIAN_POINT('Ctrl Pts',(-30.5652971510249,31.147616030279,178.668795971049));
#28412=CARTESIAN_POINT('Ctrl Pts',(-30.8469292699128,30.673512602522,178.631752707976));
#28413=CARTESIAN_POINT('Ctrl Pts',(-31.3868503395524,30.3528944979624,178.594709444902));
#28414=CARTESIAN_POINT('Ctrl Pts',(-31.9379143943192,30.3323875246469,178.557666181829));
#28415=CARTESIAN_POINT('Ctrl Pts',(-32.488978449086,30.3118805513313,178.520622918756));
#28416=CARTESIAN_POINT('Ctrl Pts',(-33.05118548898,30.5914847092598,178.483579655683));
#28417=CARTESIAN_POINT('Ctrl Pts',(-33.3673124104994,31.0432975272097,178.44653639261));
#28418=CARTESIAN_POINT('Ctrl Pts',(-33.5607972342972,31.3198286212731,178.42386414061));
#28419=CARTESIAN_POINT('Ctrl Pts',(-33.6620997929986,31.6608695361818,178.40119188861));
#28420=CARTESIAN_POINT('Ctrl Pts',(-33.6638666530066,32.0009462971081,178.37851963661));
#28421=CARTESIAN_POINT('Origin',(-32.,32.,180.545925280538));
#28422=CARTESIAN_POINT('',(-34.0533144349913,32.0018139164182,166.254074719462));
#28423=CARTESIAN_POINT('',(-34.0546693143771,31.9981396895887,166.195925280538));
#28424=CARTESIAN_POINT('',(-34.05475,32.0000000000002,180.545925280538));
#28425=CARTESIAN_POINT('',(-31.6163320011528,34.0186125009919,166.));
#28426=CARTESIAN_POINT('Ctrl Pts',(-34.0546693143771,31.9981396895887,166.195925280538));
#28427=CARTESIAN_POINT('Ctrl Pts',(-34.0494207118803,32.5195349242374,166.167660116765));
#28428=CARTESIAN_POINT('Ctrl Pts',(-33.5818272109704,33.7318555427796,166.102351689919));
#28429=CARTESIAN_POINT('Ctrl Pts',(-32.2875197530244,34.146181938655,166.037043263073));
#28430=CARTESIAN_POINT('Ctrl Pts',(-31.6163320011528,34.0186125009919,166.));
#28431=CARTESIAN_POINT('',(-30.6584058692254,33.5612502425942,166.));
#28432=CARTESIAN_POINT('Origin',(-32.,32.,166.));
#28433=CARTESIAN_POINT('Ctrl Pts',(-34.0533144349913,32.0018139164182,166.254074719462));
#28434=CARTESIAN_POINT('Ctrl Pts',(-34.0549811521398,32.2111665085478,166.242741226219));
#28435=CARTESIAN_POINT('Ctrl Pts',(-33.9292853981704,33.1027772342694,166.194364469902));
#28436=CARTESIAN_POINT('Ctrl Pts',(-32.6547057991862,34.3307279683718,166.109672896748));
#28437=CARTESIAN_POINT('Ctrl Pts',(-31.1647193509792,33.9951595187684,166.036314816837));
#28438=CARTESIAN_POINT('Ctrl Pts',(-30.6584039191552,33.5612522752606,166.));
#28439=CARTESIAN_POINT('Origin',(-32.,32.,180.545925280538));
#28440=CARTESIAN_POINT('',(-34.0520397258479,31.9988941582834,166.954074719462));
#28441=CARTESIAN_POINT('',(-34.0578396023064,32.0007586512867,166.895925280538));
#28442=CARTESIAN_POINT('',(-34.05475,32.0000000000002,180.545925280538));
#28443=CARTESIAN_POINT('Ctrl Pts',(-34.0578396023064,32.0007586512867,166.895925280538));
#28444=CARTESIAN_POINT('Ctrl Pts',(-34.0580398859891,32.0429254328027,166.893629624944));
#28445=CARTESIAN_POINT('Ctrl Pts',(-34.0377495998064,32.7653095502187,166.854290706278));
#28446=CARTESIAN_POINT('Ctrl Pts',(-33.1886966129007,34.1178213986476,166.777908524538));
#28447=CARTESIAN_POINT('Ctrl Pts',(-30.8656448664525,34.1473555806342,166.666778735318));
#28448=CARTESIAN_POINT('Ctrl Pts',(-29.580472395857,32.2117592705426,166.555648946099));
#28449=CARTESIAN_POINT('Ctrl Pts',(-30.5101755690543,30.0821472363061,166.444519156879));
#28450=CARTESIAN_POINT('Ctrl Pts',(-32.8022294248721,29.7081731264144,166.333389367659));
#28451=CARTESIAN_POINT('Ctrl Pts',(-33.9655640366591,30.9926240191872,166.250524742212));
#28452=CARTESIAN_POINT('Ctrl Pts',(-34.0562993333743,31.8362138935308,166.204703379838));
#28453=CARTESIAN_POINT('Ctrl Pts',(-34.0546693143771,31.9981396895887,166.195925280538));
#28454=CARTESIAN_POINT('Ctrl Pts',(-34.0520397258479,31.9988941582834,166.954074719462));
#28455=CARTESIAN_POINT('Ctrl Pts',(-34.0500128717713,32.413460949173,166.931667471325));
#28456=CARTESIAN_POINT('Ctrl Pts',(-33.7267813329344,33.5162878439086,166.872216960114));
#28457=CARTESIAN_POINT('Ctrl Pts',(-31.9269554489549,34.4275128925295,166.77572318583));
#28458=CARTESIAN_POINT('Ctrl Pts',(-29.9209653652486,33.2553461090702,166.66459339661));
#28459=CARTESIAN_POINT('Ctrl Pts',(-29.8177243014505,30.9342420640658,166.553463607391));
#28460=CARTESIAN_POINT('Ctrl Pts',(-31.7115987485412,29.5886264481624,166.442333818171));
#28461=CARTESIAN_POINT('Ctrl Pts',(-33.6494969660935,30.3618237184509,166.342537522195));
#28462=CARTESIAN_POINT('Ctrl Pts',(-34.0495335253161,31.5269023563923,166.279784489292));
#28463=CARTESIAN_POINT('Ctrl Pts',(-34.0533144349913,32.0018139164182,166.254074719462));
#28464=CARTESIAN_POINT('Origin',(-32.,32.,180.545925280538));
#28465=CARTESIAN_POINT('',(-34.0574025789111,31.998873138922,167.654074719462));
#28466=CARTESIAN_POINT('',(-34.0524751566312,32.0013942609758,167.595925280538));
#28467=CARTESIAN_POINT('',(-34.05475,32.0000000000002,180.545925280538));
#28468=CARTESIAN_POINT('Ctrl Pts',(-34.0524751566312,32.0013942609758,167.595925280538));
#28469=CARTESIAN_POINT('Ctrl Pts',(-34.0540188898388,32.2486160605419,167.582555870051));
#28470=CARTESIAN_POINT('Ctrl Pts',(-33.898241798428,33.1789471714754,167.53214319649));
#28471=CARTESIAN_POINT('Ctrl Pts',(-32.5140741057304,34.3735883477403,167.444687259856));
#28472=CARTESIAN_POINT('Ctrl Pts',(-30.2847464657706,33.7193294309385,167.333557470637));
#28473=CARTESIAN_POINT('Ctrl Pts',(-29.6251964648778,31.4915603532478,167.222427681417));
#28474=CARTESIAN_POINT('Ctrl Pts',(-31.1390486307216,29.7291066950132,167.111297892197));
#28475=CARTESIAN_POINT('Ctrl Pts',(-33.3932697819141,30.038431497626,167.002463758571));
#28476=CARTESIAN_POINT('Ctrl Pts',(-34.0548080592417,31.3625118789545,166.930672888018));
#28477=CARTESIAN_POINT('Ctrl Pts',(-34.0578396023064,32.0007586512867,166.895925280538));
#28478=CARTESIAN_POINT('Ctrl Pts',(-34.0574025789111,31.9988731389219,167.654074719462));
#28479=CARTESIAN_POINT('Ctrl Pts',(-34.0533392486364,32.6141954663041,167.620593716431));
#28480=CARTESIAN_POINT('Ctrl Pts',(-33.4332618733263,33.9174120761424,167.550069450326));
#28481=CARTESIAN_POINT('Ctrl Pts',(-31.2169834524517,34.2989297408903,167.442501921148));
#28482=CARTESIAN_POINT('Ctrl Pts',(-29.6439176314904,32.5891267679911,167.331372131929));
#28483=CARTESIAN_POINT('Ctrl Pts',(-30.2271133920415,30.3401605499161,167.220242342709));
#28484=CARTESIAN_POINT('Ctrl Pts',(-32.4328346333002,29.6102630575578,167.109112553489));
#28485=CARTESIAN_POINT('Ctrl Pts',(-33.8775609285965,30.7736143033716,167.020390012407));
#28486=CARTESIAN_POINT('Ctrl Pts',(-34.0533636307896,31.7281065226901,166.968710734398));
#28487=CARTESIAN_POINT('Ctrl Pts',(-34.0520397258479,31.9988941582834,166.954074719462));
#28488=CARTESIAN_POINT('Origin',(-32.,32.,180.545925280538));
#28489=CARTESIAN_POINT('',(-34.0554334607891,32.0018241253936,168.354074719462));
#28490=CARTESIAN_POINT('',(-34.052787823778,31.9984585248469,168.295925280538));
#28491=CARTESIAN_POINT('',(-34.05475,32.0000000000002,180.545925280538));
#28492=CARTESIAN_POINT('Ctrl Pts',(-34.052787823778,31.9984585248469,168.295925280538));
#28493=CARTESIAN_POINT('Ctrl Pts',(-34.0496367476198,32.450278669858,168.271482115157));
#28494=CARTESIAN_POINT('Ctrl Pts',(-33.6800738256301,33.5915111338001,168.209995686702));
#28495=CARTESIAN_POINT('Ctrl Pts',(-31.7940424397143,34.4198708436861,168.111465995175));
#28496=CARTESIAN_POINT('Ctrl Pts',(-29.8553132008219,33.1395226443526,168.000336205955));
#28497=CARTESIAN_POINT('Ctrl Pts',(-29.8793780091033,30.8162956994218,167.889206416735));
#28498=CARTESIAN_POINT('Ctrl Pts',(-31.8442131747296,29.5763820510783,167.778076627516));
#28499=CARTESIAN_POINT('Ctrl Pts',(-33.6980917649276,30.4368608971767,167.680316248783));
#28500=CARTESIAN_POINT('Ctrl Pts',(-34.0497415946373,31.5636268332647,167.619599133124));
#28501=CARTESIAN_POINT('Ctrl Pts',(-34.0524751566312,32.0013942609758,167.595925280538));
#28502=CARTESIAN_POINT('Ctrl Pts',(-34.0554334607891,32.0018241253936,168.354074719462));
#28503=CARTESIAN_POINT('Ctrl Pts',(-34.0567078357127,32.140216458308,168.34656322461));
#28504=CARTESIAN_POINT('Ctrl Pts',(-33.980880674796,32.9597080078657,168.302008466685));
#28505=CARTESIAN_POINT('Ctrl Pts',(-32.880554936408,34.2633639788494,168.220410445686));
#28506=CARTESIAN_POINT('Ctrl Pts',(-30.5761275089639,33.9674299515833,168.109280656467));
#28507=CARTESIAN_POINT('Ctrl Pts',(-29.5748127402796,31.870925374144,167.998150867247));
#28508=CARTESIAN_POINT('Ctrl Pts',(-30.7930030593313,29.8925484830768,167.887021078027));
#28509=CARTESIAN_POINT('Ctrl Pts',(-33.1158238734678,29.8428883892604,167.775891288808));
#28510=CARTESIAN_POINT('Ctrl Pts',(-34.025301548937,31.1875816460392,167.698242502619));
#28511=CARTESIAN_POINT('Ctrl Pts',(-34.057834902849,31.9334050244322,167.657636979504));
#28512=CARTESIAN_POINT('Ctrl Pts',(-34.0574025789111,31.9988731389219,167.654074719462));
#28513=CARTESIAN_POINT('Origin',(-32.,32.,180.545925280538));
#28514=CARTESIAN_POINT('',(-34.0514403583153,31.9999806718109,169.054074719462));
#28515=CARTESIAN_POINT('',(-34.0580205430257,31.9994845592736,168.995925280538));
#28516=CARTESIAN_POINT('',(-34.05475,32.0000000000002,180.545925280538));
#28517=CARTESIAN_POINT('Ctrl Pts',(-34.0580205430257,31.9994845592736,168.995925280538));
#28518=CARTESIAN_POINT('Ctrl Pts',(-34.055824427603,32.6517037300251,168.960408360263));
#28519=CARTESIAN_POINT('Ctrl Pts',(-33.3683227053502,33.9881561453664,168.887848176915));
#28520=CARTESIAN_POINT('Ctrl Pts',(-31.0921885701096,34.2525700451136,168.778244730493));
#28521=CARTESIAN_POINT('Ctrl Pts',(-29.6151760590397,32.4591385080545,168.667114941274));
#28522=CARTESIAN_POINT('Ctrl Pts',(-30.32072855565,30.2455083878672,168.555985152054));
#28523=CARTESIAN_POINT('Ctrl Pts',(-32.5631320687118,29.637569963837,168.444855362834));
#28524=CARTESIAN_POINT('Ctrl Pts',(-33.910300100793,30.8498682204949,168.358168738995));
#28525=CARTESIAN_POINT('Ctrl Pts',(-34.0544121578939,31.7655517847545,168.30852537823));
#28526=CARTESIAN_POINT('Ctrl Pts',(-34.052787823778,31.9984585248469,168.295925280538));
#28527=CARTESIAN_POINT('Ctrl Pts',(-34.0514403583153,31.9999806718109,169.054074719462));
#28528=CARTESIAN_POINT('Ctrl Pts',(-34.0514114848212,32.3440857144559,169.035489469716));
#28529=CARTESIAN_POINT('Ctrl Pts',(-33.8062204233054,33.3740837335787,168.979860956897));
#28530=CARTESIAN_POINT('Ctrl Pts',(-32.1767327307596,34.4221806365661,168.887189181005));
#28531=CARTESIAN_POINT('Ctrl Pts',(-30.0609459727286,33.4622800598482,168.776059391785));
#28532=CARTESIAN_POINT('Ctrl Pts',(-29.7197604322381,31.1641166302031,168.664929602565));
#28533=CARTESIAN_POINT('Ctrl Pts',(-31.4654254161029,29.6309445956577,168.553799813346));
#28534=CARTESIAN_POINT('Ctrl Pts',(-33.5492655722574,30.2229879815584,168.450181518978));
#28535=CARTESIAN_POINT('Ctrl Pts',(-34.050423200433,31.4577286584152,168.383606487684));
#28536=CARTESIAN_POINT('Ctrl Pts',(-34.0554334607891,32.0018241253936,168.354074719462));
#28537=CARTESIAN_POINT('Origin',(-32.,32.,180.545925280538));
#28538=CARTESIAN_POINT('',(-34.0555043948901,31.9981860244241,169.754074719462));
#28539=CARTESIAN_POINT('',(-34.0543001799161,32.0018685375719,169.695925280538));
#28540=CARTESIAN_POINT('',(-34.05475,32.0000000000002,180.545925280538));
#28541=CARTESIAN_POINT('Ctrl Pts',(-34.0543001799161,32.0018685375718,169.695925280538));
#28542=CARTESIAN_POINT('Ctrl Pts',(-34.0558755534125,32.1780191654457,169.686377868442));
#28543=CARTESIAN_POINT('Ctrl Pts',(-33.9545116436601,33.0358359111826,169.639787193273));
#28544=CARTESIAN_POINT('Ctrl Pts',(-32.7552096073727,34.3082139954844,169.556153255031));
#28545=CARTESIAN_POINT('Ctrl Pts',(-30.4704602652025,33.8864521196416,169.445023465811));
#28546=CARTESIAN_POINT('Ctrl Pts',(-29.5855291011564,31.7382297216221,169.333893676592));
#28547=CARTESIAN_POINT('Ctrl Pts',(-30.9102955198749,29.8295766435978,169.222763887372));
#28548=CARTESIAN_POINT('Ctrl Pts',(-33.2323476614723,29.9072714840831,169.111634098152));
#28549=CARTESIAN_POINT('Ctrl Pts',(-34.0448973027964,31.2632688876247,169.036021229208));
#28550=CARTESIAN_POINT('Ctrl Pts',(-34.0581149212807,31.9714553825744,168.997451623336));
#28551=CARTESIAN_POINT('Ctrl Pts',(-34.0580205430257,31.9994845592736,168.995925280538));
#28552=CARTESIAN_POINT('Ctrl Pts',(-34.0555043948901,31.9981860244241,169.754074719462));
#28553=CARTESIAN_POINT('Ctrl Pts',(-34.0504819393845,32.5445771872936,169.724415714822));
#28554=CARTESIAN_POINT('Ctrl Pts',(-33.5457293608021,33.7815914750713,169.65771344711));
#28555=CARTESIAN_POINT('Ctrl Pts',(-31.4573116781621,34.3672099356773,169.553967916323));
#28556=CARTESIAN_POINT('Ctrl Pts',(-29.7169099061327,32.8280658895954,169.442838127104));
#28557=CARTESIAN_POINT('Ctrl Pts',(-30.0659674289288,30.5310849213574,169.331708337884));
#28558=CARTESIAN_POINT('Ctrl Pts',(-32.1850305870609,29.5784391033703,169.220578548664));
#28559=CARTESIAN_POINT('Ctrl Pts',(-33.8086854086604,30.6306661455679,169.12803400919));
#28560=CARTESIAN_POINT('Ctrl Pts',(-34.0514690341387,31.658231405593,169.07253273279));
#28561=CARTESIAN_POINT('Ctrl Pts',(-34.0514403583153,31.9999806718109,169.054074719462));
#28562=CARTESIAN_POINT('Origin',(-32.,32.,180.545925280538));
#28563=CARTESIAN_POINT('',(-34.0573517780835,32.0011604961581,170.454074719462));
#28564=CARTESIAN_POINT('',(-34.0516184036866,31.9993739362734,170.395925280538));
#28565=CARTESIAN_POINT('',(-34.05475,32.0000000000002,180.545925280538));
#28566=CARTESIAN_POINT('Ctrl Pts',(-34.0516184036866,31.9993739362734,170.395925280538));
#28567=CARTESIAN_POINT('Ctrl Pts',(-34.0505756284383,32.3810911960151,170.375304113548));
#28568=CARTESIAN_POINT('Ctrl Pts',(-33.765219332864,33.4499626319616,170.317639683486));
#28569=CARTESIAN_POINT('Ctrl Pts',(-32.0437423814044,34.4282256905171,170.22293199035));
#28570=CARTESIAN_POINT('Ctrl Pts',(-29.9837327342869,33.3538314936623,170.11180220113));
#28571=CARTESIAN_POINT('Ctrl Pts',(-29.768989023242,31.0404253954989,170.00067241191));
#28572=CARTESIAN_POINT('Ctrl Pts',(-31.5960423638194,29.6052115692218,169.88954262269));
#28573=CARTESIAN_POINT('Ctrl Pts',(-33.6040654953814,30.2966920425492,169.787960245566));
#28574=CARTESIAN_POINT('Ctrl Pts',(-34.0497632190666,31.494567567931,169.723421131515));
#28575=CARTESIAN_POINT('Ctrl Pts',(-34.0543001799161,32.0018685375718,169.695925280538));
#28576=CARTESIAN_POINT('Ctrl Pts',(-34.0573517780835,32.0011604961581,170.454074719462));
#28577=CARTESIAN_POINT('Ctrl Pts',(-34.0578102020088,32.0689714028747,170.450385223002));
#28578=CARTESIAN_POINT('Ctrl Pts',(-34.0240039615804,32.8171543593945,170.409652463468));
#28579=CARTESIAN_POINT('Ctrl Pts',(-33.1084266208509,34.1609220070185,170.331876440861));
#28580=CARTESIAN_POINT('Ctrl Pts',(-30.7857895731111,34.1033037187868,170.220746651641));
#28581=CARTESIAN_POINT('Ctrl Pts',(-29.5743847404962,32.1207646765004,170.109616862422));
#28582=CARTESIAN_POINT('Ctrl Pts',(-30.582876688677,30.0277031119193,169.998487073202));
#28583=CARTESIAN_POINT('Ctrl Pts',(-32.8883045233183,29.7396662706405,169.887357283983));
#28584=CARTESIAN_POINT('Ctrl Pts',(-33.9824484353958,31.0450458660859,169.805886499402));
#28585=CARTESIAN_POINT('Ctrl Pts',(-34.0567548451285,31.8621499840586,169.761458977896));
#28586=CARTESIAN_POINT('Ctrl Pts',(-34.0555043948901,31.9981860244241,169.754074719462));
#28587=CARTESIAN_POINT('Origin',(-32.,32.,180.545925280538));
#28588=CARTESIAN_POINT('',(-34.0520023281243,32.0010746918646,171.154074719462));
#28589=CARTESIAN_POINT('',(-34.0565936314237,31.9984640339053,171.095925280538));
#28590=CARTESIAN_POINT('',(-34.05475,32.0000000000002,180.545925280538));
#28591=CARTESIAN_POINT('Ctrl Pts',(-34.0565936314237,31.9984640339053,171.095925280538));
#28592=CARTESIAN_POINT('Ctrl Pts',(-34.0517293483252,32.5815615602143,171.064230358654));
#28593=CARTESIAN_POINT('Ctrl Pts',(-33.4873352336299,33.854384656826,170.995492173698));
#28594=CARTESIAN_POINT('Ctrl Pts',(-31.3284143499829,34.3339164755211,170.889710725668));
#28595=CARTESIAN_POINT('Ctrl Pts',(-29.6749656940012,32.7017185161778,170.778580936448));
#28596=CARTESIAN_POINT('Ctrl Pts',(-30.1493632209224,30.4273153806489,170.667451147228));
#28597=CARTESIAN_POINT('Ctrl Pts',(-32.3174434587353,29.5922161536956,170.556321358009));
#28598=CARTESIAN_POINT('Ctrl Pts',(-33.8466042542176,30.7067606771023,170.465812735778));
#28599=CARTESIAN_POINT('Ctrl Pts',(-34.0524488394874,31.695385441368,170.412347376621));
#28600=CARTESIAN_POINT('Ctrl Pts',(-34.0516184036866,31.9993739362734,170.395925280538));
#28601=CARTESIAN_POINT('Ctrl Pts',(-34.0520023281243,32.0010746918646,171.154074719462));
#28602=CARTESIAN_POINT('Ctrl Pts',(-34.0532978514709,32.2742285901281,171.139311468108));
#28603=CARTESIAN_POINT('Ctrl Pts',(-33.8754247390233,33.2311488262767,171.087504953681));
#28604=CARTESIAN_POINT('Ctrl Pts',(-32.4246449842735,34.3912068357963,170.99865517618));
#28605=CARTESIAN_POINT('Ctrl Pts',(-30.2214365358583,33.6537549692286,170.88752538696));
#28606=CARTESIAN_POINT('Ctrl Pts',(-29.645950082108,31.4028044890487,170.77639559774));
#28607=CARTESIAN_POINT('Ctrl Pts',(-31.224864584604,29.6984008641758,170.665265808521));
#28608=CARTESIAN_POINT('Ctrl Pts',(-33.4372029785745,30.0870496218184,170.557825515761));
#28609=CARTESIAN_POINT('Ctrl Pts',(-34.0532075365108,31.3881366917763,170.487428486075));
#28610=CARTESIAN_POINT('Ctrl Pts',(-34.0573517780835,32.0011604961581,170.454074719462));
#28611=CARTESIAN_POINT('Origin',(-32.,32.,180.545925280538));
#28612=CARTESIAN_POINT('',(-34.0534331717271,31.9982546175746,171.854074719462));
#28613=CARTESIAN_POINT('',(-34.0564014405732,32.0016034613785,171.795925280538));
#28614=CARTESIAN_POINT('',(-34.05475,32.0000000000002,180.545925280538));
#28615=CARTESIAN_POINT('Ctrl Pts',(-34.0564014405732,32.0016034613785,171.795925280538));
#28616=CARTESIAN_POINT('Ctrl Pts',(-34.0573060965439,32.1069606022137,171.790199866834));
#28617=CARTESIAN_POINT('Ctrl Pts',(-34.0020448223411,32.8930239103454,171.747431190057));
#28618=CARTESIAN_POINT('Ctrl Pts',(-32.9883523019571,34.2184122987475,171.667619250206));
#28619=CARTESIAN_POINT('Ctrl Pts',(-30.6723620474344,34.0336103036043,171.556489460986));
#28620=CARTESIAN_POINT('Ctrl Pts',(-29.5714116494658,31.9876702121879,171.445359671767));
#28621=CARTESIAN_POINT('Ctrl Pts',(-30.693078972962,29.9530142088661,171.334229882547));
#28622=CARTESIAN_POINT('Ctrl Pts',(-33.0108262474351,29.7917374029535,171.223100093327));
#28623=CARTESIAN_POINT('Ctrl Pts',(-34.0062836592036,31.121039988534,171.143665225991));
#28624=CARTESIAN_POINT('Ctrl Pts',(-34.0574144520508,31.9000695803972,171.101273621728));
#28625=CARTESIAN_POINT('Ctrl Pts',(-34.0565936314237,31.9984640339053,171.095925280538));
#28626=CARTESIAN_POINT('Ctrl Pts',(-34.0534331717271,31.9982546175746,171.854074719462));
#28627=CARTESIAN_POINT('Ctrl Pts',(-34.0495792571287,32.4754606590366,171.828237713214));
#28628=CARTESIAN_POINT('Ctrl Pts',(-33.6462714964515,33.64272521891,171.765357443893));
#28629=CARTESIAN_POINT('Ctrl Pts',(-31.7033831827247,34.4104381257226,171.665433911498));
#28630=CARTESIAN_POINT('Ctrl Pts',(-29.81406369269,33.0582419168657,171.554304122278));
#28631=CARTESIAN_POINT('Ctrl Pts',(-29.9252894056131,30.7375541818489,171.443174333058));
#28632=CARTESIAN_POINT('Ctrl Pts',(-31.9352677552198,29.5722431689493,171.332044543839));
#28633=CARTESIAN_POINT('Ctrl Pts',(-33.729598748851,30.4884300255591,171.235678005973));
#28634=CARTESIAN_POINT('Ctrl Pts',(-34.0500471845957,31.5888435438389,171.176354731181));
#28635=CARTESIAN_POINT('Ctrl Pts',(-34.0520023281243,32.0010746918646,171.154074719462));
#28636=CARTESIAN_POINT('Origin',(-32.,32.,180.545925280538));
#28637=CARTESIAN_POINT('',(-34.0581778177724,31.9999545502976,172.554074719462));
#28638=CARTESIAN_POINT('',(-34.0515604146746,32.0005167850725,172.495925280538));
#28639=CARTESIAN_POINT('',(-34.05475,32.0000000000002,180.545925280538));
#28640=CARTESIAN_POINT('Ctrl Pts',(-34.0515604146746,32.0005167850725,172.495925280538));
#28641=CARTESIAN_POINT('Ctrl Pts',(-34.0522605175172,32.311507193629,172.47912611194));
#28642=CARTESIAN_POINT('Ctrl Pts',(-33.839795546903,33.307343922864,172.425283680269));
#28643=CARTESIAN_POINT('Ctrl Pts',(-32.2929793955673,34.4108829241154,172.334397985524));
#28644=CARTESIAN_POINT('Ctrl Pts',(-30.1334901928539,33.5538129037453,172.223268196305));
#28645=CARTESIAN_POINT('Ctrl Pts',(-29.6822105241847,31.2747101642669,172.112138407085));
#28646=CARTESIAN_POINT('Ctrl Pts',(-31.3521466484014,29.6593848170106,172.001008617865));
#28647=CARTESIAN_POINT('Ctrl Pts',(-33.49840924462,30.1590253490049,171.895604242349));
#28648=CARTESIAN_POINT('Ctrl Pts',(-34.0514529982616,31.4253029113651,171.827243129907));
#28649=CARTESIAN_POINT('Ctrl Pts',(-34.0564014405732,32.0016034613785,171.795925280538));
#28650=CARTESIAN_POINT('Ctrl Pts',(-34.0581773322723,31.9999545567349,172.554074719462));
#28651=CARTESIAN_POINT('Ctrl Pts',(-34.0579568195032,32.6776310956056,172.51716395832));
#28652=CARTESIAN_POINT('Ctrl Pts',(-33.32180623737,34.0358274377969,172.443209934105));
#28653=CARTESIAN_POINT('Ctrl Pts',(-31.0083014790376,34.2169184779213,172.332212646816));
#28654=CARTESIAN_POINT('Ctrl Pts',(-29.5996267287836,32.3693259441983,172.221082857597));
#28655=CARTESIAN_POINT('Ctrl Pts',(-30.3877475653827,30.183730311518,172.109953068377));
#28656=CARTESIAN_POINT('Ctrl Pts',(-32.6513843459939,29.660365001112,171.998823279157));
#28657=CARTESIAN_POINT('Ctrl Pts',(-33.9311982594295,30.902069459774,171.913530496186));
#28658=CARTESIAN_POINT('Ctrl Pts',(-34.0551047259449,31.7912765564278,171.865280976287));
#28659=CARTESIAN_POINT('Ctrl Pts',(-34.0534331717271,31.9982546175746,171.854074719462));
#28660=CARTESIAN_POINT('Origin',(-32.,32.,180.545925280538));
#28661=CARTESIAN_POINT('',(-34.0535655946932,32.0017741612571,173.254074719462));
#28662=CARTESIAN_POINT('',(-34.054507140811,31.998123038607,173.195925280538));
#28663=CARTESIAN_POINT('',(-34.05475,32.0000000000002,180.545925280538));
#28664=CARTESIAN_POINT('Ctrl Pts',(-34.054507140811,31.998123038607,173.195925280538));
#28665=CARTESIAN_POINT('Ctrl Pts',(-34.0498473910169,32.5122490193519,173.168052357046));
#28666=CARTESIAN_POINT('Ctrl Pts',(-33.5941675160557,33.7170162573815,173.103136170481));
#28667=CARTESIAN_POINT('Ctrl Pts',(-31.5717474387099,34.3905633528034,173.001176720843));
#28668=CARTESIAN_POINT('Ctrl Pts',(-29.7593608834192,32.93687232282,172.890046931623));
#28669=CARTESIAN_POINT('Ctrl Pts',(-29.9975829489038,30.625765902949,172.778917142403));
#28670=CARTESIAN_POINT('Ctrl Pts',(-32.068395384243,29.5723436257509,172.667787353184));
#28671=CARTESIAN_POINT('Ctrl Pts',(-33.7730366450004,30.5640711797273,172.573456732562));
#28672=CARTESIAN_POINT('Ctrl Pts',(-34.0507167450606,31.6257530475051,172.516169375013));
#28673=CARTESIAN_POINT('Ctrl Pts',(-34.0515604146746,32.0005167850725,172.495925280538));
#28674=CARTESIAN_POINT('Ctrl Pts',(-34.0535655946932,32.0017741612571,173.254074719462));
#28675=CARTESIAN_POINT('Ctrl Pts',(-34.0552323561726,32.2038246657458,173.2431334665));
#28676=CARTESIAN_POINT('Ctrl Pts',(-33.9350351245523,33.0880078984862,173.195148950464));
#28677=CARTESIAN_POINT('Ctrl Pts',(-32.6680632717471,34.3349271849826,173.110121171355));
#28678=CARTESIAN_POINT('Ctrl Pts',(-30.4007494190391,33.8277283916173,172.998991382135));
#28679=CARTESIAN_POINT('Ctrl Pts',(-29.5970523548762,31.6478123951331,172.887861592915));
#28680=CARTESIAN_POINT('Ctrl Pts',(-30.9925069166485,29.7902146753074,172.776731803695));
#28681=CARTESIAN_POINT('Ctrl Pts',(-33.3100082224966,29.9549885205165,172.665602014476));
#28682=CARTESIAN_POINT('Ctrl Pts',(-34.0570726014949,31.3149806065769,172.591382986398));
#28683=CARTESIAN_POINT('Ctrl Pts',(-34.0581781238671,31.9975218393558,172.554207221394));
#28684=CARTESIAN_POINT('Ctrl Pts',(-34.0581773322723,31.9999545567349,172.554074719462));
#28685=CARTESIAN_POINT('Origin',(-32.,32.,180.545925280538));
#28686=CARTESIAN_POINT('',(-34.0519273834553,31.9989926864668,173.954074719462));
#28687=CARTESIAN_POINT('',(-34.0579373256583,32.0006373959877,173.895925280538));
#28688=CARTESIAN_POINT('',(-34.05475,32.0000000000002,180.545925280538));
#28689=CARTESIAN_POINT('Ctrl Pts',(-34.0579373256583,32.0006373959877,173.895925280538));
#28690=CARTESIAN_POINT('Ctrl Pts',(-34.0580796886322,32.0355947629004,173.894021865225));
#28691=CARTESIAN_POINT('Ctrl Pts',(-34.041431950888,32.7507355168895,173.85507518684));
#28692=CARTESIAN_POINT('Ctrl Pts',(-33.2110353847761,34.1051334154486,173.779085245381));
#28693=CARTESIAN_POINT('Ctrl Pts',(-30.8883140600557,34.1592470379621,173.667955456161));
#28694=CARTESIAN_POINT('Ctrl Pts',(-29.5829956518403,32.2372411873918,173.556825666941));
#28695=CARTESIAN_POINT('Ctrl Pts',(-30.48969341174,30.098114774894,173.445695877722));
#28696=CARTESIAN_POINT('Ctrl Pts',(-32.7786073826223,29.6995730953269,173.334566088502));
#28697=CARTESIAN_POINT('Ctrl Pts',(-33.9595797099711,30.9782715764583,173.251309222774));
#28698=CARTESIAN_POINT('Ctrl Pts',(-34.0560402231944,31.8289728655904,173.205095620119));
#28699=CARTESIAN_POINT('Ctrl Pts',(-34.054507140811,31.998123038607,173.195925280538));
#28700=CARTESIAN_POINT('Ctrl Pts',(-34.0519273834553,31.9989926864668,173.954074719462));
#28701=CARTESIAN_POINT('Ctrl Pts',(-34.0501205240319,32.4063578939422,173.932059711606));
#28702=CARTESIAN_POINT('Ctrl Pts',(-33.7354249649502,33.501743785199,173.873001440676));
#28703=CARTESIAN_POINT('Ctrl Pts',(-31.9525937468572,34.4281569433195,173.776899906673));
#28704=CARTESIAN_POINT('Ctrl Pts',(-29.9343509763561,33.2772186991064,173.665770117453));
#28705=CARTESIAN_POINT('Ctrl Pts',(-29.8065677912631,30.9573837523311,173.554640328233));
#28706=CARTESIAN_POINT('Ctrl Pts',(-31.6861899768242,29.59173988872,173.443510539014));
#28707=CARTESIAN_POINT('Ctrl Pts',(-33.6396742476966,30.3475681058338,173.343322002757));
#28708=CARTESIAN_POINT('Ctrl Pts',(-34.0495892836497,31.5197521909239,173.280176729573));
#28709=CARTESIAN_POINT('Ctrl Pts',(-34.0535655946932,32.0017741612571,173.254074719462));
#28710=CARTESIAN_POINT('Origin',(-32.,32.,180.545925280538));
#28711=CARTESIAN_POINT('',(-34.0572421730302,31.9987715047938,174.654074719462));
#28712=CARTESIAN_POINT('',(-34.0526302784379,32.0014721866858,174.595925280538));
#28713=CARTESIAN_POINT('',(-34.05475,32.0000000000002,180.545925280538));
#28714=CARTESIAN_POINT('Ctrl Pts',(-34.052630278438,32.0014721866858,174.595925280538));
#28715=CARTESIAN_POINT('Ctrl Pts',(-34.0542200654754,32.2413952503059,174.582948110331));
#28716=CARTESIAN_POINT('Ctrl Pts',(-33.9044368370703,33.1642554087556,174.532927677052));
#28717=CARTESIAN_POINT('Ctrl Pts',(-32.53911584455,34.368026078018,174.445863980699));
#28718=CARTESIAN_POINT('Ctrl Pts',(-30.3030006968699,33.737350501538,174.33473419148));
#28719=CARTESIAN_POINT('Ctrl Pts',(-29.6199609082234,31.516670586832,174.22360440226));
#28720=CARTESIAN_POINT('Ctrl Pts',(-31.1151070859216,29.7383285095682,174.11247461304));
#28721=CARTESIAN_POINT('Ctrl Pts',(-33.3806181097287,30.0248506233853,174.003248239133));
#28722=CARTESIAN_POINT('Ctrl Pts',(-34.0553090956569,31.3552729589962,173.931065128299));
#28723=CARTESIAN_POINT('Ctrl Pts',(-34.0579373256583,32.0006373959877,173.895925280538));
#28724=CARTESIAN_POINT('Ctrl Pts',(-34.0572421730302,31.9987715047937,174.654074719462));
#28725=CARTESIAN_POINT('Ctrl Pts',(-34.0529417874593,32.6070099230316,174.620985956712));
#28726=CARTESIAN_POINT('Ctrl Pts',(-33.445367295585,33.9036433939219,174.550853930888));
#28727=CARTESIAN_POINT('Ctrl Pts',(-31.2413084093575,34.3070718594175,174.443678641991));
#28728=CARTESIAN_POINT('Ctrl Pts',(-29.650271574393,32.6139786805113,174.332548852772));
#28729=CARTESIAN_POINT('Ctrl Pts',(-30.2096807128004,30.3589788715227,174.221419063552));
#28730=CARTESIAN_POINT('Ctrl Pts',(-32.4075706476486,29.6058238031834,174.110289274332));
#28731=CARTESIAN_POINT('Ctrl Pts',(-33.8709432602969,30.7589286188374,174.021174492969));
#28732=CARTESIAN_POINT('Ctrl Pts',(-34.0531608122478,31.720910191825,173.969102974679));
#28733=CARTESIAN_POINT('Ctrl Pts',(-34.0519273834553,31.9989926864668,173.954074719462));
#28734=CARTESIAN_POINT('Origin',(-32.,32.,180.545925280538));
#28735=CARTESIAN_POINT('',(-34.0556515462546,32.0017900557631,175.354074719462));
#28736=CARTESIAN_POINT('',(-34.0526241093217,31.9985307172981,175.295925280538));
#28737=CARTESIAN_POINT('',(-34.05475,32.0000000000002,180.545925280538));
#28738=CARTESIAN_POINT('Ctrl Pts',(-34.0526241093217,31.9985307172981,175.295925280538));
#28739=CARTESIAN_POINT('Ctrl Pts',(-34.0496840965633,32.4431896949484,175.271874355438));
#28740=CARTESIAN_POINT('Ctrl Pts',(-33.6893167705434,33.5770541420994,175.210780167264));
#28741=CARTESIAN_POINT('Ctrl Pts',(-31.8196126720174,34.4219111899327,175.112642716018));
#28742=CARTESIAN_POINT('Ctrl Pts',(-29.867468483099,33.1621113240314,175.001512926798));
#28743=CARTESIAN_POINT('Ctrl Pts',(-29.8669940121071,30.8387597769491,174.890383137578));
#28744=CARTESIAN_POINT('Ctrl Pts',(-31.8186234897481,29.5781626888771,174.779253348358));
#28745=CARTESIAN_POINT('Ctrl Pts',(-33.6889615308727,30.4223864705328,174.681100729345));
#28746=CARTESIAN_POINT('Ctrl Pts',(-34.0496820268643,31.5565361460665,174.619991373405));
#28747=CARTESIAN_POINT('Ctrl Pts',(-34.052630278438,32.0014721866858,174.595925280538));
#28748=CARTESIAN_POINT('Ctrl Pts',(-34.0556515462546,32.0017900557631,175.354074719462));
#28749=CARTESIAN_POINT('Ctrl Pts',(-34.0568506849504,32.1329198985566,175.346955464891));
#28750=CARTESIAN_POINT('Ctrl Pts',(-33.9856838785989,32.94505453146,175.302792947247));
#28751=CARTESIAN_POINT('Ctrl Pts',(-32.9044115271646,34.2539372847887,175.221587166529));
#28752=CARTESIAN_POINT('Ctrl Pts',(-30.5969869759018,33.9823591875437,175.11045737731));
#28753=CARTESIAN_POINT('Ctrl Pts',(-29.5735847292512,31.8965474596491,174.99932758809));
#28754=CARTESIAN_POINT('Ctrl Pts',(-30.7708114250119,29.9054143747875,174.88819779887));
#28755=CARTESIAN_POINT('Ctrl Pts',(-33.0929781746067,29.8312233392852,174.77706800965));
#28756=CARTESIAN_POINT('Ctrl Pts',(-34.0212734697525,31.172979462216,174.699026983181));
#28757=CARTESIAN_POINT('Ctrl Pts',(-34.0577561202048,31.9260797864791,174.658029219785));
#28758=CARTESIAN_POINT('Ctrl Pts',(-34.0572421730302,31.9987715047937,174.654074719462));
#28759=CARTESIAN_POINT('Origin',(-32.,32.,180.545925280538));
#28760=CARTESIAN_POINT('',(-34.0514445903522,32.000099796643,176.054074719462));
#28761=CARTESIAN_POINT('',(-34.0579336495468,31.9993577651623,175.995925280538));
#28762=CARTESIAN_POINT('',(-34.05475,32.0000000000002,180.545925280538));
#28763=CARTESIAN_POINT('Ctrl Pts',(-34.0579336495468,31.9993577651623,175.995925280538));
#28764=CARTESIAN_POINT('Ctrl Pts',(-34.0552889021134,32.6444467097459,175.960800600544));
#28765=CARTESIAN_POINT('Ctrl Pts',(-33.3811101331092,33.9746252333219,175.888632657476));
#28766=CARTESIAN_POINT('Ctrl Pts',(-31.1160309092789,34.2620327244924,175.779421451336));
#28767=CARTESIAN_POINT('Ctrl Pts',(-29.6201585161938,32.4843014680682,175.668291662116));
#28768=CARTESIAN_POINT('Ctrl Pts',(-30.3022912407822,30.2633427601015,175.557161872896));
#28769=CARTESIAN_POINT('Ctrl Pts',(-32.5381486109218,29.631753924825,175.446032083677));
#28770=CARTESIAN_POINT('Ctrl Pts',(-33.9041990981139,30.8351764637911,175.358953219557));
#28771=CARTESIAN_POINT('Ctrl Pts',(-34.0542123076651,31.7583254155745,175.308917618511));
#28772=CARTESIAN_POINT('Ctrl Pts',(-34.0526241093217,31.9985307172981,175.295925280538));
#28773=CARTESIAN_POINT('Ctrl Pts',(-34.0514445903522,32.000099796643,176.054074719462));
#28774=CARTESIAN_POINT('Ctrl Pts',(-34.051590542369,32.3369407953034,176.035881709997));
#28775=CARTESIAN_POINT('Ctrl Pts',(-33.8137830896685,33.3594384891899,175.980645437459));
#28776=CARTESIAN_POINT('Ctrl Pts',(-32.2023060055888,34.4201788723936,175.888365901848));
#28777=CARTESIAN_POINT('Ctrl Pts',(-30.0764987714868,33.4826788317565,175.777236112628));
#28778=CARTESIAN_POINT('Ctrl Pts',(-29.7110590022335,31.1882472032951,175.666106323408));
#28779=CARTESIAN_POINT('Ctrl Pts',(-31.4404332115969,29.6367229312773,175.554976534189));
#28780=CARTESIAN_POINT('Ctrl Pts',(-33.5383217807162,30.2088814213863,175.45096599954));
#28781=CARTESIAN_POINT('Ctrl Pts',(-34.0506112662406,31.4506185122487,175.383998727964));
#28782=CARTESIAN_POINT('Ctrl Pts',(-34.0556515462546,32.0017900557631,175.354074719462));
#28783=CARTESIAN_POINT('Origin',(-32.,32.,180.545925280538));
#28784=CARTESIAN_POINT('',(-34.0552853099115,31.9981575238583,176.754074719462));
#28785=CARTESIAN_POINT('',(-34.0545155163552,32.0018771437926,176.695925280538));
#28786=CARTESIAN_POINT('',(-34.05475,32.0000000000002,180.545925280538));
#28787=CARTESIAN_POINT('Ctrl Pts',(-34.0545155163552,32.0018771437926,176.695925280538));
#28788=CARTESIAN_POINT('Ctrl Pts',(-34.0560467546979,32.1707457859868,176.686770108723));
#28789=CARTESIAN_POINT('Ctrl Pts',(-33.9597818030922,33.0211610160312,176.640571673835));
#28790=CARTESIAN_POINT('Ctrl Pts',(-32.7795468963266,34.3001087007756,176.557329975874));
#28791=CARTESIAN_POINT('Ctrl Pts',(-30.4904703373783,33.9025019311548,176.446200186654));
#28792=CARTESIAN_POINT('Ctrl Pts',(-29.5828989554375,31.7637460255249,176.335070397434));
#28793=CARTESIAN_POINT('Ctrl Pts',(-30.8874322371387,29.8412071954588,176.223940608215));
#28794=CARTESIAN_POINT('Ctrl Pts',(-33.210175470102,29.8943721288814,176.112810818995));
#28795=CARTESIAN_POINT('Ctrl Pts',(-34.0412910121703,31.2487010232944,176.036805709769));
#28796=CARTESIAN_POINT('Ctrl Pts',(-34.0580781111525,31.9641216652496,175.997843863617));
#28797=CARTESIAN_POINT('Ctrl Pts',(-34.0579336495468,31.9993577651623,175.995925280538));
#28798=CARTESIAN_POINT('Ctrl Pts',(-34.0552853099115,31.9981575238583,176.754074719462));
#28799=CARTESIAN_POINT('Ctrl Pts',(-34.0503077464059,32.5374704460802,176.724807955103));
#28800=CARTESIAN_POINT('Ctrl Pts',(-33.5565883061217,33.7674634392079,176.658497927671));
#28801=CARTESIAN_POINT('Ctrl Pts',(-31.4823444807967,34.3728097817195,176.555144637166));
#28802=CARTESIAN_POINT('Ctrl Pts',(-29.7257833087973,32.8521337550634,176.444014847946));
#28803=CARTESIAN_POINT('Ctrl Pts',(-30.0505605908462,30.5515941579779,176.332885058727));
#28804=CARTESIAN_POINT('Ctrl Pts',(-32.1594436788161,29.5766198796149,176.221755269507));
#28805=CARTESIAN_POINT('Ctrl Pts',(-33.8010499920725,30.6160259659334,176.128818489752));
#28806=CARTESIAN_POINT('Ctrl Pts',(-34.051293365645,31.651090015572,176.072924973071));
#28807=CARTESIAN_POINT('Ctrl Pts',(-34.0514445903522,32.000099796643,176.054074719462));
#28808=CARTESIAN_POINT('Origin',(-32.,32.,180.545925280538));
#28809=CARTESIAN_POINT('',(-34.0575043898772,32.0010548445575,177.454074719462));
#28810=CARTESIAN_POINT('',(-34.0515583141596,31.999487637131,177.395925280538));
#28811=CARTESIAN_POINT('',(-34.05475,32.0000000000002,180.545925280538));
#28812=CARTESIAN_POINT('Ctrl Pts',(-34.0515583141596,31.999487637131,177.395925280538));
#28813=CARTESIAN_POINT('Ctrl Pts',(-34.0507225647854,32.3739715482354,177.375696353829));
#28814=CARTESIAN_POINT('Ctrl Pts',(-33.7733489562679,33.4353641275151,177.318424164048));
#28815=CARTESIAN_POINT('Ctrl Pts',(-32.0693869201392,34.4276282208927,177.224108711192));
#28816=CARTESIAN_POINT('Ctrl Pts',(-29.9981444046188,33.3750518506594,177.112978921973));
#28817=CARTESIAN_POINT('Ctrl Pts',(-29.758978416765,31.0640429106968,177.001849132753));
#28818=CARTESIAN_POINT('Ctrl Pts',(-31.5707710809886,29.6096117624978,176.890719343533));
#28819=CARTESIAN_POINT('Ctrl Pts',(-33.5937669922501,30.2824328445151,176.788744726128));
#28820=CARTESIAN_POINT('Ctrl Pts',(-34.0498511238672,31.487476737163,176.723813371796));
#28821=CARTESIAN_POINT('Ctrl Pts',(-34.0545155163552,32.0018771437926,176.695925280538));
#28822=CARTESIAN_POINT('Ctrl Pts',(-34.0575043898772,32.0010548445575,177.454074719462));
#28823=CARTESIAN_POINT('Ctrl Pts',(-34.0578837084661,32.06164475004,177.450777463283));
#28824=CARTESIAN_POINT('Ctrl Pts',(-34.0279763621718,32.8025565918032,177.41043694403));
#28825=CARTESIAN_POINT('Ctrl Pts',(-33.1311884148471,34.1490941434474,177.333053161704));
#28826=CARTESIAN_POINT('Ctrl Pts',(-30.8080724930038,34.1160109663009,177.221923372484));
#28827=CARTESIAN_POINT('Ctrl Pts',(-29.5757955383114,32.1463773261312,177.110793583265));
#28828=CARTESIAN_POINT('Ctrl Pts',(-30.5621242967963,30.0427808298698,176.999663794045));
#28829=CARTESIAN_POINT('Ctrl Pts',(-32.8643812668194,29.7304100510143,176.888534004825));
#28830=CARTESIAN_POINT('Ctrl Pts',(-33.9775854365096,31.0303892118588,176.806670979964));
#28831=CARTESIAN_POINT('Ctrl Pts',(-34.0566079028612,31.8548561942385,176.761851218177));
#28832=CARTESIAN_POINT('Ctrl Pts',(-34.0552853099115,31.9981575238583,176.754074719462));
#28833=CARTESIAN_POINT('Origin',(-32.,32.,180.545925280538));
#28834=CARTESIAN_POINT('',(-34.0521188506995,32.0011671092335,178.154074719462));
#28835=CARTESIAN_POINT('',(-34.0563933814841,31.9983925126321,178.095925280538));
#28836=CARTESIAN_POINT('',(-34.05475,32.0000000000002,180.545925280538));
#28837=CARTESIAN_POINT('Ctrl Pts',(-34.0563933814841,31.9983925126321,178.095925280538));
#28838=CARTESIAN_POINT('Ctrl Pts',(-34.0514420886706,32.5744194654198,178.064622598935));
#28839=CARTESIAN_POINT('Ctrl Pts',(-33.4988525240404,33.840436615865,177.99627665426));
#28840=CARTESIAN_POINT('Ctrl Pts',(-31.3531025346477,34.3408784778579,177.890887446511));
#28841=CARTESIAN_POINT('Ctrl Pts',(-29.6825070314679,32.7262369940422,177.779757657291));
#28842=CARTESIAN_POINT('Ctrl Pts',(-30.1328556755869,30.4469493074261,177.668627868071));
#28843=CARTESIAN_POINT('Ctrl Pts',(-32.2919946972204,29.588997745803,177.557498078852));
#28844=CARTESIAN_POINT('Ctrl Pts',(-33.8395196429225,30.6920887795438,177.46659721634));
#28845=CARTESIAN_POINT('Ctrl Pts',(-34.0522529912079,31.6882156386111,177.412739616902));
#28846=CARTESIAN_POINT('Ctrl Pts',(-34.0515583141596,31.999487637131,177.395925280538));
#28847=CARTESIAN_POINT('Ctrl Pts',(-34.0521188506995,32.0011671092335,178.154074719462));
#28848=CARTESIAN_POINT('Ctrl Pts',(-34.0535001213909,32.2670274833358,178.139703708389));
#28849=CARTESIAN_POINT('Ctrl Pts',(-33.8819824988062,33.2164703631673,178.088289434242));
#28850=CARTESIAN_POINT('Ctrl Pts',(-32.4498708069788,34.3865813639729,177.999831897023));
#28851=CARTESIAN_POINT('Ctrl Pts',(-30.239005926868,33.6724513835904,177.888702107803));
#28852=CARTESIAN_POINT('Ctrl Pts',(-29.6397722337213,31.4276996511778,177.777572318583));
#28853=CARTESIAN_POINT('Ctrl Pts',(-31.2005990409054,29.7067170736135,177.666442529363));
#28854=CARTESIAN_POINT('Ctrl Pts',(-33.4250091228452,30.0733096650126,177.558609996323));
#28855=CARTESIAN_POINT('Ctrl Pts',(-34.0536222263393,31.3809430738059,177.487820726356));
#28856=CARTESIAN_POINT('Ctrl Pts',(-34.0575043898772,32.0010548445575,177.454074719462));
#28857=CARTESIAN_POINT('Origin',(-32.,32.,180.545925280538));
#28858=CARTESIAN_POINT('',(-34.0526600320705,31.9978184065947,178.854074719462));
#28859=CARTESIAN_POINT('',(-34.0565967526292,32.0015021117824,178.795925280538));
#28860=CARTESIAN_POINT('',(-34.05475,32.0000000000002,180.545925280538));
#28861=CARTESIAN_POINT('',(-32.5301702171895,30.0148256743285,179.));
#28862=CARTESIAN_POINT('Ctrl Pts',(-32.5301702171895,30.0148256743285,179.));
#28863=CARTESIAN_POINT('Ctrl Pts',(-33.1902397907536,30.1911070339307,178.962956736927));
#28864=CARTESIAN_POINT('Ctrl Pts',(-33.9248822846665,30.8874020551484,178.914314976748));
#28865=CARTESIAN_POINT('Ctrl Pts',(-34.0542719955,31.7835489011663,178.865673216568));
#28866=CARTESIAN_POINT('Ctrl Pts',(-34.0526600320705,31.9978184065947,178.854074719462));
#28867=CARTESIAN_POINT('',(-31.4686665574919,30.0112662655011,179.));
#28868=CARTESIAN_POINT('Origin',(-32.,32.,179.));
#28869=CARTESIAN_POINT('Ctrl Pts',(-31.4686656825477,30.0112635882183,179.));
#28870=CARTESIAN_POINT('Ctrl Pts',(-32.1131054357931,29.8400086888077,178.963685183163));
#28871=CARTESIAN_POINT('Ctrl Pts',(-33.4929539281089,30.1591334335668,178.895660276675));
#28872=CARTESIAN_POINT('Ctrl Pts',(-34.051753790298,31.4182518043251,178.827635370188));
#28873=CARTESIAN_POINT('Ctrl Pts',(-34.0565967526292,32.0015021117824,178.795925280538));
#28874=CARTESIAN_POINT('Origin',(-32.,-32.,172.));
#28875=CARTESIAN_POINT('',(-33.6685050984025,-31.9993848812913,166.67148036339));
#28876=CARTESIAN_POINT('',(-33.6648360717667,-31.9985292840412,166.47851963661));
#28877=CARTESIAN_POINT('',(-33.666,-32.,172.));
#28878=CARTESIAN_POINT('',(-31.324922814325,-33.5230977622533,166.));
#28879=CARTESIAN_POINT('Ctrl Pts',(-33.6648360717667,-31.9985292840412,
166.47851963661));
#28880=CARTESIAN_POINT('Ctrl Pts',(-33.6661874534241,-31.8287853144728,
166.467186143366));
#28881=CARTESIAN_POINT('Ctrl Pts',(-33.6423113385545,-31.6594223896045,
166.455852650123));
#28882=CARTESIAN_POINT('Ctrl Pts',(-33.5916296652012,-31.4985231924663,
166.444519156879));
#28883=CARTESIAN_POINT('Ctrl Pts',(-33.4259777767092,-30.9726278520149,
166.407475893806));
#28884=CARTESIAN_POINT('Ctrl Pts',(-32.9739636477032,-30.5371500284145,
166.370432630732));
#28885=CARTESIAN_POINT('Ctrl Pts',(-32.4421510491472,-30.390950974798,166.333389367659));
#28886=CARTESIAN_POINT('Ctrl Pts',(-31.9103384505912,-30.2447519211814,
166.296346104586));
#28887=CARTESIAN_POINT('Ctrl Pts',(-31.2987273824852,-30.3878316375487,
166.259302841513));
#28888=CARTESIAN_POINT('Ctrl Pts',(-30.8877524141389,-30.7555629540326,
166.222259578439));
#28889=CARTESIAN_POINT('Ctrl Pts',(-30.4767774457927,-31.1232942705165,
166.185216315366));
#28890=CARTESIAN_POINT('Ctrl Pts',(-30.2664385772063,-31.715677187117,166.148173052293));
#28891=CARTESIAN_POINT('Ctrl Pts',(-30.3518675885088,-32.2595123446316,
166.11112978922));
#28892=CARTESIAN_POINT('Ctrl Pts',(-30.4372965998113,-32.803347502146,166.074086526147));
#28893=CARTESIAN_POINT('Ctrl Pts',(-30.8184934910026,-33.2986349005746,
166.037043263073));
#28894=CARTESIAN_POINT('Ctrl Pts',(-31.3249228143249,-33.5230977622533,
166.));
#28895=CARTESIAN_POINT('',(-33.666,-32.,166.));
#28896=CARTESIAN_POINT('Origin',(-32.,-32.,166.));
#28897=CARTESIAN_POINT('',(-33.666,-32.,165.));
#28898=CARTESIAN_POINT('',(-33.666,-32.,172.));
#28899=CARTESIAN_POINT('Origin',(-32.,-32.,165.));
#28900=CARTESIAN_POINT('',(-33.6146845439263,-32.4224457957945,166.));
#28901=CARTESIAN_POINT('Origin',(-32.,-32.,166.));
#28902=CARTESIAN_POINT('Ctrl Pts',(-33.6146867820777,-32.422446252051,166.));
#28903=CARTESIAN_POINT('Ctrl Pts',(-33.4771459066945,-32.9453079307942,
166.036314816837));
#28904=CARTESIAN_POINT('Ctrl Pts',(-33.0618726640047,-33.3962489478611,
166.072629633674));
#28905=CARTESIAN_POINT('Ctrl Pts',(-32.5515457289897,-33.5749074758773,
166.108944450512));
#28906=CARTESIAN_POINT('Ctrl Pts',(-32.0309820430471,-33.7571497513442,
166.145987713585));
#28907=CARTESIAN_POINT('Ctrl Pts',(-31.4115130155003,-33.6560764402868,
166.183030976658));
#28908=CARTESIAN_POINT('Ctrl Pts',(-30.9761439618779,-33.3177567144518,
166.220074239731));
#28909=CARTESIAN_POINT('Ctrl Pts',(-30.5407749082555,-32.9794369886167,
166.257117502805));
#28910=CARTESIAN_POINT('Ctrl Pts',(-30.2895058285574,-32.4038708480041,
166.294160765878));
#28911=CARTESIAN_POINT('Ctrl Pts',(-30.3375418344799,-31.8545228184461,
166.331204028951));
#28912=CARTESIAN_POINT('Ctrl Pts',(-30.3855778404025,-31.3051747888881,
166.368247292024));
#28913=CARTESIAN_POINT('Ctrl Pts',(-30.7329189319458,-30.7820448703847,
166.405290555098));
#28914=CARTESIAN_POINT('Ctrl Pts',(-31.2205128528787,-30.524470987755,166.442333818171));
#28915=CARTESIAN_POINT('Ctrl Pts',(-31.7081067738115,-30.2668971051253,
166.479377081244));
#28916=CARTESIAN_POINT('Ctrl Pts',(-32.3359535241339,-30.2748792583693,
166.516420344317));
#28917=CARTESIAN_POINT('Ctrl Pts',(-32.8168082811324,-30.5447862155172,
166.553463607391));
#28918=CARTESIAN_POINT('Ctrl Pts',(-33.2976630381309,-30.8146931726652,
166.590506870464));
#28919=CARTESIAN_POINT('Ctrl Pts',(-33.6315258018055,-31.3465249337172,
166.627550133537));
#28920=CARTESIAN_POINT('Ctrl Pts',(-33.6655960406503,-31.89690767857,166.66459339661));
#28921=CARTESIAN_POINT('Ctrl Pts',(-33.6677074511438,-31.9310161539537,
166.666889052204));
#28922=CARTESIAN_POINT('Ctrl Pts',(-33.66866748929,-31.965195875576,166.669184707797));
#28923=CARTESIAN_POINT('Ctrl Pts',(-33.6685050984025,-31.9993848812913,
166.67148036339));
#28924=CARTESIAN_POINT('Origin',(-32.,-32.,172.));
#28925=CARTESIAN_POINT('',(-33.6641555841304,-31.9988695272541,167.37148036339));
#28926=CARTESIAN_POINT('',(-33.6638025332639,-32.0008966213188,167.17851963661));
#28927=CARTESIAN_POINT('',(-33.666,-32.,172.));
#28928=CARTESIAN_POINT('Ctrl Pts',(-33.6638025332639,-32.0008966213188,
167.17851963661));
#28929=CARTESIAN_POINT('Ctrl Pts',(-33.6621591514203,-31.6647641050848,
167.156112388472));
#28930=CARTESIAN_POINT('Ctrl Pts',(-33.5633805945885,-31.3277436228238,
167.133705140335));
#28931=CARTESIAN_POINT('Ctrl Pts',(-33.374109387648,-31.053083959077,167.111297892197));
#28932=CARTESIAN_POINT('Ctrl Pts',(-33.061209603263,-30.5990215004767,167.074254629124));
#28933=CARTESIAN_POINT('Ctrl Pts',(-32.500992385075,-30.3153918625114,167.037211366051));
#28934=CARTESIAN_POINT('Ctrl Pts',(-31.9498062283038,-30.3319766798985,
167.000168102978));
#28935=CARTESIAN_POINT('Ctrl Pts',(-31.3986200715327,-30.3485614972856,
166.963124839904));
#28936=CARTESIAN_POINT('Ctrl Pts',(-30.8564649761784,-30.6653607700251,
166.926081576831));
#28937=CARTESIAN_POINT('Ctrl Pts',(-30.5714360458764,-31.1374205753515,
166.889038313758));
#28938=CARTESIAN_POINT('Ctrl Pts',(-30.2864071155743,-31.6094803806779,
166.851995050685));
#28939=CARTESIAN_POINT('Ctrl Pts',(-30.2585043503244,-32.2368007185912,
166.814951787611));
#28940=CARTESIAN_POINT('Ctrl Pts',(-30.5004798770101,-32.7322993685983,
166.777908524538));
#28941=CARTESIAN_POINT('Ctrl Pts',(-30.7424554036959,-33.2277980186054,
166.740865261465));
#28942=CARTESIAN_POINT('Ctrl Pts',(-31.2543092223174,-33.5914749807064,
166.703821998392));
#28943=CARTESIAN_POINT('Ctrl Pts',(-31.8018524330799,-33.6569621792094,
166.666778735318));
#28944=CARTESIAN_POINT('Ctrl Pts',(-32.3493956438423,-33.7224493777124,
166.629735472245));
#28945=CARTESIAN_POINT('Ctrl Pts',(-32.9326282467458,-33.4897468126174,
166.592692209172));
#28946=CARTESIAN_POINT('Ctrl Pts',(-33.2845997242085,-33.0652391014188,
166.555648946099));
#28947=CARTESIAN_POINT('Ctrl Pts',(-33.5288845123565,-32.770610749585,166.529939176269));
#28948=CARTESIAN_POINT('Ctrl Pts',(-33.6617704934304,-32.383589591023,166.504229406439));
#28949=CARTESIAN_POINT('Ctrl Pts',(-33.6648360717667,-31.9985292840412,
166.47851963661));
#28950=CARTESIAN_POINT('Ctrl Pts',(-33.6685050984025,-31.9993848812913,
166.67148036339));
#28951=CARTESIAN_POINT('Ctrl Pts',(-33.6660471100033,-32.5168780776586,
166.70622797087));
#28952=CARTESIAN_POINT('Ctrl Pts',(-33.4064339640194,-33.0364983148561,
166.74097557835));
#28953=CARTESIAN_POINT('Ctrl Pts',(-32.9900353939139,-33.3433730273871,
166.77572318583));
#28954=CARTESIAN_POINT('Ctrl Pts',(-32.5461267943179,-33.670521902698,166.812766448903));
#28955=CARTESIAN_POINT('Ctrl Pts',(-31.9240318811112,-33.7558859246661,
166.849809711976));
#28956=CARTESIAN_POINT('Ctrl Pts',(-31.4084114626267,-33.560400449204,166.88685297505));
#28957=CARTESIAN_POINT('Ctrl Pts',(-30.8927910441422,-33.3649149737418,
166.923896238123));
#28958=CARTESIAN_POINT('Ctrl Pts',(-30.48364512038,-32.8885800008494,166.960939501196));
#28959=CARTESIAN_POINT('Ctrl Pts',(-30.3681998158689,-32.3493650741656,
166.99798276427));
#28960=CARTESIAN_POINT('Ctrl Pts',(-30.2527545113577,-31.8101501474818,
167.035026027343));
#28961=CARTESIAN_POINT('Ctrl Pts',(-30.4310098260976,-31.2080552670066,
167.072069290416));
#28962=CARTESIAN_POINT('Ctrl Pts',(-30.8213955384865,-30.8185951748872,
167.109112553489));
#28963=CARTESIAN_POINT('Ctrl Pts',(-31.2117812508753,-30.4291350827678,
167.146155816562));
#28964=CARTESIAN_POINT('Ctrl Pts',(-31.8142973609132,-30.2523097790042,
167.183199079636));
#28965=CARTESIAN_POINT('Ctrl Pts',(-32.3532365279495,-30.3690338636197,
167.220242342709));
#28966=CARTESIAN_POINT('Ctrl Pts',(-32.8921756949857,-30.4857579482353,
167.257285605782));
#28967=CARTESIAN_POINT('Ctrl Pts',(-33.3675379190203,-30.8960314212301,
167.294328868855));
#28968=CARTESIAN_POINT('Ctrl Pts',(-33.561799648494,-31.4121152187214,167.331372131929));
#28969=CARTESIAN_POINT('Ctrl Pts',(-33.6319113122031,-31.5983767832275,
167.344741542416));
#28970=CARTESIAN_POINT('Ctrl Pts',(-33.6654072495738,-31.7984210409715,
167.358110952903));
#28971=CARTESIAN_POINT('Ctrl Pts',(-33.6641555841304,-31.9988695272541,
167.37148036339));
#28972=CARTESIAN_POINT('Origin',(-32.,-32.,172.));
#28973=CARTESIAN_POINT('',(-33.6644090960075,-32.0012498346086,168.07148036339));
#28974=CARTESIAN_POINT('',(-33.6681507572914,-32.0009136637507,167.87851963661));
#28975=CARTESIAN_POINT('',(-33.666,-32.,172.));
#28976=CARTESIAN_POINT('Ctrl Pts',(-33.6681507572914,-32.0009136637507,
167.87851963661));
#28977=CARTESIAN_POINT('Ctrl Pts',(-33.6648561918328,-31.5020077048909,
167.845038633578));
#28978=CARTESIAN_POINT('Ctrl Pts',(-33.4261730271947,-31.0003673015641,
167.811557630547));
#28979=CARTESIAN_POINT('Ctrl Pts',(-33.0352709879811,-30.6911682472265,
167.778076627516));
#28980=CARTESIAN_POINT('Ctrl Pts',(-32.6027783574323,-30.3490715095306,
167.741033364442));
#28981=CARTESIAN_POINT('Ctrl Pts',(-31.983952605973,-30.2425447512435,167.703990101369));
#28982=CARTESIAN_POINT('Ctrl Pts',(-31.461964987759,-30.4203339586322,167.666946838296));
#28983=CARTESIAN_POINT('Ctrl Pts',(-30.939977369545,-30.598123166021,167.629903575223));
#28984=CARTESIAN_POINT('Ctrl Pts',(-30.5148278845763,-31.0602283390857,
167.592860312149));
#28985=CARTESIAN_POINT('Ctrl Pts',(-30.3810627423918,-31.5951928206179,
167.555817049076));
#28986=CARTESIAN_POINT('Ctrl Pts',(-30.2472976002073,-32.1301573021501,
167.518773786003));
#28987=CARTESIAN_POINT('Ctrl Pts',(-30.404916800807,-32.7379810921499,167.48173052293));
#28988=CARTESIAN_POINT('Ctrl Pts',(-30.7817944276791,-33.1405269855266,
167.444687259856));
#28989=CARTESIAN_POINT('Ctrl Pts',(-31.1586720545513,-33.5430728789034,
167.407643996783));
#28990=CARTESIAN_POINT('Ctrl Pts',(-31.7548081076959,-33.7403408756571,
167.37060073371));
#28991=CARTESIAN_POINT('Ctrl Pts',(-32.2974144196609,-33.6420628913234,
167.333557470637));
#28992=CARTESIAN_POINT('Ctrl Pts',(-32.8400207316259,-33.5437849069897,
167.296514207564));
#28993=CARTESIAN_POINT('Ctrl Pts',(-33.3290973024113,-33.1499609415685,
167.25947094449));
#28994=CARTESIAN_POINT('Ctrl Pts',(-33.540844412513,-32.6408013192404,167.222427681417));
#28995=CARTESIAN_POINT('Ctrl Pts',(-33.6245069629724,-32.4396293052542,
167.207791666481));
#28996=CARTESIAN_POINT('Ctrl Pts',(-33.6648759609808,-32.2204523872831,
167.193155651546));
#28997=CARTESIAN_POINT('Ctrl Pts',(-33.6638025332639,-32.0008966213188,
167.17851963661));
#28998=CARTESIAN_POINT('Ctrl Pts',(-33.6641555841304,-31.9988695272541,
167.37148036339));
#28999=CARTESIAN_POINT('Ctrl Pts',(-33.6619392004519,-32.3538132190433,
167.395154215976));
#29000=CARTESIAN_POINT('Ctrl Pts',(-33.5507700631386,-32.7100243885523,
167.418828068562));
#29001=CARTESIAN_POINT('Ctrl Pts',(-33.341020485644,-32.9932222788685,167.442501921148));
#29002=CARTESIAN_POINT('Ctrl Pts',(-33.0128183584076,-33.4363514195366,
167.479545184222));
#29003=CARTESIAN_POINT('Ctrl Pts',(-32.4432528690221,-33.7007155788849,
167.516588447295));
#29004=CARTESIAN_POINT('Ctrl Pts',(-31.8929540065354,-33.6653431155281,
167.553631710368));
#29005=CARTESIAN_POINT('Ctrl Pts',(-31.3426551440488,-33.6299706521713,
167.590674973441));
#29006=CARTESIAN_POINT('Ctrl Pts',(-30.8116229084611,-33.2948615661094,
167.627718236515));
#29007=CARTESIAN_POINT('Ctrl Pts',(-30.5428548158509,-32.8133599755179,
167.664761499588));
#29008=CARTESIAN_POINT('Ctrl Pts',(-30.2740867232407,-32.3318583849265,
167.701804762661));
#29009=CARTESIAN_POINT('Ctrl Pts',(-30.267582773608,-31.7039642898055,167.738848025734));
#29010=CARTESIAN_POINT('Ctrl Pts',(-30.526319117194,-31.2169986148992,167.775891288808));
#29011=CARTESIAN_POINT('Ctrl Pts',(-30.78505546078,-30.7300329399929,167.812934551881));
#29012=CARTESIAN_POINT('Ctrl Pts',(-31.3090320975848,-30.3839956853014,
167.849977814954));
#29013=CARTESIAN_POINT('Ctrl Pts',(-31.8584801704804,-30.3372316264713,
167.887021078027));
#29014=CARTESIAN_POINT('Ctrl Pts',(-32.407928243376,-30.2904675676412,167.924064341101));
#29015=CARTESIAN_POINT('Ctrl Pts',(-32.9828477523625,-30.5429767046725,
167.961107604174));
#29016=CARTESIAN_POINT('Ctrl Pts',(-33.3201586422293,-30.9792122235664,
167.998150867247));
#29017=CARTESIAN_POINT('Ctrl Pts',(-33.542734764898,-31.2670642119921,168.022594032628));
#29018=CARTESIAN_POINT('Ctrl Pts',(-33.6618541900598,-31.6349121398867,
168.047037198009));
#29019=CARTESIAN_POINT('Ctrl Pts',(-33.6644090960075,-32.0012498346086,
168.07148036339));
#29020=CARTESIAN_POINT('Origin',(-32.,-32.,172.));
#29021=CARTESIAN_POINT('',(-33.6686518070233,-32.0004179215328,168.77148036339));
#29022=CARTESIAN_POINT('',(-33.666554187948,-31.9985209913767,168.57851963661));
#29023=CARTESIAN_POINT('',(-33.666,-32.,172.));
#29024=CARTESIAN_POINT('Ctrl Pts',(-33.666554187948,-31.9985209913767,168.57851963661));
#29025=CARTESIAN_POINT('Ctrl Pts',(-33.6675874565537,-31.8863118995242,
168.571008141758));
#29026=CARTESIAN_POINT('Ctrl Pts',(-33.6572223660562,-31.7742926181679,
168.563496646906));
#29027=CARTESIAN_POINT('Ctrl Pts',(-33.6347589832767,-31.6647543750453,
168.555985152054));
#29028=CARTESIAN_POINT('Ctrl Pts',(-33.5239798355562,-31.1245617720414,
168.51894188898));
#29029=CARTESIAN_POINT('Ctrl Pts',(-33.1189687606806,-30.6447083180542,
168.481898625907));
#29030=CARTESIAN_POINT('Ctrl Pts',(-32.6050566308058,-30.4447723522878,
168.444855362834));
#29031=CARTESIAN_POINT('Ctrl Pts',(-32.091144500931,-30.2448363865214,168.407812099761));
#29032=CARTESIAN_POINT('Ctrl Pts',(-31.4683313160572,-30.3248179089757,
168.370768836688));
#29033=CARTESIAN_POINT('Ctrl Pts',(-31.0216130117569,-30.6481178075245,
168.333725573614));
#29034=CARTESIAN_POINT('Ctrl Pts',(-30.5748947074566,-30.9714177060733,
168.296682310541));
#29035=CARTESIAN_POINT('Ctrl Pts',(-30.3042712837298,-31.5380359807166,
168.259639047468));
#29036=CARTESIAN_POINT('Ctrl Pts',(-30.3335785534306,-32.0886911836439,
168.222595784395));
#29037=CARTESIAN_POINT('Ctrl Pts',(-30.3628858231313,-32.6393463865712,
168.185552521321));
#29038=CARTESIAN_POINT('Ctrl Pts',(-30.6921237862596,-33.1740385177825,
168.148509258248));
#29039=CARTESIAN_POINT('Ctrl Pts',(-31.1706349329485,-33.4480953525865,
168.111465995175));
#29040=CARTESIAN_POINT('Ctrl Pts',(-31.6491460796373,-33.7221521873905,
168.074422732102));
#29041=CARTESIAN_POINT('Ctrl Pts',(-32.2769304098868,-33.7355737257871,
168.037379469028));
#29042=CARTESIAN_POINT('Ctrl Pts',(-32.7667172246232,-33.4822183541435,
168.000336205955));
#29043=CARTESIAN_POINT('Ctrl Pts',(-33.2565040393596,-33.2288629824998,
167.963292942882));
#29044=CARTESIAN_POINT('Ctrl Pts',(-33.6082933385829,-32.7087307008159,
167.926249679809));
#29045=CARTESIAN_POINT('Ctrl Pts',(-33.6611082333754,-32.1598312014215,
167.889206416735));
#29046=CARTESIAN_POINT('Ctrl Pts',(-33.666187170103,-32.107046360361,167.885644156694));
#29047=CARTESIAN_POINT('Ctrl Pts',(-33.6685012873779,-32.0539954892927,
167.882081896652));
#29048=CARTESIAN_POINT('Ctrl Pts',(-33.6681507572914,-32.0009136637507,
167.87851963661));
#29049=CARTESIAN_POINT('Ctrl Pts',(-33.6644090960075,-32.0012498346086,
168.07148036339));
#29050=CARTESIAN_POINT('Ctrl Pts',(-33.6657261130155,-32.1900916097992,
168.084080461082));
#29051=CARTESIAN_POINT('Ctrl Pts',(-33.6360689863127,-32.3785320778026,
168.096680558775));
#29052=CARTESIAN_POINT('Ctrl Pts',(-33.5736422385779,-32.5554067226683,
168.109280656467));
#29053=CARTESIAN_POINT('Ctrl Pts',(-33.3901126743126,-33.0754038021199,
168.14632391954));
#29054=CARTESIAN_POINT('Ctrl Pts',(-32.923351275035,-33.4954360602665,168.183367182613));
#29055=CARTESIAN_POINT('Ctrl Pts',(-32.386945524875,-33.6232990128118,168.220410445686));
#29056=CARTESIAN_POINT('Ctrl Pts',(-31.850539774715,-33.7511619653571,168.25745370876));
#29057=CARTESIAN_POINT('Ctrl Pts',(-31.2444896736727,-33.586855612301,168.294496971833));
#29058=CARTESIAN_POINT('Ctrl Pts',(-30.8461204624394,-33.2055656501328,
168.331540234906));
#29059=CARTESIAN_POINT('Ctrl Pts',(-30.4477512512061,-32.8242756879646,
168.36858349798));
#29060=CARTESIAN_POINT('Ctrl Pts',(-30.2570629297819,-32.2260021166843,
168.405626761053));
#29061=CARTESIAN_POINT('Ctrl Pts',(-30.3613134397796,-31.6845116783861,
168.442670024126));
#29062=CARTESIAN_POINT('Ctrl Pts',(-30.4655639497772,-31.1430212400879,
168.479713287199));
#29063=CARTESIAN_POINT('Ctrl Pts',(-30.8647532911966,-30.6583139347719,
168.516756550272));
#29064=CARTESIAN_POINT('Ctrl Pts',(-31.376214586069,-30.4521891971938,168.553799813346));
#29065=CARTESIAN_POINT('Ctrl Pts',(-31.8876758809413,-30.2460644596156,
168.590843076419));
#29066=CARTESIAN_POINT('Ctrl Pts',(-32.5114091292667,-30.3185222897753,
168.627886339492));
#29067=CARTESIAN_POINT('Ctrl Pts',(-32.96199737859,-30.6364063774491,168.664929602565));
#29068=CARTESIAN_POINT('Ctrl Pts',(-33.3940194414518,-30.9411922645955,
168.70044652284));
#29069=CARTESIAN_POINT('Ctrl Pts',(-33.6668711873007,-31.4715958446407,
168.735963443115));
#29070=CARTESIAN_POINT('Ctrl Pts',(-33.6686518070233,-32.0004179215328,
168.77148036339));
#29071=CARTESIAN_POINT('Origin',(-32.,-32.,172.));
#29072=CARTESIAN_POINT('',(-33.665635320795,-31.9984849817919,169.47148036339));
#29073=CARTESIAN_POINT('',(-33.6633165634872,-32.0000156713784,169.27851963661));
#29074=CARTESIAN_POINT('',(-33.666,-32.,172.));
#29075=CARTESIAN_POINT('Ctrl Pts',(-33.6633165634872,-32.0000156713784,
169.27851963661));
#29076=CARTESIAN_POINT('Ctrl Pts',(-33.6632931527355,-31.7210138399623,
169.259934386864));
#29077=CARTESIAN_POINT('Ctrl Pts',(-33.5968742643497,-31.4420015340208,
169.241349137118));
#29078=CARTESIAN_POINT('Ctrl Pts',(-33.4641220642516,-31.199267121124,169.222763887372));
#29079=CARTESIAN_POINT('Ctrl Pts',(-33.199526498466,-30.7154600786147,169.185720624299));
#29080=CARTESIAN_POINT('Ctrl Pts',(-32.6714110739412,-30.3757728607261,
169.148677361226));
#29081=CARTESIAN_POINT('Ctrl Pts',(-32.1214385453584,-30.3356444964945,
169.111634098152));
#29082=CARTESIAN_POINT('Ctrl Pts',(-31.5714660167756,-30.2955161322629,
169.074590835079));
#29083=CARTESIAN_POINT('Ctrl Pts',(-30.9996363841348,-30.5549466216884,
169.037547572006));
#29084=CARTESIAN_POINT('Ctrl Pts',(-30.6676157867046,-30.9952219794971,
169.000504308933));
#29085=CARTESIAN_POINT('Ctrl Pts',(-30.3355951892744,-31.4354973373059,
168.96346104586));
#29086=CARTESIAN_POINT('Ctrl Pts',(-30.2433836270549,-32.0566175634979,
168.926417782786));
#29087=CARTESIAN_POINT('Ctrl Pts',(-30.4331766109431,-32.5743614104843,
168.889374519713));
#29088=CARTESIAN_POINT('Ctrl Pts',(-30.6229695948312,-33.0921052574707,
168.85233125664));
#29089=CARTESIAN_POINT('Ctrl Pts',(-31.0947671248271,-33.5064727252516,
168.815287993566));
#29090=CARTESIAN_POINT('Ctrl Pts',(-31.6326772093758,-33.6278515073184,
168.778244730493));
#29091=CARTESIAN_POINT('Ctrl Pts',(-32.1705872939245,-33.7492302893852,
168.74120146742));
#29092=CARTESIAN_POINT('Ctrl Pts',(-32.7746099330261,-33.577620385738,168.704158204347));
#29093=CARTESIAN_POINT('Ctrl Pts',(-33.1683476422943,-33.1915495579041,
168.667114941273));
#29094=CARTESIAN_POINT('Ctrl Pts',(-33.4822446860581,-32.8837647339262,
168.637583173052));
#29095=CARTESIAN_POINT('Ctrl Pts',(-33.6624918475518,-32.4396759090301,
168.608051404831));
#29096=CARTESIAN_POINT('Ctrl Pts',(-33.666554187948,-31.9985209913767,168.57851963661));
#29097=CARTESIAN_POINT('Ctrl Pts',(-33.6686518070233,-32.0004179215328,
168.77148036339));
#29098=CARTESIAN_POINT('Ctrl Pts',(-33.6687283293138,-32.0231440971812,
168.773006706188));
#29099=CARTESIAN_POINT('Ctrl Pts',(-33.6683042216595,-32.0458673520174,
168.774533048987));
#29100=CARTESIAN_POINT('Ctrl Pts',(-33.6673706026167,-32.0685696534919,
168.776059391785));
#29101=CARTESIAN_POINT('Ctrl Pts',(-33.6447123269988,-32.6195384966732,
168.813102654858));
#29102=CARTESIAN_POINT('Ctrl Pts',(-33.3219525254415,-33.1581658378479,
168.850145917932));
#29103=CARTESIAN_POINT('Ctrl Pts',(-32.8467843330275,-33.4379787262727,
168.887189181005));
#29104=CARTESIAN_POINT('Ctrl Pts',(-32.3716161406135,-33.7177916146976,
168.924232444078));
#29105=CARTESIAN_POINT('Ctrl Pts',(-31.7440395573428,-33.7387900503725,
168.961275707151));
#29106=CARTESIAN_POINT('Ctrl Pts',(-31.2512302248365,-33.4913652629953,
168.998318970225));
#29107=CARTESIAN_POINT('Ctrl Pts',(-30.7584208923303,-33.2439404756181,
169.035362233298));
#29108=CARTESIAN_POINT('Ctrl Pts',(-30.4003788105884,-32.728092465189,169.072405496371));
#29109=CARTESIAN_POINT('Ctrl Pts',(-30.3409420948093,-32.179870484209,169.109448759444));
#29110=CARTESIAN_POINT('Ctrl Pts',(-30.2815053790303,-31.6316485032291,
169.146492022518));
#29111=CARTESIAN_POINT('Ctrl Pts',(-30.5206740292141,-31.0510525516985,
169.183535285591));
#29112=CARTESIAN_POINT('Ctrl Pts',(-30.9490057678768,-30.703760188888,169.220578548664));
#29113=CARTESIAN_POINT('Ctrl Pts',(-31.3773375065395,-30.3564678260775,
169.257621811737));
#29114=CARTESIAN_POINT('Ctrl Pts',(-31.9948323336809,-30.2424790519871,
169.294665074811));
#29115=CARTESIAN_POINT('Ctrl Pts',(-32.5189279646265,-30.4139545115617,
169.331708337884));
#29116=CARTESIAN_POINT('Ctrl Pts',(-33.0430235955722,-30.5854299711363,
169.368751600957));
#29117=CARTESIAN_POINT('Ctrl Pts',(-33.473720030322,-31.042369664376,169.40579486403));
#29118=CARTESIAN_POINT('Ctrl Pts',(-33.613932915689,-31.5756804653068,169.442838127103));
#29119=CARTESIAN_POINT('Ctrl Pts',(-33.6500709361183,-31.713134284681,169.452385539199));
#29120=CARTESIAN_POINT('Ctrl Pts',(-33.6669126403244,-31.8556613037164,
169.461932951295));
#29121=CARTESIAN_POINT('Ctrl Pts',(-33.665635320795,-31.9984849817919,169.47148036339));
#29122=CARTESIAN_POINT('Origin',(-32.,-32.,172.));
#29123=CARTESIAN_POINT('',(-33.6634609252252,-32.0005076151317,170.17148036339));
#29124=CARTESIAN_POINT('',(-33.6666117016187,-32.001470779109,169.97851963661));
#29125=CARTESIAN_POINT('',(-33.666,-32.,172.));
#29126=CARTESIAN_POINT('Ctrl Pts',(-33.6666117016187,-32.001470779109,169.97851963661));
#29127=CARTESIAN_POINT('Ctrl Pts',(-33.6625394733438,-31.5584545014678,
169.94886063197));
#29128=CARTESIAN_POINT('Ctrl Pts',(-33.4805649727493,-31.1124834122679,
169.91920162733));
#29129=CARTESIAN_POINT('Ctrl Pts',(-33.1642582886333,-30.8044544342897,
169.88954262269));
#29130=CARTESIAN_POINT('Ctrl Pts',(-32.7692001316305,-30.4197348995646,
169.852499359617));
#29131=CARTESIAN_POINT('Ctrl Pts',(-32.1645930666198,-30.2501955101854,
169.815456096544));
#29132=CARTESIAN_POINT('Ctrl Pts',(-31.6271020082049,-30.373416571443,169.778412833471));
#29133=CARTESIAN_POINT('Ctrl Pts',(-31.0896109497899,-30.4966376327006,
169.741369570397));
#29134=CARTESIAN_POINT('Ctrl Pts',(-30.6192358979707,-30.912619144595,169.704326307324));
#29135=CARTESIAN_POINT('Ctrl Pts',(-30.4312179259571,-31.431010222849,169.667283044251));
#29136=CARTESIAN_POINT('Ctrl Pts',(-30.2431999539434,-31.949401301103,169.630239781178));
#29137=CARTESIAN_POINT('Ctrl Pts',(-30.3375390617353,-32.5702019457165,
169.593196518104));
#29138=CARTESIAN_POINT('Ctrl Pts',(-30.6710661851401,-33.0093371478662,
169.556153255031));
#29139=CARTESIAN_POINT('Ctrl Pts',(-31.0045933085448,-33.4484723500159,
169.519109991958));
#29140=CARTESIAN_POINT('Ctrl Pts',(-31.5773084475623,-33.7059421097018,
169.482066728885));
#29141=CARTESIAN_POINT('Ctrl Pts',(-32.1271402599961,-33.6639296609623,
169.445023465812));
#29142=CARTESIAN_POINT('Ctrl Pts',(-32.6769720724299,-33.6219172122228,
169.407980202738));
#29143=CARTESIAN_POINT('Ctrl Pts',(-33.20392055828,-33.2804225550579,169.370936939665));
#29144=CARTESIAN_POINT('Ctrl Pts',(-33.4668569476818,-32.7957117929105,
169.333893676592));
#29145=CARTESIAN_POINT('Ctrl Pts',(-33.5978735746518,-32.5541888555298,
169.315435663264));
#29146=CARTESIAN_POINT('Ctrl Pts',(-33.6633398139666,-32.2771074292527,
169.296977649937));
#29147=CARTESIAN_POINT('Ctrl Pts',(-33.6633165634872,-32.0000156713784,
169.27851963661));
#29148=CARTESIAN_POINT('Ctrl Pts',(-33.665635320795,-31.9984849817919,169.47148036339));
#29149=CARTESIAN_POINT('Ctrl Pts',(-33.6619567336469,-32.4098067650291,
169.498976214368));
#29150=CARTESIAN_POINT('Ctrl Pts',(-33.5079993225544,-32.8235890324679,
169.526472065346));
#29151=CARTESIAN_POINT('Ctrl Pts',(-33.2318839646868,-33.1257390556495,
169.553967916323));
#29152=CARTESIAN_POINT('Ctrl Pts',(-32.8598927923331,-33.5328049364395,
169.591011179397));
#29153=CARTESIAN_POINT('Ctrl Pts',(-32.2661811116412,-33.7372547893976,
169.62805444247));
#29154=CARTESIAN_POINT('Ctrl Pts',(-31.7224281684284,-33.6455334703934,
169.665097705543));
#29155=CARTESIAN_POINT('Ctrl Pts',(-31.1786752252156,-33.5538121513892,
169.702140968616));
#29156=CARTESIAN_POINT('Ctrl Pts',(-30.6848810194818,-33.1659196604227,
169.739184231689));
#29157=CARTESIAN_POINT('Ctrl Pts',(-30.4670031022832,-32.6593534981007,
169.776227494763));
#29158=CARTESIAN_POINT('Ctrl Pts',(-30.2491251850846,-32.1527873357787,
169.813270757836));
#29159=CARTESIAN_POINT('Ctrl Pts',(-30.3071635564212,-31.5275475021012,
169.850314020909));
#29160=CARTESIAN_POINT('Ctrl Pts',(-30.6145601722693,-31.0697403547372,
169.887357283982));
#29161=CARTESIAN_POINT('Ctrl Pts',(-30.9219567881174,-30.6119332073732,
169.924400547056));
#29162=CARTESIAN_POINT('Ctrl Pts',(-31.4787116484771,-30.3215587463227,
169.961443810129));
#29163=CARTESIAN_POINT('Ctrl Pts',(-32.0300567481252,-30.3314907504724,
169.998487073202));
#29164=CARTESIAN_POINT('Ctrl Pts',(-32.5814018477734,-30.3414227546222,
170.035530336275));
#29165=CARTESIAN_POINT('Ctrl Pts',(-33.12733718671,-30.6516612239722,170.072573599349));
#29166=CARTESIAN_POINT('Ctrl Pts',(-33.4180457140488,-31.1202427171459,
170.109616862422));
#29167=CARTESIAN_POINT('Ctrl Pts',(-33.5798767351351,-31.3810916925667,
170.130238029411));
#29168=CARTESIAN_POINT('Ctrl Pts',(-33.66261543862,-31.6910096378651,170.150859196401));
#29169=CARTESIAN_POINT('Ctrl Pts',(-33.6634609252252,-32.0005076151317,
170.17148036339));
#29170=CARTESIAN_POINT('Origin',(-32.,-32.,172.));
#29171=CARTESIAN_POINT('',(-33.6674948610292,-32.0012453678407,170.87148036339));
#29172=CARTESIAN_POINT('',(-33.6681095677655,-31.9990590647821,170.67851963661));
#29173=CARTESIAN_POINT('',(-33.666,-32.,172.));
#29174=CARTESIAN_POINT('Ctrl Pts',(-33.6681095677655,-31.9990590647821,
170.67851963661));
#29175=CARTESIAN_POINT('Ctrl Pts',(-33.668481259833,-31.9440776933425,170.674830140149));
#29176=CARTESIAN_POINT('Ctrl Pts',(-33.6659984917278,-31.8891303002658,
170.671140643689));
#29177=CARTESIAN_POINT('Ctrl Pts',(-33.6605508651237,-31.8344784404443,
170.667451147228));
#29178=CARTESIAN_POINT('Ctrl Pts',(-33.6058556329738,-31.2857631231863,
170.630407884155));
#29179=CARTESIAN_POINT('Ctrl Pts',(-33.2522863246199,-30.7668391867544,
170.593364621082));
#29180=CARTESIAN_POINT('Ctrl Pts',(-32.7616343384148,-30.515163410712,170.556321358009));
#29181=CARTESIAN_POINT('Ctrl Pts',(-32.2709823522098,-30.2634876346696,
170.519278094936));
#29182=CARTESIAN_POINT('Ctrl Pts',(-31.6432476881537,-30.2790600190167,
170.482234831862));
#29183=CARTESIAN_POINT('Ctrl Pts',(-31.1656783247691,-30.5547547251138,
170.445191568789));
#29184=CARTESIAN_POINT('Ctrl Pts',(-30.6881089613846,-30.8304494312109,
170.408148305716));
#29185=CARTESIAN_POINT('Ctrl Pts',(-30.3607048986715,-31.3662664590579,
170.371105042643));
#29186=CARTESIAN_POINT('Ctrl Pts',(-30.3332844604529,-31.917018842059,170.334061779569));
#29187=CARTESIAN_POINT('Ctrl Pts',(-30.3058640222343,-32.4677712250601,
170.297018516496));
#29188=CARTESIAN_POINT('Ctrl Pts',(-30.5784272085101,-33.0334589632152,
170.259975253423));
#29189=CARTESIAN_POINT('Ctrl Pts',(-31.0262505831528,-33.3552264148587,
170.22293199035));
#29190=CARTESIAN_POINT('Ctrl Pts',(-31.4740739577955,-33.6769938665021,
170.185888727276));
#29191=CARTESIAN_POINT('Ctrl Pts',(-32.0971575208052,-33.7548410316338,
170.148845464203));
#29192=CARTESIAN_POINT('Ctrl Pts',(-32.6103816122786,-33.5531454695981,
170.11180220113));
#29193=CARTESIAN_POINT('Ctrl Pts',(-33.1236057037519,-33.3514499075625,
170.074758938057));
#29194=CARTESIAN_POINT('Ctrl Pts',(-33.5269703236889,-32.8702116183596,
170.037715674983));
#29195=CARTESIAN_POINT('Ctrl Pts',(-33.6358980091599,-32.3296426337226,
170.00067241191));
#29196=CARTESIAN_POINT('Ctrl Pts',(-33.6576118138667,-32.2218848188732,
169.993288153477));
#29197=CARTESIAN_POINT('Ctrl Pts',(-33.6676255719879,-32.1117693789459,
169.985903895043));
#29198=CARTESIAN_POINT('Ctrl Pts',(-33.6666117016187,-32.001470779109,169.97851963661));
#29199=CARTESIAN_POINT('Ctrl Pts',(-33.6634609252252,-32.0005076151317,
170.17148036339));
#29200=CARTESIAN_POINT('Ctrl Pts',(-33.6641342461035,-32.2469827793654,
170.187902459474));
#29201=CARTESIAN_POINT('Ctrl Pts',(-33.6128703552766,-32.4931915971372,
170.204324555558));
#29202=CARTESIAN_POINT('Ctrl Pts',(-33.5082546205404,-32.714139008517,170.220746651642));
#29203=CARTESIAN_POINT('Ctrl Pts',(-33.2722732839521,-33.2125292897169,
170.257789914715));
#29204=CARTESIAN_POINT('Ctrl Pts',(-32.7648288950345,-33.5823853351191,
170.294833177788));
#29205=CARTESIAN_POINT('Ctrl Pts',(-32.2181252546536,-33.6544630238084,
170.331876440861));
#29206=CARTESIAN_POINT('Ctrl Pts',(-31.6714216142728,-33.7265407124978,
170.368919703935));
#29207=CARTESIAN_POINT('Ctrl Pts',(-31.0854587224287,-33.5008400444744,
170.405962967008));
#29208=CARTESIAN_POINT('Ctrl Pts',(-30.7283700211778,-33.0806404216147,
170.443006230081));
#29209=CARTESIAN_POINT('Ctrl Pts',(-30.3712813199269,-32.6604407987551,
170.480049493154));
#29210=CARTESIAN_POINT('Ctrl Pts',(-30.2430668092691,-32.0457422210593,
170.517092756228));
#29211=CARTESIAN_POINT('Ctrl Pts',(-30.4023967540672,-31.5178274246166,
170.554136019301));
#29212=CARTESIAN_POINT('Ctrl Pts',(-30.5617266988653,-30.989912628174,170.591179282374));
#29213=CARTESIAN_POINT('Ctrl Pts',(-31.0086010991193,-30.5487816129845,
170.628222545447));
#29214=CARTESIAN_POINT('Ctrl Pts',(-31.5385326523485,-30.3962935396656,
170.66526580852));
#29215=CARTESIAN_POINT('Ctrl Pts',(-32.0684642055777,-30.2438054663466,
170.702309071594));
#29216=CARTESIAN_POINT('Ctrl Pts',(-32.6814529117821,-30.3799603348982,
170.739352334667));
#29217=CARTESIAN_POINT('Ctrl Pts',(-33.0969984627955,-30.7424544157402,
170.77639559774));
#29218=CARTESIAN_POINT('Ctrl Pts',(-33.4525471560164,-31.0526112599884,
170.808090519624));
#29219=CARTESIAN_POINT('Ctrl Pts',(-33.6635508796099,-31.528467414169,170.839785441507));
#29220=CARTESIAN_POINT('Ctrl Pts',(-33.6674948610292,-32.0012453678407,
170.87148036339));
#29221=CARTESIAN_POINT('Origin',(-32.,-32.,172.));
#29222=CARTESIAN_POINT('',(-33.6673390318703,-31.9986999066965,171.57148036339));
#29223=CARTESIAN_POINT('',(-33.6637722109972,-31.999128635268,171.37851963661));
#29224=CARTESIAN_POINT('',(-33.666,-32.,172.));
#29225=CARTESIAN_POINT('Ctrl Pts',(-33.6637722109972,-31.999128635268,171.37851963661));
#29226=CARTESIAN_POINT('Ctrl Pts',(-33.6648226268342,-31.7776542933398,
171.363756385255));
#29227=CARTESIAN_POINT('Ctrl Pts',(-33.6237243170056,-31.5565539606062,
171.348993133901));
#29228=CARTESIAN_POINT('Ctrl Pts',(-33.5386395965288,-31.3539235692779,
171.334229882547));
#29229=CARTESIAN_POINT('Ctrl Pts',(-33.3251489765771,-30.8454928237421,
171.297186619474));
#29230=CARTESIAN_POINT('Ctrl Pts',(-32.8347264675265,-30.4533460779589,
171.2601433564));
#29231=CARTESIAN_POINT('Ctrl Pts',(-32.2917867503132,-30.3569275564715,
171.223100093327));
#29232=CARTESIAN_POINT('Ctrl Pts',(-31.7488470330999,-30.2605090349842,
171.186056830254));
#29233=CARTESIAN_POINT('Ctrl Pts',(-31.1533901077238,-30.4598187377927,
171.149013567181));
#29234=CARTESIAN_POINT('Ctrl Pts',(-30.7778938345064,-30.8636536256037,
171.111970304108));
#29235=CARTESIAN_POINT('Ctrl Pts',(-30.4023975612891,-31.2674885134147,
171.074927041034));
#29236=CARTESIAN_POINT('Ctrl Pts',(-30.2468619402303,-31.8758485862283,
171.037883777961));
#29237=CARTESIAN_POINT('Ctrl Pts',(-30.3824592281699,-32.4103515734201,
171.000840514888));
#29238=CARTESIAN_POINT('Ctrl Pts',(-30.5180565161095,-32.9448545606118,
170.963797251814));
#29239=CARTESIAN_POINT('Ctrl Pts',(-30.9447867130474,-33.4055004621818,
170.926753988741));
#29240=CARTESIAN_POINT('Ctrl Pts',(-31.467380394713,-33.5815002113199,170.889710725668));
#29241=CARTESIAN_POINT('Ctrl Pts',(-31.9899740763786,-33.757499960458,170.852667462595));
#29242=CARTESIAN_POINT('Ctrl Pts',(-32.6084312427719,-33.6488535571644,
170.815624199522));
#29243=CARTESIAN_POINT('Ctrl Pts',(-33.0397492479957,-33.3052770064754,
170.778580936448));
#29244=CARTESIAN_POINT('Ctrl Pts',(-33.4281081259296,-32.9959205639111,
170.745227169835));
#29245=CARTESIAN_POINT('Ctrl Pts',(-33.6647493990804,-32.4961013714264,
170.711873403223));
#29246=CARTESIAN_POINT('Ctrl Pts',(-33.6681095677655,-31.9990590647821,
170.67851963661));
#29247=CARTESIAN_POINT('Ctrl Pts',(-33.6674948610292,-32.0012453678407,
170.87148036339));
#29248=CARTESIAN_POINT('Ctrl Pts',(-33.6681603858837,-32.0810240091201,
170.87682870458));
#29249=CARTESIAN_POINT('Ctrl Pts',(-33.6629299510325,-32.1607149996279,
170.88217704577));
#29250=CARTESIAN_POINT('Ctrl Pts',(-33.651503176545,-32.2395073730154,170.88752538696));
#29251=CARTESIAN_POINT('Ctrl Pts',(-33.5723599434589,-32.7852329563164,
170.924568650033));
#29252=CARTESIAN_POINT('Ctrl Pts',(-33.1959710814645,-33.2878508297859,
170.961611913106));
#29253=CARTESIAN_POINT('Ctrl Pts',(-32.6945700929267,-33.5173657798562,
170.99865517618));
#29254=CARTESIAN_POINT('Ctrl Pts',(-32.193169104389,-33.7468807299266,171.035698439253));
#29255=CARTESIAN_POINT('Ctrl Pts',(-31.5667559893079,-33.7032927565979,
171.072741702326));
#29256=CARTESIAN_POINT('Ctrl Pts',(-31.1019739925609,-33.4065474801193,
171.109784965399));
#29257=CARTESIAN_POINT('Ctrl Pts',(-30.6371919958139,-33.1098022036407,
171.146828228473));
#29258=CARTESIAN_POINT('Ctrl Pts',(-30.334041117401,-32.5598996240123,171.183871491546));
#29259=CARTESIAN_POINT('Ctrl Pts',(-30.3312415555168,-32.0084721799494,
171.220914754619));
#29260=CARTESIAN_POINT('Ctrl Pts',(-30.3284419936326,-31.4570447358866,
171.257958017692));
#29261=CARTESIAN_POINT('Ctrl Pts',(-30.625993748277,-30.9040924273892,171.295001280766));
#29262=CARTESIAN_POINT('Ctrl Pts',(-31.087738749932,-30.6026432325668,171.332044543839));
#29263=CARTESIAN_POINT('Ctrl Pts',(-31.549483751587,-30.3011940377444,171.369087806912));
#29264=CARTESIAN_POINT('Ctrl Pts',(-32.1754220002525,-30.2512479565968,
171.406131069985));
#29265=CARTESIAN_POINT('Ctrl Pts',(-32.6791275473481,-30.4756600450359,
171.443174333058));
#29266=CARTESIAN_POINT('Ctrl Pts',(-33.1828330944437,-30.700072133475,171.480217596132));
#29267=CARTESIAN_POINT('Ctrl Pts',(-33.5643059399693,-31.1988423915007,
171.517260859205));
#29268=CARTESIAN_POINT('Ctrl Pts',(-33.6489861782628,-31.7437362535097,
171.554304122278));
#29269=CARTESIAN_POINT('Ctrl Pts',(-33.6620743718116,-31.8279551512505,
171.560029535982));
#29270=CARTESIAN_POINT('Ctrl Pts',(-33.6680725307781,-31.9132758889271,
171.565754949686));
#29271=CARTESIAN_POINT('Ctrl Pts',(-33.6673390318703,-31.9986999066965,
171.57148036339));
#29272=CARTESIAN_POINT('Origin',(-32.,-32.,172.));
#29273=CARTESIAN_POINT('',(-33.6634139074877,-31.999580988466,172.27148036339));
#29274=CARTESIAN_POINT('',(-33.6649323450731,-32.0014151634909,172.07851963661));
#29275=CARTESIAN_POINT('',(-33.666,-32.,172.));
#29276=CARTESIAN_POINT('Ctrl Pts',(-33.6649323450731,-32.0014151634909,
172.07851963661));
#29277=CARTESIAN_POINT('Ctrl Pts',(-33.6618075747334,-31.6144944764027,
172.052682630362));
#29278=CARTESIAN_POINT('Ctrl Pts',(-33.5274443578025,-31.22561670968,172.026845624113));
#29279=CARTESIAN_POINT('Ctrl Pts',(-33.2809243786464,-30.9303929232983,
172.001008617865));
#29280=CARTESIAN_POINT('Ctrl Pts',(-32.9274815550867,-30.5071220427884,
171.963965354792));
#29281=CARTESIAN_POINT('Ctrl Pts',(-32.3434916893401,-30.2763642816683,
171.926922091719));
#29282=CARTESIAN_POINT('Ctrl Pts',(-31.796185377419,-30.3437131401949,171.889878828646));
#29283=CARTESIAN_POINT('Ctrl Pts',(-31.2488790654979,-30.4110619987214,
171.852835565572));
#29284=CARTESIAN_POINT('Ctrl Pts',(-30.7382563074024,-30.7765174768945,
171.815792302499));
#29285=CARTESIAN_POINT('Ctrl Pts',(-30.4979753085002,-31.272849129502,171.778749039426));
#29286=CARTESIAN_POINT('Ctrl Pts',(-30.2576943095981,-31.7691807821095,
171.741705776353));
#29287=CARTESIAN_POINT('Ctrl Pts',(-30.2877550698894,-32.3963886091514,
171.704662513279));
#29288=CARTESIAN_POINT('Ctrl Pts',(-30.5744019484625,-32.8674657098661,
171.667619250206));
#29289=CARTESIAN_POINT('Ctrl Pts',(-30.8610488270356,-33.3385428105808,
171.630575987133));
#29290=CARTESIAN_POINT('Ctrl Pts',(-31.4042818238906,-33.6534891849684,
171.59353272406));
#29291=CARTESIAN_POINT('Ctrl Pts',(-31.9555204652248,-33.6681870798346,
171.556489460986));
#29292=CARTESIAN_POINT('Ctrl Pts',(-32.506759106559,-33.6828849747009,171.519446197913));
#29293=CARTESIAN_POINT('Ctrl Pts',(-33.0660033923725,-33.3973343900459,
171.48240293484));
#29294=CARTESIAN_POINT('Ctrl Pts',(-33.3773461698529,-32.9422017250741,
171.445359671767));
#29295=CARTESIAN_POINT('Ctrl Pts',(-33.5646061506259,-32.6684579922612,
171.423079660048));
#29296=CARTESIAN_POINT('Ctrl Pts',(-33.6621869723126,-32.3333674025406,
171.400799648329));
#29297=CARTESIAN_POINT('Ctrl Pts',(-33.6637722109972,-31.999128635268,171.37851963661));
#29298=CARTESIAN_POINT('Ctrl Pts',(-33.6673390318703,-31.9986999066965,
171.57148036339));
#29299=CARTESIAN_POINT('Ctrl Pts',(-33.6633268138032,-32.4659668430872,
171.60279821276));
#29300=CARTESIAN_POINT('Ctrl Pts',(-33.4578994378697,-32.9363239805219,
171.634116062129));
#29301=CARTESIAN_POINT('Ctrl Pts',(-33.1097105413418,-33.2463422637068,
171.665433911498));
#29302=CARTESIAN_POINT('Ctrl Pts',(-32.697867035066,-33.6130369459029,171.702477174571));
#29303=CARTESIAN_POINT('Ctrl Pts',(-32.0862923914529,-33.7554088443029,
171.739520437645));
#29304=CARTESIAN_POINT('Ctrl Pts',(-31.5548398512946,-33.6083093501785,
171.776563700718));
#29305=CARTESIAN_POINT('Ctrl Pts',(-31.0233873111362,-33.4612098560541,
171.813606963791));
#29306=CARTESIAN_POINT('Ctrl Pts',(-30.5720568744324,-33.0246389694052,
171.850650226864));
#29307=CARTESIAN_POINT('Ctrl Pts',(-30.4073749017817,-32.4983691607554,
171.887693489938));
#29308=CARTESIAN_POINT('Ctrl Pts',(-30.2426929291309,-31.9720993521056,
171.924736753011));
#29309=CARTESIAN_POINT('Ctrl Pts',(-30.364659420533,-31.3561306214548,171.961780016084));
#29310=CARTESIAN_POINT('Ctrl Pts',(-30.7174631708582,-30.9323269199975,
171.998823279157));
#29311=CARTESIAN_POINT('Ctrl Pts',(-31.0702669211834,-30.5085232185402,
172.035866542231));
#29312=CARTESIAN_POINT('Ctrl Pts',(-31.6539079304317,-30.2768845462763,
172.072909805304));
#29313=CARTESIAN_POINT('Ctrl Pts',(-32.2013152374326,-30.3434075036254,
172.109953068377));
#29314=CARTESIAN_POINT('Ctrl Pts',(-32.7487225444335,-30.4099304609746,
172.14699633145));
#29315=CARTESIAN_POINT('Ctrl Pts',(-33.259896149187,-30.7746150479367,172.184039594523));
#29316=CARTESIAN_POINT('Ctrl Pts',(-33.5009257818815,-31.2705835749378,
172.221082857597));
#29317=CARTESIAN_POINT('Ctrl Pts',(-33.6102330377975,-31.4955059552325,
172.237882026195));
#29318=CARTESIAN_POINT('Ctrl Pts',(-33.6639815538493,-31.7474286428721,
172.254681194792));
#29319=CARTESIAN_POINT('Ctrl Pts',(-33.6634139074877,-31.999580988466,172.27148036339));
#29320=CARTESIAN_POINT('Origin',(-32.,-32.,172.));
#29321=CARTESIAN_POINT('',(-33.6658031255686,-32.0015218482784,172.97148036339));
#29322=CARTESIAN_POINT('',(-33.6687793242584,-32.0000368508118,172.77851963661));
#29323=CARTESIAN_POINT('',(-33.666,-32.,172.));
#29324=CARTESIAN_POINT('Ctrl Pts',(-33.6687789306113,-32.0000368455925,
172.77851963661));
#29325=CARTESIAN_POINT('Ctrl Pts',(-33.6686001379207,-31.4505738269769,
172.741608875468));
#29326=CARTESIAN_POINT('Ctrl Pts',(-33.3706978307467,-30.9009446699073,
172.704698114326));
#29327=CARTESIAN_POINT('Ctrl Pts',(-32.9101517626888,-30.6012683133584,
172.667787353184));
#29328=CARTESIAN_POINT('Ctrl Pts',(-32.4479524303382,-30.300516181216,172.63074409011));
#29329=CARTESIAN_POINT('Ctrl Pts',(-31.8219395268455,-30.2515146274405,
172.593700827037));
#29330=CARTESIAN_POINT('Ctrl Pts',(-31.3185731624352,-30.4766864973396,
172.556657563964));
#29331=CARTESIAN_POINT('Ctrl Pts',(-30.8152067980249,-30.7018583672388,
172.519614300891));
#29332=CARTESIAN_POINT('Ctrl Pts',(-30.4344869726971,-31.2012036608125,
172.482571037817));
#29333=CARTESIAN_POINT('Ctrl Pts',(-30.3506290141545,-31.7462246793086,
172.445527774744));
#29334=CARTESIAN_POINT('Ctrl Pts',(-30.2667710556119,-32.2912456978048,
172.408484511671));
#29335=CARTESIAN_POINT('Ctrl Pts',(-30.4797749638545,-32.8819424412233,
172.371441248598));
#29336=CARTESIAN_POINT('Ctrl Pts',(-30.8921713054361,-33.2480152826956,
172.334397985524));
#29337=CARTESIAN_POINT('Ctrl Pts',(-31.3045676470177,-33.6140881241679,
172.297354722451));
#29338=CARTESIAN_POINT('Ctrl Pts',(-31.9163564219383,-33.755537063694,172.260311459378));
#29339=CARTESIAN_POINT('Ctrl Pts',(-32.4475864040807,-33.6076358335217,
172.223268196305));
#29340=CARTESIAN_POINT('Ctrl Pts',(-32.9788163862231,-33.4597346033494,
172.186224933231));
#29341=CARTESIAN_POINT('Ctrl Pts',(-33.4294875755873,-33.0224832034787,
172.149181670158));
#29342=CARTESIAN_POINT('Ctrl Pts',(-33.593375279583,-32.4959655035934,172.112138407085));
#29343=CARTESIAN_POINT('Ctrl Pts',(-33.6429542731456,-32.3366843798927,
172.10093215026));
#29344=CARTESIAN_POINT('Ctrl Pts',(-33.6662876483389,-32.1692338553619,
172.089725893435));
#29345=CARTESIAN_POINT('Ctrl Pts',(-33.6649323450731,-32.0014151634909,
172.07851963661));
#29346=CARTESIAN_POINT('Ctrl Pts',(-33.6634139074877,-31.999580988466,172.27148036339));
#29347=CARTESIAN_POINT('Ctrl Pts',(-33.6627298565773,-32.3034410203875,
172.291724457866));
#29348=CARTESIAN_POINT('Ctrl Pts',(-33.5831688370359,-32.6076345575211,
172.311968552341));
#29349=CARTESIAN_POINT('Ctrl Pts',(-33.4269053276148,-32.8653136482753,
172.332212646816));
#29350=CARTESIAN_POINT('Ctrl Pts',(-33.1409695800183,-33.3368227275717,
172.36925590989));
#29351=CARTESIAN_POINT('Ctrl Pts',(-32.5982124241901,-33.6525884191244,
172.406299172963));
#29352=CARTESIAN_POINT('Ctrl Pts',(-32.0469965916589,-33.668118054647,172.443342436036));
#29353=CARTESIAN_POINT('Ctrl Pts',(-31.4957807591278,-33.6836476901697,
172.480385699109));
#29354=CARTESIAN_POINT('Ctrl Pts',(-30.9361062498938,-33.3989412696623,
172.517428962183));
#29355=CARTESIAN_POINT('Ctrl Pts',(-30.6240770846737,-32.9442789073928,
172.554472225256));
#29356=CARTESIAN_POINT('Ctrl Pts',(-30.3120479194536,-32.4896165451233,
172.591515488329));
#29357=CARTESIAN_POINT('Ctrl Pts',(-30.2476640982474,-31.8649982410916,
172.628558751402));
#29358=CARTESIAN_POINT('Ctrl Pts',(-30.4603873085324,-31.356245944371,172.665602014476));
#29359=CARTESIAN_POINT('Ctrl Pts',(-30.6731105188173,-30.8474936476504,
172.702645277549));
#29360=CARTESIAN_POINT('Ctrl Pts',(-31.1629407605934,-30.4546073582408,
172.739688540622));
#29361=CARTESIAN_POINT('Ctrl Pts',(-31.7057343712178,-30.3573697118388,
172.776731803695));
#29362=CARTESIAN_POINT('Ctrl Pts',(-32.2485279818422,-30.2601320654369,
172.813775066769));
#29363=CARTESIAN_POINT('Ctrl Pts',(-32.8442849613149,-30.4585430620426,
172.850818329842));
#29364=CARTESIAN_POINT('Ctrl Pts',(-33.2203901461869,-30.8618109054481,
172.887861592915));
#29365=CARTESIAN_POINT('Ctrl Pts',(-33.5033876516186,-31.1652467481191,
172.915734516407));
#29366=CARTESIAN_POINT('Ctrl Pts',(-33.6620249806223,-31.5846663170183,
172.943607439898));
#29367=CARTESIAN_POINT('Ctrl Pts',(-33.6658031255686,-32.0015218482784,
172.97148036339));
#29368=CARTESIAN_POINT('Origin',(-32.,-32.,172.));
#29369=CARTESIAN_POINT('',(-33.668584334028,-31.9994831966231,173.67148036339));
#29370=CARTESIAN_POINT('',(-33.665039714177,-31.9985615025105,173.47851963661));
#29371=CARTESIAN_POINT('',(-33.666,-32.,172.));
#29372=CARTESIAN_POINT('Ctrl Pts',(-33.665039714177,-31.9985615025105,173.47851963661));
#29373=CARTESIAN_POINT('Ctrl Pts',(-33.6663911314701,-31.8347380945258,
173.467578383647));
#29374=CARTESIAN_POINT('Ctrl Pts',(-33.6441694753636,-31.6712733003014,
173.456637130684));
#29375=CARTESIAN_POINT('Ctrl Pts',(-33.5968738937745,-31.5154173654344,
173.445695877722));
#29376=CARTESIAN_POINT('Ctrl Pts',(-33.4367475648267,-30.9877435773881,
173.408652614648));
#29377=CARTESIAN_POINT('Ctrl Pts',(-32.9892080527959,-30.5472873448482,
173.371609351575));
#29378=CARTESIAN_POINT('Ctrl Pts',(-32.4590470117056,-30.3955990515507,
173.334566088502));
#29379=CARTESIAN_POINT('Ctrl Pts',(-31.9288859706153,-30.2439107582531,
173.297522825429));
#29380=CARTESIAN_POINT('Ctrl Pts',(-31.3161034004654,-30.3809904041979,
173.260479562355));
#29381=CARTESIAN_POINT('Ctrl Pts',(-30.9011052826813,-30.744111086684,173.223436299282));
#29382=CARTESIAN_POINT('Ctrl Pts',(-30.4861071648973,-31.1072317691701,
173.186393036209));
#29383=CARTESIAN_POINT('Ctrl Pts',(-30.2688934994791,-31.6963934881976,
173.149349773136));
#29384=CARTESIAN_POINT('Ctrl Pts',(-30.3488600819301,-32.241999035736,173.112306510062));
#29385=CARTESIAN_POINT('Ctrl Pts',(-30.4288266643811,-32.7876045832743,
173.075263246989));
#29386=CARTESIAN_POINT('Ctrl Pts',(-30.8059734947013,-33.2896539593234,
173.038219983916));
#29387=CARTESIAN_POINT('Ctrl Pts',(-31.3077202283297,-33.5184120916527,
173.001176720843));
#29388=CARTESIAN_POINT('Ctrl Pts',(-31.809466961958,-33.7471702239819,172.96413345777));
#29389=CARTESIAN_POINT('Ctrl Pts',(-32.4358135988946,-33.7026371125912,
172.927090194696));
#29390=CARTESIAN_POINT('Ctrl Pts',(-32.9001473143004,-33.4051908677823,
172.890046931623));
#29391=CARTESIAN_POINT('Ctrl Pts',(-33.3644810297062,-33.1077446229734,
172.85300366855));
#29392=CARTESIAN_POINT('Ctrl Pts',(-33.6668018235812,-32.5573852447462,
172.815960405477));
#29393=CARTESIAN_POINT('Ctrl Pts',(-33.6687693399146,-32.005954200378,172.778917142403));
#29394=CARTESIAN_POINT('Ctrl Pts',(-33.6687763776238,-32.0039817586375,
172.778784640472));
#29395=CARTESIAN_POINT('Ctrl Pts',(-33.6687795724397,-32.0020093031855,
172.778652138541));
#29396=CARTESIAN_POINT('Ctrl Pts',(-33.6687789306113,-32.0000368455925,
172.77851963661));
#29397=CARTESIAN_POINT('Ctrl Pts',(-33.6658031255686,-32.0015218482784,
172.97148036339));
#29398=CARTESIAN_POINT('Ctrl Pts',(-33.6670461552837,-32.1386695277898,
172.980650702972));
#29399=CARTESIAN_POINT('Ctrl Pts',(-33.651526531901,-32.2755396643596,172.989821042553));
#29400=CARTESIAN_POINT('Ctrl Pts',(-33.6181580939457,-32.4079104152445,
172.998991382135));
#29401=CARTESIAN_POINT('Ctrl Pts',(-33.4833674665614,-32.9426173914303,
173.036034645208));
#29402=CARTESIAN_POINT('Ctrl Pts',(-33.0573328215213,-33.4039066535968,
173.073077908281));
#29403=CARTESIAN_POINT('Ctrl Pts',(-32.5350053023192,-33.5806947366134,
173.110121171355));
#29404=CARTESIAN_POINT('Ctrl Pts',(-32.0126777831172,-33.75748281963,173.147164434428));
#29405=CARTESIAN_POINT('Ctrl Pts',(-31.3940573897532,-33.6497697234968,
173.184207697501));
#29406=CARTESIAN_POINT('Ctrl Pts',(-30.9622214599011,-33.3068443769544,
173.221250960574));
#29407=CARTESIAN_POINT('Ctrl Pts',(-30.530385530049,-32.9639190304119,173.258294223647));
#29408=CARTESIAN_POINT('Ctrl Pts',(-30.285334063709,-32.3857814334602,173.295337486721));
#29409=CARTESIAN_POINT('Ctrl Pts',(-30.3392012831418,-31.8369842156438,
173.332380749794));
#29410=CARTESIAN_POINT('Ctrl Pts',(-30.3930685025747,-31.2881869978274,
173.369424012867));
#29411=CARTESIAN_POINT('Ctrl Pts',(-30.7458544077805,-30.7687301591463,
173.40646727594));
#29412=CARTESIAN_POINT('Ctrl Pts',(-31.236126081439,-30.5163143323435,173.443510539014));
#29413=CARTESIAN_POINT('Ctrl Pts',(-31.7263977550975,-30.2638985055407,
173.480553802087));
#29414=CARTESIAN_POINT('Ctrl Pts',(-32.3541551972087,-30.2785236906163,
173.51759706516));
#29415=CARTESIAN_POINT('Ctrl Pts',(-32.8321400061355,-30.5534974821813,
173.554640328233));
#29416=CARTESIAN_POINT('Ctrl Pts',(-33.3101248150623,-30.8284712737464,
173.591683591306));
#29417=CARTESIAN_POINT('Ctrl Pts',(-33.6383369908047,-31.363793671801,173.62872685438));
#29418=CARTESIAN_POINT('Ctrl Pts',(-33.6665884213994,-31.9145040496602,
173.665770117453));
#29419=CARTESIAN_POINT('Ctrl Pts',(-33.668040080922,-31.9428015180507,173.667673532765));
#29420=CARTESIAN_POINT('Ctrl Pts',(-33.6686997625326,-31.9711396148911,
173.669576948078));
#29421=CARTESIAN_POINT('Ctrl Pts',(-33.668584334028,-31.9994831966231,173.67148036339));
#29422=CARTESIAN_POINT('Origin',(-32.,-32.,172.));
#29423=CARTESIAN_POINT('',(-33.6642813575761,-31.9988063447756,174.37148036339));
#29424=CARTESIAN_POINT('',(-33.6637114455411,-32.0008167340949,174.17851963661));
#29425=CARTESIAN_POINT('',(-33.666,-32.,172.));
#29426=CARTESIAN_POINT('Ctrl Pts',(-33.6637114455411,-32.0008167340949,
174.17851963661));
#29427=CARTESIAN_POINT('Ctrl Pts',(-33.6622464362393,-31.6705232921065,
174.156504628753));
#29428=CARTESIAN_POINT('Ctrl Pts',(-33.5671323700757,-31.3394521882123,
174.134489620897));
#29429=CARTESIAN_POINT('Ctrl Pts',(-33.3840346023194,-31.0676509334355,
174.11247461304));
#29430=CARTESIAN_POINT('Ctrl Pts',(-33.0759475544607,-30.6103081312015,
174.075431349967));
#29431=CARTESIAN_POINT('Ctrl Pts',(-32.5187551814412,-30.3207740795586,
174.038388086894));
#29432=CARTESIAN_POINT('Ctrl Pts',(-31.9674256919048,-30.3315379906054,
174.00134482382));
#29433=CARTESIAN_POINT('Ctrl Pts',(-31.4160962023684,-30.3423019016522,
173.964301560747));
#29434=CARTESIAN_POINT('Ctrl Pts',(-30.8706295963151,-30.6533637753888,
173.927258297674));
#29435=CARTESIAN_POINT('Ctrl Pts',(-30.5806284350053,-31.1223833850562,
173.890215034601));
#29436=CARTESIAN_POINT('Ctrl Pts',(-30.2906272736955,-31.5914029947235,
173.853171771527));
#29437=CARTESIAN_POINT('Ctrl Pts',(-30.2560915571293,-32.2183803403215,
173.816128508454));
#29438=CARTESIAN_POINT('Ctrl Pts',(-30.4928246419453,-32.7164139881476,
173.779085245381));
#29439=CARTESIAN_POINT('Ctrl Pts',(-30.7295577267612,-33.2144476359738,
173.742041982308));
#29440=CARTESIAN_POINT('Ctrl Pts',(-31.2375596129593,-33.5835375860281,
173.704998719234));
#29441=CARTESIAN_POINT('Ctrl Pts',(-31.7843713919408,-33.6547902784726,
173.667955456161));
#29442=CARTESIAN_POINT('Ctrl Pts',(-32.3311831709223,-33.7260429709171,
173.630912193088));
#29443=CARTESIAN_POINT('Ctrl Pts',(-32.9168048426872,-33.4994584057518,
173.593868930015));
#29444=CARTESIAN_POINT('Ctrl Pts',(-33.2732591056372,-33.0787204513927,
173.556825666941));
#29445=CARTESIAN_POINT('Ctrl Pts',(-33.5244295480755,-32.7822534172426,
173.530723656831));
#29446=CARTESIAN_POINT('Ctrl Pts',(-33.6618157042791,-32.3893869652009,
173.50462164672));
#29447=CARTESIAN_POINT('Ctrl Pts',(-33.665039714177,-31.9985615025105,173.47851963661));
#29448=CARTESIAN_POINT('Ctrl Pts',(-33.668584334028,-31.9994831966231,173.67148036339));
#29449=CARTESIAN_POINT('Ctrl Pts',(-33.6664533539675,-32.5227474262364,
173.706620211151));
#29450=CARTESIAN_POINT('Ctrl Pts',(-33.40014474482,-33.0478810491315,173.741760058912));
#29451=CARTESIAN_POINT('Ctrl Pts',(-32.9757931867974,-33.3537555837251,
173.776899906673));
#29452=CARTESIAN_POINT('Ctrl Pts',(-32.5284558361537,-33.676198382267,173.813943169746));
#29453=CARTESIAN_POINT('Ctrl Pts',(-31.9054904494194,-33.7549856216871,
173.850986432819));
#29454=CARTESIAN_POINT('Ctrl Pts',(-31.3919626096749,-33.5540646884328,
173.888029695892));
#29455=CARTESIAN_POINT('Ctrl Pts',(-30.8784347699304,-33.3531437551784,
173.925072958966));
#29456=CARTESIAN_POINT('Ctrl Pts',(-30.4743444771757,-32.8725146492496,
173.962116222039));
#29457=CARTESIAN_POINT('Ctrl Pts',(-30.364601258287,-32.3321106434165,173.999159485112));
#29458=CARTESIAN_POINT('Ctrl Pts',(-30.2548580393983,-31.7917066375835,
174.036202748186));
#29459=CARTESIAN_POINT('Ctrl Pts',(-30.4394618943756,-31.1915277318462,
174.073246011259));
#29460=CARTESIAN_POINT('Ctrl Pts',(-30.833939100154,-30.8062125391354,174.110289274332));
#29461=CARTESIAN_POINT('Ctrl Pts',(-31.2284163059325,-30.4208973464247,
174.147332537405));
#29462=CARTESIAN_POINT('Ctrl Pts',(-31.832766862512,-30.2504458667405,174.184375800479));
#29463=CARTESIAN_POINT('Ctrl Pts',(-32.3704432321562,-30.3728557729517,
174.221419063552));
#29464=CARTESIAN_POINT('Ctrl Pts',(-32.9081196018005,-30.4952656791629,
174.258462326625));
#29465=CARTESIAN_POINT('Ctrl Pts',(-33.3791217845095,-30.9105369712694,
174.295505589698));
#29466=CARTESIAN_POINT('Ctrl Pts',(-33.5679217353786,-31.4286437577182,
174.332548852771));
#29467=CARTESIAN_POINT('Ctrl Pts',(-33.63406302246,-31.6101493648096,174.345526022978));
#29468=CARTESIAN_POINT('Ctrl Pts',(-33.6655703636659,-31.8042757046356,
174.358503193184));
#29469=CARTESIAN_POINT('Ctrl Pts',(-33.6642813575761,-31.9988063447756,
174.37148036339));
#29470=CARTESIAN_POINT('Origin',(-32.,-32.,172.));
#29471=CARTESIAN_POINT('',(-33.6642763556304,-32.0011913006623,175.07148036339));
#29472=CARTESIAN_POINT('',(-33.6680206995223,-32.0009960691358,174.87851963661));
#29473=CARTESIAN_POINT('',(-33.666,-32.,172.));
#29474=CARTESIAN_POINT('Ctrl Pts',(-33.6680206995223,-32.0009960691358,
174.87851963661));
#29475=CARTESIAN_POINT('Ctrl Pts',(-33.6645339286199,-31.5078337739205,
174.845430873859));
#29476=CARTESIAN_POINT('Ctrl Pts',(-33.4321106122014,-31.0118158279499,
174.812342111109));
#29477=CARTESIAN_POINT('Ctrl Pts',(-33.0490371619582,-30.7021758227049,
174.779253348358));
#29478=CARTESIAN_POINT('Ctrl Pts',(-32.6201818825768,-30.3555301575651,
174.742210085285));
#29479=CARTESIAN_POINT('Ctrl Pts',(-32.0025157577892,-30.2424732431291,
174.705166822212));
#29480=CARTESIAN_POINT('Ctrl Pts',(-31.4786794571432,-30.4147393104172,
174.668123559139));
#29481=CARTESIAN_POINT('Ctrl Pts',(-30.9548431564971,-30.5870053777054,
174.631080296065));
#29482=CARTESIAN_POINT('Ctrl Pts',(-30.5248366799925,-31.0445944267177,
174.594037032992));
#29483=CARTESIAN_POINT('Ctrl Pts',(-30.3854286596648,-31.5781161897994,
174.556993769919));
#29484=CARTESIAN_POINT('Ctrl Pts',(-30.2460206393372,-32.1116379528812,
174.519950506846));
#29485=CARTESIAN_POINT('Ctrl Pts',(-30.3972110751866,-32.7210924300323,
174.482907243773));
#29486=CARTESIAN_POINT('Ctrl Pts',(-30.7698160435642,-33.1275965571378,
174.445863980699));
#29487=CARTESIAN_POINT('Ctrl Pts',(-31.1424210119419,-33.5341006842432,
174.408820717626));
#29488=CARTESIAN_POINT('Ctrl Pts',(-31.7364405128478,-33.7376544613031,
174.371777454553));
#29489=CARTESIAN_POINT('Ctrl Pts',(-32.2800544436041,-33.6451127836591,
174.33473419148));
#29490=CARTESIAN_POINT('Ctrl Pts',(-32.8236683743604,-33.5525711060151,
174.297690928406));
#29491=CARTESIAN_POINT('Ctrl Pts',(-33.3168767349671,-33.1639339736673,
174.260647665333));
#29492=CARTESIAN_POINT('Ctrl Pts',(-33.5339900539215,-32.6570396310809,
174.22360440226));
#29493=CARTESIAN_POINT('Ctrl Pts',(-33.6220717750628,-32.4513952867042,
174.208576147043));
#29494=CARTESIAN_POINT('Ctrl Pts',(-33.6647115148495,-32.226287202919,174.193547891826));
#29495=CARTESIAN_POINT('Ctrl Pts',(-33.6637114455411,-32.0008167340949,
174.17851963661));
#29496=CARTESIAN_POINT('Ctrl Pts',(-33.6642813575761,-31.9988063447756,
174.37148036339));
#29497=CARTESIAN_POINT('Ctrl Pts',(-33.6618909026641,-32.3595623783854,
174.395546456257));
#29498=CARTESIAN_POINT('Ctrl Pts',(-33.5467088752249,-32.7217088616016,
174.419612549124));
#29499=CARTESIAN_POINT('Ctrl Pts',(-33.3304552697857,-33.0073307793206,
174.443678641991));
#29500=CARTESIAN_POINT('Ctrl Pts',(-32.9975911342944,-33.4469687336831,
174.480721905064));
#29501=CARTESIAN_POINT('Ctrl Pts',(-32.4252651442828,-33.7053023616173,
174.517765168138));
#29502=CARTESIAN_POINT('Ctrl Pts',(-31.8753705694715,-33.6641195957362,
174.554808431211));
#29503=CARTESIAN_POINT('Ctrl Pts',(-31.3254759946603,-33.622936829855,174.591851694284));
#29504=CARTESIAN_POINT('Ctrl Pts',(-30.7980128350495,-33.2822376701586,
174.628894957357));
#29505=CARTESIAN_POINT('Ctrl Pts',(-30.5343453724271,-32.7979242047596,
174.665938220431));
#29506=CARTESIAN_POINT('Ctrl Pts',(-30.2706779098048,-32.3136107393606,
174.702981483504));
#29507=CARTESIAN_POINT('Ctrl Pts',(-30.2708061441709,-31.6856829682592,
174.740024746577));
#29508=CARTESIAN_POINT('Ctrl Pts',(-30.5346713961749,-31.2014772347147,
174.77706800965));
#29509=CARTESIAN_POINT('Ctrl Pts',(-30.7985366481788,-30.7172715011702,
174.814111272724));
#29510=CARTESIAN_POINT('Ctrl Pts',(-31.3261389178206,-30.3767878051827,
174.851154535797));
#29511=CARTESIAN_POINT('Ctrl Pts',(-31.8760502673163,-30.3358296398401,
174.88819779887));
#29512=CARTESIAN_POINT('Ctrl Pts',(-32.4259616168121,-30.2948714744975,
174.925241061943));
#29513=CARTESIAN_POINT('Ctrl Pts',(-32.9981820461618,-30.5534388397998,
174.962284325017));
#29514=CARTESIAN_POINT('Ctrl Pts',(-33.330866589631,-30.9932127114078,174.99932758809));
#29515=CARTESIAN_POINT('Ctrl Pts',(-33.5468672972666,-31.2787428610095,
175.02337851319));
#29516=CARTESIAN_POINT('Ctrl Pts',(-33.661892580785,-31.6406599108861,175.04742943829));
#29517=CARTESIAN_POINT('Ctrl Pts',(-33.6642763556304,-32.0011913006623,
175.07148036339));
#29518=CARTESIAN_POINT('Origin',(-32.,-32.,172.));
#29519=CARTESIAN_POINT('',(-33.6685813534211,-32.0005207267373,175.77148036339));
#29520=CARTESIAN_POINT('',(-33.6667310125706,-31.9985486151775,175.57851963661));
#29521=CARTESIAN_POINT('',(-33.666,-32.,172.));
#29522=CARTESIAN_POINT('Ctrl Pts',(-33.6667310125706,-31.9985486151775,
175.57851963661));
#29523=CARTESIAN_POINT('Ctrl Pts',(-33.6677032793229,-31.8922279811891,
175.571400382039));
#29524=CARTESIAN_POINT('Ctrl Pts',(-33.6584013252062,-31.7860768205684,
175.564281127468));
#29525=CARTESIAN_POINT('Ctrl Pts',(-33.6382086695285,-31.6820394404608,
175.557161872897));
#29526=CARTESIAN_POINT('Ctrl Pts',(-33.5331412289776,-31.1407069171911,
175.520118609823));
#29527=CARTESIAN_POINT('Ctrl Pts',(-33.1332209699927,-30.6566024924382,
175.48307534675));
#29528=CARTESIAN_POINT('Ctrl Pts',(-32.6214492346079,-30.4512497260222,
175.446032083677));
#29529=CARTESIAN_POINT('Ctrl Pts',(-32.109677499223,-30.2458969596062,175.408988820604));
#29530=CARTESIAN_POINT('Ctrl Pts',(-31.4860542874383,-30.3192958515271,
175.37194555753));
#29531=CARTESIAN_POINT('Ctrl Pts',(-31.0359461995104,-30.6378594668308,
175.334902294457));
#29532=CARTESIAN_POINT('Ctrl Pts',(-30.5858381115824,-30.9564230821345,
175.297859031384));
#29533=CARTESIAN_POINT('Ctrl Pts',(-30.3092451475112,-31.5201514208209,
175.260815768311));
#29534=CARTESIAN_POINT('Ctrl Pts',(-30.3327347478929,-32.0710854517969,
175.223772505237));
#29535=CARTESIAN_POINT('Ctrl Pts',(-30.3562243482745,-32.6220194827728,
175.186729242164));
#29536=CARTESIAN_POINT('Ctrl Pts',(-30.679796513109,-33.1601592060383,175.149685979091));
#29537=CARTESIAN_POINT('Ctrl Pts',(-31.1553863742651,-33.4392548021681,
175.112642716018));
#29538=CARTESIAN_POINT('Ctrl Pts',(-31.6309762354211,-33.7183503982979,
175.075599452944));
#29539=CARTESIAN_POINT('Ctrl Pts',(-32.2585837928988,-33.7384018672921,
175.038556189871));
#29540=CARTESIAN_POINT('Ctrl Pts',(-32.7510192314565,-33.4902337656634,
175.001512926798));
#29541=CARTESIAN_POINT('Ctrl Pts',(-33.2434546700142,-33.2420656640348,
174.964469663725));
#29542=CARTESIAN_POINT('Ctrl Pts',(-33.600717989652,-32.7256779917834,174.927426400651));
#29543=CARTESIAN_POINT('Ctrl Pts',(-33.6593274324834,-32.1773669477359,
174.890383137578));
#29544=CARTESIAN_POINT('Ctrl Pts',(-33.6655841993383,-32.118832790084,174.886428637255));
#29545=CARTESIAN_POINT('Ctrl Pts',(-33.6684374100764,-32.0599348233683,
174.882474136933));
#29546=CARTESIAN_POINT('Ctrl Pts',(-33.6680206995223,-32.0009960691358,
174.87851963661));
#29547=CARTESIAN_POINT('Ctrl Pts',(-33.6642763556304,-32.0011913006623,
175.07148036339));
#29548=CARTESIAN_POINT('Ctrl Pts',(-33.6655640736003,-32.1959507806569,
175.084472701363));
#29549=CARTESIAN_POINT('Ctrl Pts',(-33.6339810497051,-32.3903059010507,
175.097465039336));
#29550=CARTESIAN_POINT('Ctrl Pts',(-33.5676882417626,-32.5719965913415,
175.11045737731));
#29551=CARTESIAN_POINT('Ctrl Pts',(-33.378676692836,-33.0900262217536,175.147500640383));
#29552=CARTESIAN_POINT('Ctrl Pts',(-32.9075049373938,-33.5051051046639,
175.184543903456));
#29553=CARTESIAN_POINT('Ctrl Pts',(-32.3697786159041,-33.6272953939243,
175.221587166529));
#29554=CARTESIAN_POINT('Ctrl Pts',(-31.8320522944143,-33.7494856831846,
175.258630429603));
#29555=CARTESIAN_POINT('Ctrl Pts',(-31.2277714068769,-33.5787873787949,
175.295673692676));
#29556=CARTESIAN_POINT('Ctrl Pts',(-30.8334516108523,-33.1933110992711,
175.332716955749));
#29557=CARTESIAN_POINT('Ctrl Pts',(-30.4391318148276,-32.8078348197473,
175.369760218822));
#29558=CARTESIAN_POINT('Ctrl Pts',(-30.2547731103158,-32.2075805650895,
175.406803481895));
#29559=CARTESIAN_POINT('Ctrl Pts',(-30.3647370408579,-31.6672214274853,
175.443846744969));
#29560=CARTESIAN_POINT('Ctrl Pts',(-30.4747009714001,-31.1268622898811,
175.480890008042));
#29561=CARTESIAN_POINT('Ctrl Pts',(-30.8789875369963,-30.6463982693306,
175.517933271115));
#29562=CARTESIAN_POINT('Ctrl Pts',(-31.3925973973822,-30.4456870964311,
175.554976534188));
#29563=CARTESIAN_POINT('Ctrl Pts',(-31.906207257768,-30.2449759235315,175.592019797262));
#29564=CARTESIAN_POINT('Ctrl Pts',(-32.5291404129435,-30.324017598283,175.629063060335));
#29565=CARTESIAN_POINT('Ctrl Pts',(-32.9763460288151,-30.6466430789026,
175.666106323408));
#29566=CARTESIAN_POINT('Ctrl Pts',(-33.400389507867,-30.9525588062043,175.701231003402));
#29567=CARTESIAN_POINT('Ctrl Pts',(-33.6664369809567,-31.47747986754,175.736355683396));
#29568=CARTESIAN_POINT('Ctrl Pts',(-33.6685813534211,-32.0005207267373,
175.77148036339));
#29569=CARTESIAN_POINT('Origin',(-32.,-32.,172.));
#29570=CARTESIAN_POINT('',(-33.6658099164955,-31.9984780038309,176.47148036339));
#29571=CARTESIAN_POINT('',(-33.6633199948406,-31.9999190844576,176.27851963661));
#29572=CARTESIAN_POINT('',(-33.666,-32.,172.));
#29573=CARTESIAN_POINT('Ctrl Pts',(-33.6633199948406,-31.9999190844576,
176.27851963661));
#29574=CARTESIAN_POINT('Ctrl Pts',(-33.6634383333563,-31.7268069707849,
176.260326627145));
#29575=CARTESIAN_POINT('Ctrl Pts',(-33.5999313242785,-31.4537466878109,
176.24213361768));
#29576=CARTESIAN_POINT('Ctrl Pts',(-33.4724977567379,-31.2147758799386,
176.223940608215));
#29577=CARTESIAN_POINT('Ctrl Pts',(-33.2130269321966,-30.728201159034,176.186897345142));
#29578=CARTESIAN_POINT('Ctrl Pts',(-32.6885287507801,-30.3829549203862,
176.149854082068));
#29579=CARTESIAN_POINT('Ctrl Pts',(-32.1390107363186,-30.3370199707946,
176.112810818995));
#29580=CARTESIAN_POINT('Ctrl Pts',(-31.5894927218572,-30.2910850212031,
176.075767555922));
#29581=CARTESIAN_POINT('Ctrl Pts',(-31.0149548743507,-30.5444613606678,
176.038724292849));
#29582=CARTESIAN_POINT('Ctrl Pts',(-30.6783025975229,-30.9812053501188,
176.001681029775));
#29583=CARTESIAN_POINT('Ctrl Pts',(-30.3416503206951,-31.4179493395698,
175.964637766702));
#29584=CARTESIAN_POINT('Ctrl Pts',(-30.2428836145458,-32.0380609790071,
175.927594503629));
#29585=CARTESIAN_POINT('Ctrl Pts',(-30.4271975882658,-32.557780544643,175.890551240556));
#29586=CARTESIAN_POINT('Ctrl Pts',(-30.6115115619858,-33.0775001102788,
175.853507977482));
#29587=CARTESIAN_POINT('Ctrl Pts',(-31.0789062155749,-33.4968276021132,
175.816464714409));
#29588=CARTESIAN_POINT('Ctrl Pts',(-31.6155042898944,-33.6238810335897,
175.779421451336));
#29589=CARTESIAN_POINT('Ctrl Pts',(-32.1521023642139,-33.7509344650662,
175.742378188263));
#29590=CARTESIAN_POINT('Ctrl Pts',(-32.7579038592636,-33.5857138361847,
175.705334925189));
#29591=CARTESIAN_POINT('Ctrl Pts',(-33.15569729573,-33.2038232108508,175.668291662116));
#29592=CARTESIAN_POINT('Ctrl Pts',(-33.4770397798243,-32.895327215323,175.638367653614));
#29593=CARTESIAN_POINT('Ctrl Pts',(-33.6626443321084,-32.4454408457679,
175.608443645112));
#29594=CARTESIAN_POINT('Ctrl Pts',(-33.6667310125706,-31.9985486151775,
175.57851963661));
#29595=CARTESIAN_POINT('Ctrl Pts',(-33.6685813534211,-32.0005207267373,
175.77148036339));
#29596=CARTESIAN_POINT('Ctrl Pts',(-33.6686984835053,-32.0290903063712,
175.773398946469));
#29597=CARTESIAN_POINT('Ctrl Pts',(-33.6680282397883,-32.0576542762874,
175.775317529549));
#29598=CARTESIAN_POINT('Ctrl Pts',(-33.6665533627086,-32.0861766390156,
175.777236112628));
#29599=CARTESIAN_POINT('Ctrl Pts',(-33.6380770041629,-32.6368754320213,
175.814279375701));
#29600=CARTESIAN_POINT('Ctrl Pts',(-33.3096462105037,-33.1720637315449,
175.851322638774));
#29601=CARTESIAN_POINT('Ctrl Pts',(-32.8315491320692,-33.4468422736528,
175.888365901848));
#29602=CARTESIAN_POINT('Ctrl Pts',(-32.3534520536346,-33.7216208157607,
175.925409164921));
#29603=CARTESIAN_POINT('Ctrl Pts',(-31.7256886904246,-33.7359896004529,
175.962452427994));
#29604=CARTESIAN_POINT('Ctrl Pts',(-31.2355201535362,-33.4833735497848,
175.999495691067));
#29605=CARTESIAN_POINT('Ctrl Pts',(-30.7453516166478,-33.2307574991166,
176.03653895414));
#29606=CARTESIAN_POINT('Ctrl Pts',(-30.392777906081,-32.7111566130881,176.073582217214));
#29607=CARTESIAN_POINT('Ctrl Pts',(-30.3391348400455,-32.1623374396888,
176.110625480287));
#29608=CARTESIAN_POINT('Ctrl Pts',(-30.2854917740099,-31.6135182662894,
176.14766874336));
#29609=CARTESIAN_POINT('Ctrl Pts',(-30.5307793525056,-31.0354808055192,
176.184712006434));
#29610=CARTESIAN_POINT('Ctrl Pts',(-30.962755309618,-30.6927318652276,176.221755269507));
#29611=CARTESIAN_POINT('Ctrl Pts',(-31.3947312667304,-30.3499829249361,
176.25879853258));
#29612=CARTESIAN_POINT('Ctrl Pts',(-32.0133956024596,-30.2425225051232,
176.295841795653));
#29613=CARTESIAN_POINT('Ctrl Pts',(-32.5356508713666,-30.4195239110553,
176.332885058727));
#29614=CARTESIAN_POINT('Ctrl Pts',(-33.0579061402737,-30.5965253169874,
176.3699283218));
#29615=CARTESIAN_POINT('Ctrl Pts',(-33.4837523423586,-31.0579885486645,
176.406971584873));
#29616=CARTESIAN_POINT('Ctrl Pts',(-33.6183245645552,-31.5927505337774,
176.444014847946));
#29617=CARTESIAN_POINT('Ctrl Pts',(-33.6515838325967,-31.7249159384278,
176.453170019761));
#29618=CARTESIAN_POINT('Ctrl Pts',(-33.6670514510545,-31.8615585907079,
176.462325191576));
#29619=CARTESIAN_POINT('Ctrl Pts',(-33.6658099164955,-31.9984780038309,
176.47148036339));
#29620=CARTESIAN_POINT('Origin',(-32.,-32.,172.));
#29621=CARTESIAN_POINT('',(-33.6634122043807,-32.0004154259855,177.17148036339));
#29622=CARTESIAN_POINT('',(-33.6664340665864,-32.0014938874889,176.97851963661));
#29623=CARTESIAN_POINT('',(-33.666,-32.,172.));
#29624=CARTESIAN_POINT('Ctrl Pts',(-33.6664340665864,-32.0014938874889,
176.97851963661));
#29625=CARTESIAN_POINT('Ctrl Pts',(-33.6623982369357,-31.5642166774555,
176.949252872251));
#29626=CARTESIAN_POINT('Ctrl Pts',(-33.485716464103,-31.1240530442927,176.919986107892));
#29627=CARTESIAN_POINT('Ctrl Pts',(-33.1768207287417,-30.8168180471713,
176.890719343533));
#29628=CARTESIAN_POINT('Ctrl Pts',(-32.7858480251356,-30.427947358081,176.85367608046));
#29629=CARTESIAN_POINT('Ctrl Pts',(-32.1830653647693,-30.2520315499555,
176.816632817387));
#29630=CARTESIAN_POINT('Ctrl Pts',(-31.6443028236447,-30.3695687437297,
176.779589554313));
#29631=CARTESIAN_POINT('Ctrl Pts',(-31.1055402825201,-30.4871059375039,
176.74254629124));
#29632=CARTESIAN_POINT('Ctrl Pts',(-30.6307978606372,-30.8980961331778,
176.705503028167));
#29633=CARTESIAN_POINT('Ctrl Pts',(-30.4373151165222,-31.4144724452213,
176.668459765094));
#29634=CARTESIAN_POINT('Ctrl Pts',(-30.2438323724072,-31.9308487572648,
176.631416502021));
#29635=CARTESIAN_POINT('Ctrl Pts',(-30.3316093060602,-32.5526111856777,
176.594373238947));
#29636=CARTESIAN_POINT('Ctrl Pts',(-30.660479668368,-32.9952446148261,176.557329975874));
#29637=CARTESIAN_POINT('Ctrl Pts',(-30.9893500306758,-33.4378780439745,
176.520286712801));
#29638=CARTESIAN_POINT('Ctrl Pts',(-31.5593138216386,-33.7013824738583,
176.483243449728));
#29639=CARTESIAN_POINT('Ctrl Pts',(-32.1095587011216,-33.6651797060375,
176.446200186654));
#29640=CARTESIAN_POINT('Ctrl Pts',(-32.6598035806047,-33.6289769382167,
176.409156923581));
#29641=CARTESIAN_POINT('Ctrl Pts',(-33.1903295486081,-33.2930669726913,
176.372113660508));
#29642=CARTESIAN_POINT('Ctrl Pts',(-33.4583707987768,-32.8111603883479,
176.335070397434));
#29643=CARTESIAN_POINT('Ctrl Pts',(-33.5947692994478,-32.5659319560578,
176.316220143826));
#29644=CARTESIAN_POINT('Ctrl Pts',(-33.6631973812051,-32.2828976986404,
176.297369890218));
#29645=CARTESIAN_POINT('Ctrl Pts',(-33.6633199948406,-31.9999190844576,
176.27851963661));
#29646=CARTESIAN_POINT('Ctrl Pts',(-33.6658099164955,-31.9984780038309,
176.47148036339));
#29647=CARTESIAN_POINT('Ctrl Pts',(-33.6620280072332,-32.4155560407657,
176.499368454649));
#29648=CARTESIAN_POINT('Ctrl Pts',(-33.5032006501307,-32.8352021617193,
176.527256545907));
#29649=CARTESIAN_POINT('Ctrl Pts',(-33.2199251662155,-33.138687451872,176.555144637166));
#29650=CARTESIAN_POINT('Ctrl Pts',(-32.843655303371,-33.5418016463048,176.592187900239));
#29651=CARTESIAN_POINT('Ctrl Pts',(-32.2478173353736,-33.7399692966219,
176.629231163313));
#29652=CARTESIAN_POINT('Ctrl Pts',(-31.7050634853874,-33.6425099619088,
176.666274426386));
#29653=CARTESIAN_POINT('Ctrl Pts',(-31.1623096354013,-33.5450506271958,
176.703317689459));
#29654=CARTESIAN_POINT('Ctrl Pts',(-30.6726399034262,-33.1519643074527,
176.740360952532));
#29655=CARTESIAN_POINT('Ctrl Pts',(-30.4601245040871,-32.6431251684204,
176.777404215605));
#29656=CARTESIAN_POINT('Ctrl Pts',(-30.247609104748,-32.1342860293882,176.814447478679));
#29657=CARTESIAN_POINT('Ctrl Pts',(-30.3122480380448,-31.5096940710668,
176.851490741752));
#29658=CARTESIAN_POINT('Ctrl Pts',(-30.6244628777836,-31.0551591924778,
176.888534004825));
#29659=CARTESIAN_POINT('Ctrl Pts',(-30.9366777175223,-30.6006243138889,
176.925577267898));
#29660=CARTESIAN_POINT('Ctrl Pts',(-31.4964684637029,-30.3161465150323,
176.962620530972));
#29661=CARTESIAN_POINT('Ctrl Pts',(-32.0476779078561,-30.3319012827413,
176.999663794045));
#29662=CARTESIAN_POINT('Ctrl Pts',(-32.5988873520092,-30.3476560504503,
177.036707057118));
#29663=CARTESIAN_POINT('Ctrl Pts',(-33.1415154941349,-30.6636433847247,
177.073750320191));
#29664=CARTESIAN_POINT('Ctrl Pts',(-33.4272586353279,-31.1352692179958,
177.110793583265));
#29665=CARTESIAN_POINT('Ctrl Pts',(-33.5832998849668,-31.3928190023175,
177.131022509973));
#29666=CARTESIAN_POINT('Ctrl Pts',(-33.6627345752346,-31.6967822785539,
177.151251436682));
#29667=CARTESIAN_POINT('Ctrl Pts',(-33.6634122043807,-32.0004154259855,
177.17148036339));
#29668=CARTESIAN_POINT('Origin',(-32.,-32.,172.));
#29669=CARTESIAN_POINT('',(-33.6673324974466,-32.0013033571361,177.87148036339));
#29670=CARTESIAN_POINT('',(-33.6682333060465,-31.9991447275653,177.67851963661));
#29671=CARTESIAN_POINT('',(-33.666,-32.,172.));
#29672=CARTESIAN_POINT('Ctrl Pts',(-33.6682333060465,-31.9991447275653,
177.67851963661));
#29673=CARTESIAN_POINT('Ctrl Pts',(-33.6685408591694,-31.9500181746268,
177.67522238043));
#29674=CARTESIAN_POINT('Ctrl Pts',(-33.6665588525363,-31.9009167876488,
177.671925124251));
#29675=CARTESIAN_POINT('Ctrl Pts',(-33.6622065197431,-31.8520264135902,
177.668627868071));
#29676=CARTESIAN_POINT('Ctrl Pts',(-33.6133099221287,-31.3027639694832,
177.631584604998));
#29677=CARTESIAN_POINT('Ctrl Pts',(-33.265241148879,-30.7801346509114,177.594541341925));
#29678=CARTESIAN_POINT('Ctrl Pts',(-32.7772747180259,-30.5232906550829,
177.557498078852));
#29679=CARTESIAN_POINT('Ctrl Pts',(-32.2893082871728,-30.2664466592544,
177.520454815778));
#29680=CARTESIAN_POINT('Ctrl Pts',(-31.6614441987163,-30.2753879861691,
177.483411552705));
#29681=CARTESIAN_POINT('Ctrl Pts',(-31.1809895889168,-30.5460232043939,
177.446368289632));
#29682=CARTESIAN_POINT('Ctrl Pts',(-30.7005349791173,-30.8166584226187,
177.409325026559));
#29683=CARTESIAN_POINT('Ctrl Pts',(-30.3674898479748,-31.3489875321536,
177.372281763485));
#29684=CARTESIAN_POINT('Ctrl Pts',(-30.3342538741355,-31.8994195839005,
177.335238500412));
#29685=CARTESIAN_POINT('Ctrl Pts',(-30.3010179002961,-32.4498516356474,
177.298195237339));
#29686=CARTESIAN_POINT('Ctrl Pts',(-30.5675910837598,-33.0183866296063,
177.261151974266));
#29687=CARTESIAN_POINT('Ctrl Pts',(-31.0119909652455,-33.3448660524889,
177.224108711192));
#29688=CARTESIAN_POINT('Ctrl Pts',(-31.4563908467312,-33.6713454753716,
177.187065448119));
#29689=CARTESIAN_POINT('Ctrl Pts',(-32.0786174262389,-33.755769327178,177.150022185046));
#29690=CARTESIAN_POINT('Ctrl Pts',(-32.5939432027082,-33.5595057026458,
177.112978921973));
#29691=CARTESIAN_POINT('Ctrl Pts',(-33.1092689791776,-33.3632420781135,
177.075935658899));
#29692=CARTESIAN_POINT('Ctrl Pts',(-33.5176939526085,-32.8862909772425,
177.038892395826));
#29693=CARTESIAN_POINT('Ctrl Pts',(-33.6323250659011,-32.3469026417795,
177.001849132753));
#29694=CARTESIAN_POINT('Ctrl Pts',(-33.656389595621,-32.2336687539068,176.994072634039));
#29695=CARTESIAN_POINT('Ctrl Pts',(-33.6675064305726,-32.1176832147392,
176.986296135324));
#29696=CARTESIAN_POINT('Ctrl Pts',(-33.6664340665864,-32.0014938874889,
176.97851963661));
#29697=CARTESIAN_POINT('Ctrl Pts',(-33.6634122043807,-32.0004154259855,
177.17148036339));
#29698=CARTESIAN_POINT('Ctrl Pts',(-33.663975451485,-32.2527960859167,177.188294699755));
#29699=CARTESIAN_POINT('Ctrl Pts',(-33.6101256220151,-32.5049486605984,
177.20510903612));
#29700=CARTESIAN_POINT('Ctrl Pts',(-33.5006277344169,-32.7300294102653,
177.221923372484));
#29701=CARTESIAN_POINT('Ctrl Pts',(-33.259395552053,-33.2258994369961,177.258966635558));
#29702=CARTESIAN_POINT('Ctrl Pts',(-32.7480730470649,-33.5903751581898,
177.296009898631));
#29703=CARTESIAN_POINT('Ctrl Pts',(-32.200638611329,-33.6566745563935,177.333053161704));
#29704=CARTESIAN_POINT('Ctrl Pts',(-31.653204175593,-33.7229739545973,177.370096424777));
#29705=CARTESIAN_POINT('Ctrl Pts',(-31.0696578091092,-33.491097029811,177.407139687851));
#29706=CARTESIAN_POINT('Ctrl Pts',(-30.717027193283,-33.0671492094921,177.444182950924));
#29707=CARTESIAN_POINT('Ctrl Pts',(-30.3643965774567,-32.6432013891732,
177.481226213997));
#29708=CARTESIAN_POINT('Ctrl Pts',(-30.2426817122881,-32.0271826733217,
177.51826947707));
#29709=CARTESIAN_POINT('Ctrl Pts',(-30.4075786025872,-31.5009802852002,
177.555312740144));
#29710=CARTESIAN_POINT('Ctrl Pts',(-30.5724754928864,-30.9747778970788,
177.592356003217));
#29711=CARTESIAN_POINT('Ctrl Pts',(-31.0239841386533,-30.5383918366873,
177.62939926629));
#29712=CARTESIAN_POINT('Ctrl Pts',(-31.5554967489003,-30.3915091864542,
177.666442529363));
#29713=CARTESIAN_POINT('Ctrl Pts',(-32.0870093591472,-30.2446265362211,
177.703485792436));
#29714=CARTESIAN_POINT('Ctrl Pts',(-32.6985259338742,-30.3872472961464,
177.74052905551));
#29715=CARTESIAN_POINT('Ctrl Pts',(-33.1102195658544,-30.7541106342973,
177.777572318583));
#29716=CARTESIAN_POINT('Ctrl Pts',(-33.4581131802515,-31.0641212897578,
177.808875000185));
#29717=CARTESIAN_POINT('Ctrl Pts',(-33.6633179681641,-31.5342582545151,
177.840177681788));
#29718=CARTESIAN_POINT('Ctrl Pts',(-33.6673324974466,-32.0013033571361,
177.87148036339));
#29719=CARTESIAN_POINT('Origin',(-32.,-32.,172.));
#29720=CARTESIAN_POINT('',(-33.6674973899495,-31.9987820730806,178.57148036339));
#29721=CARTESIAN_POINT('',(-33.6638666881858,-31.9990537019747,178.37851963661));
#29722=CARTESIAN_POINT('',(-33.666,-32.,172.));
#29723=CARTESIAN_POINT('',(-30.7309291201475,-30.9206413469517,179.));
#29724=CARTESIAN_POINT('Ctrl Pts',(-33.6674973899495,-31.9987820730806,
178.57148036339));
#29725=CARTESIAN_POINT('Ctrl Pts',(-33.6635707056189,-32.4716839165788,
178.60319045304));
#29726=CARTESIAN_POINT('Ctrl Pts',(-33.452366876924,-32.9475799899327,178.634900542691));
#29727=CARTESIAN_POINT('Ctrl Pts',(-33.0965045258218,-33.2578609118632,
178.666610632341));
#29728=CARTESIAN_POINT('Ctrl Pts',(-32.6807913305846,-33.6203265480209,
178.703653895414));
#29729=CARTESIAN_POINT('Ctrl Pts',(-32.067668858848,-33.756784295561,178.740697158487));
#29730=CARTESIAN_POINT('Ctrl Pts',(-31.5378405565417,-33.6037851722251,
178.777740421561));
#29731=CARTESIAN_POINT('Ctrl Pts',(-31.0080122542353,-33.4507860488891,
178.814783684634));
#29732=CARTESIAN_POINT('Ctrl Pts',(-30.5614781213592,-33.0083300546771,
178.851826947707));
#29733=CARTESIAN_POINT('Ctrl Pts',(-30.4024857707402,-32.4812852538864,
178.88887021078));
#29734=CARTESIAN_POINT('Ctrl Pts',(-30.2434934201212,-31.9542404530957,
178.925913473853));
#29735=CARTESIAN_POINT('Ctrl Pts',(-30.3720428517593,-31.3426068457263,
178.962956736927));
#29736=CARTESIAN_POINT('Ctrl Pts',(-30.7309291201476,-30.9206413469516,
179.));
#29737=CARTESIAN_POINT('',(-33.2714881524743,-30.9188041220687,179.));
#29738=CARTESIAN_POINT('Origin',(-32.,-32.,179.));
#29739=CARTESIAN_POINT('Ctrl Pts',(-33.2714899711315,-30.918802739816,179.));
#29740=CARTESIAN_POINT('Ctrl Pts',(-32.9207087468888,-30.5073974083421,
178.963685183163));
#29741=CARTESIAN_POINT('Ctrl Pts',(-32.3509045024841,-30.2812938695396,
178.927370366326));
#29742=CARTESIAN_POINT('Ctrl Pts',(-31.8135987861801,-30.3417506510624,
178.891055549488));
#29743=CARTESIAN_POINT('Ctrl Pts',(-31.2655151461327,-30.4034201473605,
178.854012286415));
#29744=CARTESIAN_POINT('Ctrl Pts',(-30.7512468997307,-30.7632616102458,
178.816969023342));
#29745=CARTESIAN_POINT('Ctrl Pts',(-30.5057843626736,-31.2569767104513,
178.779925760269));
#29746=CARTESIAN_POINT('Ctrl Pts',(-30.2603218256164,-31.7506918106568,
178.742882497195));
#29747=CARTESIAN_POINT('Ctrl Pts',(-30.283664997904,-32.3782805481824,178.705839234122));
#29748=CARTESIAN_POINT('Ctrl Pts',(-30.5652971229397,-32.8523839798957,
178.668795971049));
#29749=CARTESIAN_POINT('Ctrl Pts',(-30.8469292479753,-33.326487411609,178.631752707976));
#29750=CARTESIAN_POINT('Ctrl Pts',(-31.386850325759,-33.64710553751,178.594709444902));
#29751=CARTESIAN_POINT('Ctrl Pts',(-31.9379143916448,-33.6676125145974,
178.557666181829));
#29752=CARTESIAN_POINT('Ctrl Pts',(-32.4889784575306,-33.6881194916849,
178.520622918756));
#29753=CARTESIAN_POINT('Ctrl Pts',(-33.0511855115185,-33.4085153199588,
178.483579655683));
#29754=CARTESIAN_POINT('Ctrl Pts',(-33.3673124400932,-32.9567024906769,
178.446536392609));
#29755=CARTESIAN_POINT('Ctrl Pts',(-33.5607972682093,-32.6801713896778,
178.42386414061));
#29756=CARTESIAN_POINT('Ctrl Pts',(-33.6620998285923,-32.3391304687567,
178.40119188861));
#29757=CARTESIAN_POINT('Ctrl Pts',(-33.6638666881858,-31.9990537019747,
178.37851963661));
#29758=CARTESIAN_POINT('Origin',(-32.,-32.,180.545925280538));
#29759=CARTESIAN_POINT('',(-34.0533144768684,-31.9981861022711,166.254074719462));
#29760=CARTESIAN_POINT('',(-34.054669363007,-32.0018603689044,166.195925280538));
#29761=CARTESIAN_POINT('',(-34.05475,-31.9999999999998,180.545925280538));
#29762=CARTESIAN_POINT('',(-31.6163320011535,-29.981387499008,166.));
#29763=CARTESIAN_POINT('Ctrl Pts',(-34.0546693630069,-32.0018603689044,
166.195925280538));
#29764=CARTESIAN_POINT('Ctrl Pts',(-34.0494207835165,-31.4804652280817,
166.167660116765));
#29765=CARTESIAN_POINT('Ctrl Pts',(-33.5818273573597,-30.2681449287862,
166.102351689919));
#29766=CARTESIAN_POINT('Ctrl Pts',(-32.2875197530252,-29.8538180613451,
166.037043263073));
#29767=CARTESIAN_POINT('Ctrl Pts',(-31.6163320011535,-29.981387499008,166.));
#29768=CARTESIAN_POINT('',(-30.6584058382614,-30.4387497520534,166.));
#29769=CARTESIAN_POINT('Origin',(-32.,-32.,166.));
#29770=CARTESIAN_POINT('Ctrl Pts',(-34.0533144768684,-31.9981861022711,
166.254074719462));
#29771=CARTESIAN_POINT('Ctrl Pts',(-34.0549811944317,-31.7888335083511,
166.242741226219));
#29772=CARTESIAN_POINT('Ctrl Pts',(-33.9292854405696,-30.897222765403,166.194364469902));
#29773=CARTESIAN_POINT('Ctrl Pts',(-32.6547058314541,-29.6692718705854,
166.109672896748));
#29774=CARTESIAN_POINT('Ctrl Pts',(-31.1647193012354,-30.0048405258246,
166.036314816837));
#29775=CARTESIAN_POINT('Ctrl Pts',(-30.658403887814,-30.438747719014,166.));
#29776=CARTESIAN_POINT('Origin',(-32.,-32.,180.545925280538));
#29777=CARTESIAN_POINT('',(-34.052039769042,-32.0011058419296,166.954074719462));
#29778=CARTESIAN_POINT('',(-34.0578396464241,-31.9992413474394,166.895925280538));
#29779=CARTESIAN_POINT('',(-34.05475,-31.9999999999998,180.545925280538));
#29780=CARTESIAN_POINT('Ctrl Pts',(-34.0578396464241,-31.9992413474394,
166.895925280538));
#29781=CARTESIAN_POINT('Ctrl Pts',(-34.0580399301433,-31.9570745650302,
166.893629624944));
#29782=CARTESIAN_POINT('Ctrl Pts',(-34.0377496442503,-31.2346904324969,
166.854290706278));
#29783=CARTESIAN_POINT('Ctrl Pts',(-33.1886966470223,-29.8821785627325,
166.777908524538));
#29784=CARTESIAN_POINT('Ctrl Pts',(-30.8656448278897,-29.8526443561693,
166.666778735318));
#29785=CARTESIAN_POINT('Ctrl Pts',(-29.580472364777,-31.7882407548095,166.555648946099));
#29786=CARTESIAN_POINT('Ctrl Pts',(-30.5101755007489,-33.9178527489701,
166.444519156879));
#29787=CARTESIAN_POINT('Ctrl Pts',(-32.8022294941794,-34.2918270332952,
166.333389367659));
#29788=CARTESIAN_POINT('Ctrl Pts',(-33.9655640455529,-33.0073758803891,
166.250524742212));
#29789=CARTESIAN_POINT('Ctrl Pts',(-34.0562993748591,-32.1637861358238,
166.204703379838));
#29790=CARTESIAN_POINT('Ctrl Pts',(-34.0546693630069,-32.0018603689044,
166.195925280538));
#29791=CARTESIAN_POINT('Ctrl Pts',(-34.052039769042,-32.0011058419296,166.954074719462));
#29792=CARTESIAN_POINT('Ctrl Pts',(-34.0500129149945,-31.5865390425708,
166.931667471325));
#29793=CARTESIAN_POINT('Ctrl Pts',(-33.7267813695385,-30.483712125216,166.872216960114));
#29794=CARTESIAN_POINT('Ctrl Pts',(-31.9269554466752,-29.5724870533531,
166.77572318583));
#29795=CARTESIAN_POINT('Ctrl Pts',(-29.9209653227032,-30.7446538702704,
166.66459339661));
#29796=CARTESIAN_POINT('Ctrl Pts',(-29.8177242538605,-33.0657579476906,
166.553463607391));
#29797=CARTESIAN_POINT('Ctrl Pts',(-31.7115987445193,-34.4113736221389,
166.442333818171));
#29798=CARTESIAN_POINT('Ctrl Pts',(-33.6494969998368,-33.6381762860152,
166.342537522195));
#29799=CARTESIAN_POINT('Ctrl Pts',(-34.0495335662521,-32.4730976663593,
166.279784489292));
#29800=CARTESIAN_POINT('Ctrl Pts',(-34.0533144768684,-31.9981861022711,
166.254074719462));
#29801=CARTESIAN_POINT('Origin',(-32.,-32.,180.545925280538));
#29802=CARTESIAN_POINT('',(-34.0574026221756,-32.0011268610995,167.654074719462));
#29803=CARTESIAN_POINT('',(-34.052475201976,-31.9986057389706,167.595925280538));
#29804=CARTESIAN_POINT('',(-34.05475,-31.9999999999998,180.545925280538));
#29805=CARTESIAN_POINT('Ctrl Pts',(-34.052475201976,-31.9986057389706,167.595925280538));
#29806=CARTESIAN_POINT('Ctrl Pts',(-34.0540189352112,-31.7513839339351,
167.58255587005));
#29807=CARTESIAN_POINT('Ctrl Pts',(-33.8982418403506,-30.8210528024315,
167.53214319649));
#29808=CARTESIAN_POINT('Ctrl Pts',(-32.514074117309,-29.6264115999403,167.444687259856));
#29809=CARTESIAN_POINT('Ctrl Pts',(-30.2847464274524,-30.2806705307475,
167.333557470637));
#29810=CARTESIAN_POINT('Ctrl Pts',(-29.6251964131156,-32.5084396585803,
167.222427681417));
#29811=CARTESIAN_POINT('Ctrl Pts',(-31.139048610325,-34.2708933540495,167.111297892197));
#29812=CARTESIAN_POINT('Ctrl Pts',(-33.3932698151157,-33.9615685478801,
167.002463758571));
#29813=CARTESIAN_POINT('Ctrl Pts',(-34.0548081028085,-32.6374881332951,
166.930672888018));
#29814=CARTESIAN_POINT('Ctrl Pts',(-34.0578396464241,-31.9992413474394,
166.895925280538));
#29815=CARTESIAN_POINT('Ctrl Pts',(-34.0574026221756,-32.0011268610995,
167.654074719462));
#29816=CARTESIAN_POINT('Ctrl Pts',(-34.0533392918178,-31.3858045207831,
167.620593716431));
#29817=CARTESIAN_POINT('Ctrl Pts',(-33.4332619034794,-30.0825878835663,
167.550069450326));
#29818=CARTESIAN_POINT('Ctrl Pts',(-31.2169834359616,-29.7010702107005,
167.442501921148));
#29819=CARTESIAN_POINT('Ctrl Pts',(-29.643917581989,-31.4108732197425,167.331372131929));
#29820=CARTESIAN_POINT('Ctrl Pts',(-30.2271133546761,-33.6598394847521,
167.220242342709));
#29821=CARTESIAN_POINT('Ctrl Pts',(-32.4328346425493,-34.389736993149,167.109112553489));
#29822=CARTESIAN_POINT('Ctrl Pts',(-33.8775609679021,-33.2263857218232,
167.020390012407));
#29823=CARTESIAN_POINT('Ctrl Pts',(-34.0533636739647,-32.2718934830552,
166.968710734398));
#29824=CARTESIAN_POINT('Ctrl Pts',(-34.052039769042,-32.0011058419296,166.954074719462));
#29825=CARTESIAN_POINT('Origin',(-32.,-32.,180.545925280538));
#29826=CARTESIAN_POINT('',(-34.0554335040134,-31.998175874568,168.354074719462));
#29827=CARTESIAN_POINT('',(-34.0527878691605,-32.0015414751871,168.295925280538));
#29828=CARTESIAN_POINT('',(-34.05475,-31.9999999999998,180.545925280538));
#29829=CARTESIAN_POINT('Ctrl Pts',(-34.0527878691605,-32.0015414751871,
168.295925280538));
#29830=CARTESIAN_POINT('Ctrl Pts',(-34.0496367929324,-31.5497213201872,
168.271482115157));
#29831=CARTESIAN_POINT('Ctrl Pts',(-33.6800738627717,-30.4084888310145,
168.209995686702));
#29832=CARTESIAN_POINT('Ctrl Pts',(-31.7940424351662,-29.5801291028184,
168.111465995175));
#29833=CARTESIAN_POINT('Ctrl Pts',(-29.8553131533993,-30.8604773304489,
168.000336205955));
#29834=CARTESIAN_POINT('Ctrl Pts',(-29.8793779622368,-33.1837043267573,
167.889206416735));
#29835=CARTESIAN_POINT('Ctrl Pts',(-31.8442131712534,-34.4236180024818,
167.778076627516));
#29836=CARTESIAN_POINT('Ctrl Pts',(-33.6980918025173,-33.5631391374147,
167.680316248783));
#29837=CARTESIAN_POINT('Ctrl Pts',(-34.0497416399332,-32.4363731763679,
167.619599133124));
#29838=CARTESIAN_POINT('Ctrl Pts',(-34.052475201976,-31.9986057389706,167.595925280538));
#29839=CARTESIAN_POINT('Ctrl Pts',(-34.0554335040134,-31.998175874568,168.354074719462));
#29840=CARTESIAN_POINT('Ctrl Pts',(-34.0567078789638,-31.8597835387434,
168.34656322461));
#29841=CARTESIAN_POINT('Ctrl Pts',(-33.9808807164526,-31.0402919719527,
168.302008466685));
#29842=CARTESIAN_POINT('Ctrl Pts',(-32.8805549549265,-29.7366359735545,
168.220410445687));
#29843=CARTESIAN_POINT('Ctrl Pts',(-30.576127479021,-30.0325700070413,168.109280656467));
#29844=CARTESIAN_POINT('Ctrl Pts',(-29.5748126892805,-32.1290746285719,
167.998150867247));
#29845=CARTESIAN_POINT('Ctrl Pts',(-30.7930030339464,-34.1074515612365,
167.887021078027));
#29846=CARTESIAN_POINT('Ctrl Pts',(-33.1158238969359,-34.1571116561114,
167.775891288808));
#29847=CARTESIAN_POINT('Ctrl Pts',(-34.0253015915237,-32.8124183710368,
167.698242502619));
#29848=CARTESIAN_POINT('Ctrl Pts',(-34.0578349461223,-32.0665949769654,
167.657636979504));
#29849=CARTESIAN_POINT('Ctrl Pts',(-34.0574026221756,-32.0011268610995,
167.654074719462));
#29850=CARTESIAN_POINT('Origin',(-32.,-32.,180.545925280538));
#29851=CARTESIAN_POINT('',(-34.0514404014557,-32.0000193281895,169.054074719462));
#29852=CARTESIAN_POINT('',(-34.0580205885241,-32.0005154407378,168.995925280538));
#29853=CARTESIAN_POINT('',(-34.05475,-31.9999999999998,180.545925280538));
#29854=CARTESIAN_POINT('Ctrl Pts',(-34.0580205885241,-32.0005154407378,
168.995925280538));
#29855=CARTESIAN_POINT('Ctrl Pts',(-34.0558244730528,-31.3482962555674,
168.960408360263));
#29856=CARTESIAN_POINT('Ctrl Pts',(-33.3683227356013,-30.0118438106801,
168.887848176915));
#29857=CARTESIAN_POINT('Ctrl Pts',(-31.0921885500407,-29.7474299050867,
168.778244730493));
#29858=CARTESIAN_POINT('Ctrl Pts',(-29.6151760063164,-31.540861481794,168.667114941273));
#29859=CARTESIAN_POINT('Ctrl Pts',(-30.3207285185246,-33.7544916509204,
168.555985152054));
#29860=CARTESIAN_POINT('Ctrl Pts',(-32.56313208116,-34.3624300883911,168.444855362834));
#29861=CARTESIAN_POINT('Ctrl Pts',(-33.9103001430262,-33.150131804933,168.358168738995));
#29862=CARTESIAN_POINT('Ctrl Pts',(-34.0544122033125,-32.2344482204289,
168.30852537823));
#29863=CARTESIAN_POINT('Ctrl Pts',(-34.0527878691605,-32.0015414751871,
168.295925280538));
#29864=CARTESIAN_POINT('Ctrl Pts',(-34.0514404014557,-32.0000193281895,
169.054074719462));
#29865=CARTESIAN_POINT('Ctrl Pts',(-34.051411527961,-31.6559142783085,169.035489469716));
#29866=CARTESIAN_POINT('Ctrl Pts',(-33.8062204612892,-30.6259162375257,
168.979860956897));
#29867=CARTESIAN_POINT('Ctrl Pts',(-32.1767327344769,-29.5778193124972,
168.887189181005));
#29868=CARTESIAN_POINT('Ctrl Pts',(-30.0609459319521,-30.5377199094004,
168.776059391785));
#29869=CARTESIAN_POINT('Ctrl Pts',(-29.719760384286,-32.8358833873742,168.664929602565));
#29870=CARTESIAN_POINT('Ctrl Pts',(-31.4654254048604,-34.3690554541617,
168.553799813346));
#29871=CARTESIAN_POINT('Ctrl Pts',(-33.5492656048371,-33.7770120558115,
168.450181518978));
#29872=CARTESIAN_POINT('Ctrl Pts',(-34.0504232435519,-32.5422713529885,
168.383606487683));
#29873=CARTESIAN_POINT('Ctrl Pts',(-34.0554335040134,-31.998175874568,168.354074719462));
#29874=CARTESIAN_POINT('Origin',(-32.,-32.,180.545925280538));
#29875=CARTESIAN_POINT('',(-34.0555044381159,-32.0018139756141,169.754074719462));
#29876=CARTESIAN_POINT('',(-34.0543002253323,-31.9981314623868,169.695925280538));
#29877=CARTESIAN_POINT('',(-34.05475,-31.9999999999998,180.545925280538));
#29878=CARTESIAN_POINT('Ctrl Pts',(-34.0543002253323,-31.9981314623868,
169.695925280538));
#29879=CARTESIAN_POINT('Ctrl Pts',(-34.0558755988635,-31.8219808306189,
169.686377868442));
#29880=CARTESIAN_POINT('Ctrl Pts',(-33.9545116868703,-30.9641640659178,
169.639787193273));
#29881=CARTESIAN_POINT('Ctrl Pts',(-32.7552096240695,-29.6917859534862,
169.556153255031));
#29882=CARTESIAN_POINT('Ctrl Pts',(-30.4704602313883,-30.1135478386525,
169.445023465812));
#29883=CARTESIAN_POINT('Ctrl Pts',(-29.5855290477775,-32.2617702841642,
169.333893676592));
#29884=CARTESIAN_POINT('Ctrl Pts',(-30.9102954957832,-34.1704234043853,
169.222763887372));
#29885=CARTESIAN_POINT('Ctrl Pts',(-33.2323476887161,-34.0927285621829,
169.111634098152));
#29886=CARTESIAN_POINT('Ctrl Pts',(-34.0448973480045,-32.7367311286634,
169.036021229207));
#29887=CARTESIAN_POINT('Ctrl Pts',(-34.0581149667812,-32.0285446180569,
168.997451623336));
#29888=CARTESIAN_POINT('Ctrl Pts',(-34.0580205885241,-32.0005154407378,
168.995925280538));
#29889=CARTESIAN_POINT('Ctrl Pts',(-34.0555044381159,-32.001813975614,169.754074719462));
#29890=CARTESIAN_POINT('Ctrl Pts',(-34.0504819825047,-31.4554228012545,
169.724415714823));
#29891=CARTESIAN_POINT('Ctrl Pts',(-33.545729393308,-30.2184084874635,169.657713447109));
#29892=CARTESIAN_POINT('Ctrl Pts',(-31.4573116667505,-29.6327900145418,
169.553967916323));
#29893=CARTESIAN_POINT('Ctrl Pts',(-29.7169098581211,-31.1719340929902,
169.442838127103));
#29894=CARTESIAN_POINT('Ctrl Pts',(-30.065967388257,-33.4689151095322,169.331708337884));
#29895=CARTESIAN_POINT('Ctrl Pts',(-32.1850305909512,-34.4215609475536,
169.220578548664));
#29896=CARTESIAN_POINT('Ctrl Pts',(-33.8086854466956,-33.3693338832287,
169.12803400919));
#29897=CARTESIAN_POINT('Ctrl Pts',(-34.0514690772797,-32.3417686015944,
169.07253273279));
#29898=CARTESIAN_POINT('Ctrl Pts',(-34.0514404014557,-32.0000193281895,
169.054074719462));
#29899=CARTESIAN_POINT('Origin',(-32.,-32.,180.545925280538));
#29900=CARTESIAN_POINT('',(-34.0573518213482,-31.9988395038175,170.454074719462));
#29901=CARTESIAN_POINT('',(-34.0516184490435,-32.0006260637404,170.395925280538));
#29902=CARTESIAN_POINT('',(-34.05475,-31.9999999999998,180.545925280538));
#29903=CARTESIAN_POINT('Ctrl Pts',(-34.0516184490435,-32.0006260637404,
170.395925280538));
#29904=CARTESIAN_POINT('Ctrl Pts',(-34.0505756737721,-31.61890879556,170.375304113548));
#29905=CARTESIAN_POINT('Ctrl Pts',(-33.7652193718894,-30.5500373359834,
170.317639683485));
#29906=CARTESIAN_POINT('Ctrl Pts',(-32.0437423823724,-29.5717742558001,
170.22293199035));
#29907=CARTESIAN_POINT('Ctrl Pts',(-29.983732689712,-30.6461684764067,170.11180220113));
#29908=CARTESIAN_POINT('Ctrl Pts',(-29.7689889739188,-32.9595746257144,
170.00067241191));
#29909=CARTESIAN_POINT('Ctrl Pts',(-31.5960423548879,-34.3947884837217,
169.88954262269));
#29910=CARTESIAN_POINT('Ctrl Pts',(-33.6040655308435,-33.7033079951078,
169.787960245566));
#29911=CARTESIAN_POINT('Ctrl Pts',(-34.0497632643824,-32.5054324432433,
169.723421131515));
#29912=CARTESIAN_POINT('Ctrl Pts',(-34.0543002253323,-31.9981314623868,
169.695925280538));
#29913=CARTESIAN_POINT('Ctrl Pts',(-34.0573518213482,-31.9988395038175,
170.454074719462));
#29914=CARTESIAN_POINT('Ctrl Pts',(-34.0578102452832,-31.9310285956751,
170.450385223002));
#29915=CARTESIAN_POINT('Ctrl Pts',(-34.024004004144,-31.1828456234217,170.409652463468));
#29916=CARTESIAN_POINT('Ctrl Pts',(-33.1084266441611,-29.8390779475391,
170.331876440861));
#29917=CARTESIAN_POINT('Ctrl Pts',(-30.7857895475778,-29.8966962369818,
170.220746651642));
#29918=CARTESIAN_POINT('Ctrl Pts',(-29.5743846894872,-31.8792353209593,
170.109616862422));
#29919=CARTESIAN_POINT('Ctrl Pts',(-30.5828766588753,-33.9722969295563,
169.998487073202));
#29920=CARTESIAN_POINT('Ctrl Pts',(-32.888304541998,-34.2603337768931,169.887357283982));
#29921=CARTESIAN_POINT('Ctrl Pts',(-33.9824484770852,-32.9549541539966,
169.805886499403));
#29922=CARTESIAN_POINT('Ctrl Pts',(-34.0567548883806,-32.1378500188405,
169.761458977896));
#29923=CARTESIAN_POINT('Ctrl Pts',(-34.0555044381159,-32.001813975614,169.754074719462));
#29924=CARTESIAN_POINT('Origin',(-32.,-32.,180.545925280538));
#29925=CARTESIAN_POINT('',(-34.0520023712765,-31.9989253081128,171.154074719462));
#29926=CARTESIAN_POINT('',(-34.0565936768906,-32.0015359661287,171.095925280538));
#29927=CARTESIAN_POINT('',(-34.05475,-31.9999999999998,180.545925280538));
#29928=CARTESIAN_POINT('Ctrl Pts',(-34.0565936768906,-32.0015359661287,
171.095925280538));
#29929=CARTESIAN_POINT('Ctrl Pts',(-34.0517293936845,-31.4184384269289,
171.064230358654));
#29930=CARTESIAN_POINT('Ctrl Pts',(-33.4873352665121,-30.145615302178,170.995492173698));
#29931=CARTESIAN_POINT('Ctrl Pts',(-31.3284143351364,-29.6660834728807,
170.889710725668));
#29932=CARTESIAN_POINT('Ctrl Pts',(-29.6749656425999,-31.298281468308,170.778580936448));
#29933=CARTESIAN_POINT('Ctrl Pts',(-30.1493631800083,-33.5726846541191,
170.667451147229));
#29934=CARTESIAN_POINT('Ctrl Pts',(-32.3174434657525,-34.4077838995354,
170.556321358009));
#29935=CARTESIAN_POINT('Ctrl Pts',(-33.8466042950419,-33.2932393514889,
170.465812735779));
#29936=CARTESIAN_POINT('Ctrl Pts',(-34.0524488848626,-32.3046145653666,
170.412347376621));
#29937=CARTESIAN_POINT('Ctrl Pts',(-34.0516184490435,-32.0006260637404,
170.395925280538));
#29938=CARTESIAN_POINT('Ctrl Pts',(-34.0520023712765,-31.9989253081128,
171.154074719462));
#29939=CARTESIAN_POINT('Ctrl Pts',(-34.0532978946503,-31.7257714041052,
171.139311468108));
#29940=CARTESIAN_POINT('Ctrl Pts',(-33.8754247784623,-30.7688511478335,
171.08750495368));
#29941=CARTESIAN_POINT('Ctrl Pts',(-32.4246449932043,-29.6087931139184,
170.99865517618));
#29942=CARTESIAN_POINT('Ctrl Pts',(-30.2214364984569,-30.3462449959935,
170.88752538696));
#29943=CARTESIAN_POINT('Ctrl Pts',(-29.6459500326037,-32.5971955235092,
170.77639559774));
#29944=CARTESIAN_POINT('Ctrl Pts',(-31.2248645683027,-34.3015991842251,
170.66526580852));
#29945=CARTESIAN_POINT('Ctrl Pts',(-33.4372030087975,-33.91295041841,170.557825515761));
#29946=CARTESIAN_POINT('Ctrl Pts',(-34.0532075796883,-32.611863321091,170.487428486075));
#29947=CARTESIAN_POINT('Ctrl Pts',(-34.0573518213482,-31.9988395038175,
170.454074719462));
#29948=CARTESIAN_POINT('Origin',(-32.,-32.,180.545925280538));
#29949=CARTESIAN_POINT('',(-34.0534332149094,-32.0017453824621,171.854074719462));
#29950=CARTESIAN_POINT('',(-34.0564014860358,-31.998396538586,171.795925280538));
#29951=CARTESIAN_POINT('',(-34.05475,-31.9999999999998,180.545925280538));
#29952=CARTESIAN_POINT('Ctrl Pts',(-34.0564014860358,-31.998396538586,171.795925280538));
#29953=CARTESIAN_POINT('Ctrl Pts',(-34.0573061420266,-31.8930393954218,
171.790199866834));
#29954=CARTESIAN_POINT('Ctrl Pts',(-34.0020448666022,-31.1069760699122,
171.747431190056));
#29955=CARTESIAN_POINT('Ctrl Pts',(-32.9883523238082,-29.7815876522084,
171.667619250206));
#29956=CARTESIAN_POINT('Ctrl Pts',(-30.6723620180839,-29.9663896514365,
171.556489460986));
#29957=CARTESIAN_POINT('Ctrl Pts',(-29.5714115957749,-32.0123297880839,
171.445359671767));
#29958=CARTESIAN_POINT('Ctrl Pts',(-30.6930789440682,-34.046985836388,171.334229882547));
#29959=CARTESIAN_POINT('Ctrl Pts',(-33.0108262697815,-34.2082626458667,
171.223100093327));
#29960=CARTESIAN_POINT('Ctrl Pts',(-34.006283703558,-32.8789600308985,171.143665225991));
#29961=CARTESIAN_POINT('Ctrl Pts',(-34.0574144975358,-32.0999304218123,
171.101273621728));
#29962=CARTESIAN_POINT('Ctrl Pts',(-34.0565936768906,-32.0015359661287,
171.095925280538));
#29963=CARTESIAN_POINT('Ctrl Pts',(-34.0534332149094,-32.0017453824621,
171.854074719462));
#29964=CARTESIAN_POINT('Ctrl Pts',(-34.04957930023,-31.524539330965,171.828237713214));
#29965=CARTESIAN_POINT('Ctrl Pts',(-33.6462715310717,-30.357274746545,171.765357443893));
#29966=CARTESIAN_POINT('Ctrl Pts',(-31.7033831764878,-29.5895618235874,
171.665433911498));
#29967=CARTESIAN_POINT('Ctrl Pts',(-29.8140636467216,-30.9417580608795,
171.554304122278));
#29968=CARTESIAN_POINT('Ctrl Pts',(-29.925289361983,-33.2624458446987,171.443174333059));
#29969=CARTESIAN_POINT('Ctrl Pts',(-31.9352677538577,-34.4277568821048,
171.332044543839));
#29970=CARTESIAN_POINT('Ctrl Pts',(-33.729598785223,-33.5115700062286,171.235678005974));
#29971=CARTESIAN_POINT('Ctrl Pts',(-34.0500472277068,-32.4111564648077,
171.176354731181));
#29972=CARTESIAN_POINT('Ctrl Pts',(-34.0520023712765,-31.9989253081128,
171.154074719462));
#29973=CARTESIAN_POINT('Origin',(-32.,-32.,180.545925280538));
#29974=CARTESIAN_POINT('',(-34.0581778610564,-32.0000454497033,172.554074719462));
#29975=CARTESIAN_POINT('',(-34.0515604600302,-31.9994832149161,172.495925280538));
#29976=CARTESIAN_POINT('',(-34.05475,-31.9999999999998,180.545925280538));
#29977=CARTESIAN_POINT('Ctrl Pts',(-34.0515604600302,-31.9994832149161,
172.495925280538));
#29978=CARTESIAN_POINT('Ctrl Pts',(-34.0522605628883,-31.6884927994845,
172.47912611194));
#29979=CARTESIAN_POINT('Ctrl Pts',(-33.8397955875772,-30.6926560482339,
172.425283680269));
#29980=CARTESIAN_POINT('Ctrl Pts',(-32.2929794020452,-29.5891170225852,
172.334397985524));
#29981=CARTESIAN_POINT('Ctrl Pts',(-30.1334901515899,-30.4461870619026,
172.223268196305));
#29982=CARTESIAN_POINT('Ctrl Pts',(-29.6822104729431,-32.7252898517669,
172.112138407085));
#29983=CARTESIAN_POINT('Ctrl Pts',(-31.352146634078,-34.3406152347352,172.001008617865));
#29984=CARTESIAN_POINT('Ctrl Pts',(-33.4984092777462,-33.8409746916955,
171.895604242349));
#29985=CARTESIAN_POINT('Ctrl Pts',(-34.0514530436148,-32.5746971013405,
171.827243129907));
#29986=CARTESIAN_POINT('Ctrl Pts',(-34.0564014860358,-31.998396538586,171.795925280538));
#29987=CARTESIAN_POINT('Ctrl Pts',(-34.0581773755543,-32.000045443266,172.554074719462));
#29988=CARTESIAN_POINT('Ctrl Pts',(-34.0579568627806,-31.3223688901445,
172.51716395832));
#29989=CARTESIAN_POINT('Ctrl Pts',(-33.3218062651671,-29.9641725193915,
172.443209934105));
#29990=CARTESIAN_POINT('Ctrl Pts',(-31.0083014581836,-29.7830814754581,
172.332212646816));
#29991=CARTESIAN_POINT('Ctrl Pts',(-29.5996266783055,-31.6306740480343,
172.221082857597));
#29992=CARTESIAN_POINT('Ctrl Pts',(-30.3877475314776,-33.8162697266764,
172.109953068377));
#29993=CARTESIAN_POINT('Ctrl Pts',(-32.6513843596913,-34.3396350480892,
171.998823279157));
#29994=CARTESIAN_POINT('Ctrl Pts',(-33.9311983000411,-33.0979305633151,
171.913530496186));
#29995=CARTESIAN_POINT('Ctrl Pts',(-34.0551047691624,-32.2087234479617,
171.865280976287));
#29996=CARTESIAN_POINT('Ctrl Pts',(-34.0534332149094,-32.0017453824621,
171.854074719462));
#29997=CARTESIAN_POINT('Origin',(-32.,-32.,180.545925280538));
#29998=CARTESIAN_POINT('',(-34.0535656378783,-31.9982258387056,173.254074719462));
#29999=CARTESIAN_POINT('',(-34.0545071862317,-32.0018769614345,173.195925280538));
#30000=CARTESIAN_POINT('',(-34.05475,-31.9999999999998,180.545925280538));
#30001=CARTESIAN_POINT('Ctrl Pts',(-34.0545071862317,-32.0018769614345,
173.195925280538));
#30002=CARTESIAN_POINT('Ctrl Pts',(-34.0498474363346,-31.4877509693236,
173.168052357046));
#30003=CARTESIAN_POINT('Ctrl Pts',(-33.5941675512997,-30.2829837046594,
173.103136170481));
#30004=CARTESIAN_POINT('Ctrl Pts',(-31.571747429243,-29.6094365943462,173.001176720843));
#30005=CARTESIAN_POINT('Ctrl Pts',(-29.7593608338838,-31.063127656467,172.890046931623));
#30006=CARTESIAN_POINT('Ctrl Pts',(-29.9975829046342,-33.3742341274316,
172.778917142403));
#30007=CARTESIAN_POINT('Ctrl Pts',(-32.0683953857542,-34.4276564279194,
172.667787353184));
#30008=CARTESIAN_POINT('Ctrl Pts',(-33.7730366841982,-33.4359288520185,
172.573456732562));
#30009=CARTESIAN_POINT('Ctrl Pts',(-34.0507167903975,-32.374246960769,172.516169375013));
#30010=CARTESIAN_POINT('Ctrl Pts',(-34.0515604600302,-31.9994832149161,
172.495925280538));
#30011=CARTESIAN_POINT('Ctrl Pts',(-34.0535656378783,-31.9982258387056,
173.254074719462));
#30012=CARTESIAN_POINT('Ctrl Pts',(-34.0552323993927,-31.7961753299681,
173.2431334665));
#30013=CARTESIAN_POINT('Ctrl Pts',(-33.9350351652449,-30.9119920786341,
173.195148950464));
#30014=CARTESIAN_POINT('Ctrl Pts',(-32.6680632857967,-29.6650727659158,
173.110121171355));
#30015=CARTESIAN_POINT('Ctrl Pts',(-30.4007493854086,-30.1722715699463,
172.998991382135));
#30016=CARTESIAN_POINT('Ctrl Pts',(-29.5970523043438,-32.3521876122724,
172.887861592915));
#30017=CARTESIAN_POINT('Ctrl Pts',(-30.9925068954609,-34.2097853711626,
172.776731803695));
#30018=CARTESIAN_POINT('Ctrl Pts',(-33.3100082500444,-34.0450115224891,
172.665602014476));
#30019=CARTESIAN_POINT('Ctrl Pts',(-34.0570726447537,-32.685019407829,172.591382986398));
#30020=CARTESIAN_POINT('Ctrl Pts',(-34.0581781671492,-32.0024781606965,
172.554207221393));
#30021=CARTESIAN_POINT('Ctrl Pts',(-34.0581773755543,-32.000045443266,172.554074719462));
#30022=CARTESIAN_POINT('Origin',(-32.,-32.,180.545925280538));
#30023=CARTESIAN_POINT('',(-34.051927426606,-32.0010073135544,173.954074719462));
#30024=CARTESIAN_POINT('',(-34.0579373711549,-31.9993626039982,173.895925280538));
#30025=CARTESIAN_POINT('',(-34.05475,-31.9999999999998,180.545925280538));
#30026=CARTESIAN_POINT('Ctrl Pts',(-34.0579373711549,-31.9993626039982,
173.895925280538));
#30027=CARTESIAN_POINT('Ctrl Pts',(-34.058079734132,-31.9644052363129,173.894021865225));
#30028=CARTESIAN_POINT('Ctrl Pts',(-34.0414319960198,-31.2492644665138,
173.85507518684));
#30029=CARTESIAN_POINT('Ctrl Pts',(-33.2110354115502,-29.8948665380118,
173.779085245381));
#30030=CARTESIAN_POINT('Ctrl Pts',(-30.8883140354794,-29.8407529143012,
173.667955456161));
#30031=CARTESIAN_POINT('Ctrl Pts',(-29.5829955984056,-31.7627588073625,
173.556825666941));
#30032=CARTESIAN_POINT('Ctrl Pts',(-30.4896933783496,-33.9018852671521,
173.445695877722));
#30033=CARTESIAN_POINT('Ctrl Pts',(-32.7786073998349,-34.3004269555309,
173.334566088502));
#30034=CARTESIAN_POINT('Ctrl Pts',(-33.9595797532929,-33.0217284461304,
173.251309222774));
#30035=CARTESIAN_POINT('Ctrl Pts',(-34.056040268649,-32.1710271381908,173.205095620119));
#30036=CARTESIAN_POINT('Ctrl Pts',(-34.0545071862317,-32.0018769614345,
173.195925280538));
#30037=CARTESIAN_POINT('Ctrl Pts',(-34.051927426606,-32.0010073135544,173.954074719462));
#30038=CARTESIAN_POINT('Ctrl Pts',(-34.0501205671445,-31.5936420975126,
173.932059711606));
#30039=CARTESIAN_POINT('Ctrl Pts',(-33.7354250014453,-30.4982561832208,
173.873001440676));
#30040=CARTESIAN_POINT('Ctrl Pts',(-31.9525937458611,-29.571843005618,173.776899906673));
#30041=CARTESIAN_POINT('Ctrl Pts',(-29.9343509329174,-30.722781274034,173.665770117453));
#30042=CARTESIAN_POINT('Ctrl Pts',(-29.8065677451363,-33.0426162695937,
173.554640328234));
#30043=CARTESIAN_POINT('Ctrl Pts',(-31.6861899702242,-34.4082601619239,
173.443510539014));
#30044=CARTESIAN_POINT('Ctrl Pts',(-33.6396742821775,-33.6524319289162,
173.343322002757));
#30045=CARTESIAN_POINT('Ctrl Pts',(-34.0495893267512,-32.4802478191756,
173.280176729573));
#30046=CARTESIAN_POINT('Ctrl Pts',(-34.0535656378783,-31.9982258387056,
173.254074719462));
#30047=CARTESIAN_POINT('Origin',(-32.,-32.,180.545925280538));
#30048=CARTESIAN_POINT('',(-34.0572422162926,-32.0012284952321,174.654074719462));
#30049=CARTESIAN_POINT('',(-34.0526303238172,-31.9985278132817,174.595925280538));
#30050=CARTESIAN_POINT('',(-34.05475,-31.9999999999998,180.545925280538));
#30051=CARTESIAN_POINT('Ctrl Pts',(-34.0526303238172,-31.9985278132817,
174.595925280538));
#30052=CARTESIAN_POINT('Ctrl Pts',(-34.0542201108898,-31.7586047443576,
174.582948110331));
#30053=CARTESIAN_POINT('Ctrl Pts',(-33.9044368791735,-30.8357445655057,
174.532927677052));
#30054=CARTESIAN_POINT('Ctrl Pts',(-32.5391158564695,-29.6319738696303,
174.445863980699));
#30055=CARTESIAN_POINT('Ctrl Pts',(-30.3030006593535,-30.2626494600523,
174.334734191479));
#30056=CARTESIAN_POINT('Ctrl Pts',(-29.6199608556057,-32.4833294238526,
174.22360440226));
#30057=CARTESIAN_POINT('Ctrl Pts',(-31.1151070663578,-34.2616715404322,
174.11247461304));
#30058=CARTESIAN_POINT('Ctrl Pts',(-33.3806181402508,-33.9751494202814,
174.003248239133));
#30059=CARTESIAN_POINT('Ctrl Pts',(-34.0553091410954,-32.6447270552576,
173.931065128299));
#30060=CARTESIAN_POINT('Ctrl Pts',(-34.0579373711549,-31.9993626039982,
173.895925280538));
#30061=CARTESIAN_POINT('Ctrl Pts',(-34.0572422162926,-32.0012284952321,
174.654074719462));
#30062=CARTESIAN_POINT('Ctrl Pts',(-34.0529418306313,-31.3929900642036,
174.620985956712));
#30063=CARTESIAN_POINT('Ctrl Pts',(-33.4453673259805,-30.0963565660462,
174.550853930888));
#30064=CARTESIAN_POINT('Ctrl Pts',(-31.2413083934035,-29.6929280920661,
174.443678641991));
#30065=CARTESIAN_POINT('Ctrl Pts',(-29.65027152498,-31.3860213065764,174.332548852771));
#30066=CARTESIAN_POINT('Ctrl Pts',(-30.2096806751507,-33.6410211629863,
174.221419063552));
#30067=CARTESIAN_POINT('Ctrl Pts',(-32.4075706562188,-34.3941762471646,
174.110289274332));
#30068=CARTESIAN_POINT('Ctrl Pts',(-33.8709432996413,-33.2410714072619,
174.021174492969));
#30069=CARTESIAN_POINT('Ctrl Pts',(-34.0531608554243,-32.2790898140443,
173.969102974679));
#30070=CARTESIAN_POINT('Ctrl Pts',(-34.051927426606,-32.0010073135544,173.954074719462));
#30071=CARTESIAN_POINT('Origin',(-32.,-32.,180.545925280538));
#30072=CARTESIAN_POINT('',(-34.0556515894835,-31.9982099441992,175.354074719462));
#30073=CARTESIAN_POINT('',(-34.0526241547008,-32.0014692827344,175.295925280538));
#30074=CARTESIAN_POINT('',(-34.05475,-31.9999999999998,180.545925280538));
#30075=CARTESIAN_POINT('Ctrl Pts',(-34.0526241547008,-32.0014692827344,
175.295925280538));
#30076=CARTESIAN_POINT('Ctrl Pts',(-34.0496841418774,-31.5568102952538,
175.271874355438));
#30077=CARTESIAN_POINT('Ctrl Pts',(-33.6893168078909,-30.4229458230359,
175.210780167264));
#30078=CARTESIAN_POINT('Ctrl Pts',(-31.8196126680302,-29.5780887565239,
175.112642716018));
#30079=CARTESIAN_POINT('Ctrl Pts',(-29.8674684359538,-30.837888650276,175.001512926798));
#30080=CARTESIAN_POINT('Ctrl Pts',(-29.8669939649505,-33.1612402487227,
174.890383137578));
#30081=CARTESIAN_POINT('Ctrl Pts',(-31.8186234857374,-34.4218373646645,
174.779253348358));
#30082=CARTESIAN_POINT('Ctrl Pts',(-33.6889615682118,-33.5776135643453,
174.681100729345));
#30083=CARTESIAN_POINT('Ctrl Pts',(-34.0496820721784,-32.4434638637377,
174.619991373405));
#30084=CARTESIAN_POINT('Ctrl Pts',(-34.0526303238172,-31.9985278132817,
174.595925280538));
#30085=CARTESIAN_POINT('Ctrl Pts',(-34.0556515894835,-31.9982099441992,
175.354074719462));
#30086=CARTESIAN_POINT('Ctrl Pts',(-34.0568507282045,-31.8670800986484,
175.346955464891));
#30087=CARTESIAN_POINT('Ctrl Pts',(-33.9856839203566,-31.0549454486666,
175.302792947247));
#30088=CARTESIAN_POINT('Ctrl Pts',(-32.9044115461845,-29.7460626678129,
175.221587166529));
#30089=CARTESIAN_POINT('Ctrl Pts',(-30.5969869463981,-30.0176407707682,
175.110457377309));
#30090=CARTESIAN_POINT('Ctrl Pts',(-29.5735846782254,-32.1034525425256,
174.99932758809));
#30091=CARTESIAN_POINT('Ctrl Pts',(-30.7708113991622,-34.0945856692598,
174.88819779887));
#30092=CARTESIAN_POINT('Ctrl Pts',(-33.0929781975906,-34.168776706323,174.77706800965));
#30093=CARTESIAN_POINT('Ctrl Pts',(-34.0212735122584,-32.8270205551761,
174.699026983181));
#30094=CARTESIAN_POINT('Ctrl Pts',(-34.057756163478,-32.0739202150757,174.658029219785));
#30095=CARTESIAN_POINT('Ctrl Pts',(-34.0572422162926,-32.0012284952321,
174.654074719462));
#30096=CARTESIAN_POINT('Origin',(-32.,-32.,180.545925280538));
#30097=CARTESIAN_POINT('',(-34.0514446334927,-31.9999002033549,176.054074719462));
#30098=CARTESIAN_POINT('',(-34.0579336950432,-32.0006422348519,175.995925280538));
#30099=CARTESIAN_POINT('',(-34.05475,-31.9999999999998,180.545925280538));
#30100=CARTESIAN_POINT('Ctrl Pts',(-34.0579336950432,-32.0006422348519,
175.995925280538));
#30101=CARTESIAN_POINT('Ctrl Pts',(-34.0552889475514,-31.355553276007,175.960800600544));
#30102=CARTESIAN_POINT('Ctrl Pts',(-33.3811101636429,-30.0253747230238,
175.888632657477));
#30103=CARTESIAN_POINT('Ctrl Pts',(-31.116030889737,-29.7379672254987,175.779421451336));
#30104=CARTESIAN_POINT('Ctrl Pts',(-29.6201584635808,-31.5156985212241,
175.668291662116));
#30105=CARTESIAN_POINT('Ctrl Pts',(-30.302291203249,-33.7366572782917,175.557161872896));
#30106=CARTESIAN_POINT('Ctrl Pts',(-32.5381486228183,-34.368246127532,175.446032083677));
#30107=CARTESIAN_POINT('Ctrl Pts',(-33.9041991402115,-33.1648235619611,
175.358953219557));
#30108=CARTESIAN_POINT('Ctrl Pts',(-34.0542123530794,-32.2416745897686,
175.308917618511));
#30109=CARTESIAN_POINT('Ctrl Pts',(-34.0526241547008,-32.0014692827344,
175.295925280538));
#30110=CARTESIAN_POINT('Ctrl Pts',(-34.0514446334927,-31.9999002033549,
176.054074719462));
#30111=CARTESIAN_POINT('Ctrl Pts',(-34.0515905855125,-31.6630591976112,
176.035881709997));
#30112=CARTESIAN_POINT('Ctrl Pts',(-33.8137831278114,-30.6405614822225,
175.980645437459));
#30113=CARTESIAN_POINT('Ctrl Pts',(-32.2023060098439,-29.5798210767118,
175.888365901848));
#30114=CARTESIAN_POINT('Ctrl Pts',(-30.0764987310374,-30.5173211370632,
175.777236112628));
#30115=CARTESIAN_POINT('Ctrl Pts',(-29.7110589540984,-32.8117528137747,
175.666106323408));
#30116=CARTESIAN_POINT('Ctrl Pts',(-31.4404331998289,-34.3632771184206,
175.554976534188));
#30117=CARTESIAN_POINT('Ctrl Pts',(-33.5383218130657,-33.7911186162802,
175.45096599954));
#30118=CARTESIAN_POINT('Ctrl Pts',(-34.0506113093635,-32.5493814993046,
175.383998727964));
#30119=CARTESIAN_POINT('Ctrl Pts',(-34.0556515894835,-31.9982099441992,
175.354074719462));
#30120=CARTESIAN_POINT('Origin',(-32.,-32.,180.545925280538));
#30121=CARTESIAN_POINT('',(-34.0552853531323,-32.0018424761811,176.754074719462));
#30122=CARTESIAN_POINT('',(-34.0545155617762,-31.9981228561659,176.695925280538));
#30123=CARTESIAN_POINT('',(-34.05475,-31.9999999999998,180.545925280538));
#30124=CARTESIAN_POINT('Ctrl Pts',(-34.0545155617762,-31.9981228561659,
176.695925280538));
#30125=CARTESIAN_POINT('Ctrl Pts',(-34.0560468001527,-31.8292542102386,
176.686770108723));
#30126=CARTESIAN_POINT('Ctrl Pts',(-33.9597818464189,-30.9788389613939,
176.640571673835));
#30127=CARTESIAN_POINT('Ctrl Pts',(-32.7795469135615,-29.6998912483741,
176.557329975874));
#30128=CARTESIAN_POINT('Ctrl Pts',(-30.4904703040065,-30.0974980267845,
176.446200186654));
#30129=CARTESIAN_POINT('Ctrl Pts',(-29.5828989020006,-32.2362539796973,
176.335070397435));
#30130=CARTESIAN_POINT('Ctrl Pts',(-30.8874322125415,-34.1587928522671,
176.223940608215));
#30131=CARTESIAN_POINT('Ctrl Pts',(-33.2101754968556,-34.1056279176698,
176.112810818995));
#30132=CARTESIAN_POINT('Ctrl Pts',(-34.0412910572988,-32.7512989933157,
176.036805709769));
#30133=CARTESIAN_POINT('Ctrl Pts',(-34.0580781566522,-32.0358783355439,
175.997843863617));
#30134=CARTESIAN_POINT('Ctrl Pts',(-34.0579336950432,-32.0006422348519,
175.995925280538));
#30135=CARTESIAN_POINT('Ctrl Pts',(-34.0552853531323,-32.0018424761811,
176.754074719462));
#30136=CARTESIAN_POINT('Ctrl Pts',(-34.050307789522,-31.4625295426181,176.724807955103));
#30137=CARTESIAN_POINT('Ctrl Pts',(-33.5565883388568,-30.232536523623,176.658497927671));
#30138=CARTESIAN_POINT('Ctrl Pts',(-31.4823444699111,-29.6271901683823,
176.555144637166));
#30139=CARTESIAN_POINT('Ctrl Pts',(-29.7257832609726,-31.1478662270158,
176.444014847946));
#30140=CARTESIAN_POINT('Ctrl Pts',(-30.0505605498502,-33.4484058724806,
176.332885058726));
#30141=CARTESIAN_POINT('Ctrl Pts',(-32.1594436821683,-34.4233801713471,
176.221755269507));
#30142=CARTESIAN_POINT('Ctrl Pts',(-33.8010500299471,-33.3839740631711,
176.128818489752));
#30143=CARTESIAN_POINT('Ctrl Pts',(-34.0512934087822,-32.3489099917655,
176.072924973071));
#30144=CARTESIAN_POINT('Ctrl Pts',(-34.0514446334927,-31.9999002033549,
176.054074719462));
#30145=CARTESIAN_POINT('Origin',(-32.,-32.,180.545925280538));
#30146=CARTESIAN_POINT('',(-34.0575044331327,-31.9989451554411,177.454074719462));
#30147=CARTESIAN_POINT('',(-34.0515583595145,-32.0005123628719,177.395925280538));
#30148=CARTESIAN_POINT('',(-34.05475,-31.9999999999998,180.545925280538));
#30149=CARTESIAN_POINT('Ctrl Pts',(-34.0515583595145,-32.0005123628719,
177.395925280538));
#30150=CARTESIAN_POINT('Ctrl Pts',(-34.0507226101221,-31.6260284434929,
177.375696353829));
#30151=CARTESIAN_POINT('Ctrl Pts',(-33.773348995474,-30.5646358407676,177.318424164047));
#30152=CARTESIAN_POINT('Ctrl Pts',(-32.0693869216736,-29.5723717254276,
177.224108711192));
#30153=CARTESIAN_POINT('Ctrl Pts',(-29.9981443603627,-30.6249481189457,
177.112978921973));
#30154=CARTESIAN_POINT('Ctrl Pts',(-29.7589783672204,-32.9359571099918,
177.001849132753));
#30155=CARTESIAN_POINT('Ctrl Pts',(-31.5707710714985,-34.3903882903498,
176.890719343533));
#30156=CARTESIAN_POINT('Ctrl Pts',(-33.5937670274845,-33.7175671934565,
176.788744726128));
#30157=CARTESIAN_POINT('Ctrl Pts',(-34.049851169185,-32.5125232741679,176.723813371796));
#30158=CARTESIAN_POINT('Ctrl Pts',(-34.0545155617762,-31.9981228561659,
176.695925280538));
#30159=CARTESIAN_POINT('Ctrl Pts',(-34.0575044331327,-31.9989451554411,
177.454074719462));
#30160=CARTESIAN_POINT('Ctrl Pts',(-34.0578837517277,-31.9383552486882,
177.450777463283));
#30161=CARTESIAN_POINT('Ctrl Pts',(-34.0279764047848,-31.1974433913819,
177.41043694403));
#30162=CARTESIAN_POINT('Ctrl Pts',(-33.1311884386701,-29.8509058112995,
177.333053161704));
#30163=CARTESIAN_POINT('Ctrl Pts',(-30.8080724679209,-29.8839889892312,
177.221923372484));
#30164=CARTESIAN_POINT('Ctrl Pts',(-29.5757954873418,-31.853622670774,177.110793583265));
#30165=CARTESIAN_POINT('Ctrl Pts',(-30.562124266553,-33.9572192112968,176.999663794045));
#30166=CARTESIAN_POINT('Ctrl Pts',(-32.8643812849987,-34.2695899967097,
176.888534004825));
#30167=CARTESIAN_POINT('Ctrl Pts',(-33.9775854780963,-32.9696108085324,
176.806670979964));
#30168=CARTESIAN_POINT('Ctrl Pts',(-34.0566079461098,-32.1451438088147,
176.761851218177));
#30169=CARTESIAN_POINT('Ctrl Pts',(-34.0552853531323,-32.0018424761811,
176.754074719462));
#30170=CARTESIAN_POINT('Origin',(-32.,-32.,180.545925280538));
#30171=CARTESIAN_POINT('',(-34.0521188940875,-31.9988328896354,178.154074719462));
#30172=CARTESIAN_POINT('',(-34.0563934268478,-32.0016074868405,178.095925280538));
#30173=CARTESIAN_POINT('',(-34.05475,-31.9999999999998,180.545925280538));
#30174=CARTESIAN_POINT('Ctrl Pts',(-34.0563934268478,-32.0016074868405,
178.095925280538));
#30175=CARTESIAN_POINT('Ctrl Pts',(-34.0514421339048,-31.4255805212877,
178.064622598935));
#30176=CARTESIAN_POINT('Ctrl Pts',(-33.4988525573121,-30.1595633443075,
177.99627665426));
#30177=CARTESIAN_POINT('Ctrl Pts',(-31.3531025202806,-29.6591214698943,
177.890887446511));
#30178=CARTESIAN_POINT('Ctrl Pts',(-29.6825069802633,-31.2737629901632,
177.779757657291));
#30179=CARTESIAN_POINT('Ctrl Pts',(-30.1328556342944,-33.5530507267704,
177.668627868071));
#30180=CARTESIAN_POINT('Ctrl Pts',(-32.2919947036809,-34.4110023075711,
177.557498078851));
#30181=CARTESIAN_POINT('Ctrl Pts',(-33.839519683589,-33.3079112493542,177.46659721634));
#30182=CARTESIAN_POINT('Ctrl Pts',(-34.0522530365779,-32.31178436827,177.412739616902));
#30183=CARTESIAN_POINT('Ctrl Pts',(-34.0515583595145,-32.0005123628719,
177.395925280538));
#30184=CARTESIAN_POINT('Ctrl Pts',(-34.0521188940875,-31.9988328896354,
178.154074719462));
#30185=CARTESIAN_POINT('Ctrl Pts',(-34.053500164455,-31.7329725109556,178.139703708389));
#30186=CARTESIAN_POINT('Ctrl Pts',(-33.881982536996,-30.7835296150249,178.088289434242));
#30187=CARTESIAN_POINT('Ctrl Pts',(-32.4498708176529,-29.6134185829238,
177.999831897022));
#30188=CARTESIAN_POINT('Ctrl Pts',(-30.23900588914,-30.3275485827783,177.888702107803));
#30189=CARTESIAN_POINT('Ctrl Pts',(-29.6397721844782,-32.5723003600472,
177.777572318583));
#30190=CARTESIAN_POINT('Ctrl Pts',(-31.2005990238776,-34.293282975036,177.666442529363));
#30191=CARTESIAN_POINT('Ctrl Pts',(-33.42500915292,-33.9266903753032,177.558609996323));
#30192=CARTESIAN_POINT('Ctrl Pts',(-34.0536222695325,-32.619056939197,177.487820726356));
#30193=CARTESIAN_POINT('Ctrl Pts',(-34.0575044331327,-31.9989451554411,
177.454074719462));
#30194=CARTESIAN_POINT('Origin',(-32.,-32.,180.545925280538));
#30195=CARTESIAN_POINT('',(-34.0526600126176,-32.0021813586275,178.854074719462));
#30196=CARTESIAN_POINT('',(-34.0565967959177,-31.9984978779484,178.795925280538));
#30197=CARTESIAN_POINT('',(-34.05475,-31.9999999999998,180.545925280538));
#30198=CARTESIAN_POINT('',(-32.5301702171889,-33.9851743256717,179.));
#30199=CARTESIAN_POINT('Ctrl Pts',(-32.5301702171889,-33.9851743256717,
179.));
#30200=CARTESIAN_POINT('Ctrl Pts',(-33.190239790753,-33.8088929660697,178.962956736927));
#30201=CARTESIAN_POINT('Ctrl Pts',(-33.9248822331584,-33.1125975988824,
178.914314976748));
#30202=CARTESIAN_POINT('Ctrl Pts',(-34.0542719683944,-32.2164508334355,
178.865673216568));
#30203=CARTESIAN_POINT('Ctrl Pts',(-34.0526600126176,-32.0021813586275,
178.854074719462));
#30204=CARTESIAN_POINT('',(-31.4686665305884,-33.9887337536768,179.));
#30205=CARTESIAN_POINT('Origin',(-32.,-32.,179.));
#30206=CARTESIAN_POINT('Ctrl Pts',(-31.4686656554569,-33.9887364314853,
179.));
#30207=CARTESIAN_POINT('Ctrl Pts',(-32.1131053683168,-34.1599912916281,
178.963685183163));
#30208=CARTESIAN_POINT('Ctrl Pts',(-33.4929540196752,-33.8408666928276,
178.895660276675));
#30209=CARTESIAN_POINT('Ctrl Pts',(-34.0517538459607,-32.5817482158403,
178.827635370188));
#30210=CARTESIAN_POINT('Ctrl Pts',(-34.0565967959177,-31.9984978779484,
178.795925280538));
#30211=CARTESIAN_POINT('Origin',(32.,32.,172.));
#30212=CARTESIAN_POINT('',(30.3314948391898,32.0006151205084,166.67148036339));
#30213=CARTESIAN_POINT('',(30.3351639991694,32.0014707476285,166.47851963661));
#30214=CARTESIAN_POINT('',(30.334,32.,172.));
#30215=CARTESIAN_POINT('',(32.6750771856741,30.4769022377462,166.));
#30216=CARTESIAN_POINT('Ctrl Pts',(30.3351639991694,32.0014707476285,166.47851963661));
#30217=CARTESIAN_POINT('Ctrl Pts',(30.3338126182148,32.1712147141657,166.467186143366));
#30218=CARTESIAN_POINT('Ctrl Pts',(30.3576887331272,32.3405776321984,166.455852650123));
#30219=CARTESIAN_POINT('Ctrl Pts',(30.4083704059759,32.5014768155649,166.444519156879));
#30220=CARTESIAN_POINT('Ctrl Pts',(30.574022292818,33.0273721110032,166.407475893806));
#30221=CARTESIAN_POINT('Ctrl Pts',(31.0260364143234,33.4628498154943,166.370432630732));
#30222=CARTESIAN_POINT('Ctrl Pts',(31.557848973733,33.6090488989997,166.333389367659));
#30223=CARTESIAN_POINT('Ctrl Pts',(32.0896615331426,33.755247982505,166.296346104586));
#30224=CARTESIAN_POINT('Ctrl Pts',(32.7012725304564,33.6121684450247,166.259302841513));
#30225=CARTESIAN_POINT('Ctrl Pts',(33.11224753475,33.2444370308748,166.222259578439));
#30226=CARTESIAN_POINT('Ctrl Pts',(33.5232225390436,32.876705616725,166.185216315366));
#30227=CARTESIAN_POINT('Ctrl Pts',(33.7335615503171,32.2843223259056,166.148173052293));
#30228=CARTESIAN_POINT('Ctrl Pts',(33.6481325428054,31.7404871965806,166.11112978922));
#30229=CARTESIAN_POINT('Ctrl Pts',(33.5627035352937,31.1966520672555,166.074086526147));
#30230=CARTESIAN_POINT('Ctrl Pts',(33.1815065089967,30.7013650994246,166.037043263073));
#30231=CARTESIAN_POINT('Ctrl Pts',(32.6750771856741,30.4769022377462,166.));
#30232=CARTESIAN_POINT('',(30.334,32.,166.));
#30233=CARTESIAN_POINT('Origin',(32.,32.,166.));
#30234=CARTESIAN_POINT('',(30.334,32.,165.));
#30235=CARTESIAN_POINT('',(30.334,32.,172.));
#30236=CARTESIAN_POINT('Origin',(32.,32.,165.));
#30237=CARTESIAN_POINT('',(30.3853154136487,31.5775542237606,166.));
#30238=CARTESIAN_POINT('Origin',(32.,32.,166.));
#30239=CARTESIAN_POINT('Ctrl Pts',(30.3853131747228,31.5775537673674,166.));
#30240=CARTESIAN_POINT('Ctrl Pts',(30.5228540701568,31.0546921657189,166.036314816837));
#30241=CARTESIAN_POINT('Ctrl Pts',(30.9381272764309,30.6037509899059,166.072629633674));
#30242=CARTESIAN_POINT('Ctrl Pts',(31.4484542245311,30.4250924216085,166.108944450512));
#30243=CARTESIAN_POINT('Ctrl Pts',(31.9690179238214,30.2428501050523,166.145987713585));
#30244=CARTESIAN_POINT('Ctrl Pts',(32.5884870162225,30.3439234982855,166.183030976658));
#30245=CARTESIAN_POINT('Ctrl Pts',(33.0238560935078,30.6822432557804,166.220074239731));
#30246=CARTESIAN_POINT('Ctrl Pts',(33.4592251707931,31.0205630132753,166.257117502805));
#30247=CARTESIAN_POINT('Ctrl Pts',(33.7104942329626,31.596129135032,166.294160765878));
#30248=CARTESIAN_POINT('Ctrl Pts',(33.6624582200325,32.1454771760265,166.331204028951));
#30249=CARTESIAN_POINT('Ctrl Pts',(33.6144222071025,32.6948252170211,166.368247292024));
#30250=CARTESIAN_POINT('Ctrl Pts',(33.267081119073,33.2179551772535,166.405290555098));
#30251=CARTESIAN_POINT('Ctrl Pts',(32.7794871827661,33.4755290749605,166.442333818171));
#30252=CARTESIAN_POINT('Ctrl Pts',(32.2918932464593,33.7331029726675,166.479377081244));
#30253=CARTESIAN_POINT('Ctrl Pts',(31.6640464618751,33.7251208078489,166.516420344317));
#30254=CARTESIAN_POINT('Ctrl Pts',(31.1831916842018,33.4552138375921,166.553463607391));
#30255=CARTESIAN_POINT('Ctrl Pts',(30.7023369065286,33.1853068673354,166.590506870464));
#30256=CARTESIAN_POINT('Ctrl Pts',(30.3684741357662,32.6534750916404,166.627550133537));
#30257=CARTESIAN_POINT('Ctrl Pts',(30.33440389687,32.1030923269707,166.66459339661));
#30258=CARTESIAN_POINT('Ctrl Pts',(30.3322924863733,32.0689838503585,166.666889052204));
#30259=CARTESIAN_POINT('Ctrl Pts',(30.3313324482509,32.0348041274879,166.669184707797));
#30260=CARTESIAN_POINT('Ctrl Pts',(30.3314948391898,32.0006151205084,166.67148036339));
#30261=CARTESIAN_POINT('Origin',(32.,32.,172.));
#30262=CARTESIAN_POINT('',(30.3358443517282,32.0011304728208,167.37148036339));
#30263=CARTESIAN_POINT('',(30.3361975399048,31.9991033790422,167.17851963661));
#30264=CARTESIAN_POINT('',(30.334,32.,172.));
#30265=CARTESIAN_POINT('Ctrl Pts',(30.3361975399048,31.9991033790422,167.17851963661));
#30266=CARTESIAN_POINT('Ctrl Pts',(30.3378409217978,32.3352358809299,167.156112388472));
#30267=CARTESIAN_POINT('Ctrl Pts',(30.4366194744036,32.6722563487497,167.133705140335));
#30268=CARTESIAN_POINT('Ctrl Pts',(30.6258906729461,32.9469160000523,167.111297892197));
#30269=CARTESIAN_POINT('Ctrl Pts',(30.9387904434473,33.4009784380794,167.074254629124));
#30270=CARTESIAN_POINT('Ctrl Pts',(31.4990076363489,33.6846080609293,167.037211366051));
#30271=CARTESIAN_POINT('Ctrl Pts',(32.050193769109,33.6680232454317,167.000168102978));
#30272=CARTESIAN_POINT('Ctrl Pts',(32.6013799018691,33.6514384299341,166.963124839904));
#30273=CARTESIAN_POINT('Ctrl Pts',(33.1435349744877,33.334639176089,166.926081576831));
#30274=CARTESIAN_POINT('Ctrl Pts',(33.4285638919976,32.8625793893597,166.889038313758));
#30275=CARTESIAN_POINT('Ctrl Pts',(33.7135928095075,32.3905196026303,166.851995050685));
#30276=CARTESIAN_POINT('Ctrl Pts',(33.7414955719087,31.7631992830168,166.814951787611));
#30277=CARTESIAN_POINT('Ctrl Pts',(33.4995200560992,31.2677006586916,166.777908524538));
#30278=CARTESIAN_POINT('Ctrl Pts',(33.2575445402896,30.7722020343664,166.740865261465));
#30279=CARTESIAN_POINT('Ctrl Pts',(32.7456907462693,30.4085251053296,166.703821998392));
#30280=CARTESIAN_POINT('Ctrl Pts',(32.1981475596803,30.343037902655,166.666778735318));
#30281=CARTESIAN_POINT('Ctrl Pts',(31.6506043730913,30.2775506999803,166.629735472245));
#30282=CARTESIAN_POINT('Ctrl Pts',(31.0673717939337,30.5102532236679,166.592692209172));
#30283=CARTESIAN_POINT('Ctrl Pts',(30.7154003304443,30.9347609287045,166.555648946099));
#30284=CARTESIAN_POINT('Ctrl Pts',(30.4711155519947,31.2293892762612,166.529939176269));
#30285=CARTESIAN_POINT('Ctrl Pts',(30.3382295759115,31.6164104475238,166.504229406439));
#30286=CARTESIAN_POINT('Ctrl Pts',(30.3351639991694,32.0014707476285,166.47851963661));
#30287=CARTESIAN_POINT('Ctrl Pts',(30.3314948391898,32.0006151205084,166.67148036339));
#30288=CARTESIAN_POINT('Ctrl Pts',(30.3339528283677,31.4831219050117,166.70622797087));
#30289=CARTESIAN_POINT('Ctrl Pts',(30.5935659814505,30.9635016450492,166.74097557835));
#30290=CARTESIAN_POINT('Ctrl Pts',(31.0099645669336,30.6566269199928,166.77572318583));
#30291=CARTESIAN_POINT('Ctrl Pts',(31.4538731829234,30.329478031329,166.812766448903));
#30292=CARTESIAN_POINT('Ctrl Pts',(32.075968121933,30.2441140076456,166.849809711977));
#30293=CARTESIAN_POINT('Ctrl Pts',(32.5915885607143,30.4395994910286,166.88685297505));
#30294=CARTESIAN_POINT('Ctrl Pts',(33.1072089994956,30.6350849744116,166.923896238123));
#30295=CARTESIAN_POINT('Ctrl Pts',(33.5163549380486,31.1114199648611,166.960939501196));
#30296=CARTESIAN_POINT('Ctrl Pts',(33.6318002467858,31.6506349121444,166.99798276427));
#30297=CARTESIAN_POINT('Ctrl Pts',(33.747245555523,32.1898498594278,167.035026027343));
#30298=CARTESIAN_POINT('Ctrl Pts',(33.5689902344443,32.791944763545,167.072069290416));
#30299=CARTESIAN_POINT('Ctrl Pts',(33.1786045071229,33.1814048707878,167.109112553489));
#30300=CARTESIAN_POINT('Ctrl Pts',(32.7882187798016,33.5708649780306,167.146155816562));
#30301=CARTESIAN_POINT('Ctrl Pts',(32.1857026462376,33.747690288399,167.183199079636));
#30302=CARTESIAN_POINT('Ctrl Pts',(31.6467634583476,33.6309661992293,167.220242342709));
#30303=CARTESIAN_POINT('Ctrl Pts',(31.1078242704576,33.5142421100596,167.257285605782));
#30304=CARTESIAN_POINT('Ctrl Pts',(30.6324620282417,33.1039686213518,167.294328868856));
#30305=CARTESIAN_POINT('Ctrl Pts',(30.4382002913112,32.5878848039827,167.331372131929));
#30306=CARTESIAN_POINT('Ctrl Pts',(30.3680886249107,32.4016232323021,167.344741542416));
#30307=CARTESIAN_POINT('Ctrl Pts',(30.3345926862457,32.201578966841,167.358110952903));
#30308=CARTESIAN_POINT('Ctrl Pts',(30.3358443517282,32.0011304728208,167.37148036339));
#30309=CARTESIAN_POINT('Origin',(32.,32.,172.));
#30310=CARTESIAN_POINT('',(30.3355908397978,31.9987501653433,168.07148036339));
#30311=CARTESIAN_POINT('',(30.3318493159965,31.9990863362845,167.87851963661));
#30312=CARTESIAN_POINT('',(30.334,32.,172.));
#30313=CARTESIAN_POINT('Ctrl Pts',(30.3318493159965,31.9990863362845,167.87851963661));
#30314=CARTESIAN_POINT('Ctrl Pts',(30.3351438813141,32.4979922732345,167.845038633578));
#30315=CARTESIAN_POINT('Ctrl Pts',(30.5738270354749,32.9996326545442,167.811557630547));
#30316=CARTESIAN_POINT('Ctrl Pts',(30.9647290575101,33.3088316952852,167.778076627516));
#30317=CARTESIAN_POINT('Ctrl Pts',(31.3972216690526,33.6509284179376,167.741033364442));
#30318=CARTESIAN_POINT('Ctrl Pts',(32.0160473933025,33.7574551714892,167.703990101369));
#30319=CARTESIAN_POINT('Ctrl Pts',(32.538034988592,33.5796659719367,167.666946838296));
#30320=CARTESIAN_POINT('Ctrl Pts',(33.0600225838815,33.4018767723843,167.629903575223));
#30321=CARTESIAN_POINT('Ctrl Pts',(33.4851720502105,32.9397716197278,167.592860312149));
#30322=CARTESIAN_POINT('Ctrl Pts',(33.6189371865014,32.4048071616505,167.555817049076));
#30323=CARTESIAN_POINT('Ctrl Pts',(33.7527023227924,31.8698427035731,167.518773786003));
#30324=CARTESIAN_POINT('Ctrl Pts',(33.5950831290453,31.2620189400749,167.48173052293));
#30325=CARTESIAN_POINT('Ctrl Pts',(33.21820551876,30.859473064477,167.444687259856));
#30326=CARTESIAN_POINT('Ctrl Pts',(32.8413279084747,30.4569271888792,167.407643996783));
#30327=CARTESIAN_POINT('Ctrl Pts',(32.2451918816511,30.2596592011817,167.37060073371));
#30328=CARTESIAN_POINT('Ctrl Pts',(31.7025855934752,30.3579371810217,167.333557470637));
#30329=CARTESIAN_POINT('Ctrl Pts',(31.1599793052994,30.4562151608616,167.296514207563));
#30330=CARTESIAN_POINT('Ctrl Pts',(30.6709027557713,30.8500391082389,167.25947094449));
#30331=CARTESIAN_POINT('Ctrl Pts',(30.4591556550577,31.3591987085298,167.222427681417));
#30332=CARTESIAN_POINT('Ctrl Pts',(30.3754931083076,31.5603707138087,167.207791666481));
#30333=CARTESIAN_POINT('Ctrl Pts',(30.3351241121558,31.779547622449,167.193155651545));
#30334=CARTESIAN_POINT('Ctrl Pts',(30.3361975399048,31.9991033790422,167.17851963661));
#30335=CARTESIAN_POINT('Ctrl Pts',(30.3358443517282,32.0011304728208,167.37148036339));
#30336=CARTESIAN_POINT('Ctrl Pts',(30.3380607354761,31.6461867673313,167.395154215976));
#30337=CARTESIAN_POINT('Ctrl Pts',(30.4492298770393,31.2899755840575,167.418828068562));
#30338=CARTESIAN_POINT('Ctrl Pts',(30.658979462611,31.0067776828098,167.442501921148));
#30339=CARTESIAN_POINT('Ctrl Pts',(30.9871816024865,30.5636485250366,167.479545184222));
#30340=CARTESIAN_POINT('Ctrl Pts',(31.5567471138823,30.2992843555205,167.516588447295));
#30341=CARTESIAN_POINT('Ctrl Pts',(32.1070459976037,30.3346568202484,167.553631710368));
#30342=CARTESIAN_POINT('Ctrl Pts',(32.6573448813252,30.3700292849762,167.590674973441));
#30343=CARTESIAN_POINT('Ctrl Pts',(33.1883771373722,30.7051383839478,167.627718236515));
#30344=CARTESIAN_POINT('Ctrl Pts',(33.4571452403435,31.1866399931067,167.664761499588));
#30345=CARTESIAN_POINT('Ctrl Pts',(33.7259133433149,31.6681416022655,167.701804762661));
#30346=CARTESIAN_POINT('Ctrl Pts',(33.7324172932105,32.2960357216114,167.738848025734));
#30347=CARTESIAN_POINT('Ctrl Pts',(33.4736809396483,32.7830014153016,167.775891288808));
#30348=CARTESIAN_POINT('Ctrl Pts',(33.2149445860862,33.2699671089917,167.812934551881));
#30349=CARTESIAN_POINT('Ctrl Pts',(32.6909679290662,33.6160043770262,167.849977814954));
#30350=CARTESIAN_POINT('Ctrl Pts',(32.1415198349773,33.6627684376593,167.887021078027));
#30351=CARTESIAN_POINT('Ctrl Pts',(31.5920717408885,33.7095324982925,167.924064341101));
#30352=CARTESIAN_POINT('Ctrl Pts',(31.0171522097308,33.4570233515244,167.961107604174));
#30353=CARTESIAN_POINT('Ctrl Pts',(30.6798413068547,33.0207878158059,167.998150867247));
#30354=CARTESIAN_POINT('Ctrl Pts',(30.4572651756015,32.7329358162782,168.022594032628));
#30355=CARTESIAN_POINT('Ctrl Pts',(30.3381457458446,32.3650878741953,168.047037198009));
#30356=CARTESIAN_POINT('Ctrl Pts',(30.3355908397978,31.9987501653433,168.07148036339));
#30357=CARTESIAN_POINT('Origin',(32.,32.,172.));
#30358=CARTESIAN_POINT('',(30.3313481286181,31.9995820784511,168.77148036339));
#30359=CARTESIAN_POINT('',(30.3334458852718,32.0014790085581,168.57851963661));
#30360=CARTESIAN_POINT('',(30.334,32.,172.));
#30361=CARTESIAN_POINT('Ctrl Pts',(30.3334458852718,32.0014790085581,168.57851963661));
#30362=CARTESIAN_POINT('Ctrl Pts',(30.3324126167116,32.113688095481,168.571008141758));
#30363=CARTESIAN_POINT('Ctrl Pts',(30.3427777067538,32.225707371916,168.563496646906));
#30364=CARTESIAN_POINT('Ctrl Pts',(30.3652410885464,32.3352456102263,168.555985152054));
#30365=CARTESIAN_POINT('Ctrl Pts',(30.4760202314001,32.875438189497,168.51894188898));
#30366=CARTESIAN_POINT('Ctrl Pts',(30.8810312884822,33.3552916224022,168.481898625907));
#30367=CARTESIAN_POINT('Ctrl Pts',(31.3949433957783,33.5552275793839,168.444855362834));
#30368=CARTESIAN_POINT('Ctrl Pts',(31.9088555030743,33.7551635363657,168.407812099761));
#30369=CARTESIAN_POINT('Ctrl Pts',(32.5316686605844,33.675182017424,168.370768836687));
#30370=CARTESIAN_POINT('Ctrl Pts',(32.9783869452582,33.3518821330796,168.333725573614));
#30371=CARTESIAN_POINT('Ctrl Pts',(33.425105229932,33.0285822487352,168.296682310541));
#30372=CARTESIAN_POINT('Ctrl Pts',(33.6957286417695,32.4619639989881,168.259639047468));
#30373=CARTESIAN_POINT('Ctrl Pts',(33.6664213733557,31.9113088202529,168.222595784395));
#30374=CARTESIAN_POINT('Ctrl Pts',(33.6371141049419,31.3606536415177,168.185552521321));
#30375=CARTESIAN_POINT('Ctrl Pts',(33.3078761562767,30.8259615337943,168.148509258248));
#30376=CARTESIAN_POINT('Ctrl Pts',(32.8293650306118,30.5519047110331,168.111465995175));
#30377=CARTESIAN_POINT('Ctrl Pts',(32.3508539049469,30.2778478882719,168.074422732102));
#30378=CARTESIAN_POINT('Ctrl Pts',(31.7230696022823,30.2644263504728,168.037379469028));
#30379=CARTESIAN_POINT('Ctrl Pts',(31.2332828090634,30.517781710982,168.000336205955));
#30380=CARTESIAN_POINT('Ctrl Pts',(30.7434960158445,30.7711370714911,167.963292942882));
#30381=CARTESIAN_POINT('Ctrl Pts',(30.3917067320712,31.2912693303086,167.926249679809));
#30382=CARTESIAN_POINT('Ctrl Pts',(30.338891839602,31.840168805594,167.889206416735));
#30383=CARTESIAN_POINT('Ctrl Pts',(30.3338129030979,31.8929536443358,167.885644156694));
#30384=CARTESIAN_POINT('Ctrl Pts',(30.331498785925,31.9460045130738,167.882081896652));
#30385=CARTESIAN_POINT('Ctrl Pts',(30.3318493159965,31.9990863362845,167.87851963661));
#30386=CARTESIAN_POINT('Ctrl Pts',(30.3355908397978,31.9987501653433,168.07148036339));
#30387=CARTESIAN_POINT('Ctrl Pts',(30.3342738227387,31.8099083828695,168.084080461082));
#30388=CARTESIAN_POINT('Ctrl Pts',(30.363930950585,31.6214679075983,168.096680558775));
#30389=CARTESIAN_POINT('Ctrl Pts',(30.4263577007272,31.4445932559108,168.109280656467));
#30390=CARTESIAN_POINT('Ctrl Pts',(30.6098872720703,30.924596156403,168.14632391954));
#30391=CARTESIAN_POINT('Ctrl Pts',(31.0766486893511,30.5045638820563,168.183367182613));
#30392=CARTESIAN_POINT('Ctrl Pts',(31.6130544602,30.3767009245792,168.220410445687));
#30393=CARTESIAN_POINT('Ctrl Pts',(32.1494602310488,30.2488379671021,168.25745370876));
#30394=CARTESIAN_POINT('Ctrl Pts',(32.7555103554658,30.4131443264948,168.294496971833));
#30395=CARTESIAN_POINT('Ctrl Pts',(33.153879582064,30.7944343033687,168.331540234906));
#30396=CARTESIAN_POINT('Ctrl Pts',(33.5522488086622,31.1757242802426,168.368583497979));
#30397=CARTESIAN_POINT('Ctrl Pts',(33.7429371374417,31.7739978745979,168.405626761053));
#30398=CARTESIAN_POINT('Ctrl Pts',(33.6386866234236,32.315488333781,168.442670024126));
#30399=CARTESIAN_POINT('Ctrl Pts',(33.5344361094055,32.8569787929641,168.479713287199));
#30400=CARTESIAN_POINT('Ctrl Pts',(33.1352467525898,33.3416861169752,168.516756550273));
#30401=CARTESIAN_POINT('Ctrl Pts',(32.6237854379909,33.5478108625037,168.553799813346));
#30402=CARTESIAN_POINT('Ctrl Pts',(32.112324123392,33.7539356080322,168.590843076419));
#30403=CARTESIAN_POINT('Ctrl Pts',(31.4885908510098,33.6814777750783,168.627886339492));
#30404=CARTESIAN_POINT('Ctrl Pts',(31.0380025843074,33.3635936751443,168.664929602565));
#30405=CARTESIAN_POINT('Ctrl Pts',(30.6059805047824,33.0588077762426,168.70044652284));
#30406=CARTESIAN_POINT('Ctrl Pts',(30.3331287484094,32.5284041757398,168.735963443115));
#30407=CARTESIAN_POINT('Ctrl Pts',(30.3313481286181,31.9995820784511,168.77148036339));
#30408=CARTESIAN_POINT('Origin',(32.,32.,172.));
#30409=CARTESIAN_POINT('',(30.3343646149627,32.0015150182665,169.47148036339));
#30410=CARTESIAN_POINT('',(30.3366835095906,31.9999843286223,169.27851963661));
#30411=CARTESIAN_POINT('',(30.334,32.,172.));
#30412=CARTESIAN_POINT('Ctrl Pts',(30.3366835095906,31.9999843286223,169.27851963661));
#30413=CARTESIAN_POINT('Ctrl Pts',(30.3367069203412,32.2789861477807,169.259934386864));
#30414=CARTESIAN_POINT('Ctrl Pts',(30.4031258058091,32.5579984414641,169.241349137118));
#30415=CARTESIAN_POINT('Ctrl Pts',(30.535878000075,32.8007328436966,169.222763887372));
#30416=CARTESIAN_POINT('Ctrl Pts',(30.8004735542359,33.2845398649497,169.185720624299));
#30417=CARTESIAN_POINT('Ctrl Pts',(31.3285889555581,33.6242270679139,169.148677361226));
#30418=CARTESIAN_POINT('Ctrl Pts',(31.8785614599778,33.6643554303822,169.111634098152));
#30419=CARTESIAN_POINT('Ctrl Pts',(32.4285339643976,33.7044837928504,169.074590835079));
#30420=CARTESIAN_POINT('Ctrl Pts',(33.000363571915,33.4450533148228,169.037547572006));
#30421=CARTESIAN_POINT('Ctrl Pts',(33.3323841547577,33.0047779763573,169.000504308933));
#30422=CARTESIAN_POINT('Ctrl Pts',(33.6644047376003,32.5645026378919,168.963461045859));
#30423=CARTESIAN_POINT('Ctrl Pts',(33.7566162957683,31.9433824389887,168.926417782786));
#30424=CARTESIAN_POINT('Ctrl Pts',(33.5668233202183,31.4256386147494,168.889374519713));
#30425=CARTESIAN_POINT('Ctrl Pts',(33.3770303446684,30.9078947905101,168.85233125664));
#30426=CARTESIAN_POINT('Ctrl Pts',(32.9052328354007,30.4935273409347,168.815287993566));
#30427=CARTESIAN_POINT('Ctrl Pts',(32.367322774485,30.3721485642009,168.778244730493));
#30428=CARTESIAN_POINT('Ctrl Pts',(31.8294127135693,30.2507697874672,168.74120146742));
#30429=CARTESIAN_POINT('Ctrl Pts',(31.2253901010056,30.4223796835752,168.704158204347));
#30430=CARTESIAN_POINT('Ctrl Pts',(30.8316524090365,30.8084504944473,168.667114941273));
#30431=CARTESIAN_POINT('Ctrl Pts',(30.517755379064,31.1162353049026,168.637583173052));
#30432=CARTESIAN_POINT('Ctrl Pts',(30.3375082254896,31.5603241102872,168.608051404831));
#30433=CARTESIAN_POINT('Ctrl Pts',(30.3334458852718,32.0014790085581,168.57851963661));
#30434=CARTESIAN_POINT('Ctrl Pts',(30.3313481286181,31.9995820784511,168.77148036339));
#30435=CARTESIAN_POINT('Ctrl Pts',(30.3312716063247,31.9768559019265,168.773006706189));
#30436=CARTESIAN_POINT('Ctrl Pts',(30.3316957139953,31.9541326462143,168.774533048987));
#30437=CARTESIAN_POINT('Ctrl Pts',(30.332629333074,31.9314303438645,168.776059391785));
#30438=CARTESIAN_POINT('Ctrl Pts',(30.3552876095656,31.3804614794328,168.813102654858));
#30439=CARTESIAN_POINT('Ctrl Pts',(30.6780474235711,30.8418341174834,168.850145917932));
#30440=CARTESIAN_POINT('Ctrl Pts',(31.1532156343118,30.5620212182661,168.887189181005));
#30441=CARTESIAN_POINT('Ctrl Pts',(31.6283838450525,30.2822083190488,168.924232444078));
#30442=CARTESIAN_POINT('Ctrl Pts',(32.2559604525283,30.2612098825636,168.961275707151));
#30443=CARTESIAN_POINT('Ctrl Pts',(32.748769804042,30.5086346794834,168.998318970225));
#30444=CARTESIAN_POINT('Ctrl Pts',(33.2415791555557,30.7560594764032,169.035362233298));
#30445=CARTESIAN_POINT('Ctrl Pts',(33.5996212511073,31.271907506728,169.072405496371));
#30446=CARTESIAN_POINT('Ctrl Pts',(33.6590579691791,31.8201295088524,169.109448759444));
#30447=CARTESIAN_POINT('Ctrl Pts',(33.7184946872509,32.3683515109768,169.146492022518));
#30448=CARTESIAN_POINT('Ctrl Pts',(33.479326027843,32.9489474849006,169.183535285591));
#30449=CARTESIAN_POINT('Ctrl Pts',(33.0509942726601,33.2962398611062,169.220578548664));
#30450=CARTESIAN_POINT('Ctrl Pts',(32.6226625174773,33.6435322373118,169.257621811737));
#30451=CARTESIAN_POINT('Ctrl Pts',(32.0051676665196,33.7575210157991,169.294665074811));
#30452=CARTESIAN_POINT('Ctrl Pts',(31.4810720153599,33.5860455496112,169.331708337884));
#30453=CARTESIAN_POINT('Ctrl Pts',(30.9569763642001,33.4145700834232,169.368751600957));
#30454=CARTESIAN_POINT('Ctrl Pts',(30.5262799128384,32.95763037256,169.40579486403));
#30455=CARTESIAN_POINT('Ctrl Pts',(30.3860670220631,32.4243195510599,169.442838127103));
#30456=CARTESIAN_POINT('Ctrl Pts',(30.3499290002398,32.2868657263839,169.452385539199));
#30457=CARTESIAN_POINT('Ctrl Pts',(30.3330872953841,32.144338701851,169.461932951295));
#30458=CARTESIAN_POINT('Ctrl Pts',(30.3343646149627,32.0015150182665,169.47148036339));
#30459=CARTESIAN_POINT('Origin',(32.,32.,172.));
#30460=CARTESIAN_POINT('',(30.3365390106164,31.9994923848488,170.17148036339));
#30461=CARTESIAN_POINT('',(30.3333883716037,31.9985292209557,169.97851963661));
#30462=CARTESIAN_POINT('',(30.334,32.,172.));
#30463=CARTESIAN_POINT('Ctrl Pts',(30.3333883716037,31.9985292209557,169.97851963661));
#30464=CARTESIAN_POINT('Ctrl Pts',(30.3374605996998,32.4415454791333,169.94886063197));
#30465=CARTESIAN_POINT('Ctrl Pts',(30.5194350922995,32.8875165487396,169.91920162733));
#30466=CARTESIAN_POINT('Ctrl Pts',(30.835741762519,33.1955455131847,169.88954262269));
#30467=CARTESIAN_POINT('Ctrl Pts',(31.2307999021651,33.5802650310069,169.852499359617));
#30468=CARTESIAN_POINT('Ctrl Pts',(31.8354069406125,33.7498044129371,169.815456096544));
#30469=CARTESIAN_POINT('Ctrl Pts',(32.3728979754128,33.6265833570929,169.778412833471));
#30470=CARTESIAN_POINT('Ctrl Pts',(32.910389010213,33.5033623012487,169.741369570397));
#30471=CARTESIAN_POINT('Ctrl Pts',(33.3807640413661,33.0873808076302,169.704326307324));
#30472=CARTESIAN_POINT('Ctrl Pts',(33.5687820051189,32.5689897521516,169.667283044251));
#30473=CARTESIAN_POINT('Ctrl Pts',(33.7567999688717,32.050598696673,169.630239781178));
#30474=CARTESIAN_POINT('Ctrl Pts',(33.6624608652242,31.4297980793344,169.593196518104));
#30475=CARTESIAN_POINT('Ctrl Pts',(33.3289337564728,30.9906628964783,169.556153255031));
#30476=CARTESIAN_POINT('Ctrl Pts',(32.9954066477213,30.5515277136221,169.519109991958));
#30477=CARTESIAN_POINT('Ctrl Pts',(32.4226915338659,30.2940579652485,169.482066728885));
#30478=CARTESIAN_POINT('Ctrl Pts',(31.872859745589,30.3360704121425,169.445023465812));
#30479=CARTESIAN_POINT('Ctrl Pts',(31.323027957312,30.3780828590364,169.407980202738));
#30480=CARTESIAN_POINT('Ctrl Pts',(30.7960794946136,30.7195775011981,169.370936939665));
#30481=CARTESIAN_POINT('Ctrl Pts',(30.5331431167641,31.2042882420498,169.333893676592));
#30482=CARTESIAN_POINT('Ctrl Pts',(30.4021264955506,31.4458111688191,169.315435663264));
#30483=CARTESIAN_POINT('Ctrl Pts',(30.3366602591122,31.7228925829223,169.296977649937));
#30484=CARTESIAN_POINT('Ctrl Pts',(30.3366835095906,31.9999843286223,169.27851963661));
#30485=CARTESIAN_POINT('Ctrl Pts',(30.3343646149627,32.0015150182665,169.47148036339));
#30486=CARTESIAN_POINT('Ctrl Pts',(30.3380432022527,31.5901932191653,169.498976214368));
#30487=CARTESIAN_POINT('Ctrl Pts',(30.492000619283,31.1764109357676,169.526472065346));
#30488=CARTESIAN_POINT('Ctrl Pts',(30.7681159877996,30.8742609009325,169.553967916323));
#30489=CARTESIAN_POINT('Ctrl Pts',(31.1401071745005,30.467195004442,169.591011179397));
#30490=CARTESIAN_POINT('Ctrl Pts',(31.7338188780912,30.262745143598,169.62805444247));
#30491=CARTESIAN_POINT('Ctrl Pts',(32.2775718422762,30.3544664661395,169.665097705543));
#30492=CARTESIAN_POINT('Ctrl Pts',(32.8213248064612,30.4461877886809,169.702140968616));
#30493=CARTESIAN_POINT('Ctrl Pts',(33.3151190312405,30.8340802946078,169.73918423169));
#30494=CARTESIAN_POINT('Ctrl Pts',(33.5329969568429,31.3406464764675,169.776227494763));
#30495=CARTESIAN_POINT('Ctrl Pts',(33.7508748824452,31.8472126583272,169.813270757836));
#30496=CARTESIAN_POINT('Ctrl Pts',(33.6928365088705,32.4724525161198,169.850314020909));
#30497=CARTESIAN_POINT('Ctrl Pts',(33.3854398811667,32.9302596811413,169.887357283983));
#30498=CARTESIAN_POINT('Ctrl Pts',(33.0780432534628,33.3880668461628,169.924400547056));
#30499=CARTESIAN_POINT('Ctrl Pts',(32.5212883716297,33.6784413184132,169.961443810129));
#30500=CARTESIAN_POINT('Ctrl Pts',(31.9699432507166,33.6685093138807,169.998487073202));
#30501=CARTESIAN_POINT('Ctrl Pts',(31.4185981298035,33.6585773093483,170.035530336275));
#30502=CARTESIAN_POINT('Ctrl Pts',(30.8726627698104,33.348338828033,170.072573599349));
#30503=CARTESIAN_POINT('Ctrl Pts',(30.5819542312589,32.8797573167866,170.109616862422));
#30504=CARTESIAN_POINT('Ctrl Pts',(30.4201232039306,32.6189083313048,170.130238029411));
#30505=CARTESIAN_POINT('Ctrl Pts',(30.3373844972543,32.3089903740528,170.150859196401));
#30506=CARTESIAN_POINT('Ctrl Pts',(30.3365390106164,31.9994923848488,170.17148036339));
#30507=CARTESIAN_POINT('Origin',(32.,32.,172.));
#30508=CARTESIAN_POINT('',(30.3325050746568,31.9987546321113,170.87148036339));
#30509=CARTESIAN_POINT('',(30.3318905055228,32.0009409351765,170.67851963661));
#30510=CARTESIAN_POINT('',(30.334,32.,172.));
#30511=CARTESIAN_POINT('Ctrl Pts',(30.3318905055228,32.0009409351765,170.67851963661));
#30512=CARTESIAN_POINT('Ctrl Pts',(30.3315188134717,32.0559223042009,170.674830140149));
#30513=CARTESIAN_POINT('Ctrl Pts',(30.3340015814678,32.1108696948638,170.671140643689));
#30514=CARTESIAN_POINT('Ctrl Pts',(30.3394492078326,32.1655215522844,170.667451147229));
#30515=CARTESIAN_POINT('Ctrl Pts',(30.3941444375797,32.7142368454346,170.630407884155));
#30516=CARTESIAN_POINT('Ctrl Pts',(30.7477137303999,33.2331607590674,170.593364621082));
#30517=CARTESIAN_POINT('Ctrl Pts',(31.2383656950483,33.4848365240522,170.556321358009));
#30518=CARTESIAN_POINT('Ctrl Pts',(31.7290176596967,33.736512289037,170.519278094935));
#30519=CARTESIAN_POINT('Ctrl Pts',(32.3567522961734,33.7209399053737,170.482234831862));
#30520=CARTESIAN_POINT('Ctrl Pts',(32.8343216385758,33.445245211389,170.445191568789));
#30521=CARTESIAN_POINT('Ctrl Pts',(33.3118909809782,33.1695505174043,170.408148305716));
#30522=CARTESIAN_POINT('Ctrl Pts',(33.6392950293065,32.6337335130981,170.371105042643));
#30523=CARTESIAN_POINT('Ctrl Pts',(33.6667154663201,32.0829811542943,170.334061779569));
#30524=CARTESIAN_POINT('Ctrl Pts',(33.6941359033337,31.5322287954904,170.297018516496));
#30525=CARTESIAN_POINT('Ctrl Pts',(33.4215727290326,30.9665410821889,170.259975253423));
#30526=CARTESIAN_POINT('Ctrl Pts',(32.9737493740648,30.6447736446826,170.22293199035));
#30527=CARTESIAN_POINT('Ctrl Pts',(32.525926019097,30.3230062071763,170.185888727276));
#30528=CARTESIAN_POINT('Ctrl Pts',(31.9028424834624,30.2451590454651,170.148845464203));
#30529=CARTESIAN_POINT('Ctrl Pts',(31.3896184145377,30.4468545986395,170.11180220113));
#30530=CARTESIAN_POINT('Ctrl Pts',(30.8763943456129,30.648550151814,170.074758938057));
#30531=CARTESIAN_POINT('Ctrl Pts',(30.473029743398,31.129788419874,170.037715674983));
#30532=CARTESIAN_POINT('Ctrl Pts',(30.364102062713,31.6703573807611,170.00067241191));
#30533=CARTESIAN_POINT('Ctrl Pts',(30.3423882589603,31.7781151908759,169.993288153477));
#30534=CARTESIAN_POINT('Ctrl Pts',(30.3323745012792,31.888230625965,169.985903895043));
#30535=CARTESIAN_POINT('Ctrl Pts',(30.3333883716037,31.9985292209557,169.97851963661));
#30536=CARTESIAN_POINT('Ctrl Pts',(30.3365390106164,31.9994923848488,170.17148036339));
#30537=CARTESIAN_POINT('Ctrl Pts',(30.3358656897121,31.753017211109,170.187902459474));
#30538=CARTESIAN_POINT('Ctrl Pts',(30.3871295825161,31.5068083838415,170.204324555558));
#30539=CARTESIAN_POINT('Ctrl Pts',(30.491745321287,31.2858609639402,170.220746651642));
#30540=CARTESIAN_POINT('Ctrl Pts',(30.7277266669766,30.7874706635177,170.257789914715));
#30541=CARTESIAN_POINT('Ctrl Pts',(31.2351710754656,30.4176146038501,170.294833177788));
#30542=CARTESIAN_POINT('Ctrl Pts',(31.7818747369324,30.3455369123804,170.331876440861));
#30543=CARTESIAN_POINT('Ctrl Pts',(32.3285783983991,30.2734592209107,170.368919703935));
#30544=CARTESIAN_POINT('Ctrl Pts',(32.9145413128434,30.4991598976388,170.405962967008));
#30545=CARTESIAN_POINT('Ctrl Pts',(33.2716300278673,30.919359536705,170.443006230081));
#30546=CARTESIAN_POINT('Ctrl Pts',(33.6287187428911,31.3395591757712,170.480049493154));
#30547=CARTESIAN_POINT('Ctrl Pts',(33.7569332584945,31.9542577771753,170.517092756228));
#30548=CARTESIAN_POINT('Ctrl Pts',(33.5976033075515,32.4821725939794,170.554136019301));
#30549=CARTESIAN_POINT('Ctrl Pts',(33.4382733566085,33.0100874107834,170.591179282374));
#30550=CARTESIAN_POINT('Ctrl Pts',(32.9913989391192,33.4512184429872,170.628222545447));
#30551=CARTESIAN_POINT('Ctrl Pts',(32.461467365451,33.6037065221879,170.665265808521));
#30552=CARTESIAN_POINT('Ctrl Pts',(31.9315357917828,33.7561946013885,170.702309071594));
#30553=CARTESIAN_POINT('Ctrl Pts',(31.3185470619358,33.6200397275859,170.739352334667));
#30554=CARTESIAN_POINT('Ctrl Pts',(30.9030014948949,33.2575456327631,170.77639559774));
#30555=CARTESIAN_POINT('Ctrl Pts',(30.5474527879603,32.9473887765523,170.808090519624));
#30556=CARTESIAN_POINT('Ctrl Pts',(30.3364490562282,32.471532604018,170.839785441507));
#30557=CARTESIAN_POINT('Ctrl Pts',(30.3325050746568,31.9987546321113,170.87148036339));
#30558=CARTESIAN_POINT('Origin',(32.,32.,172.));
#30559=CARTESIAN_POINT('',(30.3326609038217,32.0013000933536,171.57148036339));
#30560=CARTESIAN_POINT('',(30.3362278621005,32.0008713646937,171.37851963661));
#30561=CARTESIAN_POINT('',(30.334,32.,172.));
#30562=CARTESIAN_POINT('Ctrl Pts',(30.3362278621005,32.0008713646937,171.37851963661));
#30563=CARTESIAN_POINT('Ctrl Pts',(30.3351774463097,32.2223456968917,171.363756385255));
#30564=CARTESIAN_POINT('Ctrl Pts',(30.3762757543327,32.4434460199116,171.348993133901));
#30565=CARTESIAN_POINT('Ctrl Pts',(30.4613604710716,32.6460764023376,171.334229882547));
#30566=CARTESIAN_POINT('Ctrl Pts',(30.6748510816438,33.1545071255354,171.297186619474));
#30567=CARTESIAN_POINT('Ctrl Pts',(31.165273569148,33.5466538540894,171.2601433564));
#30568=CARTESIAN_POINT('Ctrl Pts',(31.7082132625074,33.6430723713403,171.223100093327));
#30569=CARTESIAN_POINT('Ctrl Pts',(32.2511529558667,33.7394908885913,171.186056830254));
#30570=CARTESIAN_POINT('Ctrl Pts',(32.8466098550813,33.5401811945391,171.149013567181));
#30571=CARTESIAN_POINT('Ctrl Pts',(33.222106111801,33.1363463244703,171.111970304107));
#30572=CARTESIAN_POINT('Ctrl Pts',(33.5976023685207,32.7325114544016,171.074927041034));
#30573=CARTESIAN_POINT('Ctrl Pts',(33.7531379827457,32.1241514083162,171.037883777961));
#30574=CARTESIAN_POINT('Ctrl Pts',(33.6175407007633,31.5896484446078,171.000840514888));
#30575=CARTESIAN_POINT('Ctrl Pts',(33.4819434187809,31.0551454808995,170.963797251814));
#30576=CARTESIAN_POINT('Ctrl Pts',(33.0552132405911,30.5944995995682,170.926753988741));
#30577=CARTESIAN_POINT('Ctrl Pts',(32.5326195818855,30.4184998581629,170.889710725668));
#30578=CARTESIAN_POINT('Ctrl Pts',(32.0100259231799,30.2425001167576,170.852667462595));
#30579=CARTESIAN_POINT('Ctrl Pts',(31.3915687839586,30.3511465152783,170.815624199521));
#30580=CARTESIAN_POINT('Ctrl Pts',(30.9602507976849,30.6947230508724,170.778580936448));
#30581=CARTESIAN_POINT('Ctrl Pts',(30.5718919368139,31.0040794798452,170.745227169835));
#30582=CARTESIAN_POINT('Ctrl Pts',(30.3352506740603,31.5038986503701,170.711873403223));
#30583=CARTESIAN_POINT('Ctrl Pts',(30.3318905055228,32.0009409351765,170.67851963661));
#30584=CARTESIAN_POINT('Ctrl Pts',(30.3325050746568,31.9987546321113,170.87148036339));
#30585=CARTESIAN_POINT('Ctrl Pts',(30.3318395497766,31.9189759877552,170.87682870458));
#30586=CARTESIAN_POINT('Ctrl Pts',(30.3370699848296,31.8392849941742,170.88217704577));
#30587=CARTESIAN_POINT('Ctrl Pts',(30.3484967597576,31.760492617748,170.88752538696));
#30588=CARTESIAN_POINT('Ctrl Pts',(30.4276399958959,31.2147670133988,170.924568650033));
#30589=CARTESIAN_POINT('Ctrl Pts',(30.804028872407,30.7121491205435,170.961611913106));
#30590=CARTESIAN_POINT('Ctrl Pts',(31.3054298802833,30.4826341616206,170.99865517618));
#30591=CARTESIAN_POINT('Ctrl Pts',(31.8068308881596,30.2531192026977,171.035698439253));
#30592=CARTESIAN_POINT('Ctrl Pts',(32.4332440274009,30.2967071777072,171.072741702326));
#30593=CARTESIAN_POINT('Ctrl Pts',(32.8980260420744,30.5934524656307,171.109784965399));
#30594=CARTESIAN_POINT('Ctrl Pts',(33.3628080567478,30.8901977535542,171.146828228473));
#30595=CARTESIAN_POINT('Ctrl Pts',(33.6659589468533,31.4401003543917,171.183871491546));
#30596=CARTESIAN_POINT('Ctrl Pts',(33.6687585088459,31.9915278197227,171.220914754619));
#30597=CARTESIAN_POINT('Ctrl Pts',(33.6715580708384,32.5429552850537,171.257958017692));
#30598=CARTESIAN_POINT('Ctrl Pts',(33.374006304718,33.0959076148782,171.295001280766));
#30599=CARTESIAN_POINT('Ctrl Pts',(32.9122612852541,33.3973568213276,171.332044543839));
#30600=CARTESIAN_POINT('Ctrl Pts',(32.4505162657902,33.698806027777,171.369087806912));
#30601=CARTESIAN_POINT('Ctrl Pts',(31.8245779929827,33.7487521108513,171.406131069985));
#30602=CARTESIAN_POINT('Ctrl Pts',(31.3208724264595,33.5243400137571,171.443174333059));
#30603=CARTESIAN_POINT('Ctrl Pts',(30.8171668599362,33.299927916663,171.480217596132));
#30604=CARTESIAN_POINT('Ctrl Pts',(30.4356939996972,32.8011576394003,171.517260859205));
#30605=CARTESIAN_POINT('Ctrl Pts',(30.3510137581373,32.2562637563753,171.554304122278));
#30606=CARTESIAN_POINT('Ctrl Pts',(30.3379255640836,32.1720448553858,171.560029535982));
#30607=CARTESIAN_POINT('Ctrl Pts',(30.3319274048857,32.0867241144181,171.565754949686));
#30608=CARTESIAN_POINT('Ctrl Pts',(30.3326609038217,32.0013000933536,171.57148036339));
#30609=CARTESIAN_POINT('Origin',(32.,32.,172.));
#30610=CARTESIAN_POINT('',(30.3365860283557,32.0004190115501,172.27148036339));
#30611=CARTESIAN_POINT('',(30.3350677280756,31.9985848365712,172.07851963661));
#30612=CARTESIAN_POINT('',(30.334,32.,172.));
#30613=CARTESIAN_POINT('Ctrl Pts',(30.3350677280756,31.9985848365712,172.07851963661));
#30614=CARTESIAN_POINT('Ctrl Pts',(30.3381924982781,32.3855055066604,172.052682630362));
#30615=CARTESIAN_POINT('Ctrl Pts',(30.4725557093059,32.7743832562982,172.026845624113));
#30616=CARTESIAN_POINT('Ctrl Pts',(30.7190756776316,33.0696070297093,172.001008617865));
#30617=CARTESIAN_POINT('Ctrl Pts',(31.072518485663,33.4928778916226,171.963965354792));
#30618=CARTESIAN_POINT('Ctrl Pts',(31.6565083257521,33.723635642604,171.926922091719));
#30619=CARTESIAN_POINT('Ctrl Pts',(32.2038146136273,33.6562867870361,171.889878828646));
#30620=CARTESIAN_POINT('Ctrl Pts',(32.7511209015025,33.5889379314683,171.852835565572));
#30621=CARTESIAN_POINT('Ctrl Pts',(33.2617436371637,33.2234824693511,171.815792302499));
#30622=CARTESIAN_POINT('Ctrl Pts',(33.5020246255088,32.7271508385498,171.778749039426));
#30623=CARTESIAN_POINT('Ctrl Pts',(33.7423056138539,32.2308192077485,171.741705776353));
#30624=CARTESIAN_POINT('Ctrl Pts',(33.712244854883,31.6036114082629,171.704662513279));
#30625=CARTESIAN_POINT('Ctrl Pts',(33.4255979889034,31.1325343282452,171.667619250206));
#30626=CARTESIAN_POINT('Ctrl Pts',(33.1389511229238,30.6614572482273,171.630575987133));
#30627=CARTESIAN_POINT('Ctrl Pts',(32.5957181499356,30.3465108876772,171.59353272406));
#30628=CARTESIAN_POINT('Ctrl Pts',(32.04447953282,30.3318129934571,171.556489460986));
#30629=CARTESIAN_POINT('Ctrl Pts',(31.4932409157044,30.3171150992369,171.519446197913));
#30630=CARTESIAN_POINT('Ctrl Pts',(30.9339966544615,30.6026656713466,171.48240293484));
#30631=CARTESIAN_POINT('Ctrl Pts',(30.6226538906602,31.0577983163223,171.445359671767));
#30632=CARTESIAN_POINT('Ctrl Pts',(30.4353939181147,31.3315420371081,171.423079660048));
#30633=CARTESIAN_POINT('Ctrl Pts',(30.3378131007155,31.6666326121062,171.400799648329));
#30634=CARTESIAN_POINT('Ctrl Pts',(30.3362278621005,32.0008713646937,171.37851963661));
#30635=CARTESIAN_POINT('Ctrl Pts',(30.3326609038217,32.0013000933536,171.57148036339));
#30636=CARTESIAN_POINT('Ctrl Pts',(30.3366731220436,31.5340331389412,171.60279821276));
#30637=CARTESIAN_POINT('Ctrl Pts',(30.5421005058999,31.0636759833655,171.634116062129));
#30638=CARTESIAN_POINT('Ctrl Pts',(30.8902894158567,30.7536576882235,171.665433911498));
#30639=CARTESIAN_POINT('Ctrl Pts',(31.3021329380168,30.386962991884,171.702477174571));
#30640=CARTESIAN_POINT('Ctrl Pts',(31.9137076052177,30.2445910879924,171.739520437645));
#30641=CARTESIAN_POINT('Ctrl Pts',(32.4451601658739,30.39169058779,171.776563700718));
#30642=CARTESIAN_POINT('Ctrl Pts',(32.9766127265301,30.5387900875876,171.813606963791));
#30643=CARTESIAN_POINT('Ctrl Pts',(33.4279431806416,30.9753609910743,171.850650226864));
#30644=CARTESIAN_POINT('Ctrl Pts',(33.5926251596443,31.5016308200218,171.887693489938));
#30645=CARTESIAN_POINT('Ctrl Pts',(33.7573071386471,32.0279006489693,171.924736753011));
#30646=CARTESIAN_POINT('Ctrl Pts',(33.6353406425412,32.6438694033776,171.961780016084));
#30647=CARTESIAN_POINT('Ctrl Pts',(33.2825368786089,33.067673121181,171.998823279157));
#30648=CARTESIAN_POINT('Ctrl Pts',(32.9297331146766,33.4914768389843,172.035866542231));
#30649=CARTESIAN_POINT('Ctrl Pts',(32.3460920829179,33.7231155201827,172.072909805304));
#30650=CARTESIAN_POINT('Ctrl Pts',(31.7986847548039,33.6565925602682,172.109953068377));
#30651=CARTESIAN_POINT('Ctrl Pts',(31.2512774266899,33.5900696003537,172.14699633145));
#30652=CARTESIAN_POINT('Ctrl Pts',(30.7401038022206,33.2253849993263,172.184039594523));
#30653=CARTESIAN_POINT('Ctrl Pts',(30.4990741602295,32.7294164531962,172.221082857597));
#30654=CARTESIAN_POINT('Ctrl Pts',(30.3897669000973,32.5044940642262,172.237882026195));
#30655=CARTESIAN_POINT('Ctrl Pts',(30.3360183819722,32.2525713668698,172.254681194792));
#30656=CARTESIAN_POINT('Ctrl Pts',(30.3365860283557,32.0004190115501,172.27148036339));
#30657=CARTESIAN_POINT('Origin',(32.,32.,172.));
#30658=CARTESIAN_POINT('',(30.3341968101826,31.9984781516629,172.97148036339));
#30659=CARTESIAN_POINT('',(30.3312207490626,31.9999631491892,172.77851963661));
#30660=CARTESIAN_POINT('',(30.334,32.,172.));
#30661=CARTESIAN_POINT('Ctrl Pts',(30.3312211427064,31.9999631544086,172.77851963661));
#30662=CARTESIAN_POINT('Ctrl Pts',(30.331399935389,32.5494261488841,172.741608875468));
#30663=CARTESIAN_POINT('Ctrl Pts',(30.6293022294751,33.0990552818063,172.704698114326));
#30664=CARTESIAN_POINT('Ctrl Pts',(31.0898482772994,33.398731625189,172.667787353184));
#30665=CARTESIAN_POINT('Ctrl Pts',(31.5520475893435,33.6994837441175,172.63074409011));
#30666=CARTESIAN_POINT('Ctrl Pts',(32.1780604653325,33.7484852957398,172.593700827037));
#30667=CARTESIAN_POINT('Ctrl Pts',(32.6814268076273,33.5233134357333,172.556657563964));
#30668=CARTESIAN_POINT('Ctrl Pts',(33.184793149922,33.2981415757268,172.519614300891));
#30669=CARTESIAN_POINT('Ctrl Pts',(33.5655129585226,32.7987963040915,172.482571037817));
#30670=CARTESIAN_POINT('Ctrl Pts',(33.6493709133806,32.2537753095408,172.445527774744));
#30671=CARTESIAN_POINT('Ctrl Pts',(33.7332288682386,31.7087543149901,172.408484511671));
#30672=CARTESIAN_POINT('Ctrl Pts',(33.520224969354,31.1180575975239,172.371441248598));
#30673=CARTESIAN_POINT('Ctrl Pts',(33.1078286458908,30.7519847721352,172.334397985524));
#30674=CARTESIAN_POINT('Ctrl Pts',(32.6954323224276,30.3859119467466,172.297354722451));
#30675=CARTESIAN_POINT('Ctrl Pts',(32.0836435743859,30.2444630134353,172.260311459378));
#30676=CARTESIAN_POINT('Ctrl Pts',(31.5524136155831,30.3923642371099,172.223268196305));
#30677=CARTESIAN_POINT('Ctrl Pts',(31.0211836567803,30.5402654607845,172.186224933231));
#30678=CARTESIAN_POINT('Ctrl Pts',(30.5705124872166,30.9775168414449,172.149181670158));
#30679=CARTESIAN_POINT('Ctrl Pts',(30.4066247904215,31.5040345181977,172.112138407085));
#30680=CARTESIAN_POINT('Ctrl Pts',(30.3570457990374,31.6633156349002,172.10093215026));
#30681=CARTESIAN_POINT('Ctrl Pts',(30.3337124248693,31.8307661520737,172.089725893435));
#30682=CARTESIAN_POINT('Ctrl Pts',(30.3350677280756,31.9985848365712,172.07851963661));
#30683=CARTESIAN_POINT('Ctrl Pts',(30.3365860283557,32.0004190115501,172.27148036339));
#30684=CARTESIAN_POINT('Ctrl Pts',(30.3372700792925,31.6965589679093,172.291724457866));
#30685=CARTESIAN_POINT('Ctrl Pts',(30.4168311019023,31.3923654190436,172.311968552341));
#30686=CARTESIAN_POINT('Ctrl Pts',(30.5730946173501,31.1346863183511,172.332212646816));
#30687=CARTESIAN_POINT('Ctrl Pts',(30.8590303759745,30.6631772208688,172.36925590989));
#30688=CARTESIAN_POINT('Ctrl Pts',(31.4017875527363,30.347411517137,172.406299172963));
#30689=CARTESIAN_POINT('Ctrl Pts',(31.9530034065273,30.331881881015,172.443342436036));
#30690=CARTESIAN_POINT('Ctrl Pts',(32.5042192603184,30.316352244893,172.480385699109));
#30691=CARTESIAN_POINT('Ctrl Pts',(33.0638937911388,30.6010586763809,172.517428962183));
#30692=CARTESIAN_POINT('Ctrl Pts',(33.375922968394,31.0557210561862,172.554472225256));
#30693=CARTESIAN_POINT('Ctrl Pts',(33.6879521456491,31.5103834359915,172.591515488329));
#30694=CARTESIAN_POINT('Ctrl Pts',(33.7523359693389,32.1350017641142,172.628558751402));
#30695=CARTESIAN_POINT('Ctrl Pts',(33.5396127508497,32.6437540804571,172.665602014476));
#30696=CARTESIAN_POINT('Ctrl Pts',(33.3268895323605,33.1525063968,172.702645277549));
#30697=CARTESIAN_POINT('Ctrl Pts',(32.8370592716923,33.5453927013633,172.739688540622));
#30698=CARTESIAN_POINT('Ctrl Pts',(32.2942656401328,33.6426303515159,172.776731803695));
#30699=CARTESIAN_POINT('Ctrl Pts',(31.7514720085734,33.7398680016686,172.813775066769));
#30700=CARTESIAN_POINT('Ctrl Pts',(31.1557150061227,33.5414569974107,172.850818329842));
#30701=CARTESIAN_POINT('Ctrl Pts',(30.7796098067444,33.1381891384518,172.887861592915));
#30702=CARTESIAN_POINT('Ctrl Pts',(30.4966122903972,32.8347532840774,172.915734516407));
#30703=CARTESIAN_POINT('Ctrl Pts',(30.3379749552747,32.4153336990011,172.943607439898));
#30704=CARTESIAN_POINT('Ctrl Pts',(30.3341968101826,31.9984781516629,172.97148036339));
#30705=CARTESIAN_POINT('Origin',(32.,32.,172.));
#30706=CARTESIAN_POINT('',(30.331415601616,32.0005168033969,173.67148036339));
#30707=CARTESIAN_POINT('',(30.3349603589764,32.0014384974263,173.47851963661));
#30708=CARTESIAN_POINT('',(30.334,32.,172.));
#30709=CARTESIAN_POINT('Ctrl Pts',(30.3349603589764,32.0014384974263,173.47851963661));
#30710=CARTESIAN_POINT('Ctrl Pts',(30.3336089417427,32.1652618982138,173.467578383647));
#30711=CARTESIAN_POINT('Ctrl Pts',(30.355830596873,32.3287266852567,173.456637130684));
#30712=CARTESIAN_POINT('Ctrl Pts',(30.4031261763844,32.4845826132764,173.445695877722));
#30713=CARTESIAN_POINT('Ctrl Pts',(30.5632524982974,33.0122563781393,173.408652614648));
#30714=CARTESIAN_POINT('Ctrl Pts',(31.0107919906657,33.4527125913275,173.371609351575));
#30715=CARTESIAN_POINT('Ctrl Pts',(31.5409530084635,33.6044008779603,173.334566088502));
#30716=CARTESIAN_POINT('Ctrl Pts',(32.0711140262613,33.7560891645932,173.297522825429));
#30717=CARTESIAN_POINT('Ctrl Pts',(32.6838965694886,33.6190095246707,173.260479562355));
#30718=CARTESIAN_POINT('Ctrl Pts',(33.0988946690395,33.255888858138,173.223436299282));
#30719=CARTESIAN_POINT('Ctrl Pts',(33.5138927685904,32.8927681916053,173.186393036209));
#30720=CARTESIAN_POINT('Ctrl Pts',(33.731106424465,32.3036064984624,173.149349773136));
#30721=CARTESIAN_POINT('Ctrl Pts',(33.651139845527,31.7580009748953,173.112306510062));
#30722=CARTESIAN_POINT('Ctrl Pts',(33.571173266589,31.2123954513282,173.075263246989));
#30723=CARTESIAN_POINT('Ctrl Pts',(33.1940264528385,30.7103460973368,173.038219983916));
#30724=CARTESIAN_POINT('Ctrl Pts',(32.6922797412542,30.4815879750583,173.001176720843));
#30725=CARTESIAN_POINT('Ctrl Pts',(32.1905330296699,30.2528298527798,172.96413345777));
#30726=CARTESIAN_POINT('Ctrl Pts',(31.5641864202519,30.2973629622143,172.927090194696));
#30727=CARTESIAN_POINT('Ctrl Pts',(31.0998527252467,30.5948091939552,172.890046931623));
#30728=CARTESIAN_POINT('Ctrl Pts',(30.6355190302416,30.8922554256961,172.85300366855));
#30729=CARTESIAN_POINT('Ctrl Pts',(30.3331982496493,31.4426147797435,172.815960405477));
#30730=CARTESIAN_POINT('Ctrl Pts',(30.3312307334027,31.9940457998846,172.778917142403));
#30731=CARTESIAN_POINT('Ctrl Pts',(30.3312236956938,31.9960182415379,172.778784640472));
#30732=CARTESIAN_POINT('Ctrl Pts',(30.331220500878,31.9979906969028,172.778652138541));
#30733=CARTESIAN_POINT('Ctrl Pts',(30.3312211427064,31.9999631544086,172.77851963661));
#30734=CARTESIAN_POINT('Ctrl Pts',(30.3341968101826,31.9984781516629,172.97148036339));
#30735=CARTESIAN_POINT('Ctrl Pts',(30.3329537804196,31.8613304668622,172.980650702972));
#30736=CARTESIAN_POINT('Ctrl Pts',(30.3484734044008,31.7244603250137,172.989821042553));
#30737=CARTESIAN_POINT('Ctrl Pts',(30.3818418436429,31.5920895690238,172.998991382135));
#30738=CARTESIAN_POINT('Ctrl Pts',(30.5166324762257,31.0573825722146,173.036034645208));
#30739=CARTESIAN_POINT('Ctrl Pts',(30.9426671376973,30.5960932922563,173.073077908281));
#30740=CARTESIAN_POINT('Ctrl Pts',(31.464994677045,30.4193052024208,173.110121171354));
#30741=CARTESIAN_POINT('Ctrl Pts',(31.9873222163927,30.2425171125853,173.147164434428));
#30742=CARTESIAN_POINT('Ctrl Pts',(32.6059426336165,30.3502302128725,173.184207697501));
#30743=CARTESIAN_POINT('Ctrl Pts',(33.0377785801244,30.693155572641,173.221250960574));
#30744=CARTESIAN_POINT('Ctrl Pts',(33.4696145266322,31.0360809324095,173.258294223647));
#30745=CARTESIAN_POINT('Ctrl Pts',(33.7146660024241,31.6142185516594,173.295337486721));
#30746=CARTESIAN_POINT('Ctrl Pts',(33.660798780914,32.1630157906425,173.332380749794));
#30747=CARTESIAN_POINT('Ctrl Pts',(33.6069315594039,32.7118130296256,173.369424012867));
#30748=CARTESIAN_POINT('Ctrl Pts',(33.2541456405917,33.231269888342,173.40646727594));
#30749=CARTESIAN_POINT('Ctrl Pts',(32.7638739480239,33.4836857248806,173.443510539014));
#30750=CARTESIAN_POINT('Ctrl Pts',(32.2736022554562,33.7361015614192,173.480553802087));
#30751=CARTESIAN_POINT('Ctrl Pts',(31.6458447891329,33.72147637578,173.51759706516));
#30752=CARTESIAN_POINT('Ctrl Pts',(31.1678599617704,33.4465025736097,173.554640328233));
#30753=CARTESIAN_POINT('Ctrl Pts',(30.6898751344079,33.1715287714394,173.591683591307));
#30754=CARTESIAN_POINT('Ctrl Pts',(30.3616629460063,32.636206352738,173.62872685438));
#30755=CARTESIAN_POINT('Ctrl Pts',(30.3334115143217,32.0854959536384,173.665770117453));
#30756=CARTESIAN_POINT('Ctrl Pts',(30.331959854743,32.0571984841561,173.667673532766));
#30757=CARTESIAN_POINT('Ctrl Pts',(30.331300173107,32.0288603862224,173.669576948078));
#30758=CARTESIAN_POINT('Ctrl Pts',(30.331415601616,32.0005168033969,173.67148036339));
#30759=CARTESIAN_POINT('Origin',(32.,32.,172.));
#30760=CARTESIAN_POINT('',(30.3357185782339,32.0011936552705,174.37148036339));
#30761=CARTESIAN_POINT('',(30.336288627554,31.999183265941,174.17851963661));
#30762=CARTESIAN_POINT('',(30.334,32.,172.));
#30763=CARTESIAN_POINT('Ctrl Pts',(30.336288627554,31.999183265941,174.17851963661));
#30764=CARTESIAN_POINT('Ctrl Pts',(30.3377536367914,32.3294766934183,174.156504628753));
#30765=CARTESIAN_POINT('Ctrl Pts',(30.4328676987764,32.6605477827672,174.134489620897));
#30766=CARTESIAN_POINT('Ctrl Pts',(30.6159654584887,32.9323490256026,174.11247461304));
#30767=CARTESIAN_POINT('Ctrl Pts',(30.9240524928118,33.389691807743,174.075431349967));
#30768=CARTESIAN_POINT('Ctrl Pts',(31.4812448413513,33.679225846665,174.038388086894));
#30769=CARTESIAN_POINT('Ctrl Pts',(32.032574306665,33.6684619360908,174.00134482382));
#30770=CARTESIAN_POINT('Ctrl Pts',(32.5839037719788,33.6576980255166,173.964301560747));
#30771=CARTESIAN_POINT('Ctrl Pts',(33.1293703540669,33.3466361654461,173.927258297674));
#30772=CARTESIAN_POINT('Ctrl Pts',(33.4193715026352,32.877616576385,173.890215034601));
#30773=CARTESIAN_POINT('Ctrl Pts',(33.7093726512035,32.4085969873239,173.853171771527));
#30774=CARTESIAN_POINT('Ctrl Pts',(33.743908366252,31.781619669272,173.816128508454));
#30775=CARTESIAN_POINT('Ctrl Pts',(33.5071752918366,31.2835860433271,173.779085245381));
#30776=CARTESIAN_POINT('Ctrl Pts',(33.2704422174213,30.7855524173822,173.742041982308));
#30777=CARTESIAN_POINT('Ctrl Pts',(32.762440353542,30.4164624835441,173.704998719234));
#30778=CARTESIAN_POINT('Ctrl Pts',(32.2156285985846,30.3452097942304,173.667955456161));
#30779=CARTESIAN_POINT('Ctrl Pts',(31.6688168436272,30.2739571049167,173.630912193088));
#30780=CARTESIAN_POINT('Ctrl Pts',(31.0831951975917,30.5005416601273,173.593868930015));
#30781=CARTESIAN_POINT('Ctrl Pts',(30.7267409503027,30.9212795960015,173.556825666941));
#30782=CARTESIAN_POINT('Ctrl Pts',(30.4755705189,31.2177466171263,173.530723656831));
#30783=CARTESIAN_POINT('Ctrl Pts',(30.3381843687327,31.6106130519071,173.50462164672));
#30784=CARTESIAN_POINT('Ctrl Pts',(30.3349603589764,32.0014384974263,173.47851963661));
#30785=CARTESIAN_POINT('Ctrl Pts',(30.331415601616,32.0005168033969,173.67148036339));
#30786=CARTESIAN_POINT('Ctrl Pts',(30.3335465817587,31.477252553602,173.706620211151));
#30787=CARTESIAN_POINT('Ctrl Pts',(30.5998552011771,30.9521189104532,173.741760058912));
#30788=CARTESIAN_POINT('Ctrl Pts',(31.0242067755662,30.6462443640623,173.776899906673));
#30789=CARTESIAN_POINT('Ctrl Pts',(31.4715441434631,30.3238015530837,173.813943169746));
#30790=CARTESIAN_POINT('Ctrl Pts',(32.0945095542247,30.2450143106244,173.850986432819));
#30791=CARTESIAN_POINT('Ctrl Pts',(32.6080374137757,30.4459352516278,173.888029695893));
#30792=CARTESIAN_POINT('Ctrl Pts',(33.1215652733267,30.6468561926312,173.925072958966));
#30793=CARTESIAN_POINT('Ctrl Pts',(33.5256555816671,31.1274853170972,173.962116222039));
#30794=CARTESIAN_POINT('Ctrl Pts',(33.6353988047888,31.6678893437732,173.999159485112));
#30795=CARTESIAN_POINT('Ctrl Pts',(33.7451420279106,32.2082933704491,174.036202748185));
#30796=CARTESIAN_POINT('Ctrl Pts',(33.5605381658136,32.808472299335,174.073246011259));
#30797=CARTESIAN_POINT('Ctrl Pts',(33.1660609448208,33.1937875069073,174.110289274332));
#30798=CARTESIAN_POINT('Ctrl Pts',(32.771583723828,33.5791027144796,174.147332537405));
#30799=CARTESIAN_POINT('Ctrl Pts',(32.1672331439392,33.7495542007383,174.184375800478));
#30800=CARTESIAN_POINT('Ctrl Pts',(31.6295567535571,33.6271442898062,174.221419063552));
#30801=CARTESIAN_POINT('Ctrl Pts',(31.0918803631751,33.5047343788742,174.258462326625));
#30802=CARTESIAN_POINT('Ctrl Pts',(30.6208781622996,33.0894630707512,174.295505589698));
#30803=CARTESIAN_POINT('Ctrl Pts',(30.4320782041483,32.5713562643196,174.332548852772));
#30804=CARTESIAN_POINT('Ctrl Pts',(30.3659369145156,32.3898506502273,174.345526022978));
#30805=CARTESIAN_POINT('Ctrl Pts',(30.3344295720944,32.1957243029137,174.358503193184));
#30806=CARTESIAN_POINT('Ctrl Pts',(30.3357185782339,32.0011936552705,174.37148036339));
#30807=CARTESIAN_POINT('Origin',(32.,32.,172.));
#30808=CARTESIAN_POINT('',(30.3357235801798,31.9988086992918,175.07148036339));
#30809=CARTESIAN_POINT('',(30.3319793737621,31.999003930908,174.87851963661));
#30810=CARTESIAN_POINT('',(30.334,32.,172.));
#30811=CARTESIAN_POINT('Ctrl Pts',(30.3319793737621,31.999003930908,174.87851963661));
#30812=CARTESIAN_POINT('Ctrl Pts',(30.3354661445113,32.4921662044565,174.845430873859));
#30813=CARTESIAN_POINT('Ctrl Pts',(30.5678894507187,32.988184128635,174.812342111109));
#30814=CARTESIAN_POINT('Ctrl Pts',(30.950962884132,33.2978241202759,174.779253348358));
#30815=CARTESIAN_POINT('Ctrl Pts',(31.3798181446719,33.6444697701856,174.742210085285));
#30816=CARTESIAN_POINT('Ctrl Pts',(31.9974842423223,33.7575266796541,174.705166822212));
#30817=CARTESIAN_POINT('Ctrl Pts',(32.5213205199536,33.5852606199341,174.668123559139));
#30818=CARTESIAN_POINT('Ctrl Pts',(33.0451567975848,33.4129945602141,174.631080296065));
#30819=CARTESIAN_POINT('Ctrl Pts',(33.4751632551969,32.9554055313057,174.594037032992));
#30820=CARTESIAN_POINT('Ctrl Pts',(33.6145712693993,32.4218837916642,174.556993769919));
#30821=CARTESIAN_POINT('Ctrl Pts',(33.7539792836017,31.8883620520226,174.519950506846));
#30822=CARTESIAN_POINT('Ctrl Pts',(33.6027888543946,31.2789076016479,174.482907243772));
#30823=CARTESIAN_POINT('Ctrl Pts',(33.230183902387,30.8724034924024,174.445863980699));
#30824=CARTESIAN_POINT('Ctrl Pts',(32.8575789503795,30.4658993831569,174.408820717626));
#30825=CARTESIAN_POINT('Ctrl Pts',(32.2635594755717,30.2623456150405,174.371777454553));
#30826=CARTESIAN_POINT('Ctrl Pts',(31.7199455686991,30.354887288619,174.33473419148));
#30827=CARTESIAN_POINT('Ctrl Pts',(31.1763316618265,30.4474289621975,174.297690928406));
#30828=CARTESIAN_POINT('Ctrl Pts',(30.6831233228891,30.8360660774709,174.260647665333));
#30829=CARTESIAN_POINT('Ctrl Pts',(30.4660100134739,31.3429603977871,174.22360440226));
#30830=CARTESIAN_POINT('Ctrl Pts',(30.3779282962027,31.5486047331285,174.208576147043));
#30831=CARTESIAN_POINT('Ctrl Pts',(30.3352885582895,31.7737128070232,174.193547891827));
#30832=CARTESIAN_POINT('Ctrl Pts',(30.336288627554,31.999183265941,174.17851963661));
#30833=CARTESIAN_POINT('Ctrl Pts',(30.3357185782339,32.0011936552705,174.37148036339));
#30834=CARTESIAN_POINT('Ctrl Pts',(30.338109033238,31.640437607747,174.395546456257));
#30835=CARTESIAN_POINT('Ctrl Pts',(30.4532910651195,31.2782911105634,174.419612549124));
#30836=CARTESIAN_POINT('Ctrl Pts',(30.6695446788991,30.9926691818284,174.443678641991));
#30837=CARTESIAN_POINT('Ctrl Pts',(31.0024088272283,30.5530312105091,174.480721905065));
#30838=CARTESIAN_POINT('Ctrl Pts',(31.574734839314,30.2946975726108,174.517765168138));
#30839=CARTESIAN_POINT('Ctrl Pts',(32.1246294353343,30.3358803400799,174.554808431211));
#30840=CARTESIAN_POINT('Ctrl Pts',(32.6745240313545,30.3770631075491,174.591851694284));
#30841=CARTESIAN_POINT('Ctrl Pts',(33.2019872113094,30.7177622803858,174.628894957357));
#30842=CARTESIAN_POINT('Ctrl Pts',(33.4656546841015,31.2020757644642,174.665938220431));
#30843=CARTESIAN_POINT('Ctrl Pts',(33.7293221568936,31.6863892485425,174.702981483504));
#30844=CARTESIAN_POINT('Ctrl Pts',(33.729193922523,32.3143170438626,174.740024746577));
#30845=CARTESIAN_POINT('Ctrl Pts',(33.4653286603423,32.7985227960827,174.77706800965));
#30846=CARTESIAN_POINT('Ctrl Pts',(33.2014633981616,33.2827285483028,174.814111272724));
#30847=CARTESIAN_POINT('Ctrl Pts',(32.6738611081708,33.6232122574229,174.851154535797));
#30848=CARTESIAN_POINT('Ctrl Pts',(32.1239497374654,33.6641704243456,174.88819779887));
#30849=CARTESIAN_POINT('Ctrl Pts',(31.57403836676,33.7051285912683,174.925241061943));
#30850=CARTESIAN_POINT('Ctrl Pts',(31.0018179153401,33.4465612159936,174.962284325017));
#30851=CARTESIAN_POINT('Ctrl Pts',(30.6691333590391,33.0067873274241,174.99932758809));
#30852=CARTESIAN_POINT('Ctrl Pts',(30.4531326430722,32.7212571668096,175.02337851319));
#30853=CARTESIAN_POINT('Ctrl Pts',(30.3381073551171,32.3593401029738,175.04742943829));
#30854=CARTESIAN_POINT('Ctrl Pts',(30.3357235801798,31.9988086992918,175.07148036339));
#30855=CARTESIAN_POINT('Origin',(32.,32.,172.));
#30856=CARTESIAN_POINT('',(30.331418582223,31.9994792732426,175.77148036339));
#30857=CARTESIAN_POINT('',(30.3332690606571,32.0014513847588,175.57851963661));
#30858=CARTESIAN_POINT('',(30.334,32.,172.));
#30859=CARTESIAN_POINT('Ctrl Pts',(30.3332690606571,32.0014513847588,175.57851963661));
#30860=CARTESIAN_POINT('Ctrl Pts',(30.3322967939476,32.1077720140763,175.571400382039));
#30861=CARTESIAN_POINT('Ctrl Pts',(30.3415987476557,32.2139231700336,175.564281127468));
#30862=CARTESIAN_POINT('Ctrl Pts',(30.3617914024463,32.3179605455706,175.557161872896));
#30863=CARTESIAN_POINT('Ctrl Pts',(30.4668588383814,32.8592930450568,175.520118609823));
#30864=CARTESIAN_POINT('Ctrl Pts',(30.8667790797961,33.3433974485404,175.48307534675));
#30865=CARTESIAN_POINT('Ctrl Pts',(31.3785507926964,33.5487502059339,175.446032083677));
#30866=CARTESIAN_POINT('Ctrl Pts',(31.8903225055966,33.7541029633274,175.408988820603));
#30867=CARTESIAN_POINT('Ctrl Pts',(32.5139456899825,33.6807040746309,175.37194555753));
#30868=CARTESIAN_POINT('Ctrl Pts',(32.9640537581348,33.362140473323,175.334902294457));
#30869=CARTESIAN_POINT('Ctrl Pts',(33.4141618262871,33.0435768720152,175.297859031384));
#30870=CARTESIAN_POINT('Ctrl Pts',(33.6907547782058,32.4798485580959,175.260815768311));
#30871=CARTESIAN_POINT('Ctrl Pts',(33.6672651788558,31.9289145513253,175.223772505237));
#30872=CARTESIAN_POINT('Ctrl Pts',(33.6437755795059,31.3779805445546,175.186729242164));
#30873=CARTESIAN_POINT('Ctrl Pts',(33.3202034288872,30.8398408449325,175.149685979091));
#30874=CARTESIAN_POINT('Ctrl Pts',(32.844613588626,30.560745261065,175.112642716018));
#30875=CARTESIAN_POINT('Ctrl Pts',(32.3690237483648,30.2816496771975,175.075599452944));
#30876=CARTESIAN_POINT('Ctrl Pts',(31.7414162184611,30.2615982090847,175.038556189871));
#30877=CARTESIAN_POINT('Ctrl Pts',(31.2489808015386,30.5097662998103,175.001512926798));
#30878=CARTESIAN_POINT('Ctrl Pts',(30.7565453846161,30.757934390536,174.964469663725));
#30879=CARTESIAN_POINT('Ctrl Pts',(30.399282080675,31.2743220401002,174.927426400651));
#30880=CARTESIAN_POINT('Ctrl Pts',(30.340672640419,31.8226330600577,174.890383137578));
#30881=CARTESIAN_POINT('Ctrl Pts',(30.3344158738391,31.8811672151375,174.886428637255));
#30882=CARTESIAN_POINT('Ctrl Pts',(30.3315626632264,31.9400651792653,174.882474136933));
#30883=CARTESIAN_POINT('Ctrl Pts',(30.3319793737621,31.999003930908,174.87851963661));
#30884=CARTESIAN_POINT('Ctrl Pts',(30.3357235801798,31.9988086992918,175.07148036339));
#30885=CARTESIAN_POINT('Ctrl Pts',(30.3344358621602,31.8040492117858,175.084472701363));
#30886=CARTESIAN_POINT('Ctrl Pts',(30.3660188872735,31.6096940838962,175.097465039336));
#30887=CARTESIAN_POINT('Ctrl Pts',(30.4323116977725,31.428003386598,175.11045737731));
#30888=CARTESIAN_POINT('Ctrl Pts',(30.6213232539889,30.9099737362059,175.147500640383));
#30889=CARTESIAN_POINT('Ctrl Pts',(31.0924950276034,30.4948948372859,175.184543903456));
#30890=CARTESIAN_POINT('Ctrl Pts',(31.6302213698328,30.3727045433124,175.221587166529));
#30891=CARTESIAN_POINT('Ctrl Pts',(32.1679477120622,30.250514249339,175.258630429603));
#30892=CARTESIAN_POINT('Ctrl Pts',(32.7722286229063,30.421212560312,175.295673692676));
#30893=CARTESIAN_POINT('Ctrl Pts',(33.1665484341398,30.8066888547031,175.332716955749));
#30894=CARTESIAN_POINT('Ctrl Pts',(33.5608682453733,31.1921651490941,175.369760218822));
#30895=CARTESIAN_POINT('Ctrl Pts',(33.7452269569961,31.7924194269032,175.406803481896));
#30896=CARTESIAN_POINT('Ctrl Pts',(33.6352630222131,32.3327785853487,175.443846744969));
#30897=CARTESIAN_POINT('Ctrl Pts',(33.52529908743,32.8731377437941,175.480890008042));
#30898=CARTESIAN_POINT('Ctrl Pts',(33.1210125062411,33.3536017828761,175.517933271115));
#30899=CARTESIAN_POINT('Ctrl Pts',(32.6074026260459,33.5543129635172,175.554976534188));
#30900=CARTESIAN_POINT('Ctrl Pts',(32.0937927458506,33.7550241441583,175.592019797262));
#30901=CARTESIAN_POINT('Ctrl Pts',(31.470859566649,33.6759824663586,175.629063060335));
#30902=CARTESIAN_POINT('Ctrl Pts',(31.0236539335289,33.3533569732959,175.666106323408));
#30903=CARTESIAN_POINT('Ctrl Pts',(30.5996104381214,33.0474412341954,175.701231003402));
#30904=CARTESIAN_POINT('Ctrl Pts',(30.3335629547701,32.5225201526135,175.736355683396));
#30905=CARTESIAN_POINT('Ctrl Pts',(30.331418582223,31.9994792732426,175.77148036339));
#30906=CARTESIAN_POINT('Origin',(32.,32.,172.));
#30907=CARTESIAN_POINT('',(30.3341900192556,32.0015219962278,176.47148036339));
#30908=CARTESIAN_POINT('',(30.3366800782372,32.0000809155388,176.27851963661));
#30909=CARTESIAN_POINT('',(30.334,32.,172.));
#30910=CARTESIAN_POINT('Ctrl Pts',(30.3366800782372,32.0000809155388,176.27851963661));
#30911=CARTESIAN_POINT('Ctrl Pts',(30.3365617397268,32.2731930172127,176.260326627145));
#30912=CARTESIAN_POINT('Ctrl Pts',(30.4000687460146,32.5462532881901,176.24213361768));
#30913=CARTESIAN_POINT('Ctrl Pts',(30.5275023079567,32.7852240855635,176.223940608215));
#30914=CARTESIAN_POINT('Ctrl Pts',(30.7869731210985,33.2717987850903,176.186897345142));
#30915=CARTESIAN_POINT('Ctrl Pts',(31.3114712794713,33.6170450085694,176.149854082068));
#30916=CARTESIAN_POINT('Ctrl Pts',(31.8609892697898,33.6629799561425,176.112810818995));
#30917=CARTESIAN_POINT('Ctrl Pts',(32.4105072601082,33.7089149037156,176.075767555922));
#30918=CARTESIAN_POINT('Ctrl Pts',(32.9850450823722,33.4555385753826,176.038724292849));
#30919=CARTESIAN_POINT('Ctrl Pts',(33.321697344409,33.0187946051197,176.001681029775));
#30920=CARTESIAN_POINT('Ctrl Pts',(33.6583496064458,32.5820506348568,175.964637766702));
#30921=CARTESIAN_POINT('Ctrl Pts',(33.7571163082553,31.961939022664,175.927594503629));
#30922=CARTESIAN_POINT('Ctrl Pts',(33.5728023426329,31.4422194798622,175.890551240556));
#30923=CARTESIAN_POINT('Ctrl Pts',(33.3884883770104,30.9224999370603,175.853507977482));
#30924=CARTESIAN_POINT('Ctrl Pts',(32.921093743956,30.5031724636493,175.816464714409));
#30925=CARTESIAN_POINT('Ctrl Pts',(32.3844956932118,30.3761190377552,175.779421451336));
#30926=CARTESIAN_POINT('Ctrl Pts',(31.8478976424677,30.2490656118612,175.742378188263));
#30927=CARTESIAN_POINT('Ctrl Pts',(31.2420961740338,30.414286233484,175.705334925189));
#30928=CARTESIAN_POINT('Ctrl Pts',(30.8443027550447,30.7961768420398,175.668291662116));
#30929=CARTESIAN_POINT('Ctrl Pts',(30.522960285069,31.1046728240138,175.638367653614));
#30930=CARTESIAN_POINT('Ctrl Pts',(30.3373557409398,31.5545591738029,175.608443645112));
#30931=CARTESIAN_POINT('Ctrl Pts',(30.3332690606571,32.0014513847588,175.57851963661));
#30932=CARTESIAN_POINT('Ctrl Pts',(30.331418582223,31.9994792732426,175.77148036339));
#30933=CARTESIAN_POINT('Ctrl Pts',(30.3313014521343,31.9709096925072,175.773398946469));
#30934=CARTESIAN_POINT('Ctrl Pts',(30.3319716958771,31.9423457214897,175.775317529549));
#30935=CARTESIAN_POINT('Ctrl Pts',(30.3334465730137,31.9138233576617,175.777236112628));
#30936=CARTESIAN_POINT('Ctrl Pts',(30.3619229326574,31.363124543416,175.814279375701));
#30937=CARTESIAN_POINT('Ctrl Pts',(30.6903537389835,30.8279362232504,175.851322638774));
#30938=CARTESIAN_POINT('Ctrl Pts',(31.1684508358577,30.5531576705442,175.888365901848));
#30939=CARTESIAN_POINT('Ctrl Pts',(31.6465479327319,30.278379117838,175.925409164921));
#30940=CARTESIAN_POINT('Ctrl Pts',(32.2743113201543,30.2640103325911,175.962452427994));
#30941=CARTESIAN_POINT('Ctrl Pts',(32.7644798759482,30.5166263930021,175.999495691067));
#30942=CARTESIAN_POINT('Ctrl Pts',(33.2546484317422,30.7692424534132,176.036538954141));
#30943=CARTESIAN_POINT('Ctrl Pts',(33.6072221559078,31.2888433594821,176.073582217214));
#30944=CARTESIAN_POINT('Ctrl Pts',(33.6608652240127,31.8376625540489,176.110625480287));
#30945=CARTESIAN_POINT('Ctrl Pts',(33.7145082921176,32.3864817486158,176.14766874336));
#30946=CARTESIAN_POINT('Ctrl Pts',(33.4692207041618,32.9645192316805,176.184712006434));
#30947=CARTESIAN_POINT('Ctrl Pts',(33.0372447303886,33.307268185192,176.221755269507));
#30948=CARTESIAN_POINT('Ctrl Pts',(32.6052687566154,33.6500171387034,176.25879853258));
#30949=CARTESIAN_POINT('Ctrl Pts',(31.9866043970249,33.7574775626615,176.295841795653));
#30950=CARTESIAN_POINT('Ctrl Pts',(31.4643491079747,33.5804761499029,176.332885058727));
#30951=CARTESIAN_POINT('Ctrl Pts',(30.9420938189246,33.4034747371442,176.3699283218));
#30952=CARTESIAN_POINT('Ctrl Pts',(30.5162476004149,32.9420114876688,176.406971584873));
#30953=CARTESIAN_POINT('Ctrl Pts',(30.3816753730276,32.4072494819308,176.444014847946));
#30954=CARTESIAN_POINT('Ctrl Pts',(30.3484161037031,32.2750840721826,176.453170019761));
#30955=CARTESIAN_POINT('Ctrl Pts',(30.3329484846486,32.138441414632,176.462325191576));
#30956=CARTESIAN_POINT('Ctrl Pts',(30.3341900192556,32.0015219962278,176.47148036339));
#30957=CARTESIAN_POINT('Origin',(32.,32.,172.));
#30958=CARTESIAN_POINT('',(30.3365877314637,31.9995845740104,177.17148036339));
#30959=CARTESIAN_POINT('',(30.3335660066275,31.9985061125779,176.97851963661));
#30960=CARTESIAN_POINT('',(30.334,32.,172.));
#30961=CARTESIAN_POINT('Ctrl Pts',(30.3335660066275,31.9985061125779,176.97851963661));
#30962=CARTESIAN_POINT('Ctrl Pts',(30.3376018361009,32.4357833033998,176.949252872251));
#30963=CARTESIAN_POINT('Ctrl Pts',(30.5142836011723,32.8759469172232,176.919986107892));
#30964=CARTESIAN_POINT('Ctrl Pts',(30.8231793229629,33.1831819008459,176.890719343533));
#30965=CARTESIAN_POINT('Ctrl Pts',(31.2141520093921,33.5720525728505,176.85367608046));
#30966=CARTESIAN_POINT('Ctrl Pts',(31.8169346432747,33.7479683732478,176.816632817387));
#30967=CARTESIAN_POINT('Ctrl Pts',(32.3556971607286,33.6304311846374,176.779589554313));
#30968=CARTESIAN_POINT('Ctrl Pts',(32.8944596781825,33.5128939960271,176.74254629124));
#30969=CARTESIAN_POINT('Ctrl Pts',(33.3692020792077,33.1019038184092,176.705503028167));
#30970=CARTESIAN_POINT('Ctrl Pts',(33.5626848148218,32.5855275290525,176.668459765094));
#30971=CARTESIAN_POINT('Ctrl Pts',(33.7561675504359,32.0691512396958,176.63141650202));
#30972=CARTESIAN_POINT('Ctrl Pts',(33.6683906206388,31.4473888386002,176.594373238947));
#30973=CARTESIAN_POINT('Ctrl Pts',(33.3395202727796,31.0047554288992,176.557329975874));
#30974=CARTESIAN_POINT('Ctrl Pts',(33.0106499249203,30.5621220191981,176.520286712801));
#30975=CARTESIAN_POINT('Ctrl Pts',(32.4406861589989,30.2986176008915,176.483243449727));
#30976=CARTESIAN_POINT('Ctrl Pts',(31.8904413036908,30.3348203671221,176.446200186654));
#30977=CARTESIAN_POINT('Ctrl Pts',(31.3401964483828,30.3710231333526,176.409156923581));
#30978=CARTESIAN_POINT('Ctrl Pts',(30.8096705036882,30.7069330841203,176.372113660508));
#30979=CARTESIAN_POINT('Ctrl Pts',(30.5416292652962,31.1888396472913,176.335070397435));
#30980=CARTESIAN_POINT('Ctrl Pts',(30.4052307706181,31.4340680688071,176.316220143826));
#30981=CARTESIAN_POINT('Ctrl Pts',(30.3368026918674,31.717102313789,176.297369890218));
#30982=CARTESIAN_POINT('Ctrl Pts',(30.3366800782372,32.0000809155388,176.27851963661));
#30983=CARTESIAN_POINT('Ctrl Pts',(30.3341900192556,32.0015219962278,176.47148036339));
#30984=CARTESIAN_POINT('Ctrl Pts',(30.3379719286637,31.5844439432072,176.499368454649));
#30985=CARTESIAN_POINT('Ctrl Pts',(30.4967992918917,31.1647978060687,176.527256545907));
#30986=CARTESIAN_POINT('Ctrl Pts',(30.7800747867322,30.8613125042108,176.555144637166));
#30987=CARTESIAN_POINT('Ctrl Pts',(31.1563446640889,30.4581982942296,176.592187900239));
#30988=CARTESIAN_POINT('Ctrl Pts',(31.7521826550671,30.2600306362681,176.629231163313));
#30989=CARTESIAN_POINT('Ctrl Pts',(32.294936525987,30.3574899747402,176.666274426386));
#30990=CARTESIAN_POINT('Ctrl Pts',(32.8376903969068,30.4549493132123,176.703317689459));
#30991=CARTESIAN_POINT('Ctrl Pts',(33.3273601477684,30.8480356481179,176.740360952532));
#30992=CARTESIAN_POINT('Ctrl Pts',(33.5398755553043,31.3568748067747,176.777404215605));
#30993=CARTESIAN_POINT('Ctrl Pts',(33.7523909628403,31.8657139654314,176.814447478679));
#30994=CARTESIAN_POINT('Ctrl Pts',(33.6877520270506,32.4903059478392,176.851490741752));
#30995=CARTESIAN_POINT('Ctrl Pts',(33.3755371752704,32.9448408439612,176.888534004825));
#30996=CARTESIAN_POINT('Ctrl Pts',(33.0633223234901,33.3993757400832,176.925577267898));
#30997=CARTESIAN_POINT('Ctrl Pts',(32.5035315557193,33.6838535499193,176.962620530972));
#30998=CARTESIAN_POINT('Ctrl Pts',(31.9523220903062,33.6680987815996,176.999663794045));
#30999=CARTESIAN_POINT('Ctrl Pts',(31.4011126248931,33.65234401328,177.036707057118));
#31000=CARTESIAN_POINT('Ctrl Pts',(30.8584844618377,33.3363566668047,177.073750320191));
#31001=CARTESIAN_POINT('Ctrl Pts',(30.5727413096241,32.86473081535,177.110793583265));
#31002=CARTESIAN_POINT('Ctrl Pts',(30.4167000539667,32.6071810210981,177.131022509973));
#31003=CARTESIAN_POINT('Ctrl Pts',(30.3372653606356,32.3032177331473,177.151251436682));
#31004=CARTESIAN_POINT('Ctrl Pts',(30.3365877314637,31.9995845740104,177.17148036339));
#31005=CARTESIAN_POINT('Origin',(32.,32.,172.));
#31006=CARTESIAN_POINT('',(30.3326674383851,31.998696643609,177.87148036339));
#31007=CARTESIAN_POINT('',(30.3317667672262,32.0008552724323,177.67851963661));
#31008=CARTESIAN_POINT('',(30.334,32.,172.));
#31009=CARTESIAN_POINT('Ctrl Pts',(30.3317667672262,32.0008552724323,177.67851963661));
#31010=CARTESIAN_POINT('Ctrl Pts',(30.3314592141136,32.0499818232188,177.67522238043));
#31011=CARTESIAN_POINT('Ctrl Pts',(30.3334412206569,32.0990832080451,177.671925124251));
#31012=CARTESIAN_POINT('Ctrl Pts',(30.3377935532569,32.1479735799601,177.668627868071));
#31013=CARTESIAN_POINT('Ctrl Pts',(30.3866901486996,32.6972359999809,177.631584604998));
#31014=CARTESIAN_POINT('Ctrl Pts',(30.7347589067126,33.2198652954923,177.594541341925));
#31015=CARTESIAN_POINT('Ctrl Pts',(31.22272531614,33.4767092800123,177.557498078852));
#31016=CARTESIAN_POINT('Ctrl Pts',(31.7106917255674,33.7335532645324,177.520454815778));
#31017=CARTESIAN_POINT('Ctrl Pts',(32.3385557864092,33.724611938061,177.483411552705));
#31018=CARTESIAN_POINT('Ctrl Pts',(32.8190103750928,33.4539767317386,177.446368289632));
#31019=CARTESIAN_POINT('Ctrl Pts',(33.2994649637764,33.1833415254162,177.409325026559));
#31020=CARTESIAN_POINT('Ctrl Pts',(33.6325100803019,32.6510124392426,177.372281763485));
#31021=CARTESIAN_POINT('Ctrl Pts',(33.6657460526844,32.1005804116725,177.335238500412));
#31022=CARTESIAN_POINT('Ctrl Pts',(33.698982025067,31.5501483841025,177.298195237339));
#31023=CARTESIAN_POINT('Ctrl Pts',(33.4324088533065,30.9816134151359,177.261151974266));
#31024=CARTESIAN_POINT('Ctrl Pts',(32.9880089913433,30.6551340066007,177.224108711192));
#31025=CARTESIAN_POINT('Ctrl Pts',(32.5436091293801,30.3286545980654,177.187065448119));
#31026=CARTESIAN_POINT('Ctrl Pts',(31.9213825772142,30.2442307499615,177.150022185046));
#31027=CARTESIAN_POINT('Ctrl Pts',(31.4060568233868,30.4404943658696,177.112978921973));
#31028=CARTESIAN_POINT('Ctrl Pts',(30.8907310695595,30.6367579817777,177.075935658899));
#31029=CARTESIAN_POINT('Ctrl Pts',(30.4823061140706,31.1137090616976,177.038892395826));
#31030=CARTESIAN_POINT('Ctrl Pts',(30.3676750058142,31.6530973734636,177.001849132753));
#31031=CARTESIAN_POINT('Ctrl Pts',(30.3436104771516,31.7663312563613,176.994072634039));
#31032=CARTESIAN_POINT('Ctrl Pts',(30.3324936426885,31.8823167904328,176.986296135324));
#31033=CARTESIAN_POINT('Ctrl Pts',(30.3335660066275,31.9985061125779,176.97851963661));
#31034=CARTESIAN_POINT('Ctrl Pts',(30.3365877314637,31.9995845740104,177.17148036339));
#31035=CARTESIAN_POINT('Ctrl Pts',(30.336024484338,31.7472039043504,177.188294699755));
#31036=CARTESIAN_POINT('Ctrl Pts',(30.3898743158847,31.4950513199463,177.20510903612));
#31037=CARTESIAN_POINT('Ctrl Pts',(30.4993722077054,31.2699705615928,177.221923372484));
#31038=CARTESIAN_POINT('Ctrl Pts',(30.740604399372,30.7741005157242,177.258966635558));
#31039=CARTESIAN_POINT('Ctrl Pts',(31.2519269240771,30.4096247804211,177.296009898631));
#31040=CARTESIAN_POINT('Ctrl Pts',(31.7993613809296,30.3433253796834,177.333053161704));
#31041=CARTESIAN_POINT('Ctrl Pts',(32.3467958377822,30.2770259789457,177.370096424777));
#31042=CARTESIAN_POINT('Ctrl Pts',(32.9303422267822,30.5089029127736,177.407139687851));
#31043=CARTESIAN_POINT('Ctrl Pts',(33.2829728562038,30.9328507493989,177.444182950924));
#31044=CARTESIAN_POINT('Ctrl Pts',(33.6356034856253,31.3567985860242,177.481226213997));
#31045=CARTESIAN_POINT('Ctrl Pts',(33.7573183554684,31.972817325447,177.51826947707));
#31046=CARTESIAN_POINT('Ctrl Pts',(33.5924214588221,32.4990197339482,177.555312740144));
#31047=CARTESIAN_POINT('Ctrl Pts',(33.4275245621758,33.0252221424493,177.592356003217));
#31048=CARTESIAN_POINT('Ctrl Pts',(32.9760158990401,33.4616082200288,177.62939926629));
#31049=CARTESIAN_POINT('Ctrl Pts',(32.444503268266,33.6084908757691,177.666442529363));
#31050=CARTESIAN_POINT('Ctrl Pts',(31.9129906374918,33.7553735315094,177.703485792436));
#31051=CARTESIAN_POINT('Ctrl Pts',(31.3014740390791,33.6127527654104,177.74052905551));
#31052=CARTESIAN_POINT('Ctrl Pts',(30.8897803912795,33.2458894134051,177.777572318583));
#31053=CARTESIAN_POINT('Ctrl Pts',(30.5418867635142,32.935878746237,177.808875000185));
#31054=CARTESIAN_POINT('Ctrl Pts',(30.3366819678508,32.4657417642871,177.840177681788));
#31055=CARTESIAN_POINT('Ctrl Pts',(30.3326674383851,31.998696643609,177.87148036339));
#31056=CARTESIAN_POINT('Origin',(32.,32.,172.));
#31057=CARTESIAN_POINT('',(30.3325025488117,32.0012179414303,178.57148036339));
#31058=CARTESIAN_POINT('',(30.3361333853116,32.0009462961084,178.37851963661));
#31059=CARTESIAN_POINT('',(30.334,32.,172.));
#31060=CARTESIAN_POINT('',(33.2690708798533,33.0793586530475,179.));
#31061=CARTESIAN_POINT('Ctrl Pts',(30.3325025488117,32.0012179414303,178.57148036339));
#31062=CARTESIAN_POINT('Ctrl Pts',(30.3364292156548,31.5283160549018,178.60319045304));
#31063=CARTESIAN_POINT('Ctrl Pts',(30.5476330207047,31.0524199115449,178.634900542691));
#31064=CARTESIAN_POINT('Ctrl Pts',(30.9034954080308,30.7421389970656,178.666610632341));
#31065=CARTESIAN_POINT('Ctrl Pts',(31.3192086455844,30.3796733696121,178.703653895414));
#31066=CARTESIAN_POINT('Ctrl Pts',(31.9323312413379,30.243215736475,178.740697158487));
#31067=CARTESIAN_POINT('Ctrl Pts',(32.4621594780356,30.3962147962734,178.777740421561));
#31068=CARTESIAN_POINT('Ctrl Pts',(32.9919877147334,30.5492138560719,178.814783684634));
#31069=CARTESIAN_POINT('Ctrl Pts',(33.4385215923753,30.9916696088058,178.851826947707));
#31070=CARTESIAN_POINT('Ctrl Pts',(33.5975139507523,31.518714433356,178.88887021078));
#31071=CARTESIAN_POINT('Ctrl Pts',(33.7565063091292,32.0457592579062,178.925913473853));
#31072=CARTESIAN_POINT('Ctrl Pts',(33.6279571482411,32.6573931542727,178.962956736927));
#31073=CARTESIAN_POINT('Ctrl Pts',(33.2690708798531,33.0793586530476,179.));
#31074=CARTESIAN_POINT('',(30.72851190076,33.0811958771907,179.));
#31075=CARTESIAN_POINT('Origin',(32.,32.,179.));
#31076=CARTESIAN_POINT('Ctrl Pts',(30.7285100828332,33.0811972589182,179.));
#31077=CARTESIAN_POINT('Ctrl Pts',(31.0792913246103,33.4926026794485,178.963685183163));
#31078=CARTESIAN_POINT('Ctrl Pts',(31.6490955279031,33.7187060371509,178.927370366326));
#31079=CARTESIAN_POINT('Ctrl Pts',(32.1864012108571,33.658249220712,178.891055549488));
#31080=CARTESIAN_POINT('Ctrl Pts',(32.7344848168854,33.5965796887974,178.854012286415));
#31081=CARTESIAN_POINT('Ctrl Pts',(33.2487530373446,33.2367383424031,178.816969023342));
#31082=CARTESIAN_POINT('Ctrl Pts',(33.4942155657675,32.7430232864054,178.779925760269));
#31083=CARTESIAN_POINT('Ctrl Pts',(33.7396780941904,32.2493082304078,178.742882497195));
#31084=CARTESIAN_POINT('Ctrl Pts',(33.716334930577,31.6217194648069,178.705839234122));
#31085=CARTESIAN_POINT('Ctrl Pts',(33.4347028183851,31.1476160413552,178.668795971049));
#31086=CARTESIAN_POINT('Ctrl Pts',(33.1530707061932,30.6735126179035,178.631752707976));
#31087=CARTESIAN_POINT('Ctrl Pts',(32.6131496454229,30.352894536601,178.594709444902));
#31088=CARTESIAN_POINT('Ctrl Pts',(32.0620856027671,30.3323875673963,178.557666181829));
#31089=CARTESIAN_POINT('Ctrl Pts',(31.5110215601112,30.3118805981917,178.520622918756));
#31090=CARTESIAN_POINT('Ctrl Pts',(30.9488145355698,30.5914847410848,178.483579655683));
#31091=CARTESIAN_POINT('Ctrl Pts',(30.6326876217354,31.0432975466902,178.446536392609));
#31092=CARTESIAN_POINT('Ctrl Pts',(30.4392028026414,31.319828633198,178.42386414061));
#31093=CARTESIAN_POINT('Ctrl Pts',(30.3379002457712,31.6608695415591,178.40119188861));
#31094=CARTESIAN_POINT('Ctrl Pts',(30.3361333853116,32.0009462961084,178.37851963661));
#31095=CARTESIAN_POINT('Origin',(32.,32.,180.545925280538));
#31096=CARTESIAN_POINT('',(29.9466856106202,32.0018139367885,166.254074719462));
#31097=CARTESIAN_POINT('',(29.9453305521271,31.9981395289548,166.195925280538));
#31098=CARTESIAN_POINT('',(29.94525,32.0000000000002,180.545925280538));
#31099=CARTESIAN_POINT('',(32.3836679988478,34.0186125009917,166.));
#31100=CARTESIAN_POINT('Ctrl Pts',(29.9453305521271,31.9981395289548,166.195925280538));
#31101=CARTESIAN_POINT('Ctrl Pts',(29.9505790914998,32.5195345061705,166.167660116765));
#31102=CARTESIAN_POINT('Ctrl Pts',(30.4181723873308,33.7318542488392,166.102351689919));
#31103=CARTESIAN_POINT('Ctrl Pts',(31.7124802469762,34.1461819386551,166.037043263073));
#31104=CARTESIAN_POINT('Ctrl Pts',(32.3836679988478,34.0186125009917,166.));
#31105=CARTESIAN_POINT('',(33.3415940970262,33.5612502368267,166.));
#31106=CARTESIAN_POINT('Origin',(32.,32.,166.));
#31107=CARTESIAN_POINT('Ctrl Pts',(29.9466856106202,32.0018139367885,166.254074719462));
#31108=CARTESIAN_POINT('Ctrl Pts',(29.9450188939236,32.21116652697,166.242741226219));
#31109=CARTESIAN_POINT('Ctrl Pts',(30.0707146480112,33.1027772339307,166.194364469902));
#31110=CARTESIAN_POINT('Ctrl Pts',(31.3452942359773,34.3307277928868,166.109672896748));
#31111=CARTESIAN_POINT('Ctrl Pts',(32.8352805948106,33.9951595674105,166.036314816837));
#31112=CARTESIAN_POINT('Ctrl Pts',(33.3415960466846,33.561252269086,166.));
#31113=CARTESIAN_POINT('Origin',(32.,32.,180.545925280538));
#31114=CARTESIAN_POINT('',(29.9479603212001,31.9988941585155,166.954074719462));
#31115=CARTESIAN_POINT('',(29.9421602766058,32.0007586547802,166.895925280538));
#31116=CARTESIAN_POINT('',(29.94525,32.0000000000002,180.545925280538));
#31117=CARTESIAN_POINT('Ctrl Pts',(29.9421602766058,32.0007586547802,166.895925280538));
#31118=CARTESIAN_POINT('Ctrl Pts',(29.9419599928232,32.0429254387486,166.893629624944));
#31119=CARTESIAN_POINT('Ctrl Pts',(29.9622502782122,32.7653095976581,166.854290706278));
#31120=CARTESIAN_POINT('Ctrl Pts',(30.8113032934655,34.1178215046619,166.777908524538));
#31121=CARTESIAN_POINT('Ctrl Pts',(33.1343552393677,34.1473557540512,166.666778735318));
#31122=CARTESIAN_POINT('Ctrl Pts',(34.4195276894793,32.2117592010123,166.555648946099));
#31123=CARTESIAN_POINT('Ctrl Pts',(33.4898246183641,30.0821472766194,166.444519156879));
#31124=CARTESIAN_POINT('Ctrl Pts',(31.1977703849704,29.7081726882415,166.333389367659));
#31125=CARTESIAN_POINT('Ctrl Pts',(30.034435938876,30.9926242945928,166.250524742212));
#31126=CARTESIAN_POINT('Ctrl Pts',(29.943700552734,31.8362138128461,166.204703379838));
#31127=CARTESIAN_POINT('Ctrl Pts',(29.9453305521271,31.9981395289548,166.195925280538));
#31128=CARTESIAN_POINT('Ctrl Pts',(29.9479603212001,31.9988941585155,166.954074719462));
#31129=CARTESIAN_POINT('Ctrl Pts',(29.9499871753085,32.4134609401804,166.931667471325));
#31130=CARTESIAN_POINT('Ctrl Pts',(30.2732187069358,33.5162878102792,166.872216960114));
#31131=CARTESIAN_POINT('Ctrl Pts',(32.073044548561,34.4275128335807,166.77572318583));
#31132=CARTESIAN_POINT('Ctrl Pts',(34.0790345884103,33.255346086573,166.66459339661));
#31133=CARTESIAN_POINT('Ctrl Pts',(34.1822756467128,30.9342420768624,166.553463607391));
#31134=CARTESIAN_POINT('Ctrl Pts',(32.2884012470789,29.5886265247524,166.442333818171));
#31135=CARTESIAN_POINT('Ctrl Pts',(30.3505030706617,30.3618237232923,166.342537522195));
#31136=CARTESIAN_POINT('Ctrl Pts',(29.9504665192701,31.5269023811822,166.279784489292));
#31137=CARTESIAN_POINT('Ctrl Pts',(29.9466856106202,32.0018139367885,166.254074719462));
#31138=CARTESIAN_POINT('Origin',(32.,32.,180.545925280538));
#31139=CARTESIAN_POINT('',(29.9425974682135,31.9988731389439,167.654074719462));
#31140=CARTESIAN_POINT('',(29.9475247189157,32.0013942611211,167.595925280538));
#31141=CARTESIAN_POINT('',(29.94525,32.0000000000002,180.545925280538));
#31142=CARTESIAN_POINT('Ctrl Pts',(29.9475247189157,32.0013942611211,167.595925280538));
#31143=CARTESIAN_POINT('Ctrl Pts',(29.9459809856321,32.2486160756999,167.582555870051));
#31144=CARTESIAN_POINT('Ctrl Pts',(30.1017580865117,33.1789472430918,167.53214319649));
#31145=CARTESIAN_POINT('Ctrl Pts',(31.4859258624946,34.3735884913369,167.444687259856));
#31146=CARTESIAN_POINT('Ctrl Pts',(33.7152536393985,33.7193295360918,167.333557470637));
#31147=CARTESIAN_POINT('Ctrl Pts',(34.3748036771893,31.4915603207829,167.222427681417));
#31148=CARTESIAN_POINT('Ctrl Pts',(32.8609514252531,29.7291065603519,167.111297892197));
#31149=CARTESIAN_POINT('Ctrl Pts',(30.606730126964,30.0384313727369,167.002463758571));
#31150=CARTESIAN_POINT('Ctrl Pts',(29.9451918211818,31.3625118453315,166.930672888018));
#31151=CARTESIAN_POINT('Ctrl Pts',(29.9421602766058,32.0007586547802,166.895925280538));
#31152=CARTESIAN_POINT('Ctrl Pts',(29.9425974682135,31.9988731389439,167.654074719462));
#31153=CARTESIAN_POINT('Ctrl Pts',(29.9466607983974,32.6141954522381,167.620593716431));
#31154=CARTESIAN_POINT('Ctrl Pts',(30.5667381595166,33.9174120322558,167.550069450326));
#31155=CARTESIAN_POINT('Ctrl Pts',(32.7830165295865,34.2989296881618,167.442501921148));
#31156=CARTESIAN_POINT('Ctrl Pts',(34.3560823145915,32.5891267546308,167.331372131929));
#31157=CARTESIAN_POINT('Ctrl Pts',(33.7728865672594,30.3401605876776,167.220242342709));
#31158=CARTESIAN_POINT('Ctrl Pts',(31.5671653767747,29.6102631127892,167.109112553489));
#31159=CARTESIAN_POINT('Ctrl Pts',(30.1224391142159,30.7736143308135,167.020390012407));
#31160=CARTESIAN_POINT('Ctrl Pts',(29.9466364162377,31.7281065289479,166.968710734398));
#31161=CARTESIAN_POINT('Ctrl Pts',(29.9479603212001,31.9988941585155,166.954074719462));
#31162=CARTESIAN_POINT('Origin',(32.,32.,180.545925280538));
#31163=CARTESIAN_POINT('',(29.9445665862919,32.0018241253517,168.354074719462));
#31164=CARTESIAN_POINT('',(29.9472120516653,31.998458524753,168.295925280538));
#31165=CARTESIAN_POINT('',(29.94525,32.0000000000002,180.545925280538));
#31166=CARTESIAN_POINT('Ctrl Pts',(29.9472120516653,31.998458524753,168.295925280538));
#31167=CARTESIAN_POINT('Ctrl Pts',(29.9503631280156,32.4502786971803,168.271482115157));
#31168=CARTESIAN_POINT('Ctrl Pts',(30.3199260724322,33.5915112303712,168.209995686702));
#31169=CARTESIAN_POINT('Ctrl Pts',(32.2059575727712,34.4198709905092,168.111465995175));
#31170=CARTESIAN_POINT('Ctrl Pts',(34.1446869293352,33.1395227135096,168.000336205955));
#31171=CARTESIAN_POINT('Ctrl Pts',(34.1206221195246,30.8162956275684,167.889206416735));
#31172=CARTESIAN_POINT('Ctrl Pts',(32.1557868348082,29.5763819040772,167.778076627516));
#31173=CARTESIAN_POINT('Ctrl Pts',(30.3019081319035,30.4368608022391,167.680316248783));
#31174=CARTESIAN_POINT('Ctrl Pts',(29.9502582810442,31.5636268068268,167.619599133124));
#31175=CARTESIAN_POINT('Ctrl Pts',(29.9475247189157,32.0013942611211,167.595925280538));
#31176=CARTESIAN_POINT('Ctrl Pts',(29.9445665862919,32.0018241253517,168.354074719462));
#31177=CARTESIAN_POINT('Ctrl Pts',(29.9432922113974,32.1402164550963,168.34656322461));
#31178=CARTESIAN_POINT('Ctrl Pts',(30.0191193705774,32.9597079858832,168.302008466685));
#31179=CARTESIAN_POINT('Ctrl Pts',(31.1194450837624,34.2633639270065,168.220410445687));
#31180=CARTESIAN_POINT('Ctrl Pts',(33.4238724584211,33.9674299065165,168.109280656467));
#31181=CARTESIAN_POINT('Ctrl Pts',(34.4251872041711,31.8709253771026,167.998150867247));
#31182=CARTESIAN_POINT('Ctrl Pts',(33.206996913019,29.8925485313441,167.887021078027));
#31183=CARTESIAN_POINT('Ctrl Pts',(30.8841761520946,29.8428884386802,167.775891288808));
#31184=CARTESIAN_POINT('Ctrl Pts',(29.9746984974497,31.187581664638,167.698242502619));
#31185=CARTESIAN_POINT('Ctrl Pts',(29.9421651442853,31.9334050259535,167.657636979504));
#31186=CARTESIAN_POINT('Ctrl Pts',(29.9425974682135,31.9988731389439,167.654074719462));
#31187=CARTESIAN_POINT('Origin',(32.,32.,180.545925280538));
#31188=CARTESIAN_POINT('',(29.9485596886742,31.9999806718114,169.054074719462));
#31189=CARTESIAN_POINT('',(29.9419793320997,31.9994845592423,168.995925280538));
#31190=CARTESIAN_POINT('',(29.94525,32.0000000000002,180.545925280538));
#31191=CARTESIAN_POINT('Ctrl Pts',(29.9419793320997,31.9994845592423,168.995925280538));
#31192=CARTESIAN_POINT('Ctrl Pts',(29.9441754476556,32.6517037695688,168.960408360263));
#31193=CARTESIAN_POINT('Ctrl Pts',(30.6316772116244,33.9881562660024,168.887848176915));
#31194=CARTESIAN_POINT('Ctrl Pts',(32.9078114849742,34.2525701817925,168.778244730493));
#31195=CARTESIAN_POINT('Ctrl Pts',(34.384824085665,32.4591385359132,168.667114941273));
#31196=CARTESIAN_POINT('Ctrl Pts',(33.6792715462419,30.2455082814088,168.555985152054));
#31197=CARTESIAN_POINT('Ctrl Pts',(31.43686789712,29.6375698204928,168.444855362834));
#31198=CARTESIAN_POINT('Ctrl Pts',(30.0896997832934,30.8498681507073,168.358168738995));
#31199=CARTESIAN_POINT('Ctrl Pts',(29.9455877174504,31.7655517705286,168.30852537823));
#31200=CARTESIAN_POINT('Ctrl Pts',(29.9472120516653,31.998458524753,168.295925280538));
#31201=CARTESIAN_POINT('Ctrl Pts',(29.9485596886742,31.9999806718114,169.054074719462));
#31202=CARTESIAN_POINT('Ctrl Pts',(29.9485885621676,32.3440857065745,169.035489469716));
#31203=CARTESIAN_POINT('Ctrl Pts',(30.1937796180674,33.3740837021047,168.979860956897));
#31204=CARTESIAN_POINT('Ctrl Pts',(31.8232672732892,34.4221805810845,168.887189181005));
#31205=CARTESIAN_POINT('Ctrl Pts',(33.9390539828564,33.4622800263533,168.776059391785));
#31206=CARTESIAN_POINT('Ctrl Pts',(34.2802395155314,31.1641166493491,168.664929602565));
#31207=CARTESIAN_POINT('Ctrl Pts',(32.5345745716517,29.6309446499222,168.553799813346));
#31208=CARTESIAN_POINT('Ctrl Pts',(30.4507344632293,30.2229880222625,168.450181518978));
#31209=CARTESIAN_POINT('Ctrl Pts',(29.9495768465332,31.4577286708363,168.383606487683));
#31210=CARTESIAN_POINT('Ctrl Pts',(29.9445665862919,32.0018241253517,168.354074719462));
#31211=CARTESIAN_POINT('Origin',(32.,32.,180.545925280538));
#31212=CARTESIAN_POINT('',(29.9444956521926,31.9981860244656,169.754074719462));
#31213=CARTESIAN_POINT('',(29.945699695435,32.0018685376852,169.695925280538));
#31214=CARTESIAN_POINT('',(29.94525,32.0000000000002,180.545925280538));
#31215=CARTESIAN_POINT('Ctrl Pts',(29.945699695435,32.0018685376852,169.695925280538));
#31216=CARTESIAN_POINT('Ctrl Pts',(29.944124321843,32.1780191762476,169.686377868442));
#31217=CARTESIAN_POINT('Ctrl Pts',(30.045488237746,33.0358359740345,169.639787193273));
#31218=CARTESIAN_POINT('Ctrl Pts',(31.2447903468041,34.3082141355403,169.556153255031));
#31219=CARTESIAN_POINT('Ctrl Pts',(33.5295398276061,33.8864522341055,169.445023465811));
#31220=CARTESIAN_POINT('Ctrl Pts',(34.4144710453466,31.738229705738,169.333893676592));
#31221=CARTESIAN_POINT('Ctrl Pts',(33.0897045462445,29.8295765119025,169.222763887372));
#31222=CARTESIAN_POINT('Ctrl Pts',(30.7676522637518,29.9072713571029,169.111634098153));
#31223=CARTESIAN_POINT('Ctrl Pts',(29.9551025731251,31.2632688429224,169.036021229208));
#31224=CARTESIAN_POINT('Ctrl Pts',(29.9418849538389,31.9714553808426,168.997451623336));
#31225=CARTESIAN_POINT('Ctrl Pts',(29.9419793320997,31.9994845592423,168.995925280538));
#31226=CARTESIAN_POINT('Ctrl Pts',(29.9444956521925,31.9981860244657,169.754074719462));
#31227=CARTESIAN_POINT('Ctrl Pts',(29.949518107583,32.5445771748198,169.724415714823));
#31228=CARTESIAN_POINT('Ctrl Pts',(30.454270674604,33.7815914342631,169.65771344711));
#31229=CARTESIAN_POINT('Ctrl Pts',(32.5426883094078,34.3672098814547,169.553967916323));
#31230=CARTESIAN_POINT('Ctrl Pts',(34.2830900415719,32.8280658706275,169.442838127104));
#31231=CARTESIAN_POINT('Ctrl Pts',(33.9340325267706,30.5310849550035,169.331708337884));
#31232=CARTESIAN_POINT('Ctrl Pts',(31.8149694171768,29.5784391588377,169.220578548664));
#31233=CARTESIAN_POINT('Ctrl Pts',(30.1913146327685,30.6306661769337,169.12803400919));
#31234=CARTESIAN_POINT('Ctrl Pts',(29.9485310128515,31.6582314134216,169.07253273279));
#31235=CARTESIAN_POINT('Ctrl Pts',(29.9485596886742,31.9999806718114,169.054074719462));
#31236=CARTESIAN_POINT('Origin',(32.,32.,180.545925280538));
#31237=CARTESIAN_POINT('',(29.9426482690414,32.0011604961315,170.454074719462));
#31238=CARTESIAN_POINT('',(29.9483814718272,31.9993739362355,170.395925280538));
#31239=CARTESIAN_POINT('',(29.94525,32.0000000000002,180.545925280538));
#31240=CARTESIAN_POINT('Ctrl Pts',(29.9483814718272,31.9993739362354,170.395925280538));
#31241=CARTESIAN_POINT('Ctrl Pts',(29.9494242471388,32.3810912191388,170.375304113548));
#31242=CARTESIAN_POINT('Ctrl Pts',(30.2347805600279,33.4499627199415,170.317639683485));
#31243=CARTESIAN_POINT('Ctrl Pts',(31.9562576159421,34.4282258378547,170.22293199035));
#31244=CARTESIAN_POINT('Ctrl Pts',(34.0162673880548,33.3538315758082,170.11180220113));
#31245=CARTESIAN_POINT('Ctrl Pts',(34.2310111121289,31.0404253372741,170.00067241191));
#31246=CARTESIAN_POINT('Ctrl Pts',(32.4039576606909,29.6052114239129,169.88954262269));
#31247=CARTESIAN_POINT('Ctrl Pts',(30.3959344072883,30.2966919391978,169.787960245566));
#31248=CARTESIAN_POINT('Ctrl Pts',(29.9502366565598,31.494567537263,169.723421131515));
#31249=CARTESIAN_POINT('Ctrl Pts',(29.945699695435,32.0018685376852,169.695925280538));
#31250=CARTESIAN_POINT('Ctrl Pts',(29.9426482690414,32.0011604961315,170.454074719462));
#31251=CARTESIAN_POINT('Ctrl Pts',(29.9421898451266,32.068971401295,170.450385223002));
#31252=CARTESIAN_POINT('Ctrl Pts',(29.9759960847807,32.8171543406774,170.409652463468));
#31253=CARTESIAN_POINT('Ctrl Pts',(30.8915734045388,34.1609219575215,170.331876440861));
#31254=CARTESIAN_POINT('Ctrl Pts',(33.2142103990771,34.1033036706089,170.220746651642));
#31255=CARTESIAN_POINT('Ctrl Pts',(34.4256152039436,32.1207646737337,170.109616862422));
#31256=CARTESIAN_POINT('Ctrl Pts',(33.4171232788624,30.0277031570956,169.998487073202));
#31257=CARTESIAN_POINT('Ctrl Pts',(31.1116954970284,29.7396663224151,169.887357283982));
#31258=CARTESIAN_POINT('Ctrl Pts',(30.0175516100133,31.0450458879601,169.805886499402));
#31259=CARTESIAN_POINT('Ctrl Pts',(29.9432452019828,31.8621499872163,169.761458977896));
#31260=CARTESIAN_POINT('Ctrl Pts',(29.9444956521925,31.9981860244657,169.754074719462));
#31261=CARTESIAN_POINT('Origin',(32.,32.,180.545925280538));
#31262=CARTESIAN_POINT('',(29.9479977188782,32.00107469184,171.154074719462));
#31263=CARTESIAN_POINT('',(29.9434062437882,31.9984640338121,171.095925280538));
#31264=CARTESIAN_POINT('',(29.94525,32.0000000000002,180.545925280538));
#31265=CARTESIAN_POINT('Ctrl Pts',(29.9434062437882,31.9984640338121,171.095925280538));
#31266=CARTESIAN_POINT('Ctrl Pts',(29.9482705271819,32.581561595502,171.064230358654));
#31267=CARTESIAN_POINT('Ctrl Pts',(30.5126646761233,33.8543847693451,170.995492173698));
#31268=CARTESIAN_POINT('Ctrl Pts',(32.6715856907677,34.3339166171362,170.889710725668));
#31269=CARTESIAN_POINT('Ctrl Pts',(34.3250344470753,32.7017185587553,170.778580936448));
#31270=CARTESIAN_POINT('Ctrl Pts',(33.8506368913683,30.4273152852224,170.667451147229));
#31271=CARTESIAN_POINT('Ctrl Pts',(31.6825565220024,29.5922160075984,170.556321358009));
#31272=CARTESIAN_POINT('Ctrl Pts',(30.1533956337356,30.7067605986327,170.465812735779));
#31273=CARTESIAN_POINT('Ctrl Pts',(29.947551035976,31.6953854228851,170.412347376621));
#31274=CARTESIAN_POINT('Ctrl Pts',(29.9483814718272,31.9993739362354,170.395925280538));
#31275=CARTESIAN_POINT('Ctrl Pts',(29.9479977188782,32.00107469184,171.154074719462));
#31276=CARTESIAN_POINT('Ctrl Pts',(29.9467021955612,32.2742285838469,171.139311468108));
#31277=CARTESIAN_POINT('Ctrl Pts',(30.1245753039347,33.2311487980768,171.087504953681));
#31278=CARTESIAN_POINT('Ctrl Pts',(31.5753550254538,34.3912067810244,170.99865517618));
#31279=CARTESIAN_POINT('Ctrl Pts',(33.7785634234029,33.6537549313479,170.88752538696));
#31280=CARTESIAN_POINT('Ctrl Pts',(34.3540498639709,31.4028045027273,170.77639559774));
#31281=CARTESIAN_POINT('Ctrl Pts',(32.7751353976405,29.6984009168952,170.66526580852));
#31282=CARTESIAN_POINT('Ctrl Pts',(30.5627970543453,30.087049665636,170.557825515761));
#31283=CARTESIAN_POINT('Ctrl Pts',(29.9467925105193,31.3881367057915,170.487428486075));
#31284=CARTESIAN_POINT('Ctrl Pts',(29.9426482690414,32.0011604961315,170.454074719462));
#31285=CARTESIAN_POINT('Origin',(32.,32.,180.545925280538));
#31286=CARTESIAN_POINT('',(29.9465668753081,31.9982546176146,171.854074719462));
#31287=CARTESIAN_POINT('',(29.9435984346504,32.0016034614759,171.795925280538));
#31288=CARTESIAN_POINT('',(29.94525,32.0000000000002,180.545925280538));
#31289=CARTESIAN_POINT('Ctrl Pts',(29.9435984346504,32.0016034614759,171.795925280538));
#31290=CARTESIAN_POINT('Ctrl Pts',(29.9426937786247,32.106960608704,171.790199866834));
#31291=CARTESIAN_POINT('Ctrl Pts',(29.9979550561808,32.8930239645319,171.747431190057));
#31292=CARTESIAN_POINT('Ctrl Pts',(31.0116476380733,34.2184124333546,171.667619250206));
#31293=CARTESIAN_POINT('Ctrl Pts',(33.3276380331233,34.0336104269975,171.556489460986));
#31294=CARTESIAN_POINT('Ctrl Pts',(34.4285884978939,31.987670211439,171.445359671767));
#31295=CARTESIAN_POINT('Ctrl Pts',(33.3069211063375,29.9530140846606,171.334229882547));
#31296=CARTESIAN_POINT('Ctrl Pts',(30.9891736912303,29.7917372689629,171.223100093327));
#31297=CARTESIAN_POINT('Ctrl Pts',(29.9937162190609,31.1210399352016,171.143665225991));
#31298=CARTESIAN_POINT('Ctrl Pts',(29.9425854231113,31.9000695743339,171.101273621728));
#31299=CARTESIAN_POINT('Ctrl Pts',(29.9434062437882,31.9984640338121,171.095925280538));
#31300=CARTESIAN_POINT('Ctrl Pts',(29.9465668753081,31.9982546176146,171.854074719462));
#31301=CARTESIAN_POINT('Ctrl Pts',(29.9504207898182,32.475460648146,171.828237713214));
#31302=CARTESIAN_POINT('Ctrl Pts',(30.3537285412576,33.6427251812827,171.765357443893));
#31303=CARTESIAN_POINT('Ctrl Pts',(32.2966168104817,34.41043807051,171.665433911498));
#31304=CARTESIAN_POINT('Ctrl Pts',(34.1859362572401,33.0582418926255,171.554304122278));
#31305=CARTESIAN_POINT('Ctrl Pts',(34.0747105468639,30.7375542107656,171.443174333058));
#31306=CARTESIAN_POINT('Ctrl Pts',(32.064732243297,29.5722432245585,171.332044543839));
#31307=CARTESIAN_POINT('Ctrl Pts',(30.2704012907663,30.4884300601829,171.235678005973));
#31308=CARTESIAN_POINT('Ctrl Pts',(29.9499528623619,31.5888435532568,171.176354731181));
#31309=CARTESIAN_POINT('Ctrl Pts',(29.9479977188782,32.00107469184,171.154074719462));
#31310=CARTESIAN_POINT('Origin',(32.,32.,180.545925280538));
#31311=CARTESIAN_POINT('',(29.9418222293735,31.9999545502986,172.554074719462));
#31312=CARTESIAN_POINT('',(29.9484394608427,32.0005167851038,172.495925280538));
#31313=CARTESIAN_POINT('',(29.94525,32.0000000000002,180.545925280538));
#31314=CARTESIAN_POINT('Ctrl Pts',(29.9484394608427,32.0005167851038,172.495925280538));
#31315=CARTESIAN_POINT('Ctrl Pts',(29.9477393579576,32.3115072125305,172.47912611194));
#31316=CARTESIAN_POINT('Ctrl Pts',(30.1602043414638,33.3073440021902,172.425283680269));
#31317=CARTESIAN_POINT('Ctrl Pts',(31.7070205866564,34.4108830704008,172.334397985525));
#31318=CARTESIAN_POINT('Ctrl Pts',(33.8665099204009,33.5538129980256,172.223268196305));
#31319=CARTESIAN_POINT('Ctrl Pts',(34.3177896164518,31.2747101202577,172.112138407085));
#31320=CARTESIAN_POINT('Ctrl Pts',(32.6478533909077,29.6593846749887,172.001008617865));
#31321=CARTESIAN_POINT('Ctrl Pts',(30.5015906644606,30.1590252373003,171.89560424235));
#31322=CARTESIAN_POINT('Ctrl Pts',(29.9485468772622,31.4253028764944,171.827243129907));
#31323=CARTESIAN_POINT('Ctrl Pts',(29.9435984346504,32.0016034614759,171.795925280538));
#31324=CARTESIAN_POINT('Ctrl Pts',(29.9418227148716,31.999954556736,172.554074719462));
#31325=CARTESIAN_POINT('Ctrl Pts',(29.9420432276356,32.6776310800843,172.51716395832));
#31326=CARTESIAN_POINT('Ctrl Pts',(30.6781937929071,34.0358273911652,172.443209934105));
#31327=CARTESIAN_POINT('Ctrl Pts',(32.9916984982474,34.2169184271411,172.332212646816));
#31328=CARTESIAN_POINT('Ctrl Pts',(34.4003732162344,32.369325935738,172.221082857597));
#31329=CARTESIAN_POINT('Ctrl Pts',(33.6122523976872,30.1837303531204,172.109953068377));
#31330=CARTESIAN_POINT('Ctrl Pts',(31.3486156689259,29.6603650547029,171.998823279157));
#31331=CARTESIAN_POINT('Ctrl Pts',(30.0688017848057,30.9020694849232,171.913530496186));
#31332=CARTESIAN_POINT('Ctrl Pts',(29.9448953211285,31.791276561209,171.865280976287));
#31333=CARTESIAN_POINT('Ctrl Pts',(29.9465668753081,31.9982546176146,171.854074719462));
#31334=CARTESIAN_POINT('Origin',(32.,32.,180.545925280538));
#31335=CARTESIAN_POINT('',(29.946434452345,32.0017741612164,173.254074719462));
#31336=CARTESIAN_POINT('',(29.9454927345275,31.9981230384932,173.195925280538));
#31337=CARTESIAN_POINT('',(29.94525,32.0000000000002,180.545925280538));
#31338=CARTESIAN_POINT('Ctrl Pts',(29.9454927345275,31.9981230384932,173.195925280538));
#31339=CARTESIAN_POINT('Ctrl Pts',(29.9501524846043,32.5122490504339,173.168052357046));
#31340=CARTESIAN_POINT('Ctrl Pts',(30.4058323872152,33.7170163615654,173.103136170481));
#31341=CARTESIAN_POINT('Ctrl Pts',(32.4282525872759,34.3905634978557,173.001176720843));
#31342=CARTESIAN_POINT('Ctrl Pts',(34.2406392525365,32.936872379666,172.890046931623));
#31343=CARTESIAN_POINT('Ctrl Pts',(34.0024171725965,30.6257658195639,172.778917142403));
#31344=CARTESIAN_POINT('Ctrl Pts',(31.9316046116063,29.5723434784478,172.667787353184));
#31345=CARTESIAN_POINT('Ctrl Pts',(30.2269632474166,30.5640710925998,172.573456732562));
#31346=CARTESIAN_POINT('Ctrl Pts',(29.9492831305079,31.6257530247971,172.516169375013));
#31347=CARTESIAN_POINT('Ctrl Pts',(29.9484394608427,32.0005167851038,172.495925280538));
#31348=CARTESIAN_POINT('Ctrl Pts',(29.946434452345,32.0017741612165,173.254074719462));
#31349=CARTESIAN_POINT('Ctrl Pts',(29.9447676909038,32.2038246610773,173.2431334665));
#31350=CARTESIAN_POINT('Ctrl Pts',(30.0649649197711,33.0880078735651,173.195148950464));
#31351=CARTESIAN_POINT('Ctrl Pts',(31.3319367435559,34.3349271314997,173.110121171355));
#31352=CARTESIAN_POINT('Ctrl Pts',(33.5992505443295,33.8277283497517,172.998991382135));
#31353=CARTESIAN_POINT('Ctrl Pts',(34.4029475900826,31.6478124031995,172.887861592915));
#31354=CARTESIAN_POINT('Ctrl Pts',(33.0074930602737,29.7902147259237,172.776731803695));
#31355=CARTESIAN_POINT('Ctrl Pts',(30.6899918075095,29.9549885673591,172.665602014476));
#31356=CARTESIAN_POINT('Ctrl Pts',(29.9429274456235,31.3149806222681,172.591382986398));
#31357=CARTESIAN_POINT('Ctrl Pts',(29.9418219232767,31.9975218394128,172.554207221394));
#31358=CARTESIAN_POINT('Ctrl Pts',(29.9418227148716,31.999954556736,172.554074719462));
#31359=CARTESIAN_POINT('Origin',(32.,32.,180.545925280538));
#31360=CARTESIAN_POINT('',(29.9480726635453,31.9989926864899,173.954074719462));
#31361=CARTESIAN_POINT('',(29.942062549472,32.0006373960264,173.895925280538));
#31362=CARTESIAN_POINT('',(29.94525,32.0000000000002,180.545925280538));
#31363=CARTESIAN_POINT('Ctrl Pts',(29.942062549472,32.0006373960264,173.895925280538));
#31364=CARTESIAN_POINT('Ctrl Pts',(29.9419201864895,32.0355947650604,173.894021865225));
#31365=CARTESIAN_POINT('Ctrl Pts',(29.958567925244,32.7507355624424,173.85507518684));
#31366=CARTESIAN_POINT('Ctrl Pts',(30.7889645417425,34.1051335431823,173.779085245381));
#31367=CARTESIAN_POINT('Ctrl Pts',(33.1116860073988,34.1592471689786,173.667955456161));
#31368=CARTESIAN_POINT('Ctrl Pts',(34.4170044948166,32.2372412017861,173.556825666941));
#31369=CARTESIAN_POINT('Ctrl Pts',(33.5103066799004,30.0981146594927,173.445695877722));
#31370=CARTESIAN_POINT('Ctrl Pts',(31.2213925701334,29.6995729557439,173.334566088502));
#31371=CARTESIAN_POINT('Ctrl Pts',(30.0404201711272,30.9782715144633,173.251309222774));
#31372=CARTESIAN_POINT('Ctrl Pts',(29.9439596520511,31.8289728552132,173.205095620119));
#31373=CARTESIAN_POINT('Ctrl Pts',(29.9454927345275,31.9981230384932,173.195925280538));
#31374=CARTESIAN_POINT('Ctrl Pts',(29.9480726635453,31.9989926864899,173.954074719462));
#31375=CARTESIAN_POINT('Ctrl Pts',(29.9498795229274,32.4063578846345,173.932059711606));
#31376=CARTESIAN_POINT('Ctrl Pts',(30.264575074801,33.501743750801,173.873001440676));
#31377=CARTESIAN_POINT('Ctrl Pts',(32.0474062520575,34.428156887701,173.776899906673));
#31378=CARTESIAN_POINT('Ctrl Pts',(34.0656489763292,33.2772186698503,173.665770117453));
#31379=CARTESIAN_POINT('Ctrl Pts',(34.1934321584947,30.9573837762123,173.554640328233));
#31380=CARTESIAN_POINT('Ctrl Pts',(32.3138100159872,29.5917399438827,173.443510539014));
#31381=CARTESIAN_POINT('Ctrl Pts',(30.3603257898609,30.3475681436841,173.343322002757));
#31382=CARTESIAN_POINT('Ctrl Pts',(29.9504107632974,31.5197522019245,173.280176729573));
#31383=CARTESIAN_POINT('Ctrl Pts',(29.946434452345,32.0017741612165,173.254074719462));
#31384=CARTESIAN_POINT('Origin',(32.,32.,180.545925280538));
#31385=CARTESIAN_POINT('',(29.9427578740922,31.9987715048219,174.654074719462));
#31386=CARTESIAN_POINT('',(29.9473695970145,32.0014721867752,174.595925280538));
#31387=CARTESIAN_POINT('',(29.94525,32.0000000000002,180.545925280538));
#31388=CARTESIAN_POINT('Ctrl Pts',(29.9473695970144,32.0014721867751,174.595925280538));
#31389=CARTESIAN_POINT('Ctrl Pts',(29.9457798098806,32.2413952649533,174.582948110331));
#31390=CARTESIAN_POINT('Ctrl Pts',(30.0955630473742,33.1642554793996,174.532927677052));
#31391=CARTESIAN_POINT('Ctrl Pts',(31.4608841227388,34.3680262217031,174.445863980699));
#31392=CARTESIAN_POINT('Ctrl Pts',(33.6969994060995,33.7373506069548,174.33473419148));
#31393=CARTESIAN_POINT('Ctrl Pts',(34.3800392361903,31.5166705575043,174.22360440226));
#31394=CARTESIAN_POINT('Ctrl Pts',(32.8848929677704,29.7383283723363,174.11247461304));
#31395=CARTESIAN_POINT('Ctrl Pts',(30.6193818064991,30.0248505035395,174.003248239133));
#31396=CARTESIAN_POINT('Ctrl Pts',(29.944690779633,31.3552729198763,173.931065128299));
#31397=CARTESIAN_POINT('Ctrl Pts',(29.942062549472,32.0006373960264,173.895925280538));
#31398=CARTESIAN_POINT('Ctrl Pts',(29.9427578740922,31.9987715048219,174.654074719462));
#31399=CARTESIAN_POINT('Ctrl Pts',(29.9470582595646,32.6070099091279,174.620985956712));
#31400=CARTESIAN_POINT('Ctrl Pts',(30.5546327375223,33.9036433503181,174.550853930888));
#31401=CARTESIAN_POINT('Ctrl Pts',(32.7586915732648,34.3070718065724,174.443678641991));
#31402=CARTESIAN_POINT('Ctrl Pts',(34.3497283717851,32.6139786664471,174.332548852772));
#31403=CARTESIAN_POINT('Ctrl Pts',(33.7903192461908,30.3589789091108,174.221419063552));
#31404=CARTESIAN_POINT('Ctrl Pts',(31.5924293616864,29.6058238580236,174.110289274332));
#31405=CARTESIAN_POINT('Ctrl Pts',(30.1290567825581,30.7589286472653,174.021174492969));
#31406=CARTESIAN_POINT('Ctrl Pts',(29.9468392347812,31.7209101982179,173.969102974679));
#31407=CARTESIAN_POINT('Ctrl Pts',(29.9480726635453,31.9989926864899,173.954074719462));
#31408=CARTESIAN_POINT('Origin',(32.,32.,180.545925280538));
#31409=CARTESIAN_POINT('',(29.9443485008314,32.0017900557221,175.354074719462));
#31410=CARTESIAN_POINT('',(29.947375766131,31.998530717209,175.295925280538));
#31411=CARTESIAN_POINT('',(29.94525,32.0000000000002,180.545925280538));
#31412=CARTESIAN_POINT('Ctrl Pts',(29.947375766131,31.998530717209,175.295925280538));
#31413=CARTESIAN_POINT('Ctrl Pts',(29.9503157790678,32.4431897218401,175.271874355438));
#31414=CARTESIAN_POINT('Ctrl Pts',(30.3106831269541,33.5770542377908,175.210780167264));
#31415=CARTESIAN_POINT('Ctrl Pts',(32.1803873389287,34.4219113368872,175.112642716017));
#31416=CARTESIAN_POINT('Ctrl Pts',(34.1325316462971,33.1621113945443,175.001512926798));
#31417=CARTESIAN_POINT('Ctrl Pts',(34.1330061173171,30.8387597064878,174.890383137578));
#31418=CARTESIAN_POINT('Ctrl Pts',(32.1813765212566,29.578162541927,174.779253348358));
#31419=CARTESIAN_POINT('Ctrl Pts',(30.3110383666457,30.4223863748083,174.681100729345));
#31420=CARTESIAN_POINT('Ctrl Pts',(29.9503178487669,31.5565361191587,174.619991373405));
#31421=CARTESIAN_POINT('Ctrl Pts',(29.9473695970144,32.0014721867751,174.595925280538));
#31422=CARTESIAN_POINT('Ctrl Pts',(29.9443485008314,32.0017900557221,175.354074719462));
#31423=CARTESIAN_POINT('Ctrl Pts',(29.9431493621631,32.1329198955122,175.346955464891));
#31424=CARTESIAN_POINT('Ctrl Pts',(30.0143161668846,32.9450545098133,175.302792947247));
#31425=CARTESIAN_POINT('Ctrl Pts',(31.0955884935522,34.2539372331611,175.221587166529));
#31426=CARTESIAN_POINT('Ctrl Pts',(33.4030129919618,33.982359142136,175.11045737731));
#31427=CARTESIAN_POINT('Ctrl Pts',(34.4264152151701,31.8965474620181,174.99932758809));
#31428=CARTESIAN_POINT('Ctrl Pts',(33.2291885468321,29.905414422765,174.88819779887));
#31429=CARTESIAN_POINT('Ctrl Pts',(30.9070218504281,29.8312233889627,174.77706800965));
#31430=CARTESIAN_POINT('Ctrl Pts',(29.9787265765459,31.1729794811598,174.699026983181));
#31431=CARTESIAN_POINT('Ctrl Pts',(29.9422439269294,31.9260797881724,174.658029219785));
#31432=CARTESIAN_POINT('Ctrl Pts',(29.9427578740922,31.9987715048219,174.654074719462));
#31433=CARTESIAN_POINT('Origin',(32.,32.,180.545925280538));
#31434=CARTESIAN_POINT('',(29.9485554566374,32.0000997966407,176.054074719462));
#31435=CARTESIAN_POINT('',(29.9420662255838,31.9993577651234,175.995925280538));
#31436=CARTESIAN_POINT('',(29.94525,32.0000000000002,180.545925280538));
#31437=CARTESIAN_POINT('Ctrl Pts',(29.9420662255838,31.9993577651234,175.995925280538));
#31438=CARTESIAN_POINT('Ctrl Pts',(29.9447109731776,32.6444467488492,175.960800600544));
#31439=CARTESIAN_POINT('Ctrl Pts',(30.6188897830895,33.9746253531368,175.888632657477));
#31440=CARTESIAN_POINT('Ctrl Pts',(32.8839691443584,34.2620328617456,175.779421451336));
#31441=CARTESIAN_POINT('Ctrl Pts',(34.3798416282082,32.4843014974535,175.668291662116));
#31442=CARTESIAN_POINT('Ctrl Pts',(33.6977088622292,30.2633426547257,175.557161872896));
#31443=CARTESIAN_POINT('Ctrl Pts',(31.4618513564243,29.6317537811269,175.446032083677));
#31444=CARTESIAN_POINT('Ctrl Pts',(30.0958007863447,30.8351763931134,175.358953219557));
#31445=CARTESIAN_POINT('Ctrl Pts',(29.9457875676912,31.7583254009107,175.308917618511));
#31446=CARTESIAN_POINT('Ctrl Pts',(29.947375766131,31.998530717209,175.295925280538));
#31447=CARTESIAN_POINT('Ctrl Pts',(29.9485554566374,32.0000997966407,176.054074719462));
#31448=CARTESIAN_POINT('Ctrl Pts',(29.948409504624,32.3369407875857,176.035881709997));
#31449=CARTESIAN_POINT('Ctrl Pts',(30.1862169518775,33.3594384580515,175.980645437459));
#31450=CARTESIAN_POINT('Ctrl Pts',(31.7976939990458,34.4201788169579,175.888365901848));
#31451=CARTESIAN_POINT('Ctrl Pts',(33.9235011844546,33.4826787977943,175.777236112628));
#31452=CARTESIAN_POINT('Ctrl Pts',(34.2889409453366,31.1882472218883,175.666106323408));
#31453=CARTESIAN_POINT('Ctrl Pts',(32.5595667755852,29.6367229854095,175.554976534189));
#31454=CARTESIAN_POINT('Ctrl Pts',(30.4616782545197,30.2088814624134,175.45096599954));
#31455=CARTESIAN_POINT('Ctrl Pts',(29.9493887807299,31.4506185248328,175.383998727964));
#31456=CARTESIAN_POINT('Ctrl Pts',(29.9443485008314,32.0017900557221,175.354074719462));
#31457=CARTESIAN_POINT('Origin',(32.,32.,180.545925280538));
#31458=CARTESIAN_POINT('',(29.9447147371656,31.9981575239013,176.754074719462));
#31459=CARTESIAN_POINT('',(29.9454843589828,32.0018771439066,176.695925280538));
#31460=CARTESIAN_POINT('',(29.94525,32.0000000000002,180.545925280538));
#31461=CARTESIAN_POINT('Ctrl Pts',(29.9454843589828,32.0018771439066,176.695925280538));
#31462=CARTESIAN_POINT('Ctrl Pts',(29.9439531205472,32.1707457963473,176.686770108723));
#31463=CARTESIAN_POINT('Ctrl Pts',(30.0402180779942,33.021161077992,176.640571673835));
#31464=CARTESIAN_POINT('Ctrl Pts',(31.2204530563734,34.3001088403402,176.557329975874));
#31465=CARTESIAN_POINT('Ctrl Pts',(33.5095297542162,33.9025020465923,176.446200186654));
#31466=CARTESIAN_POINT('Ctrl Pts',(34.417101191225,31.7637460111891,176.335070397435));
#31467=CARTESIAN_POINT('Ctrl Pts',(33.112567830368,29.8412070644691,176.223940608215));
#31468=CARTESIAN_POINT('Ctrl Pts',(30.7898244564675,29.8943720011186,176.112810818995));
#31469=CARTESIAN_POINT('Ctrl Pts',(29.95870886397,31.2487009777082,176.036805709769));
#31470=CARTESIAN_POINT('Ctrl Pts',(29.9419217639693,31.9641216630728,175.997843863617));
#31471=CARTESIAN_POINT('Ctrl Pts',(29.9420662255838,31.9993577651234,175.995925280538));
#31472=CARTESIAN_POINT('Ctrl Pts',(29.9447147371656,31.9981575239013,176.754074719462));
#31473=CARTESIAN_POINT('Ctrl Pts',(29.9496923005573,32.53747043377,176.724807955104));
#31474=CARTESIAN_POINT('Ctrl Pts',(30.4434117295339,33.7674633987223,176.658497927671));
#31475=CARTESIAN_POINT('Ctrl Pts',(32.5176555073463,34.3728097273692,176.555144637166));
#31476=CARTESIAN_POINT('Ctrl Pts',(34.2742166391108,32.8521337355438,176.444014847946));
#31477=CARTESIAN_POINT('Ctrl Pts',(33.9494393645001,30.5515941911541,176.332885058726));
#31478=CARTESIAN_POINT('Ctrl Pts',(31.8405563248355,29.5766199351239,176.221755269507));
#31479=CARTESIAN_POINT('Ctrl Pts',(30.1989500491814,30.6160259976346,176.128818489752));
#31480=CARTESIAN_POINT('Ctrl Pts',(29.9487066813412,31.6510900235642,176.072924973071));
#31481=CARTESIAN_POINT('Ctrl Pts',(29.9485554566374,32.0000997966407,176.054074719462));
#31482=CARTESIAN_POINT('Origin',(32.,32.,180.545925280538));
#31483=CARTESIAN_POINT('',(29.9424956572377,32.001054844556,177.454074719462));
#31484=CARTESIAN_POINT('',(29.9484415613596,31.9994876371231,177.395925280538));
#31485=CARTESIAN_POINT('',(29.94525,32.0000000000002,180.545925280538));
#31486=CARTESIAN_POINT('Ctrl Pts',(29.9484415613596,31.9994876371231,177.395925280538));
#31487=CARTESIAN_POINT('Ctrl Pts',(29.9492773107838,32.3739715709387,177.375696353829));
#31488=CARTESIAN_POINT('Ctrl Pts',(30.2266509361282,33.4353642145681,177.318424164048));
#31489=CARTESIAN_POINT('Ctrl Pts',(31.9306130756526,34.4276283682218,177.224108711192));
#31490=CARTESIAN_POINT('Ctrl Pts',(34.0018557168478,33.3750519340786,177.112978921973));
#31491=CARTESIAN_POINT('Ctrl Pts',(34.2410217192136,31.0640428539123,177.001849132753));
#31492=CARTESIAN_POINT('Ctrl Pts',(32.429228945055,29.6096116174522,176.890719343533));
#31493=CARTESIAN_POINT('Ctrl Pts',(30.4062329110444,30.2824327403001,176.788744726128));
#31494=CARTESIAN_POINT('Ctrl Pts',(29.9501487517539,31.4874767060651,176.723813371796));
#31495=CARTESIAN_POINT('Ctrl Pts',(29.9454843589828,32.0018771439066,176.695925280538));
#31496=CARTESIAN_POINT('Ctrl Pts',(29.9424956572377,32.001054844556,177.454074719462));
#31497=CARTESIAN_POINT('Ctrl Pts',(29.9421163386554,32.0616447486548,177.450777463283));
#31498=CARTESIAN_POINT('Ctrl Pts',(29.9720236842432,32.802556573488,177.41043694403));
#31499=CARTESIAN_POINT('Ctrl Pts',(30.8688116111015,34.1490940941566,177.333053161704));
#31500=CARTESIAN_POINT('Ctrl Pts',(33.1919274796751,34.1160109178655,177.221923372484));
#31501=CARTESIAN_POINT('Ctrl Pts',(34.4242044061711,32.1463773227603,177.110793583265));
#31502=CARTESIAN_POINT('Ctrl Pts',(33.4378756702622,30.0427808747097,176.999663794045));
#31503=CARTESIAN_POINT('Ctrl Pts',(31.135618752982,29.7304101029964,176.888534004825));
#31504=CARTESIAN_POINT('Ctrl Pts',(30.0224146087878,31.0303892340693,176.806670979964));
#31505=CARTESIAN_POINT('Ctrl Pts',(29.9433921442462,31.8548561975641,176.761851218177));
#31506=CARTESIAN_POINT('Ctrl Pts',(29.9447147371656,31.9981575239013,176.754074719462));
#31507=CARTESIAN_POINT('Origin',(32.,32.,180.545925280538));
#31508=CARTESIAN_POINT('',(29.94788119656,32.0011671080005,178.154074719462));
#31509=CARTESIAN_POINT('',(29.9436064940107,31.9983925140785,178.095925280538));
#31510=CARTESIAN_POINT('',(29.94525,32.0000000000002,180.545925280538));
#31511=CARTESIAN_POINT('Ctrl Pts',(29.9436064940107,31.9983925140785,178.095925280538));
#31512=CARTESIAN_POINT('Ctrl Pts',(29.9485577871795,32.5744195019018,178.064622598935));
#31513=CARTESIAN_POINT('Ctrl Pts',(30.5011473846441,33.8404367251789,177.99627665426));
#31514=CARTESIAN_POINT('Ctrl Pts',(32.6468975047867,34.3408786212549,177.890887446511));
#31515=CARTESIAN_POINT('Ctrl Pts',(34.3174931090689,32.7262370373898,177.779757657291));
#31516=CARTESIAN_POINT('Ctrl Pts',(33.8671444377423,30.4469492135679,177.668627868071));
#31517=CARTESIAN_POINT('Ctrl Pts',(31.7080052850452,29.5889975993134,177.557498078852));
#31518=CARTESIAN_POINT('Ctrl Pts',(30.1604802454635,30.6920887002321,177.46659721634));
#31519=CARTESIAN_POINT('Ctrl Pts',(29.9477468842698,31.688215619726,177.412739616902));
#31520=CARTESIAN_POINT('Ctrl Pts',(29.9484415613596,31.9994876371231,177.395925280538));
#31521=CARTESIAN_POINT('Ctrl Pts',(29.94788119656,32.0011671080005,178.154074719462));
#31522=CARTESIAN_POINT('Ctrl Pts',(29.9464999255155,32.2670274771179,178.139703708389));
#31523=CARTESIAN_POINT('Ctrl Pts',(30.1180175427899,33.2164703394171,178.088289434242));
#31524=CARTESIAN_POINT('Ctrl Pts',(31.5501292046485,34.3865813061288,177.999831897022));
#31525=CARTESIAN_POINT('Ctrl Pts',(33.7609940320372,33.6724513469602,177.888702107803));
#31526=CARTESIAN_POINT('Ctrl Pts',(34.3602277126424,31.4276996634035,177.777572318583));
#31527=CARTESIAN_POINT('Ctrl Pts',(32.7994009405473,29.7067171266042,177.666442529363));
#31528=CARTESIAN_POINT('Ctrl Pts',(30.5749909099132,30.073309708925,177.558609996323));
#31529=CARTESIAN_POINT('Ctrl Pts',(29.9463778207077,31.3809430879688,177.487820726356));
#31530=CARTESIAN_POINT('Ctrl Pts',(29.9424956572377,32.001054844556,177.454074719462));
#31531=CARTESIAN_POINT('Origin',(32.,32.,180.545925280538));
#31532=CARTESIAN_POINT('',(29.9473399467332,31.997818150837,178.854074719462));
#31533=CARTESIAN_POINT('',(29.943403128554,32.0015021399478,178.795925280538));
#31534=CARTESIAN_POINT('',(29.94525,32.0000000000002,180.545925280538));
#31535=CARTESIAN_POINT('',(31.4698297828098,30.0148256743287,179.));
#31536=CARTESIAN_POINT('Ctrl Pts',(31.4698297828098,30.0148256743287,179.));
#31537=CARTESIAN_POINT('Ctrl Pts',(30.8097602092458,30.191107033931,178.962956736927));
#31538=CARTESIAN_POINT('Ctrl Pts',(30.0751176592089,30.8874016782087,178.914314976748));
#31539=CARTESIAN_POINT('Ctrl Pts',(29.9457279749651,31.7835486120402,178.865673216568));
#31540=CARTESIAN_POINT('Ctrl Pts',(29.9473399467332,31.997818150837,178.854074719462));
#31541=CARTESIAN_POINT('',(32.5313335162366,30.0112662127558,179.));
#31542=CARTESIAN_POINT('Origin',(32.,32.,179.));
#31543=CARTESIAN_POINT('Ctrl Pts',(32.5313343916937,30.0112635340336,179.));
#31544=CARTESIAN_POINT('Ctrl Pts',(31.8868947492701,29.8400087423844,178.963685183163));
#31545=CARTESIAN_POINT('Ctrl Pts',(30.5070458206693,30.1591330867848,178.895660276675));
#31546=CARTESIAN_POINT('Ctrl Pts',(29.9482460569429,31.418251748985,178.827635370188));
#31547=CARTESIAN_POINT('Ctrl Pts',(29.943403128554,32.0015021399478,178.795925280538));
#31548=CARTESIAN_POINT('Origin',(32.,32.,166.));
#31549=CARTESIAN_POINT('Ctrl Pts',(32.6750771856741,30.4769022377462,166.));
#31550=CARTESIAN_POINT('Ctrl Pts',(32.7347503609899,30.4954853005658,166.));
#31551=CARTESIAN_POINT('Ctrl Pts',(32.7931107758957,30.517643791226,166.));
#31552=CARTESIAN_POINT('Ctrl Pts',(32.8500021112569,30.543078531189,166.));
#31553=CARTESIAN_POINT('Ctrl Pts',(32.8860692382174,30.5592032712681,166.));
#31554=CARTESIAN_POINT('Ctrl Pts',(32.9215459750197,30.5766458765615,166.));
#31555=CARTESIAN_POINT('Ctrl Pts',(32.9563915928315,30.595340546146,166.));
#31556=CARTESIAN_POINT('Ctrl Pts',(32.9799636192767,30.6079869353767,166.));
#31557=CARTESIAN_POINT('Ctrl Pts',(33.003246819653,30.6212064489651,166.));
#31558=CARTESIAN_POINT('Ctrl Pts',(33.026228134647,30.6349806231606,166.));
#31559=CARTESIAN_POINT('Ctrl Pts',(33.0386988538539,30.6424551240212,166.));
#31560=CARTESIAN_POINT('Ctrl Pts',(33.0510807692731,30.6500931856874,166.));
#31561=CARTESIAN_POINT('Ctrl Pts',(33.0633592146747,30.6578836587174,166.));
#31562=CARTESIAN_POINT('Ctrl Pts',(33.1190569517964,30.6932229630581,166.));
#31563=CARTESIAN_POINT('Ctrl Pts',(33.1726914481055,30.7317324396433,166.));
#31564=CARTESIAN_POINT('Ctrl Pts',(33.2240811435114,30.7731091649049,166.));
#31565=CARTESIAN_POINT('Ctrl Pts',(33.26116458371,30.8029671219278,166.));
#31566=CARTESIAN_POINT('Ctrl Pts',(33.2970790166423,30.8343193445405,166.));
#31567=CARTESIAN_POINT('Ctrl Pts',(33.3317509313883,30.8670679003715,166.));
#31568=CARTESIAN_POINT('Ctrl Pts',(33.3411297504378,30.8759264471671,166.));
#31569=CARTESIAN_POINT('Ctrl Pts',(33.3504176191284,30.8848872340675,166.));
#31570=CARTESIAN_POINT('Ctrl Pts',(33.3596130010376,30.8939484703997,166.));
#31571=CARTESIAN_POINT('Ctrl Pts',(33.3693213148669,30.9035151558146,166.));
#31572=CARTESIAN_POINT('Ctrl Pts',(33.3789211058175,30.9131885267339,166.));
#31573=CARTESIAN_POINT('Ctrl Pts',(33.3884063294392,30.9229612927792,166.));
#31574=CARTESIAN_POINT('Ctrl Pts',(33.4356623618964,30.971649881246,166.));
#31575=CARTESIAN_POINT('Ctrl Pts',(33.4801121956722,31.0228370852842,166.));
#31576=CARTESIAN_POINT('Ctrl Pts',(33.521572359897,31.076215396252,166.));
#31577=CARTESIAN_POINT('Ctrl Pts',(33.5636369413539,31.1303718703451,166.));
#31578=CARTESIAN_POINT('Ctrl Pts',(33.6026249400945,31.1867843836557,166.));
#31579=CARTESIAN_POINT('Ctrl Pts',(33.6383203879709,31.2451787105165,166.));
#31580=CARTESIAN_POINT('Ctrl Pts',(33.6604356779493,31.2813572024097,166.));
#31581=CARTESIAN_POINT('Ctrl Pts',(33.681286598243,31.3182973027154,166.));
#31582=CARTESIAN_POINT('Ctrl Pts',(33.7008148714994,31.3559410756793,166.));
#31583=CARTESIAN_POINT('Ctrl Pts',(33.7167939181414,31.3867431643266,166.));
#31584=CARTESIAN_POINT('Ctrl Pts',(33.7318873234198,31.4180165031838,166.));
#31585=CARTESIAN_POINT('Ctrl Pts',(33.7460598402509,31.4497315614662,166.));
#31586=CARTESIAN_POINT('Ctrl Pts',(33.7518824450571,31.4627613043825,166.));
#31587=CARTESIAN_POINT('Ctrl Pts',(33.7575504884881,31.4758681482794,166.));
#31588=CARTESIAN_POINT('Ctrl Pts',(33.7630523129776,31.4890274543404,166.));
#31589=CARTESIAN_POINT('Ctrl Pts',(33.7902428497693,31.5540619890274,166.));
#31590=CARTESIAN_POINT('Ctrl Pts',(33.8134282692681,31.6204867128424,166.));
#31591=CARTESIAN_POINT('Ctrl Pts',(33.8323971728471,31.6880059658203,166.));
#31592=CARTESIAN_POINT('Ctrl Pts',(33.8345003075094,31.6954920116385,166.));
#31593=CARTESIAN_POINT('Ctrl Pts',(33.8365515737096,31.7029915509816,166.));
#31594=CARTESIAN_POINT('Ctrl Pts',(33.8385506551699,31.7105042086362,166.));
#31595=CARTESIAN_POINT('Ctrl Pts',(33.8558906957491,31.7756690311676,166.));
#31596=CARTESIAN_POINT('Ctrl Pts',(33.8693083355635,31.841818801265,166.));
#31597=CARTESIAN_POINT('Ctrl Pts',(33.8789575263444,31.9086493575129,166.));
#31598=CARTESIAN_POINT('Ctrl Pts',(33.8893364873223,31.9805343218772,166.));
#31599=CARTESIAN_POINT('Ctrl Pts',(33.8953560454952,32.053207734444,166.));
#31600=CARTESIAN_POINT('Ctrl Pts',(33.8971476570148,32.1263135842633,166.));
#31601=CARTESIAN_POINT('Ctrl Pts',(33.8974689398799,32.139423377666,166.));
#31602=CARTESIAN_POINT('Ctrl Pts',(33.8976541013751,32.1525471118987,166.));
#31603=CARTESIAN_POINT('Ctrl Pts',(33.897703691189,32.1656827687867,166.));
#31604=CARTESIAN_POINT('Ctrl Pts',(33.8977482228948,32.1774786026478,166.));
#31605=CARTESIAN_POINT('Ctrl Pts',(33.8976833755783,32.1892753621347,166.));
#31606=CARTESIAN_POINT('Ctrl Pts',(33.8975100927964,32.2010683060168,166.));
#31607=CARTESIAN_POINT('Ctrl Pts',(33.8964659681176,32.2721273206843,166.));
#31608=CARTESIAN_POINT('Ctrl Pts',(33.8914890591272,32.3430829139215,166.));
#31609=CARTESIAN_POINT('Ctrl Pts',(33.8827593811525,32.4135998306956,166.));
#31610=CARTESIAN_POINT('Ctrl Pts',(33.8738459191009,32.4856013253083,166.));
#31611=CARTESIAN_POINT('Ctrl Pts',(33.8610200659792,32.5571464132172,166.));
#31612=CARTESIAN_POINT('Ctrl Pts',(33.8444207498015,32.6278943811675,166.));
#31613=CARTESIAN_POINT('Ctrl Pts',(33.8277211179619,32.6990699046362,166.));
#31614=CARTESIAN_POINT('Ctrl Pts',(33.8072021977498,32.7694397140702,166.));
#31615=CARTESIAN_POINT('Ctrl Pts',(33.7829530525617,32.838657794496,166.));
#31616=CARTESIAN_POINT('Ctrl Pts',(33.7769688688708,32.8557393742708,166.));
#31617=CARTESIAN_POINT('Ctrl Pts',(33.7707572694931,32.8727507741706,166.));
#31618=CARTESIAN_POINT('Ctrl Pts',(33.7643191147679,32.8896866837861,166.));
#31619=CARTESIAN_POINT('Ctrl Pts',(33.7592567630984,32.9030034700357,166.));
#31620=CARTESIAN_POINT('Ctrl Pts',(33.7540535771897,32.9162751484824,166.));
#31621=CARTESIAN_POINT('Ctrl Pts',(33.7487183848038,32.9294790135144,166.));
#31622=CARTESIAN_POINT('Ctrl Pts',(33.7204961526954,32.9993251440211,166.));
#31623=CARTESIAN_POINT('Ctrl Pts',(33.6885374698854,33.0674004678931,166.));
#31624=CARTESIAN_POINT('Ctrl Pts',(33.6530002833894,33.1333480759195,166.));
#31625=CARTESIAN_POINT('Ctrl Pts',(33.6174247832409,33.1993667839398,166.));
#31626=CARTESIAN_POINT('Ctrl Pts',(33.5782628879173,33.2632543000954,166.));
#31627=CARTESIAN_POINT('Ctrl Pts',(33.5356212918425,33.3246481266484,166.));
#31628=CARTESIAN_POINT('Ctrl Pts',(33.4939489743217,33.3846464210237,166.));
#31629=CARTESIAN_POINT('Ctrl Pts',(33.4489530129887,33.4422640865906,166.));
#31630=CARTESIAN_POINT('Ctrl Pts',(33.4006876508977,33.4971431728771,166.));
#31631=CARTESIAN_POINT('Ctrl Pts',(33.390360214247,33.5088857614027,166.));
#31632=CARTESIAN_POINT('Ctrl Pts',(33.3798829330801,33.5205028633375,166.));
#31633=CARTESIAN_POINT('Ctrl Pts',(33.3692560829687,33.5319907854683,166.));
#31634=CARTESIAN_POINT('Ctrl Pts',(33.3601453871862,33.541839702373,166.));
#31635=CARTESIAN_POINT('Ctrl Pts',(33.3509247547157,33.5515936692396,166.));
#31636=CARTESIAN_POINT('Ctrl Pts',(33.3415960466845,33.5612522690861,166.));
#31637=CARTESIAN_POINT('Ctrl Pts',(32.3836679988478,34.0186125009918,166.));
#31638=CARTESIAN_POINT('Ctrl Pts',(32.3093572659554,34.025632435417,166.));
#31639=CARTESIAN_POINT('Ctrl Pts',(32.2347977339105,34.0282488060548,166.));
#31640=CARTESIAN_POINT('Ctrl Pts',(32.1603115857106,34.0266257027317,166.));
#31641=CARTESIAN_POINT('Ctrl Pts',(32.0877757087159,34.0250450971313,166.));
#31642=CARTESIAN_POINT('Ctrl Pts',(32.0153086399907,34.0194434654372,166.));
#31643=CARTESIAN_POINT('Ctrl Pts',(31.9432211087107,34.0099284747844,166.));
#31644=CARTESIAN_POINT('Ctrl Pts',(31.9271313205272,34.0078047485109,166.));
#31645=CARTESIAN_POINT('Ctrl Pts',(31.9110583935699,34.0054855770819,166.));
#31646=CARTESIAN_POINT('Ctrl Pts',(31.8950127275189,34.0029729711849,166.));
#31647=CARTESIAN_POINT('Ctrl Pts',(31.8213764524233,33.9914421978003,166.));
#31648=CARTESIAN_POINT('Ctrl Pts',(31.7484594020235,33.9758656436188,166.));
#31649=CARTESIAN_POINT('Ctrl Pts',(31.6765936654897,33.9563833455214,166.));
#31650=CARTESIAN_POINT('Ctrl Pts',(31.6261432248504,33.9427065842289,166.));
#31651=CARTESIAN_POINT('Ctrl Pts',(31.5762111638781,33.9271039121742,166.));
#31652=CARTESIAN_POINT('Ctrl Pts',(31.5269203117965,33.9096106347237,166.));
#31653=CARTESIAN_POINT('Ctrl Pts',(31.5081989768218,33.9029664503949,166.));
#31654=CARTESIAN_POINT('Ctrl Pts',(31.489570224729,33.89604942776,166.));
#31655=CARTESIAN_POINT('Ctrl Pts',(31.4710411187568,33.8888611393757,166.));
#31656=CARTESIAN_POINT('Ctrl Pts',(31.453339056705,33.8819936991863,166.));
#31657=CARTESIAN_POINT('Ctrl Pts',(31.4357224678685,33.8748762081473,166.));
#31658=CARTESIAN_POINT('Ctrl Pts',(31.418228472615,33.8675232892194,166.));
#31659=CARTESIAN_POINT('Ctrl Pts',(31.3512969247421,33.839391222296,166.));
#31660=CARTESIAN_POINT('Ctrl Pts',(31.286085531597,33.8077910186021,166.));
#31661=CARTESIAN_POINT('Ctrl Pts',(31.222902662924,33.7728503444856,166.));
#31662=CARTESIAN_POINT('Ctrl Pts',(31.1610752783328,33.7386592648171,166.));
#31663=CARTESIAN_POINT('Ctrl Pts',(31.101189617399,33.7012688782765,166.));
#31664=CARTESIAN_POINT('Ctrl Pts',(31.0435669985648,33.6607619986751,166.));
#31665=CARTESIAN_POINT('Ctrl Pts',(30.9872087184241,33.6211439092098,166.));
#31666=CARTESIAN_POINT('Ctrl Pts',(30.9330146978204,33.5785440615488,166.));
#31667=CARTESIAN_POINT('Ctrl Pts',(30.881326012577,33.533012736002,166.));
#31668=CARTESIAN_POINT('Ctrl Pts',(30.8645070947255,33.518197353865,166.));
#31669=CARTESIAN_POINT('Ctrl Pts',(30.847953796244,33.5030714073101,166.));
#31670=CARTESIAN_POINT('Ctrl Pts',(30.8316789699842,33.4876361269411,166.));
#31671=CARTESIAN_POINT('Ctrl Pts',(30.822544331258,33.4789727035929,166.));
#31672=CARTESIAN_POINT('Ctrl Pts',(30.8134965950441,33.4702108648157,166.));
#31673=CARTESIAN_POINT('Ctrl Pts',(30.8045505016545,33.4613634585313,166.));
#31674=CARTESIAN_POINT('Ctrl Pts',(30.755981374825,33.4133301126647,166.));
#31675=CARTESIAN_POINT('Ctrl Pts',(30.7103172604148,33.362695681989,166.));
#31676=CARTESIAN_POINT('Ctrl Pts',(30.6678506938977,33.3095416270432,166.));
#31677=CARTESIAN_POINT('Ctrl Pts',(30.6617467956725,33.3019015711532,166.));
#31678=CARTESIAN_POINT('Ctrl Pts',(30.6557090297941,33.294209411133,166.));
#31679=CARTESIAN_POINT('Ctrl Pts',(30.6497383407345,33.2864653404541,166.));
#31680=CARTESIAN_POINT('Ctrl Pts',(30.6073793742087,33.231525143873,166.));
#31681=CARTESIAN_POINT('Ctrl Pts',(30.5683924357624,33.1739735703695,166.));
#31682=CARTESIAN_POINT('Ctrl Pts',(30.5328446438884,33.1141723821926,166.));
#31683=CARTESIAN_POINT('Ctrl Pts',(30.4996834403046,33.0583860936178,166.));
#31684=CARTESIAN_POINT('Ctrl Pts',(30.4695154958343,33.0006411409872,166.));
#31685=CARTESIAN_POINT('Ctrl Pts',(30.4424350121092,32.9412257684441,166.));
#31686=CARTESIAN_POINT('Ctrl Pts',(30.4365396641451,32.9282912027578,166.));
#31687=CARTESIAN_POINT('Ctrl Pts',(30.4307907839553,32.9152774801085,166.));
#31688=CARTESIAN_POINT('Ctrl Pts',(30.425189589237,32.9021876017612,166.));
#31689=CARTESIAN_POINT('Ctrl Pts',(30.4206630898284,32.8916092645353,166.));
#31690=CARTESIAN_POINT('Ctrl Pts',(30.4162332674005,32.8809814978217,166.));
#31691=CARTESIAN_POINT('Ctrl Pts',(30.4119057840018,32.8703189087348,166.));
#31692=CARTESIAN_POINT('Ctrl Pts',(30.3861953241676,32.8069702963444,166.));
#31693=CARTESIAN_POINT('Ctrl Pts',(30.3640424511415,32.7422771632775,166.));
#31694=CARTESIAN_POINT('Ctrl Pts',(30.3454933162505,32.6765891288769,166.));
#31695=CARTESIAN_POINT('Ctrl Pts',(30.3270294720946,32.6112031344786,166.));
#31696=CARTESIAN_POINT('Ctrl Pts',(30.312136294192,32.5448302322262,166.));
#31697=CARTESIAN_POINT('Ctrl Pts',(30.3009103653718,32.4778126146351,166.));
#31698=CARTESIAN_POINT('Ctrl Pts',(30.2899244778469,32.4122280183993,166.));
#31699=CARTESIAN_POINT('Ctrl Pts',(30.2824508141855,32.3460250202532,166.));
#31700=CARTESIAN_POINT('Ctrl Pts',(30.2786277887395,32.2795372024809,166.));
#31701=CARTESIAN_POINT('Ctrl Pts',(30.2778239402128,32.2655571400626,166.));
#31702=CARTESIAN_POINT('Ctrl Pts',(30.2771816595994,32.2515645602645,166.));
#31703=CARTESIAN_POINT('Ctrl Pts',(30.2767025029043,32.2375626988325,166.));
#31704=CARTESIAN_POINT('Ctrl Pts',(30.2762461158735,32.2242262098933,166.));
#31705=CARTESIAN_POINT('Ctrl Pts',(30.275937815966,32.2108794399599,166.));
#31706=CARTESIAN_POINT('Ctrl Pts',(30.2757789255977,32.1975468702567,166.));
#31707=CARTESIAN_POINT('Ctrl Pts',(30.2750003283029,32.1322143846253,166.));
#31708=CARTESIAN_POINT('Ctrl Pts',(30.2778000976172,32.0671060893232,166.));
#31709=CARTESIAN_POINT('Ctrl Pts',(30.2842564239881,32.0025315850275,166.));
#31710=CARTESIAN_POINT('Ctrl Pts',(30.2905901747519,31.9391830502096,166.));
#31711=CARTESIAN_POINT('Ctrl Pts',(30.3004431130711,31.8763473623559,166.));
#31712=CARTESIAN_POINT('Ctrl Pts',(30.313935719542,31.8143339857026,166.));
#31713=CARTESIAN_POINT('Ctrl Pts',(30.326990711639,31.7543319287344,166.));
#31714=CARTESIAN_POINT('Ctrl Pts',(30.3434533403295,31.6950990830377,166.));
#31715=CARTESIAN_POINT('Ctrl Pts',(30.3634738587928,31.6369426601543,166.));
#31716=CARTESIAN_POINT('Ctrl Pts',(30.3667806417163,31.6273369815383,166.));
#31717=CARTESIAN_POINT('Ctrl Pts',(30.3701845768421,31.6177607418433,166.));
#31718=CARTESIAN_POINT('Ctrl Pts',(30.3736864471722,31.608215416664,166.));
#31719=CARTESIAN_POINT('Ctrl Pts',(30.3774492972764,31.5979587182547,166.));
#31720=CARTESIAN_POINT('Ctrl Pts',(30.3813252251034,31.5877377137682,166.));
#31721=CARTESIAN_POINT('Ctrl Pts',(30.3853131747227,31.5775537673674,166.));
#31722=CARTESIAN_POINT('Origin',(32.,32.,180.545925280538));
#31723=CARTESIAN_POINT('Ctrl Pts',(29.943403128554,32.0015021399478,178.795925280538));
#31724=CARTESIAN_POINT('Ctrl Pts',(29.9425886188109,32.0995963275832,178.790592107115));
#31725=CARTESIAN_POINT('Ctrl Pts',(29.9935746829529,32.8782050744218,178.748215670618));
#31726=CARTESIAN_POINT('Ctrl Pts',(30.9882484770451,34.2080115613757,178.668795971049));
#31727=CARTESIAN_POINT('Ctrl Pts',(33.3060964076047,34.0474400400451,178.557666181829));
#31728=CARTESIAN_POINT('Ctrl Pts',(34.4285776240291,32.013360755941,178.446536392609));
#31729=CARTESIAN_POINT('Ctrl Pts',(33.3284712910932,29.9669128233058,178.33540660339));
#31730=CARTESIAN_POINT('Ctrl Pts',(31.0125524422092,29.7811934898284,178.22427681417));
#31731=CARTESIAN_POINT('Ctrl Pts',(29.9981273146683,31.1064095349383,178.144449706553));
#31732=CARTESIAN_POINT('Ctrl Pts',(29.9426984790942,31.8927552432854,178.101665862009));
#31733=CARTESIAN_POINT('Ctrl Pts',(29.9436064940107,31.9983925140785,178.095925280538));
#31734=CARTESIAN_POINT('Ctrl Pts',(29.9473399467332,31.997818150837,178.854074719462));
#31735=CARTESIAN_POINT('Ctrl Pts',(29.9508762880376,32.4678823512929,178.828629953495));
#31736=CARTESIAN_POINT('Ctrl Pts',(30.3432698080826,33.6292029591439,178.766141924455));
#31737=CARTESIAN_POINT('Ctrl Pts',(32.2716026719728,34.4129388487757,178.666610632341));
#31738=CARTESIAN_POINT('Ctrl Pts',(34.1744105218922,33.0815150675564,178.555480843121));
#31739=CARTESIAN_POINT('Ctrl Pts',(34.0880401159474,30.7594177996359,178.444351053901));
#31740=CARTESIAN_POINT('Ctrl Pts',(32.0903159869838,29.5731212764253,178.333221264682));
#31741=CARTESIAN_POINT('Ctrl Pts',(30.2791368816166,30.4738805328492,178.236462486535));
#31742=CARTESIAN_POINT('Ctrl Pts',(29.9500603421358,31.5817357085946,178.176746971462));
#31743=CARTESIAN_POINT('Ctrl Pts',(29.94788119656,32.0011671080005,178.154074719462));
#31744=CARTESIAN_POINT('Ctrl Pts',(33.2690708798531,33.0793586530476,179.));
#31745=CARTESIAN_POINT('Ctrl Pts',(33.6279571482411,32.6573931542727,178.962956736927));
#31746=CARTESIAN_POINT('Ctrl Pts',(33.8850554700173,31.4341253615397,178.88887021078));
#31747=CARTESIAN_POINT('Ctrl Pts',(32.5454538370914,30.106758103338,178.777740421561));
#31748=CARTESIAN_POINT('Ctrl Pts',(30.7060860498309,30.5161310027492,178.666610632341));
#31749=CARTESIAN_POINT('Ctrl Pts',(30.0511744117699,32.2815518680592,178.555480843121));
#31750=CARTESIAN_POINT('Ctrl Pts',(31.1796675813394,33.7902651228869,178.444351053901));
#31751=CARTESIAN_POINT('Ctrl Pts',(33.0589884974179,33.6600730535175,178.333221264682));
#31752=CARTESIAN_POINT('Ctrl Pts',(33.9691010203833,32.0108329574877,178.222091475462));
#31753=CARTESIAN_POINT('Ctrl Pts',(33.0771301476877,30.3515643088587,178.110961686242));
#31754=CARTESIAN_POINT('Ctrl Pts',(31.1993733391997,30.2009822869226,177.999831897022));
#31755=CARTESIAN_POINT('Ctrl Pts',(30.0543453491064,31.6968141855763,177.888702107803));
#31756=CARTESIAN_POINT('Ctrl Pts',(30.6899574406665,33.4701319993115,177.777572318583));
#31757=CARTESIAN_POINT('Ctrl Pts',(32.5245072359045,33.8979942976083,177.666442529363));
#31758=CARTESIAN_POINT('Ctrl Pts',(33.8790332253115,32.5888360648699,177.555312740143));
#31759=CARTESIAN_POINT('Ctrl Pts',(33.5138886157823,30.7407798466014,177.444182950924));
#31760=CARTESIAN_POINT('Ctrl Pts',(31.7632494487822,30.0451490451179,177.333053161704));
#31761=CARTESIAN_POINT('Ctrl Pts',(30.2292818746669,31.1385762510273,177.221923372484));
#31762=CARTESIAN_POINT('Ctrl Pts',(30.3158562987823,33.0203693203293,177.110793583265));
#31763=CARTESIAN_POINT('Ctrl Pts',(31.9437407879485,33.9683313597554,176.999663794045));
#31764=CARTESIAN_POINT('Ctrl Pts',(33.6231130912609,33.114897930247,176.888534004825));
#31765=CARTESIAN_POINT('Ctrl Pts',(33.8170298986299,31.2411219830236,176.777404215605));
#31766=CARTESIAN_POINT('Ctrl Pts',(32.3480206460453,30.0618629783066,176.666274426386));
#31767=CARTESIAN_POINT('Ctrl Pts',(30.5605066731107,30.6563659521911,176.555144637166));
#31768=CARTESIAN_POINT('Ctrl Pts',(30.0904013819051,32.4805482381934,176.444014847946));
#31769=CARTESIAN_POINT('Ctrl Pts',(31.3679400374343,33.8649379866196,176.332885058727));
#31770=CARTESIAN_POINT('Ctrl Pts',(33.223933116206,33.5425567147453,176.221755269507));
#31771=CARTESIAN_POINT('Ctrl Pts',(33.9597958800734,31.808444265551,176.110625480287));
#31772=CARTESIAN_POINT('Ctrl Pts',(32.9020747075766,30.2496415473443,175.999495691067));
#31773=CARTESIAN_POINT('Ctrl Pts',(31.0187845453096,30.2927479030848,175.888365901848));
#31774=CARTESIAN_POINT('Ctrl Pts',(30.0334921263313,31.8983128635815,175.777236112628));
#31775=CARTESIAN_POINT('Ctrl Pts',(30.8479263874474,33.596940788559,175.666106323408));
#31776=CARTESIAN_POINT('Ctrl Pts',(32.7167259250522,33.834065821958,175.554976534188));
#31777=CARTESIAN_POINT('Ctrl Pts',(33.929585668619,32.3926737047122,175.443846744969));
#31778=CARTESIAN_POINT('Ctrl Pts',(33.3765095337505,30.5919108712851,175.332716955749));
#31779=CARTESIAN_POINT('Ctrl Pts',(31.563666801218,30.0798159383659,175.22158716653));
#31780=CARTESIAN_POINT('Ctrl Pts',(30.1501514803743,31.3250526351259,175.110457377309));
#31781=CARTESIAN_POINT('Ctrl Pts',(30.4295974639201,33.1879938407189,174.99932758809));
#31782=CARTESIAN_POINT('Ctrl Pts',(32.14625881818,33.963695966543,174.88819779887));
#31783=CARTESIAN_POINT('Ctrl Pts',(33.7290656881523,32.9422448391827,174.777068009651));
#31784=CARTESIAN_POINT('Ctrl Pts',(33.7294503912643,31.0584614532224,174.66593822043));
#31785=CARTESIAN_POINT('Ctrl Pts',(32.1470608513997,30.0363639347125,174.554808431211));
#31786=CARTESIAN_POINT('Ctrl Pts',(30.4300828151426,30.8113648484074,174.443678641991));
#31787=CARTESIAN_POINT('Ctrl Pts',(30.1498759614241,32.6741917626283,174.332548852772));
#31788=CARTESIAN_POINT('Ctrl Pts',(31.5628825640505,33.9200056869971,174.221419063552));
#31789=CARTESIAN_POINT('Ctrl Pts',(33.3759343037167,33.4086512282208,174.110289274332));
#31790=CARTESIAN_POINT('Ctrl Pts',(33.9297458900076,31.6081144415633,173.999159485112));
#31791=CARTESIAN_POINT('Ctrl Pts',(32.7174749649862,30.1662270681651,173.888029695893));
#31792=CARTESIAN_POINT('Ctrl Pts',(30.8485787327015,30.4025887955429,173.776899906673));
#31793=CARTESIAN_POINT('Ctrl Pts',(30.0334507576047,32.1008839340366,173.665770117453));
#31794=CARTESIAN_POINT('Ctrl Pts',(31.0180873228095,33.7068511901408,173.554640328233));
#31795=CARTESIAN_POINT('Ctrl Pts',(32.9013597217795,33.7507267470584,173.443510539014));
#31796=CARTESIAN_POINT('Ctrl Pts',(33.959717478216,32.1923561709092,173.332380749794));
#31797=CARTESIAN_POINT('Ctrl Pts',(33.2245630508403,30.4579433131597,173.221250960574));
#31798=CARTESIAN_POINT('Ctrl Pts',(31.3687017991688,30.134804012298,173.110121171354));
#31799=CARTESIAN_POINT('Ctrl Pts',(30.0905978147541,31.5186718521729,172.998991382135));
#31800=CARTESIAN_POINT('Ctrl Pts',(30.559958003672,33.3430459931528,172.887861592915));
#31801=CARTESIAN_POINT('Ctrl Pts',(32.347229011024,33.9382790059265,172.776731803695));
#31802=CARTESIAN_POINT('Ctrl Pts',(33.8167197930288,32.7596200922368,172.665602014476));
#31803=CARTESIAN_POINT('Ctrl Pts',(33.6235683219593,30.8857651078688,172.554472225256));
#31804=CARTESIAN_POINT('Ctrl Pts',(31.944544729498,30.0316458134051,172.443342436036));
#31805=CARTESIAN_POINT('Ctrl Pts',(30.3162731992128,30.9789429246006,172.332212646816));
#31806=CARTESIAN_POINT('Ctrl Pts',(30.2289301777512,32.8607003982989,172.221082857597));
#31807=CARTESIAN_POINT('Ctrl Pts',(31.7624510511593,33.954754201381,172.109953068377));
#31808=CARTESIAN_POINT('Ctrl Pts',(33.5133741464353,33.259838157786,171.998823279157));
#31809=CARTESIAN_POINT('Ctrl Pts',(33.879273634753,31.411931894561,171.887693489937));
#31810=CARTESIAN_POINT('Ctrl Pts',(32.5252822724187,30.1022191841008,171.776563700718));
#31811=CARTESIAN_POINT('Ctrl Pts',(30.6905582708158,30.5293348957756,171.665433911498));
#31812=CARTESIAN_POINT('Ctrl Pts',(30.0542211394581,32.3023873621376,171.554304122278));
#31813=CARTESIAN_POINT('Ctrl Pts',(31.1986397201752,33.7986981939257,171.443174333059));
#31814=CARTESIAN_POINT('Ctrl Pts',(33.0764545385976,33.6488599447027,171.332044543839));
#31815=CARTESIAN_POINT('Ctrl Pts',(33.9691098369589,31.9900029552293,171.220914754619));
#31816=CARTESIAN_POINT('Ctrl Pts',(33.0596571666423,30.3402951527166,171.109784965399));
#31817=CARTESIAN_POINT('Ctrl Pts',(31.1804177489182,30.2095312276882,170.99865517618));
#31818=CARTESIAN_POINT('Ctrl Pts',(30.0512511193847,31.7173849062541,170.88752538696));
#31819=CARTESIAN_POINT('Ctrl Pts',(30.7055583320888,33.4838848537833,170.77639559774));
#31820=CARTESIAN_POINT('Ctrl Pts',(32.5445245216298,33.8923494751911,170.665265808521));
#31821=CARTESIAN_POINT('Ctrl Pts',(33.8851477740978,32.5689563785795,170.554136019301));
#31822=CARTESIAN_POINT('Ctrl Pts',(33.5005042272877,30.724860574367,170.443006230081));
#31823=CARTESIAN_POINT('Ctrl Pts',(31.7426154839547,30.0477585441825,170.331876440861));
#31824=CARTESIAN_POINT('Ctrl Pts',(30.2202822584875,31.1573267231852,170.220746651642));
#31825=CARTESIAN_POINT('Ctrl Pts',(30.3267274098173,33.0381003467177,170.109616862422));
#31826=CARTESIAN_POINT('Ctrl Pts',(31.9645334897966,33.9688157906636,169.998487073202));
#31827=CARTESIAN_POINT('Ctrl Pts',(33.6347981352959,33.0976923739124,169.887357283982));
#31828=CARTESIAN_POINT('Ctrl Pts',(33.8089132560199,31.2219728005347,169.776227494763));
#31829=CARTESIAN_POINT('Ctrl Pts',(32.3275305816819,30.058295282754,169.665097705543));
#31830=CARTESIAN_POINT('Ctrl Pts',(30.5463954709098,30.671644865286,169.553967916323));
#31831=CARTESIAN_POINT('Ctrl Pts',(30.0955834614767,32.5006906616968,169.442838127103));
#31832=CARTESIAN_POINT('Ctrl Pts',(31.3876728155618,33.8715097942865,169.331708337884));
#31833=CARTESIAN_POINT('Ctrl Pts',(33.240157368435,33.5295434588245,169.220578548664));
#31834=CARTESIAN_POINT('Ctrl Pts',(33.9576633466589,31.7877555370529,169.109448759444));
#31835=CARTESIAN_POINT('Ctrl Pts',(32.883537060004,30.2402114460784,168.998318970225));
#31836=CARTESIAN_POINT('Ctrl Pts',(31.0008072375767,30.303206755534,168.887189181005));
#31837=CARTESIAN_POINT('Ctrl Pts',(30.03252779556,31.9190888413822,168.776059391785));
#31838=CARTESIAN_POINT('Ctrl Pts',(30.8648575786276,33.6090199421243,168.664929602565));
#31839=CARTESIAN_POINT('Ctrl Pts',(32.7360573957742,33.8263934409862,168.553799813346));
#31840=CARTESIAN_POINT('Ctrl Pts',(33.9336254662211,32.3722714689531,168.442670024126));
#31841=CARTESIAN_POINT('Ctrl Pts',(33.3615604798827,30.5774506858874,168.331540234906));
#31842=CARTESIAN_POINT('Ctrl Pts',(31.5434101066319,30.0845316077095,168.220410445687));
#31843=CARTESIAN_POINT('Ctrl Pts',(30.1431258547895,31.3446284307498,168.109280656467));
#31844=CARTESIAN_POINT('Ctrl Pts',(30.4422326785732,33.2045142047563,167.998150867247));
#31845=CARTESIAN_POINT('Ctrl Pts',(32.1669912720462,33.9620416450606,167.887021078027));
#31846=CARTESIAN_POINT('Ctrl Pts',(33.7389212431062,32.9239298409573,167.775891288808));
#31847=CARTESIAN_POINT('Ctrl Pts',(33.7194093934192,31.0402474829195,167.664761499588));
#31848=CARTESIAN_POINT('Ctrl Pts',(32.1263126252782,30.0349201860045,167.553631710368));
#31849=CARTESIAN_POINT('Ctrl Pts',(30.4176160910906,30.8280126945526,167.442501921148));
#31850=CARTESIAN_POINT('Ctrl Pts',(30.1570997860257,32.693695132644,167.331372131929));
#31851=CARTESIAN_POINT('Ctrl Pts',(31.5831865126735,33.9245155987673,167.220242342709));
#31852=CARTESIAN_POINT('Ctrl Pts',(33.3907349133656,33.3940396676622,167.109112553489));
#31853=CARTESIAN_POINT('Ctrl Pts',(33.9255008766017,31.5877549553105,166.997982764269));
#31854=CARTESIAN_POINT('Ctrl Pts',(32.6980630609426,30.1587499839622,166.88685297505));
#31855=CARTESIAN_POINT('Ctrl Pts',(30.8317782439138,30.4148420550124,166.77572318583));
#31856=CARTESIAN_POINT('Ctrl Pts',(30.0346113650038,32.1216433159453,166.66459339661));
#31857=CARTESIAN_POINT('Ctrl Pts',(31.0361996772909,33.7171386430304,166.553463607391));
#31858=CARTESIAN_POINT('Ctrl Pts',(32.9197400310435,33.741085137486,166.442333818171));
#31859=CARTESIAN_POINT('Ctrl Pts',(33.961763295132,32.1716952567886,166.331204028951));
#31860=CARTESIAN_POINT('Ctrl Pts',(33.2079561086236,30.4449968915186,166.220074239731));
#31861=CARTESIAN_POINT('Ctrl Pts',(31.3495488314203,30.1417767118191,166.108944450512));
#31862=CARTESIAN_POINT('Ctrl Pts',(30.0845739128819,31.5384507908558,165.997814661292));
#31863=CARTESIAN_POINT('Ctrl Pts',(30.5763936504527,33.3590412771596,165.886684872072));
#31864=CARTESIAN_POINT('Ctrl Pts',(31.7668777668633,33.7401334029928,165.812598345926));
#31865=CARTESIAN_POINT('Ctrl Pts',(32.3110796379513,33.6366995627946,165.775555082853));
#31866=CARTESIAN_POINT('Ctrl Pts',(33.3677806246596,33.1633123698088,179.074814972382));
#31867=CARTESIAN_POINT('Ctrl Pts',(33.754581466244,32.7085259251257,179.037771709309));
#31868=CARTESIAN_POINT('Ctrl Pts',(34.0316771814958,31.3901110026558,178.963685183163));
#31869=CARTESIAN_POINT('Ctrl Pts',(32.5878798433277,29.9594996424882,178.852555393943));
#31870=CARTESIAN_POINT('Ctrl Pts',(30.6054439833786,30.4007140214203,178.741425604723));
#31871=CARTESIAN_POINT('Ctrl Pts',(29.8995925895562,32.3034512855678,178.630295815504));
#31872=CARTESIAN_POINT('Ctrl Pts',(31.1158612132413,33.9295139357165,178.519166026284));
#31873=CARTESIAN_POINT('Ctrl Pts',(33.1413578008135,33.7891953823601,178.408036237064));
#31874=CARTESIAN_POINT('Ctrl Pts',(34.1222598882652,32.0116755569721,178.296906447844));
#31875=CARTESIAN_POINT('Ctrl Pts',(33.1609105288229,30.2233471470077,178.185776658625));
#31876=CARTESIAN_POINT('Ctrl Pts',(31.1370997068695,30.0610526878912,178.074646869405));
#31877=CARTESIAN_POINT('Ctrl Pts',(29.9030101659262,31.6732320556528,177.963517080185));
#31878=CARTESIAN_POINT('Ctrl Pts',(30.5880608730512,33.5844805016589,177.852387290966));
#31879=CARTESIAN_POINT('Ctrl Pts',(32.5653039921985,34.0456224054905,177.741257501746));
#31880=CARTESIAN_POINT('Ctrl Pts',(34.0251865198973,32.6346363890432,177.630127712526));
#31881=CARTESIAN_POINT('Ctrl Pts',(33.6316405564356,30.6428363022569,177.518997923306));
#31882=CARTESIAN_POINT('Ctrl Pts',(31.7448347275366,29.8930985631831,177.407868134087));
#31883=CARTESIAN_POINT('Ctrl Pts',(30.091553449052,31.0715737535457,177.296738344867));
#31884=CARTESIAN_POINT('Ctrl Pts',(30.1848617281844,33.0997347811692,177.185608555647));
#31885=CARTESIAN_POINT('Ctrl Pts',(31.9393648838499,34.1214303625775,177.074478766427));
#31886=CARTESIAN_POINT('Ctrl Pts',(33.7493606331233,33.2016159315242,176.963348977208));
#31887=CARTESIAN_POINT('Ctrl Pts',(33.9583605054912,31.1820956066532,176.852219187988));
#31888=CARTESIAN_POINT('Ctrl Pts',(32.3750900790485,29.9111125246884,176.741089398768));
#31889=CARTESIAN_POINT('Ctrl Pts',(30.4485412807881,30.5518566012337,176.629959609548));
#31890=CARTESIAN_POINT('Ctrl Pts',(29.9418706770663,32.5179258147436,176.518829820329));
#31891=CARTESIAN_POINT('Ctrl Pts',(31.318777710414,34.0099949378598,176.407700031109));
#31892=CARTESIAN_POINT('Ctrl Pts',(33.3191319955427,33.6625384920277,176.29657024189));
#31893=CARTESIAN_POINT('Ctrl Pts',(34.1122309837906,31.7935448474304,176.18544045267));
#31894=CARTESIAN_POINT('Ctrl Pts',(32.9722390818404,30.1134967197192,176.07431066345));
#31895=CARTESIAN_POINT('Ctrl Pts',(30.9424645156955,30.1599559357627,175.96318087423));
#31896=CARTESIAN_POINT('Ctrl Pts',(29.8805349562855,31.8904035249895,175.85205108501));
#31897=CARTESIAN_POINT('Ctrl Pts',(30.7583168202445,33.7211526196019,175.740921295791));
#31898=CARTESIAN_POINT('Ctrl Pts',(32.772473664821,33.9767215018872,175.629791506571));
#31899=CARTESIAN_POINT('Ctrl Pts',(34.079670988482,32.4232163022927,175.518661717351));
#31900=CARTESIAN_POINT('Ctrl Pts',(33.4835759765767,30.4823881324319,175.407531928132));
#31901=CARTESIAN_POINT('Ctrl Pts',(31.5297283196201,29.9304618859529,175.296402138912));
#31902=CARTESIAN_POINT('Ctrl Pts',(30.0062682046631,31.2725544782441,175.185272349692));
#31903=CARTESIAN_POINT('Ctrl Pts',(30.3074498076774,33.2803973232278,175.074142560472));
#31904=CARTESIAN_POINT('Ctrl Pts',(32.1576349917629,34.1164344233243,174.963012771253));
#31905=CARTESIAN_POINT('Ctrl Pts',(33.8635543408672,33.01553369097,174.851882982033));
#31906=CARTESIAN_POINT('Ctrl Pts',(33.8639689666152,30.9852275376442,174.740753192813));
#31907=CARTESIAN_POINT('Ctrl Pts',(32.1584994080186,29.8836301371174,174.629623403593));
#31908=CARTESIAN_POINT('Ctrl Pts',(30.307972910058,30.7189114840252,174.518493614374));
#31909=CARTESIAN_POINT('Ctrl Pts',(30.0059712555425,32.7266311479268,174.407363825154));
#31910=CARTESIAN_POINT('Ctrl Pts',(31.5288830836133,34.0693458652324,174.296234035934));
#31911=CARTESIAN_POINT('Ctrl Pts',(33.482956004511,33.5182176877988,174.185104246715));
#31912=CARTESIAN_POINT('Ctrl Pts',(34.0798436720685,31.5776331468769,174.073974457495));
#31913=CARTESIAN_POINT('Ctrl Pts',(32.7732809659143,30.0235941695556,173.962844668275));
#31914=CARTESIAN_POINT('Ctrl Pts',(30.7590199056383,30.2783403750282,173.851714879056));
#31915=CARTESIAN_POINT('Ctrl Pts',(29.8804903698533,32.1087307986539,173.740585089835));
#31916=CARTESIAN_POINT('Ctrl Pts',(30.9417130624539,33.839611974488,173.629455300616));
#31917=CARTESIAN_POINT('Ctrl Pts',(32.9714684836526,33.8869002210318,173.518325511396));
#31918=CARTESIAN_POINT('Ctrl Pts',(34.1121464837495,32.2073178478682,173.407195722176));
#31919=CARTESIAN_POINT('Ctrl Pts',(33.3198109271937,30.338000428604,173.296065932957));
#31920=CARTESIAN_POINT('Ctrl Pts',(31.3195987228237,29.9897269934467,173.184936143737));
#31921=CARTESIAN_POINT('Ctrl Pts',(29.9420823886808,31.4812336133839,173.073806354517));
#31922=CARTESIAN_POINT('Ctrl Pts',(30.4479499352301,33.447509604565,172.962676565297));
#31923=CARTESIAN_POINT('Ctrl Pts',(32.3742368697747,34.0890405032362,172.851546776078));
#31924=CARTESIAN_POINT('Ctrl Pts',(33.9580262795313,32.8187041880466,172.740416986858));
#31925=CARTESIAN_POINT('Ctrl Pts',(33.7498512721717,30.7990986784339,172.629287197638));
#31926=CARTESIAN_POINT('Ctrl Pts',(31.9402313568674,29.878545035086,172.518157408419));
#31927=CARTESIAN_POINT('Ctrl Pts',(30.1853110555941,30.8995239694063,172.407027619199));
#31928=CARTESIAN_POINT('Ctrl Pts',(30.091174396759,32.9276466327604,172.295897829979));
#31929=CARTESIAN_POINT('Ctrl Pts',(31.7439742296583,34.106797157721,172.184768040759));
#31930=CARTESIAN_POINT('Ctrl Pts',(33.6310860710905,33.3578297711992,172.07363825154));
#31931=CARTESIAN_POINT('Ctrl Pts',(34.0254456286525,31.3661913031266,171.96250846232));
#31932=CARTESIAN_POINT('Ctrl Pts',(32.566139311915,29.9546076810635,171.8513786731));
#31933=CARTESIAN_POINT('Ctrl Pts',(30.588708436438,30.414944927935,171.74024888388));
#31934=CARTESIAN_POINT('Ctrl Pts',(29.9028762951132,32.325907387554,171.629119094661));
#31935=CARTESIAN_POINT('Ctrl Pts',(31.1363090261413,33.938602940402,171.517989305441));
#31936=CARTESIAN_POINT('Ctrl Pts',(33.1601823701062,33.7771101054676,171.406859516221));
#31937=CARTESIAN_POINT('Ctrl Pts',(34.1222693906039,31.9892253739659,171.295729727002));
#31938=CARTESIAN_POINT('Ctrl Pts',(33.142078479874,30.2112014633646,171.184599937782));
#31939=CARTESIAN_POINT('Ctrl Pts',(31.1166697296889,30.0702665747797,171.073470148562));
#31940=CARTESIAN_POINT('Ctrl Pts',(29.8996752635746,31.6954027898688,170.962340359342));
#31941=CARTESIAN_POINT('Ctrl Pts',(30.6048752191635,33.5993030684508,170.851210570123));
#31942=CARTESIAN_POINT('Ctrl Pts',(32.5868782446758,34.0395385225061,170.740080780903));
#31943=CARTESIAN_POINT('Ctrl Pts',(34.0317766650903,32.6132104386381,170.628950991683));
#31944=CARTESIAN_POINT('Ctrl Pts',(33.6172151153146,30.6256788113188,170.517821202463));
#31945=CARTESIAN_POINT('Ctrl Pts',(31.7225958299706,29.8959110319878,170.406691413244));
#31946=CARTESIAN_POINT('Ctrl Pts',(30.0818538327146,31.0917826582869,170.295561624024));
#31947=CARTESIAN_POINT('Ctrl Pts',(30.1965784063291,33.1188449465149,170.184431834804));
#31948=CARTESIAN_POINT('Ctrl Pts',(31.9617748651785,34.1219524730606,170.073302045585));
#31949=CARTESIAN_POINT('Ctrl Pts',(33.7619545528822,33.1830721078777,169.962172256365));
#31950=CARTESIAN_POINT('Ctrl Pts',(33.9496125413895,31.1614569794478,169.851042467145));
#31951=CARTESIAN_POINT('Ctrl Pts',(32.3530062746849,29.907267329807,169.739912677925));
#31952=CARTESIAN_POINT('Ctrl Pts',(30.433332493582,30.5683239251859,169.628782888706));
#31953=CARTESIAN_POINT('Ctrl Pts',(29.9474558245518,32.5396349383544,169.517653099486));
#31954=CARTESIAN_POINT('Ctrl Pts',(31.3400453259759,34.0170779080377,169.406523310266));
#31955=CARTESIAN_POINT('Ctrl Pts',(33.3366181881587,33.6485130505849,169.295393521047));
#31956=CARTESIAN_POINT('Ctrl Pts',(34.1099325795548,31.7712469266146,169.184263731827));
#31957=CARTESIAN_POINT('Ctrl Pts',(32.9522595554175,30.1033331346864,169.073133942607));
#31958=CARTESIAN_POINT('Ctrl Pts',(30.9230889129684,30.1712282893903,168.962004153387));
#31959=CARTESIAN_POINT('Ctrl Pts',(29.8794956187941,31.9127954814557,168.850874364168));
#31960=CARTESIAN_POINT('Ctrl Pts',(30.7765649383097,33.7341713031689,168.739744574948));
#31961=CARTESIAN_POINT('Ctrl Pts',(32.7933087588409,33.9684523545883,168.628614785728));
#31962=CARTESIAN_POINT('Ctrl Pts',(34.0840250060357,32.4012271579398,168.517484996508));
#31963=CARTESIAN_POINT('Ctrl Pts',(33.4674641686691,30.4668032177279,168.406355207289));
#31964=CARTESIAN_POINT('Ctrl Pts',(31.5078960367946,29.9355443453039,168.295225418069));
#31965=CARTESIAN_POINT('Ctrl Pts',(29.9986961181047,31.2936529010287,168.184095628849));
#31966=CARTESIAN_POINT('Ctrl Pts',(30.3210678033822,33.298202659558,168.07296583963));
#31967=CARTESIAN_POINT('Ctrl Pts',(32.1799800389545,34.1146514268768,167.96183605041));
#31968=CARTESIAN_POINT('Ctrl Pts',(33.8741764718491,32.9957941318081,167.85070626119));
#31969=CARTESIAN_POINT('Ctrl Pts',(33.8531469687877,30.9655968644692,167.73957647197));
#31970=CARTESIAN_POINT('Ctrl Pts',(32.1361373617882,29.8820740920287,167.628446682751));
#31971=CARTESIAN_POINT('Ctrl Pts',(30.2945365103406,30.7368542181635,167.517316893531));
#31972=CARTESIAN_POINT('Ctrl Pts',(30.0137569572577,32.7476515117587,167.406187104311));
#31973=CARTESIAN_POINT('Ctrl Pts',(31.5507662959473,34.0742065629572,167.295057315091));
#31974=CARTESIAN_POINT('Ctrl Pts',(33.4989078220432,33.5024696238054,167.183927525872));
#31975=CARTESIAN_POINT('Ctrl Pts',(34.0752684767976,31.5556900771347,167.072797736652));
#31976=CARTESIAN_POINT('Ctrl Pts',(32.7523591823794,30.0155355094255,166.961667947433));
#31977=CARTESIAN_POINT('Ctrl Pts',(30.740912656143,30.2915467066502,166.850538158212));
#31978=CARTESIAN_POINT('Ctrl Pts',(29.8817412505871,32.1311048683811,166.739408368993));
#31979=CARTESIAN_POINT('Ctrl Pts',(30.9612342160158,33.8506995969076,166.628278579773));
#31980=CARTESIAN_POINT('Ctrl Pts',(32.9912784338182,33.8765086763411,166.517148790554));
#31981=CARTESIAN_POINT('Ctrl Pts',(34.1143514265811,32.1850499048632,166.406019001334));
#31982=CARTESIAN_POINT('Ctrl Pts',(33.3019122785371,30.3240470198856,166.294889212114));
#31983=CARTESIAN_POINT('Ctrl Pts',(31.298956015937,29.9972420372932,166.183759422894));
#31984=CARTESIAN_POINT('Ctrl Pts',(29.9355899410197,31.5025509799206,166.072629633675));
#31985=CARTESIAN_POINT('Ctrl Pts',(30.4656639649012,33.4647490195557,165.961499844455));
#31986=CARTESIAN_POINT('Ctrl Pts',(31.7487452602343,33.8754829148802,165.887413318308));
#31987=CARTESIAN_POINT('Ctrl Pts',(32.3352757582502,33.764003875527,165.850370055235));
#31988=CARTESIAN_POINT('Ctrl Pts',(33.4664903694662,33.2472660865699,179.149629944765));
#31989=CARTESIAN_POINT('Ctrl Pts',(33.881205784247,32.7596586959787,179.112586681692));
#31990=CARTESIAN_POINT('Ctrl Pts',(34.1782988929742,31.3460966437719,179.038500155545));
#31991=CARTESIAN_POINT('Ctrl Pts',(32.6303058495641,29.8122411816384,178.927370366326));
#31992=CARTESIAN_POINT('Ctrl Pts',(30.5048019169264,30.2852970400916,178.816240577106));
#31993=CARTESIAN_POINT('Ctrl Pts',(29.7480107673423,32.3253507030764,178.705110787886));
#31994=CARTESIAN_POINT('Ctrl Pts',(31.0520548451432,34.0687627485461,178.593980998666));
#31995=CARTESIAN_POINT('Ctrl Pts',(33.2237271042091,33.9183177112026,178.482851209447));
#31996=CARTESIAN_POINT('Ctrl Pts',(34.2754187561472,32.0125181564566,178.371721420227));
#31997=CARTESIAN_POINT('Ctrl Pts',(33.244690909958,30.0951299851567,178.260591631007));
#31998=CARTESIAN_POINT('Ctrl Pts',(31.0748260745393,29.9211230888598,178.149461841787));
#31999=CARTESIAN_POINT('Ctrl Pts',(29.7516749827459,31.6496499257294,178.038332052568));
#32000=CARTESIAN_POINT('Ctrl Pts',(30.486164305436,33.6988290040063,177.927202263348));
#32001=CARTESIAN_POINT('Ctrl Pts',(32.6061007484926,34.1932505133727,177.816072474128));
#32002=CARTESIAN_POINT('Ctrl Pts',(34.1713398144831,32.6804367132165,177.704942684908));
#32003=CARTESIAN_POINT('Ctrl Pts',(33.7493924970889,30.5448927579124,177.593812895689));
#32004=CARTESIAN_POINT('Ctrl Pts',(31.7264200062909,29.7410480812482,177.482683106469));
#32005=CARTESIAN_POINT('Ctrl Pts',(29.9538250234371,31.0045712560641,177.371553317249));
#32006=CARTESIAN_POINT('Ctrl Pts',(30.0538671575865,33.1791002420091,177.26042352803));
#32007=CARTESIAN_POINT('Ctrl Pts',(31.9349889797512,34.2745293653997,177.14929373881));
#32008=CARTESIAN_POINT('Ctrl Pts',(33.8756081749856,33.2883339328014,177.03816394959));
#32009=CARTESIAN_POINT('Ctrl Pts',(34.0996911123523,31.1230692302828,176.92703416037));
#32010=CARTESIAN_POINT('Ctrl Pts',(32.4021595120518,29.7603620710703,176.815904371151));
#32011=CARTESIAN_POINT('Ctrl Pts',(30.3365758884656,30.4473472502762,176.704774581931));
#32012=CARTESIAN_POINT('Ctrl Pts',(29.7933399722275,32.5553033912937,176.593644792711));
#32013=CARTESIAN_POINT('Ctrl Pts',(31.2696153833937,34.1550518891,176.482515003491));
#32014=CARTESIAN_POINT('Ctrl Pts',(33.4143308748795,33.78252026931,176.371385214272));
#32015=CARTESIAN_POINT('Ctrl Pts',(34.2646660875078,31.7786454293097,176.260255425052));
#32016=CARTESIAN_POINT('Ctrl Pts',(33.0424034561043,29.9773518920942,176.149125635832));
#32017=CARTESIAN_POINT('Ctrl Pts',(30.8661444860815,30.0271639684406,176.037995846613));
#32018=CARTESIAN_POINT('Ctrl Pts',(29.7275777862398,31.8824941863976,175.926866057393));
#32019=CARTESIAN_POINT('Ctrl Pts',(30.6687072530417,33.8453644506448,175.815736268173));
#32020=CARTESIAN_POINT('Ctrl Pts',(32.8282214045897,34.1193771818164,175.704606478953));
#32021=CARTESIAN_POINT('Ctrl Pts',(34.2297563083451,32.4537588998731,175.593476689734));
#32022=CARTESIAN_POINT('Ctrl Pts',(33.590642419403,30.3728653935788,175.482346900514));
#32023=CARTESIAN_POINT('Ctrl Pts',(31.4957898380222,29.7811078335399,175.371217111294));
#32024=CARTESIAN_POINT('Ctrl Pts',(29.8623849289518,31.2200563213624,175.260087322075));
#32025=CARTESIAN_POINT('Ctrl Pts',(30.1853021514348,33.3728008057367,175.148957532855));
#32026=CARTESIAN_POINT('Ctrl Pts',(32.1690111653458,34.2691728801058,175.037827743635));
#32027=CARTESIAN_POINT('Ctrl Pts',(33.9980429935822,33.0888225427571,174.926697954415));
#32028=CARTESIAN_POINT('Ctrl Pts',(33.9984875419661,30.911993622066,174.815568165196));
#32029=CARTESIAN_POINT('Ctrl Pts',(32.1699379646376,29.7308963395222,174.704438375976));
#32030=CARTESIAN_POINT('Ctrl Pts',(30.1858630049732,30.6264581196432,174.593308586756));
#32031=CARTESIAN_POINT('Ctrl Pts',(29.8620665496609,32.7790705332252,174.482178797537));
#32032=CARTESIAN_POINT('Ctrl Pts',(31.494883603176,34.2186860434678,174.371049008317));
#32033=CARTESIAN_POINT('Ctrl Pts',(33.5899777053053,33.6277841473768,174.259919219097));
#32034=CARTESIAN_POINT('Ctrl Pts',(34.2299414541294,31.5471518521906,174.148789429877));
#32035=CARTESIAN_POINT('Ctrl Pts',(32.8290869668423,29.8809612709459,174.037659640658));
#32036=CARTESIAN_POINT('Ctrl Pts',(30.669461078575,30.1540919545135,173.926529851438));
#32037=CARTESIAN_POINT('Ctrl Pts',(29.727529982102,32.116577663271,173.815400062218));
#32038=CARTESIAN_POINT('Ctrl Pts',(30.8653388020982,33.9723727588352,173.704270272998));
#32039=CARTESIAN_POINT('Ctrl Pts',(33.0415772455258,34.0230736950052,173.593140483779));
#32040=CARTESIAN_POINT('Ctrl Pts',(34.2645754892831,32.2222795248272,173.482010694559));
#32041=CARTESIAN_POINT('Ctrl Pts',(33.4150588035471,30.2180575440483,173.370880905339));
#32042=CARTESIAN_POINT('Ctrl Pts',(31.2704956464786,29.8446499745953,173.259751116119));
#32043=CARTESIAN_POINT('Ctrl Pts',(29.7935669626075,31.4437953745948,173.1486213269));
#32044=CARTESIAN_POINT('Ctrl Pts',(30.3359418667882,33.5519732159772,173.03749153768));
#32045=CARTESIAN_POINT('Ctrl Pts',(32.4012447285253,34.239802000546,172.92636174846));
#32046=CARTESIAN_POINT('Ctrl Pts',(34.0993327660339,32.8777882838563,172.81523195924));
#32047=CARTESIAN_POINT('Ctrl Pts',(33.8761342223841,30.7124322489989,172.704102170021));
#32048=CARTESIAN_POINT('Ctrl Pts',(31.9359179842369,29.7254442567669,172.592972380801));
#32049=CARTESIAN_POINT('Ctrl Pts',(30.0543489119754,30.8201050142119,172.481842591581));
#32050=CARTESIAN_POINT('Ctrl Pts',(29.9534186157667,32.9945928672219,172.370712802362));
#32051=CARTESIAN_POINT('Ctrl Pts',(31.7254974081573,34.2588401140609,172.259583013142));
#32052=CARTESIAN_POINT('Ctrl Pts',(33.7487979957457,33.4558213846124,172.148453223922));
#32053=CARTESIAN_POINT('Ctrl Pts',(34.1716176225522,31.3204507116921,172.037323434703));
#32054=CARTESIAN_POINT('Ctrl Pts',(32.6069963514114,29.8069961780261,171.926193645483));
#32055=CARTESIAN_POINT('Ctrl Pts',(30.4868586020602,30.3005549600944,171.815063856263));
#32056=CARTESIAN_POINT('Ctrl Pts',(29.7515314507684,32.3494274129703,171.703934067043));
#32057=CARTESIAN_POINT('Ctrl Pts',(31.0739783321073,34.0785076868783,171.592804277824));
#32058=CARTESIAN_POINT('Ctrl Pts',(33.2439102016148,33.9053602662325,171.481674488604));
#32059=CARTESIAN_POINT('Ctrl Pts',(34.2754289442489,31.9884477927025,171.370544699384));
#32060=CARTESIAN_POINT('Ctrl Pts',(33.2244997931058,30.0821077740126,171.259414910164));
#32061=CARTESIAN_POINT('Ctrl Pts',(31.0529217104596,29.9310019218713,171.148285120945));
#32062=CARTESIAN_POINT('Ctrl Pts',(29.7480994077644,31.6734206734835,171.037155331725));
#32063=CARTESIAN_POINT('Ctrl Pts',(30.5041921062382,33.7147212831184,170.926025542505));
#32064=CARTESIAN_POINT('Ctrl Pts',(32.6292319677217,34.1867275698212,170.814895753286));
#32065=CARTESIAN_POINT('Ctrl Pts',(34.1784055560829,32.6574644986967,170.703765964066));
#32066=CARTESIAN_POINT('Ctrl Pts',(33.7339260033414,30.5264970482706,170.592636174846));
#32067=CARTESIAN_POINT('Ctrl Pts',(31.7025761759865,29.7440635197931,170.481506385626));
#32068=CARTESIAN_POINT('Ctrl Pts',(29.9434254069416,31.0262385933886,170.370376596407));
#32069=CARTESIAN_POINT('Ctrl Pts',(30.0664294028411,33.1995895463121,170.259246807187));
#32070=CARTESIAN_POINT('Ctrl Pts',(31.9590162405603,34.2750891554577,170.148117017967));
#32071=CARTESIAN_POINT('Ctrl Pts',(33.8891109704685,33.2684518418429,170.036987228747));
#32072=CARTESIAN_POINT('Ctrl Pts',(34.0903118267592,31.1009411583609,169.925857439528));
#32073=CARTESIAN_POINT('Ctrl Pts',(32.3784819676879,29.7562393768599,169.814727650308));
#32074=CARTESIAN_POINT('Ctrl Pts',(30.3202695162544,30.4650029850859,169.703597861088));
#32075=CARTESIAN_POINT('Ctrl Pts',(29.7993281876268,32.578579215012,169.592468071868));
#32076=CARTESIAN_POINT('Ctrl Pts',(31.29241783639,34.162646021789,169.481338282649));
#32077=CARTESIAN_POINT('Ctrl Pts',(33.4330790078824,33.7674826423452,169.370208493429));
#32078=CARTESIAN_POINT('Ctrl Pts',(34.2622018124507,31.7547383161762,169.259078704209));
#32079=CARTESIAN_POINT('Ctrl Pts',(33.020982050831,29.9664548232945,169.14794891499));
#32080=CARTESIAN_POINT('Ctrl Pts',(30.8453705883601,30.0392498232466,169.03681912577));
#32081=CARTESIAN_POINT('Ctrl Pts',(29.7264634420282,31.9065021215292,168.92568933655));
#32082=CARTESIAN_POINT('Ctrl Pts',(30.6882722979918,33.8593226642135,168.81455954733));
#32083=CARTESIAN_POINT('Ctrl Pts',(32.8505601219075,34.1105112681904,168.703429758111));
#32084=CARTESIAN_POINT('Ctrl Pts',(34.2344245458504,32.4301828469265,168.592299968891));
#32085=CARTESIAN_POINT('Ctrl Pts',(33.5733678574555,30.3561557495683,168.481170179671));
#32086=CARTESIAN_POINT('Ctrl Pts',(31.4723819669573,29.7865570828984,168.370040390452));
#32087=CARTESIAN_POINT('Ctrl Pts',(29.8542663814199,31.2426773713076,168.258910601232));
#32088=CARTESIAN_POINT('Ctrl Pts',(30.1999029281912,33.3918911143597,168.147780812012));
#32089=CARTESIAN_POINT('Ctrl Pts',(32.1929688058628,34.267261208693,168.036651022792));
#32090=CARTESIAN_POINT('Ctrl Pts',(34.0094317005922,33.0676584226589,167.925521233573));
#32091=CARTESIAN_POINT('Ctrl Pts',(33.9868845441562,30.8909462460187,167.814391444353));
#32092=CARTESIAN_POINT('Ctrl Pts',(32.1459620982981,29.729227998053,167.703261655133));
#32093=CARTESIAN_POINT('Ctrl Pts',(30.1714569295906,30.6456957417745,167.592131865913));
#32094=CARTESIAN_POINT('Ctrl Pts',(29.8704141284897,32.8016078908734,167.481002076694));
#32095=CARTESIAN_POINT('Ctrl Pts',(31.5183460792209,34.2238975271471,167.369872287474));
#32096=CARTESIAN_POINT('Ctrl Pts',(33.6070807307209,33.6108995799486,167.258742498254));
#32097=CARTESIAN_POINT('Ctrl Pts',(34.2250360769934,31.5236251989588,167.147612709034));
#32098=CARTESIAN_POINT('Ctrl Pts',(32.8066553038163,29.8723210348887,167.036482919815));
#32099=CARTESIAN_POINT('Ctrl Pts',(30.6500470683722,30.1682513582881,166.925353130595));
#32100=CARTESIAN_POINT('Ctrl Pts',(29.7288711361704,32.1405664208168,166.814223341375));
#32101=CARTESIAN_POINT('Ctrl Pts',(30.8862687547407,33.9842605507847,166.703093552155));
#32102=CARTESIAN_POINT('Ctrl Pts',(33.0628168365929,34.0119322151961,166.591963762936));
#32103=CARTESIAN_POINT('Ctrl Pts',(34.2669395580302,32.1984045529377,166.480833973716));
#32104=CARTESIAN_POINT('Ctrl Pts',(33.3958684484506,30.2030971482525,166.369704184496));
#32105=CARTESIAN_POINT('Ctrl Pts',(31.2483632004537,29.8527073627674,166.258574395277));
#32106=CARTESIAN_POINT('Ctrl Pts',(29.7866059691575,31.4666511689852,166.147444606057));
#32107=CARTESIAN_POINT('Ctrl Pts',(30.3549342793497,33.5704567619518,166.036314816837));
#32108=CARTESIAN_POINT('Ctrl Pts',(31.7306127536053,34.0108324267677,165.962228290691));
#32109=CARTESIAN_POINT('Ctrl Pts',(32.359471878549,33.8913081882594,165.925185027618));
#32110=CARTESIAN_POINT('Ctrl Pts',(33.5652001142727,33.3312198033311,179.224444917147));
#32111=CARTESIAN_POINT('Ctrl Pts',(34.0078301022499,32.8107914668318,179.187401654074));
#32112=CARTESIAN_POINT('Ctrl Pts',(34.3249206044526,31.3020822848881,179.113315127928));
#32113=CARTESIAN_POINT('Ctrl Pts',(32.6727318558004,29.6649827207885,179.002185338708));
#32114=CARTESIAN_POINT('Ctrl Pts',(30.4041598504741,30.1698800587628,178.891055549488));
#32115=CARTESIAN_POINT('Ctrl Pts',(29.5964289451286,32.347250120585,178.779925760269));
#32116=CARTESIAN_POINT('Ctrl Pts',(30.9882484770451,34.2080115613757,178.668795971049));
#32117=CARTESIAN_POINT('Ctrl Pts',(33.3060964076047,34.0474400400451,178.557666181829));
#32118=CARTESIAN_POINT('Ctrl Pts',(34.4285776240291,32.013360755941,178.446536392609));
#32119=CARTESIAN_POINT('Ctrl Pts',(33.3284712910932,29.9669128233058,178.33540660339));
#32120=CARTESIAN_POINT('Ctrl Pts',(31.0125524422092,29.7811934898284,178.22427681417));
#32121=CARTESIAN_POINT('Ctrl Pts',(29.6003397995657,31.626067795806,178.11314702495));
#32122=CARTESIAN_POINT('Ctrl Pts',(30.3842677378208,33.8131775063538,178.002017235731));
#32123=CARTESIAN_POINT('Ctrl Pts',(32.6468975047867,34.3408786212549,177.890887446511));
#32124=CARTESIAN_POINT('Ctrl Pts',(34.3174931090689,32.7262370373898,177.779757657291));
#32125=CARTESIAN_POINT('Ctrl Pts',(33.8671444377423,30.4469492135679,177.668627868071));
#32126=CARTESIAN_POINT('Ctrl Pts',(31.7080052850452,29.5889975993134,177.557498078852));
#32127=CARTESIAN_POINT('Ctrl Pts',(29.8160965978222,30.9375687585825,177.446368289632));
#32128=CARTESIAN_POINT('Ctrl Pts',(29.9228725869886,33.2584657028491,177.335238500412));
#32129=CARTESIAN_POINT('Ctrl Pts',(31.9306130756526,34.4276283682218,177.224108711192));
#32130=CARTESIAN_POINT('Ctrl Pts',(34.0018557168478,33.3750519340786,177.112978921973));
#32131=CARTESIAN_POINT('Ctrl Pts',(34.2410217192136,31.0640428539123,177.001849132753));
#32132=CARTESIAN_POINT('Ctrl Pts',(32.429228945055,29.6096116174522,176.890719343533));
#32133=CARTESIAN_POINT('Ctrl Pts',(30.224610496143,30.3428378993186,176.779589554313));
#32134=CARTESIAN_POINT('Ctrl Pts',(29.6448092673887,32.5926809678439,176.668459765094));
#32135=CARTESIAN_POINT('Ctrl Pts',(31.2204530563734,34.3001088403402,176.557329975874));
#32136=CARTESIAN_POINT('Ctrl Pts',(33.5095297542162,33.9025020465923,176.446200186654));
#32137=CARTESIAN_POINT('Ctrl Pts',(34.417101191225,31.7637460111891,176.335070397435));
#32138=CARTESIAN_POINT('Ctrl Pts',(33.112567830368,29.8412070644691,176.223940608215));
#32139=CARTESIAN_POINT('Ctrl Pts',(30.7898244564675,29.8943720011186,176.112810818995));
#32140=CARTESIAN_POINT('Ctrl Pts',(29.574620616194,31.8745848478056,176.001681029775));
#32141=CARTESIAN_POINT('Ctrl Pts',(30.5790976858388,33.9695762816876,175.890551240556));
#32142=CARTESIAN_POINT('Ctrl Pts',(32.8839691443584,34.2620328617456,175.779421451336));
#32143=CARTESIAN_POINT('Ctrl Pts',(34.3798416282082,32.4843014974535,175.668291662116));
#32144=CARTESIAN_POINT('Ctrl Pts',(33.6977088622292,30.2633426547257,175.557161872896));
#32145=CARTESIAN_POINT('Ctrl Pts',(31.4618513564243,29.6317537811269,175.446032083677));
#32146=CARTESIAN_POINT('Ctrl Pts',(29.7185016532407,31.1675581644807,175.334902294457));
#32147=CARTESIAN_POINT('Ctrl Pts',(30.063154495192,33.4652042882456,175.223772505237));
#32148=CARTESIAN_POINT('Ctrl Pts',(32.1803873389287,34.4219113368872,175.112642716017));
#32149=CARTESIAN_POINT('Ctrl Pts',(34.1325316462971,33.1621113945443,175.001512926798));
#32150=CARTESIAN_POINT('Ctrl Pts',(34.1330061173171,30.8387597064878,174.890383137578));
#32151=CARTESIAN_POINT('Ctrl Pts',(32.1813765212566,29.578162541927,174.779253348358));
#32152=CARTESIAN_POINT('Ctrl Pts',(30.0637530998886,30.5340047552611,174.668123559139));
#32153=CARTESIAN_POINT('Ctrl Pts',(29.7181618437792,32.8315099185237,174.556993769919));
#32154=CARTESIAN_POINT('Ctrl Pts',(31.4608841227388,34.3680262217031,174.445863980699));
#32155=CARTESIAN_POINT('Ctrl Pts',(33.6969994060995,33.7373506069548,174.33473419148));
#32156=CARTESIAN_POINT('Ctrl Pts',(34.3800392361903,31.5166705575043,174.22360440226));
#32157=CARTESIAN_POINT('Ctrl Pts',(32.8848929677704,29.7383283723363,174.11247461304));
#32158=CARTESIAN_POINT('Ctrl Pts',(30.5799022515117,30.0298435339987,174.00134482382));
#32159=CARTESIAN_POINT('Ctrl Pts',(29.5745695943507,32.1244245278882,173.890215034601));
#32160=CARTESIAN_POINT('Ctrl Pts',(30.7889645417425,34.1051335431823,173.779085245381));
#32161=CARTESIAN_POINT('Ctrl Pts',(33.1116860073988,34.1592471689786,173.667955456161));
#32162=CARTESIAN_POINT('Ctrl Pts',(34.4170044948166,32.2372412017861,173.556825666941));
#32163=CARTESIAN_POINT('Ctrl Pts',(33.5103066799004,30.0981146594927,173.445695877722));
#32164=CARTESIAN_POINT('Ctrl Pts',(31.2213925701334,29.6995729557439,173.334566088502));
#32165=CARTESIAN_POINT('Ctrl Pts',(29.6450515365342,31.4063571358058,173.223436299282));
#32166=CARTESIAN_POINT('Ctrl Pts',(30.2239337983464,33.6564368273894,173.112306510062));
#32167=CARTESIAN_POINT('Ctrl Pts',(32.4282525872759,34.3905634978557,173.001176720843));
#32168=CARTESIAN_POINT('Ctrl Pts',(34.2406392525365,32.936872379666,172.890046931623));
#32169=CARTESIAN_POINT('Ctrl Pts',(34.0024171725965,30.6257658195639,172.778917142403));
#32170=CARTESIAN_POINT('Ctrl Pts',(31.9316046116063,29.5723434784478,172.667787353184));
#32171=CARTESIAN_POINT('Ctrl Pts',(29.9233867683568,30.7406860590175,172.556657563964));
#32172=CARTESIAN_POINT('Ctrl Pts',(29.8156628347745,33.0615391016834,172.445527774744));
#32173=CARTESIAN_POINT('Ctrl Pts',(31.7070205866564,34.4108830704008,172.334397985525));
#32174=CARTESIAN_POINT('Ctrl Pts',(33.8665099204009,33.5538129980256,172.223268196305));
#32175=CARTESIAN_POINT('Ctrl Pts',(34.3177896164518,31.2747101202577,172.112138407085));
#32176=CARTESIAN_POINT('Ctrl Pts',(32.6478533909077,29.6593846749887,172.001008617865));
#32177=CARTESIAN_POINT('Ctrl Pts',(30.3850087676824,30.1861649922538,171.889878828646));
#32178=CARTESIAN_POINT('Ctrl Pts',(29.6001866064235,32.3729474383867,171.778749039426));
#32179=CARTESIAN_POINT('Ctrl Pts',(31.0116476380733,34.2184124333546,171.667619250206));
#32180=CARTESIAN_POINT('Ctrl Pts',(33.3276380331233,34.0336104269975,171.556489460986));
#32181=CARTESIAN_POINT('Ctrl Pts',(34.4285884978939,31.987670211439,171.445359671767));
#32182=CARTESIAN_POINT('Ctrl Pts',(33.3069211063375,29.9530140846606,171.334229882547));
#32183=CARTESIAN_POINT('Ctrl Pts',(30.9891736912303,29.7917372689629,171.223100093327));
#32184=CARTESIAN_POINT('Ctrl Pts',(29.5965235519542,31.6514385570982,171.111970304107));
#32185=CARTESIAN_POINT('Ctrl Pts',(30.403508993313,33.8301394977859,171.000840514888));
#32186=CARTESIAN_POINT('Ctrl Pts',(32.6715856907677,34.3339166171362,170.889710725668));
#32187=CARTESIAN_POINT('Ctrl Pts',(34.3250344470753,32.7017185587553,170.778580936448));
#32188=CARTESIAN_POINT('Ctrl Pts',(33.8506368913683,30.4273152852224,170.667451147229));
#32189=CARTESIAN_POINT('Ctrl Pts',(31.6825565220024,29.5922160075984,170.556321358009));
#32190=CARTESIAN_POINT('Ctrl Pts',(29.8049969811687,30.9606945284903,170.445191568789));
#32191=CARTESIAN_POINT('Ctrl Pts',(29.9362803993529,33.2803341461093,170.334061779569));
#32192=CARTESIAN_POINT('Ctrl Pts',(31.9562576159421,34.4282258378547,170.22293199035));
#32193=CARTESIAN_POINT('Ctrl Pts',(34.0162673880548,33.3538315758082,170.11180220113));
#32194=CARTESIAN_POINT('Ctrl Pts',(34.2310111121289,31.0404253372741,170.00067241191));
#32195=CARTESIAN_POINT('Ctrl Pts',(32.4039576606909,29.6052114239129,169.88954262269));
#32196=CARTESIAN_POINT('Ctrl Pts',(30.2072065389267,30.3616820449858,169.778412833471));
#32197=CARTESIAN_POINT('Ctrl Pts',(29.6512005507019,32.6175234916696,169.667283044251));
#32198=CARTESIAN_POINT('Ctrl Pts',(31.2447903468041,34.3082141355403,169.556153255031));
#32199=CARTESIAN_POINT('Ctrl Pts',(33.5295398276061,33.8864522341055,169.445023465811));
#32200=CARTESIAN_POINT('Ctrl Pts',(34.4144710453466,31.738229705738,169.333893676592));
#32201=CARTESIAN_POINT('Ctrl Pts',(33.0897045462445,29.8295765119025,169.222763887372));
#32202=CARTESIAN_POINT('Ctrl Pts',(30.7676522637518,29.9072713571029,169.111634098153));
#32203=CARTESIAN_POINT('Ctrl Pts',(29.5734312652623,31.9002087616026,169.000504308933));
#32204=CARTESIAN_POINT('Ctrl Pts',(30.599979657674,33.9844740252581,168.889374519713));
#32205=CARTESIAN_POINT('Ctrl Pts',(32.9078114849742,34.2525701817925,168.778244730493));
#32206=CARTESIAN_POINT('Ctrl Pts',(34.384824085665,32.4591385359132,168.667114941273));
#32207=CARTESIAN_POINT('Ctrl Pts',(33.6792715462419,30.2455082814088,168.555985152054));
#32208=CARTESIAN_POINT('Ctrl Pts',(31.43686789712,29.6375698204928,168.444855362834));
#32209=CARTESIAN_POINT('Ctrl Pts',(29.7098366447351,31.1917018415865,168.333725573614));
#32210=CARTESIAN_POINT('Ctrl Pts',(30.0787380530001,33.4855795691615,168.222595784395));
#32211=CARTESIAN_POINT('Ctrl Pts',(32.2059575727712,34.4198709905092,168.111465995175));
#32212=CARTESIAN_POINT('Ctrl Pts',(34.1446869293352,33.1395227135096,168.000336205955));
#32213=CARTESIAN_POINT('Ctrl Pts',(34.1206221195246,30.8162956275684,167.889206416735));
#32214=CARTESIAN_POINT('Ctrl Pts',(32.1557868348082,29.5763819040772,167.778076627516));
#32215=CARTESIAN_POINT('Ctrl Pts',(30.0483773488405,30.5545372653854,167.666946838296));
#32216=CARTESIAN_POINT('Ctrl Pts',(29.7270712997217,32.8555642699881,167.555817049076));
#32217=CARTESIAN_POINT('Ctrl Pts',(31.4859258624946,34.3735884913369,167.444687259856));
#32218=CARTESIAN_POINT('Ctrl Pts',(33.7152536393985,33.7193295360918,167.333557470637));
#32219=CARTESIAN_POINT('Ctrl Pts',(34.3748036771893,31.4915603207829,167.222427681417));
#32220=CARTESIAN_POINT('Ctrl Pts',(32.8609514252531,29.7291065603519,167.111297892197));
#32221=CARTESIAN_POINT('Ctrl Pts',(30.5591814806014,30.044956009926,167.000168102977));
#32222=CARTESIAN_POINT('Ctrl Pts',(29.5760010217537,32.1500279732525,166.889038313758));
#32223=CARTESIAN_POINT('Ctrl Pts',(30.8113032934655,34.1178215046619,166.777908524538));
#32224=CARTESIAN_POINT('Ctrl Pts',(33.1343552393677,34.1473557540512,166.666778735318));
#32225=CARTESIAN_POINT('Ctrl Pts',(34.4195276894793,32.2117592010123,166.555648946099));
#32226=CARTESIAN_POINT('Ctrl Pts',(33.4898246183641,30.0821472766194,166.444519156879));
#32227=CARTESIAN_POINT('Ctrl Pts',(31.1977703849704,29.7081726882415,166.333389367659));
#32228=CARTESIAN_POINT('Ctrl Pts',(29.6376219972954,31.4307513580499,166.222259578439));
#32229=CARTESIAN_POINT('Ctrl Pts',(30.2442045937981,33.6761645043479,166.11112978922));
#32230=CARTESIAN_POINT('Ctrl Pts',(31.7124802469762,34.1461819386551,166.037043263073));
#32231=CARTESIAN_POINT('Ctrl Pts',(32.3836679988478,34.0186125009917,166.));
#32232=CARTESIAN_POINT('Ctrl Pts',(33.2690708798531,33.0793586530476,179.));
#32233=CARTESIAN_POINT('Ctrl Pts',(33.3143937781624,33.0370771991883,179.));
#32234=CARTESIAN_POINT('Ctrl Pts',(33.3569863179444,32.9922261551744,179.));
#32235=CARTESIAN_POINT('Ctrl Pts',(33.3968502279411,32.9451506656108,179.));
#32236=CARTESIAN_POINT('Ctrl Pts',(33.4393503990047,32.8949620022427,179.));
#32237=CARTESIAN_POINT('Ctrl Pts',(33.4787498348177,32.8422447205077,179.));
#32238=CARTESIAN_POINT('Ctrl Pts',(33.515021779277,32.787362334173,179.));
#32239=CARTESIAN_POINT('Ctrl Pts',(33.5467597306789,32.7393402461302,179.));
#32240=CARTESIAN_POINT('Ctrl Pts',(33.5761029525123,32.6896592737051,179.));
#32241=CARTESIAN_POINT('Ctrl Pts',(33.6030106200597,32.6385353790539,179.));
#32242=CARTESIAN_POINT('Ctrl Pts',(33.6165047704786,32.6128968311118,179.));
#32243=CARTESIAN_POINT('Ctrl Pts',(33.6293860170028,32.586895031717,179.));
#32244=CARTESIAN_POINT('Ctrl Pts',(33.641646871455,32.5605553798914,179.));
#32245=CARTESIAN_POINT('Ctrl Pts',(33.6472617019107,32.5484931961473,179.));
#32246=CARTESIAN_POINT('Ctrl Pts',(33.6527470163596,32.5363584469774,179.));
#32247=CARTESIAN_POINT('Ctrl Pts',(33.6580935559345,32.5241735966087,179.));
#32248=CARTESIAN_POINT('Ctrl Pts',(33.6850051176496,32.4628417111726,179.));
#32249=CARTESIAN_POINT('Ctrl Pts',(33.708455881982,32.4001342696333,179.));
#32250=CARTESIAN_POINT('Ctrl Pts',(33.7284226243158,32.3364092263026,179.));
#32251=CARTESIAN_POINT('Ctrl Pts',(33.7487446483798,32.2715502802415,179.));
#32252=CARTESIAN_POINT('Ctrl Pts',(33.7654581172737,32.2056363549699,179.));
#32253=CARTESIAN_POINT('Ctrl Pts',(33.778499226047,32.1390083355841,179.));
#32254=CARTESIAN_POINT('Ctrl Pts',(33.789406899287,32.0832802010578,179.));
#32255=CARTESIAN_POINT('Ctrl Pts',(33.7977449205042,32.0270515616279,179.));
#32256=CARTESIAN_POINT('Ctrl Pts',(33.8034511333226,31.9705095923301,179.));
#32257=CARTESIAN_POINT('Ctrl Pts',(33.8060782739115,31.9444776676104,179.));
#32258=CARTESIAN_POINT('Ctrl Pts',(33.8081472199985,31.9183792139312,179.));
#32259=CARTESIAN_POINT('Ctrl Pts',(33.809650107142,31.8922320972929,179.));
#32260=CARTESIAN_POINT('Ctrl Pts',(33.8103080275562,31.8807856477814,179.));
#32261=CARTESIAN_POINT('Ctrl Pts',(33.8108573512992,31.8693300330975,179.));
#32262=CARTESIAN_POINT('Ctrl Pts',(33.8112970804587,31.857880967774,179.));
#32263=CARTESIAN_POINT('Ctrl Pts',(33.8139906687424,31.7877490068823,179.));
#32264=CARTESIAN_POINT('Ctrl Pts',(33.8125841486909,31.7177313799782,179.));
#32265=CARTESIAN_POINT('Ctrl Pts',(33.8070231799885,31.6481892005974,179.));
#32266=CARTESIAN_POINT('Ctrl Pts',(33.8020529941113,31.5860350011532,179.));
#32267=CARTESIAN_POINT('Ctrl Pts',(33.7937638352136,31.5242596307283,179.));
#32268=CARTESIAN_POINT('Ctrl Pts',(33.7820838097155,31.4631087786356,179.));
#32269=CARTESIAN_POINT('Ctrl Pts',(33.769354070438,31.3964621429871,179.));
#32270=CARTESIAN_POINT('Ctrl Pts',(33.7525976732535,31.3305564900439,179.));
#32271=CARTESIAN_POINT('Ctrl Pts',(33.7320596705581,31.265605227867,179.));
#32272=CARTESIAN_POINT('Ctrl Pts',(33.7241289063575,31.2405242522486,179.));
#32273=CARTESIAN_POINT('Ctrl Pts',(33.7156337035593,31.2155856354338,179.));
#32274=CARTESIAN_POINT('Ctrl Pts',(33.706586160513,31.1908019867147,179.));
#32275=CARTESIAN_POINT('Ctrl Pts',(33.702618487712,31.1799334660092,179.));
#32276=CARTESIAN_POINT('Ctrl Pts',(33.6985446903967,31.1690953061603,179.));
#32277=CARTESIAN_POINT('Ctrl Pts',(33.6943708791898,31.1583011218621,179.));
#32278=CARTESIAN_POINT('Ctrl Pts',(33.6691493675868,31.0930740114287,179.));
#32279=CARTESIAN_POINT('Ctrl Pts',(33.6402374396347,31.0293334091269,179.));
#32280=CARTESIAN_POINT('Ctrl Pts',(33.607947561365,30.9672979393099,179.));
#32281=CARTESIAN_POINT('Ctrl Pts',(33.5749108621329,30.9038276734593,179.));
#32282=CARTESIAN_POINT('Ctrl Pts',(33.5383378486612,30.8421415079131,179.));
#32283=CARTESIAN_POINT('Ctrl Pts',(33.498507043831,30.7824773207679,179.));
#32284=CARTESIAN_POINT('Ctrl Pts',(33.4680142575527,30.736800932484,179.));
#32285=CARTESIAN_POINT('Ctrl Pts',(33.4356109333393,30.6923095509569,179.));
#32286=CARTESIAN_POINT('Ctrl Pts',(33.4014024846335,30.6491160175195,179.));
#32287=CARTESIAN_POINT('Ctrl Pts',(33.3801001770704,30.6222185121127,179.));
#32288=CARTESIAN_POINT('Ctrl Pts',(33.358097552623,30.5958244105247,179.));
#32289=CARTESIAN_POINT('Ctrl Pts',(33.3354171550448,30.5699626540177,179.));
#32290=CARTESIAN_POINT('Ctrl Pts',(33.3227587779473,30.5555286977725,179.));
#32291=CARTESIAN_POINT('Ctrl Pts',(33.3098848307075,30.5412560553495,179.));
#32292=CARTESIAN_POINT('Ctrl Pts',(33.2968228468101,30.5271750883558,179.));
#32293=CARTESIAN_POINT('Ctrl Pts',(33.2459583837086,30.4723426194361,179.));
#32294=CARTESIAN_POINT('Ctrl Pts',(33.1921974074919,30.4203552297909,179.));
#32295=CARTESIAN_POINT('Ctrl Pts',(33.1358245952464,30.3714766007923,179.));
#32296=CARTESIAN_POINT('Ctrl Pts',(33.0936773153233,30.3349323664957,179.));
#32297=CARTESIAN_POINT('Ctrl Pts',(33.0500689035381,30.3001260799766,179.));
#32298=CARTESIAN_POINT('Ctrl Pts',(33.0051019564734,30.2671776805756,179.));
#32299=CARTESIAN_POINT('Ctrl Pts',(32.9910181102745,30.2568580965266,179.));
#32300=CARTESIAN_POINT('Ctrl Pts',(32.9768009030306,30.2467208427216,179.));
#32301=CARTESIAN_POINT('Ctrl Pts',(32.9624532443534,30.2367698321705,179.));
#32302=CARTESIAN_POINT('Ctrl Pts',(32.9486742469643,30.2272132242606,179.));
#32303=CARTESIAN_POINT('Ctrl Pts',(32.9347819948037,30.2178333484506,179.));
#32304=CARTESIAN_POINT('Ctrl Pts',(32.9207843887783,30.2086363784296,179.));
#32305=CARTESIAN_POINT('Ctrl Pts',(32.857836207379,30.1672769819617,179.));
#32306=CARTESIAN_POINT('Ctrl Pts',(32.79273001494,30.1295928505755,179.));
#32307=CARTESIAN_POINT('Ctrl Pts',(32.725726822945,30.0958629167136,179.));
#32308=CARTESIAN_POINT('Ctrl Pts',(32.6745421351153,30.0700961422685,179.));
#32309=CARTESIAN_POINT('Ctrl Pts',(32.6222494513403,30.0466373077193,179.));
#32310=CARTESIAN_POINT('Ctrl Pts',(32.5689512962096,30.0256259714062,179.));
#32311=CARTESIAN_POINT('Ctrl Pts',(32.5564668873308,30.0207043355076,179.));
#32312=CARTESIAN_POINT('Ctrl Pts',(32.5439272667614,30.0159170540829,179.));
#32313=CARTESIAN_POINT('Ctrl Pts',(32.5313343916942,30.0112635340338,179.));
#32314=CARTESIAN_POINT('Ctrl Pts',(30.3326674383851,31.998696643609,177.87148036339));
#32315=CARTESIAN_POINT('Ctrl Pts',(30.3319312160462,31.9130454971719,177.877220944861));
#32316=CARTESIAN_POINT('Ctrl Pts',(30.3379613622294,31.8274983352525,177.882961526332));
#32317=CARTESIAN_POINT('Ctrl Pts',(30.3511186960486,31.7430618380899,177.888702107803));
#32318=CARTESIAN_POINT('Ctrl Pts',(30.4360213458042,31.1982035526917,177.925745370876));
#32319=CARTESIAN_POINT('Ctrl Pts',(30.8176973425019,30.6995929198072,177.962788633949));
#32320=CARTESIAN_POINT('Ctrl Pts',(31.3214948089321,30.4753846070209,177.999831897022));
#32321=CARTESIAN_POINT('Ctrl Pts',(31.8252922753623,30.2511762942346,178.036875160096));
#32322=CARTESIAN_POINT('Ctrl Pts',(32.451211211525,30.3013703015467,178.073918423169));
#32323=CARTESIAN_POINT('Ctrl Pts',(32.9128324917223,30.6030120799742,178.110961686242));
#32324=CARTESIAN_POINT('Ctrl Pts',(33.3744537719195,30.9046538584017,178.148004949315));
#32325=CARTESIAN_POINT('Ctrl Pts',(33.6717773961514,31.4577434079447,178.185048212389));
#32326=CARTESIAN_POINT('Ctrl Pts',(33.6687537877731,32.0091615320545,178.222091475462));
#32327=CARTESIAN_POINT('Ctrl Pts',(33.6657301793948,32.5605796561643,178.259134738535));
#32328=CARTESIAN_POINT('Ctrl Pts',(33.3623593384064,33.1103263548409,178.296178001608));
#32329=CARTESIAN_POINT('Ctrl Pts',(32.8974537652324,33.4068983824074,178.333221264682));
#32330=CARTESIAN_POINT('Ctrl Pts',(32.4325481920584,33.703470409974,178.370264527755));
#32331=CARTESIAN_POINT('Ctrl Pts',(31.8061078866989,33.7468677664304,178.407307790828));
#32332=CARTESIAN_POINT('Ctrl Pts',(31.3048055390909,33.5171142355207,178.444351053901));
#32333=CARTESIAN_POINT('Ctrl Pts',(30.8035031914829,33.287360704611,178.481394316975));
#32334=CARTESIAN_POINT('Ctrl Pts',(30.4273388016264,32.7844562863351,178.518437580048));
#32335=CARTESIAN_POINT('Ctrl Pts',(30.348408546375,32.2387672663122,178.555480843121));
#32336=CARTESIAN_POINT('Ctrl Pts',(30.337044840679,32.1602036102679,178.560814016544));
#32337=CARTESIAN_POINT('Ctrl Pts',(30.3318421408634,32.0807531241047,178.566147189967));
#32338=CARTESIAN_POINT('Ctrl Pts',(30.3325025488117,32.0012179414303,178.57148036339));
#32339=CARTESIAN_POINT('Ctrl Pts',(31.4698297828098,30.0148256743287,179.));
#32340=CARTESIAN_POINT('Ctrl Pts',(30.8097602092458,30.191107033931,178.962956736927));
#32341=CARTESIAN_POINT('Ctrl Pts',(29.6908221960836,31.2516371458941,178.88887021078));
#32342=CARTESIAN_POINT('Ctrl Pts',(30.1185589391069,33.5378733053769,178.777740421561));
#32343=CARTESIAN_POINT('Ctrl Pts',(32.2716026719728,34.4129388487757,178.666610632341));
#32344=CARTESIAN_POINT('Ctrl Pts',(34.1744105218922,33.0815150675564,178.555480843121));
#32345=CARTESIAN_POINT('Ctrl Pts',(34.0880401159474,30.7594177996359,178.444351053901));
#32346=CARTESIAN_POINT('Ctrl Pts',(32.0903159869838,29.5731212764253,178.333221264682));
#32347=CARTESIAN_POINT('Ctrl Pts',(30.0101331232206,30.6076649966109,178.222091475462));
#32348=CARTESIAN_POINT('Ctrl Pts',(29.7509578494046,32.9165631575214,178.110961686242));
#32349=CARTESIAN_POINT('Ctrl Pts',(31.5501292046485,34.3865813061288,177.999831897022));
#32350=CARTESIAN_POINT('Ctrl Pts',(33.7609940320372,33.6724513469602,177.888702107803));
#32351=CARTESIAN_POINT('Ctrl Pts',(34.3602277126424,31.4276996634035,177.777572318583));
#32352=CARTESIAN_POINT('Ctrl Pts',(32.7994009405473,29.7067171266042,177.666442529363));
#32353=CARTESIAN_POINT('Ctrl Pts',(30.5069738698555,30.0845192170702,177.555312740143));
#32354=CARTESIAN_POINT('Ctrl Pts',(29.580946760212,32.2153500156115,177.444182950924));
#32355=CARTESIAN_POINT('Ctrl Pts',(30.8688116111015,34.1490940941566,177.333053161704));
#32356=CARTESIAN_POINT('Ctrl Pts',(33.1919274796751,34.1160109178655,177.221923372484));
#32357=CARTESIAN_POINT('Ctrl Pts',(34.4242044061711,32.1463773227603,177.110793583265));
#32358=CARTESIAN_POINT('Ctrl Pts',(33.4378756702622,30.0427808747097,176.999663794045));
#32359=CARTESIAN_POINT('Ctrl Pts',(31.135618752982,29.7304101029964,176.888534004825));
#32360=CARTESIAN_POINT('Ctrl Pts',(29.6244341600216,31.4951434129585,176.777404215606));
#32361=CARTESIAN_POINT('Ctrl Pts',(30.2873416712654,33.7219159863135,176.666274426386));
#32362=CARTESIAN_POINT('Ctrl Pts',(32.5176555073463,34.3728097273692,176.555144637166));
#32363=CARTESIAN_POINT('Ctrl Pts',(34.2742166391108,32.8521337355438,176.444014847946));
#32364=CARTESIAN_POINT('Ctrl Pts',(33.9494393645001,30.5515941911541,176.332885058726));
#32365=CARTESIAN_POINT('Ctrl Pts',(31.8405563248355,29.5766199351239,176.221755269507));
#32366=CARTESIAN_POINT('Ctrl Pts',(29.8775944073181,30.8194968342953,176.110625480287));
#32367=CARTESIAN_POINT('Ctrl Pts',(29.857035071825,33.1427574285537,175.999495691067));
#32368=CARTESIAN_POINT('Ctrl Pts',(31.7976939990458,34.4201788169579,175.888365901848));
#32369=CARTESIAN_POINT('Ctrl Pts',(33.9235011844546,33.4826787977943,175.777236112628));
#32370=CARTESIAN_POINT('Ctrl Pts',(34.2889409453366,31.1882472218883,175.666106323408));
#32371=CARTESIAN_POINT('Ctrl Pts',(32.5595667755852,29.6367229854095,175.554976534189));
#32372=CARTESIAN_POINT('Ctrl Pts',(30.3180831610634,30.248044244016,175.443846744969));
#32373=CARTESIAN_POINT('Ctrl Pts',(29.6158715979096,32.462736411328,175.332716955749));
#32374=CARTESIAN_POINT('Ctrl Pts',(31.0955884935522,34.2539372331611,175.221587166529));
#32375=CARTESIAN_POINT('Ctrl Pts',(33.4030129919618,33.982359142136,175.11045737731));
#32376=CARTESIAN_POINT('Ctrl Pts',(34.4264152151701,31.8965474620181,174.99932758809));
#32377=CARTESIAN_POINT('Ctrl Pts',(33.2291885468321,29.905414422765,174.88819779887));
#32378=CARTESIAN_POINT('Ctrl Pts',(30.9070218504281,29.8312233889627,174.77706800965));
#32379=CARTESIAN_POINT('Ctrl Pts',(29.5851369036578,31.7418731901787,174.665938220431));
#32380=CARTESIAN_POINT('Ctrl Pts',(30.4733084745601,33.8887578484745,174.554808431211));
#32381=CARTESIAN_POINT('Ctrl Pts',(32.7586915732648,34.3070718065724,174.443678641991));
#32382=CARTESIAN_POINT('Ctrl Pts',(34.3497283717851,32.6139786664471,174.332548852772));
#32383=CARTESIAN_POINT('Ctrl Pts',(33.7903192461908,30.3589789091108,174.221419063552));
#32384=CARTESIAN_POINT('Ctrl Pts',(31.5924293616864,29.6058238580236,174.110289274332));
#32385=CARTESIAN_POINT('Ctrl Pts',(29.7675437054471,31.0437928483141,173.999159485112));
#32386=CARTESIAN_POINT('Ctrl Pts',(29.9857778400022,33.3568722541927,173.888029695893));
#32387=CARTESIAN_POINT('Ctrl Pts',(32.0474062520575,34.428156887701,173.776899906673));
#32388=CARTESIAN_POINT('Ctrl Pts',(34.0656489763292,33.2772186698503,173.665770117453));
#32389=CARTESIAN_POINT('Ctrl Pts',(34.1934321584947,30.9573837762123,173.554640328233));
#32390=CARTESIAN_POINT('Ctrl Pts',(32.3138100159872,29.5917399438827,173.443510539014));
#32391=CARTESIAN_POINT('Ctrl Pts',(30.146992349976,30.4301095984188,173.332380749794));
#32392=CARTESIAN_POINT('Ctrl Pts',(29.6760271902357,32.7052259237296,173.221250960574));
#32393=CARTESIAN_POINT('Ctrl Pts',(31.3319367435559,34.3349271314997,173.110121171355));
#32394=CARTESIAN_POINT('Ctrl Pts',(33.5992505443295,33.8277283497517,172.998991382135));
#32395=CARTESIAN_POINT('Ctrl Pts',(34.4029475900826,31.6478124031995,172.887861592915));
#32396=CARTESIAN_POINT('Ctrl Pts',(33.0074930602737,29.7902147259237,172.776731803695));
#32397=CARTESIAN_POINT('Ctrl Pts',(30.6899918075095,29.9549885673591,172.665602014476));
#32398=CARTESIAN_POINT('Ctrl Pts',(29.5713958460653,31.9913346947219,172.554472225256));
#32399=CARTESIAN_POINT('Ctrl Pts',(30.6754320691868,34.035611215504,172.443342436036));
#32400=CARTESIAN_POINT('Ctrl Pts',(32.9916984982474,34.2169184271411,172.332212646816));
#32401=CARTESIAN_POINT('Ctrl Pts',(34.4003732162344,32.369325935738,172.221082857597));
#32402=CARTESIAN_POINT('Ctrl Pts',(33.6122523976872,30.1837303531204,172.109953068377));
#32403=CARTESIAN_POINT('Ctrl Pts',(31.3486156689259,29.6603650547029,171.998823279157));
#32404=CARTESIAN_POINT('Ctrl Pts',(29.6811188159947,31.2782082859368,171.887693489937));
#32405=CARTESIAN_POINT('Ctrl Pts',(30.1358368754459,33.5566274663761,171.776563700718));
#32406=CARTESIAN_POINT('Ctrl Pts',(32.2966168104817,34.41043807051,171.665433911498));
#32407=CARTESIAN_POINT('Ctrl Pts',(34.1859362572401,33.0582418926255,171.554304122278));
#32408=CARTESIAN_POINT('Ctrl Pts',(34.0747105468639,30.7375542107656,171.443174333058));
#32409=CARTESIAN_POINT('Ctrl Pts',(32.064732243297,29.5722432245585,171.332044543839));
#32410=CARTESIAN_POINT('Ctrl Pts',(29.9955116926565,30.6287889113096,171.220914754619));
#32411=CARTESIAN_POINT('Ctrl Pts',(29.7607771031263,32.9402521162651,171.1097849654));
#32412=CARTESIAN_POINT('Ctrl Pts',(31.5753550254538,34.3912067810244,170.99865517618));
#32413=CARTESIAN_POINT('Ctrl Pts',(33.7785634234029,33.6537549313479,170.88752538696));
#32414=CARTESIAN_POINT('Ctrl Pts',(34.3540498639709,31.4028045027273,170.77639559774));
#32415=CARTESIAN_POINT('Ctrl Pts',(32.7751353976405,29.6984009168952,170.66526580852));
#32416=CARTESIAN_POINT('Ctrl Pts',(30.4868254213828,30.1003958521179,170.554136019301));
#32417=CARTESIAN_POINT('Ctrl Pts',(29.5833564097807,32.2408879031331,170.443006230081));
#32418=CARTESIAN_POINT('Ctrl Pts',(30.8915734045388,34.1609219575215,170.331876440861));
#32419=CARTESIAN_POINT('Ctrl Pts',(33.2142103990771,34.1033036706089,170.220746651642));
#32420=CARTESIAN_POINT('Ctrl Pts',(34.4256152039436,32.1207646737337,170.109616862422));
#32421=CARTESIAN_POINT('Ctrl Pts',(33.4171232788624,30.0277031570956,169.998487073202));
#32422=CARTESIAN_POINT('Ctrl Pts',(31.1116954970284,29.7396663224151,169.887357283982));
#32423=CARTESIAN_POINT('Ctrl Pts',(29.6192343630528,31.5202623571622,169.776227494763));
#32424=CARTESIAN_POINT('Ctrl Pts',(30.305624121683,33.7399090800963,169.665097705543));
#32425=CARTESIAN_POINT('Ctrl Pts',(32.5426883094078,34.3672098814547,169.553967916323));
#32426=CARTESIAN_POINT('Ctrl Pts',(34.2830900415719,32.8280658706275,169.442838127104));
#32427=CARTESIAN_POINT('Ctrl Pts',(33.9340325267706,30.5310849550035,169.331708337884));
#32428=CARTESIAN_POINT('Ctrl Pts',(31.8149694171768,29.5784391588377,169.220578548664));
#32429=CARTESIAN_POINT('Ctrl Pts',(29.8652442904127,30.8419795837744,169.109448759444));
#32430=CARTESIAN_POINT('Ctrl Pts',(29.869224438595,33.165327735423,168.998318970225));
#32431=CARTESIAN_POINT('Ctrl Pts',(31.8232672732892,34.4221805810845,168.887189181005));
#32432=CARTESIAN_POINT('Ctrl Pts',(33.9390539828564,33.4622800263533,168.776059391785));
#32433=CARTESIAN_POINT('Ctrl Pts',(34.2802395155314,31.1641166493491,168.664929602565));
#32434=CARTESIAN_POINT('Ctrl Pts',(32.5345745716517,29.6309446499222,168.553799813346));
#32435=CARTESIAN_POINT('Ctrl Pts',(30.2996727772365,30.2659064158787,168.442670024126));
#32436=CARTESIAN_POINT('Ctrl Pts',(29.620892017365,32.4878918238939,168.331540234906));
#32437=CARTESIAN_POINT('Ctrl Pts',(31.1194450837624,34.2633639270065,168.220410445687));
#32438=CARTESIAN_POINT('Ctrl Pts',(33.4238724584211,33.9674299065165,168.109280656467));
#32439=CARTESIAN_POINT('Ctrl Pts',(34.4251872041711,31.8709253771026,167.998150867247));
#32440=CARTESIAN_POINT('Ctrl Pts',(33.206996913019,29.8925485313441,167.887021078027));
#32441=CARTESIAN_POINT('Ctrl Pts',(30.8841761520946,29.8428884386802,167.775891288808));
#32442=CARTESIAN_POINT('Ctrl Pts',(29.5825452442318,31.7673934065167,167.664761499588));
#32443=CARTESIAN_POINT('Ctrl Pts',(30.493342777661,33.9047775029395,167.553631710368));
#32444=CARTESIAN_POINT('Ctrl Pts',(32.7830165295865,34.2989296881618,167.442501921148));
#32445=CARTESIAN_POINT('Ctrl Pts',(34.3560823145915,32.5891267546308,167.331372131929));
#32446=CARTESIAN_POINT('Ctrl Pts',(33.7728865672594,30.3401605876776,167.220242342709));
#32447=CARTESIAN_POINT('Ctrl Pts',(31.5671653767747,29.6102631127892,167.109112553489));
#32448=CARTESIAN_POINT('Ctrl Pts',(29.7575674653531,31.0674235375315,166.99798276427));
#32449=CARTESIAN_POINT('Ctrl Pts',(30.0002241215838,33.3780747167424,166.88685297505));
#32450=CARTESIAN_POINT('Ctrl Pts',(32.073044548561,34.4275128335807,166.77572318583));
#32451=CARTESIAN_POINT('Ctrl Pts',(34.0790345884103,33.255346086573,166.66459339661));
#32452=CARTESIAN_POINT('Ctrl Pts',(34.1822756467128,30.9342420768624,166.553463607391));
#32453=CARTESIAN_POINT('Ctrl Pts',(32.2884012470789,29.5886265247524,166.442333818171));
#32454=CARTESIAN_POINT('Ctrl Pts',(30.1304232002167,30.4496328462658,166.331204028951));
#32455=CARTESIAN_POINT('Ctrl Pts',(29.6837912905188,32.7300090226775,166.220074239731));
#32456=CARTESIAN_POINT('Ctrl Pts',(31.356257105939,34.3412895988536,166.108944450512));
#32457=CARTESIAN_POINT('Ctrl Pts',(33.619236151672,33.8118910160724,165.997814661292));
#32458=CARTESIAN_POINT('Ctrl Pts',(34.3974968060795,31.6200550614307,165.886684872072));
#32459=CARTESIAN_POINT('Ctrl Pts',(33.4572031808889,30.3983372977448,165.812598345926));
#32460=CARTESIAN_POINT('Ctrl Pts',(32.8326019491379,30.1214975228146,165.775555082853));
#32461=CARTESIAN_POINT('Ctrl Pts',(31.5032651029109,30.1400211999976,179.074814972382));
#32462=CARTESIAN_POINT('Ctrl Pts',(30.8848229855212,30.3051853306515,179.037771709309));
#32463=CARTESIAN_POINT('Ctrl Pts',(29.8364510838271,31.2988328403474,178.963685183163));
#32464=CARTESIAN_POINT('Ctrl Pts',(30.2372124999491,33.44088693275,178.852555393943));
#32465=CARTESIAN_POINT('Ctrl Pts',(32.254473980124,34.2607662442478,178.741425604723));
#32466=CARTESIAN_POINT('Ctrl Pts',(34.0372807671961,33.0133090437071,178.630295815504));
#32467=CARTESIAN_POINT('Ctrl Pts',(33.9563573329528,30.8376554328259,178.519166026284));
#32468=CARTESIAN_POINT('Ctrl Pts',(32.0846201862067,29.7261730027164,178.408036237064));
#32469=CARTESIAN_POINT('Ctrl Pts',(30.1356245858232,30.6954729590666,178.296906447844));
#32470=CARTESIAN_POINT('Ctrl Pts',(29.8927942668186,32.8587598679912,178.185776658625));
#32471=CARTESIAN_POINT('Ctrl Pts',(31.5785004212106,34.236070946757,178.074646869405));
#32472=CARTESIAN_POINT('Ctrl Pts',(33.6499364938202,33.5669777757827,177.963517080185));
#32473=CARTESIAN_POINT('Ctrl Pts',(34.2113793493719,31.4637919302408,177.852387290966));
#32474=CARTESIAN_POINT('Ctrl Pts',(32.7489865161425,29.8513435964963,177.741257501746));
#32475=CARTESIAN_POINT('Ctrl Pts',(30.6011319439267,30.2053195016732,177.630127712526));
#32476=CARTESIAN_POINT('Ctrl Pts',(29.7335049703702,32.2017689118975,177.518997923306));
#32477=CARTESIAN_POINT('Ctrl Pts',(30.9401502956429,34.0135609264389,177.407868134087));
#32478=CARTESIAN_POINT('Ctrl Pts',(33.116758268867,33.9825641491069,177.296738344867));
#32479=CARTESIAN_POINT('Ctrl Pts',(34.2713213363899,32.1371459995299,177.185608555647));
#32480=CARTESIAN_POINT('Ctrl Pts',(33.3471956740235,30.1662133985295,177.074478766427));
#32481=CARTESIAN_POINT('Ctrl Pts',(31.1901311770041,29.8735423692835,176.963348977208));
#32482=CARTESIAN_POINT('Ctrl Pts',(29.7742498262084,31.5269823225115,176.852219187988));
#32483=CARTESIAN_POINT('Ctrl Pts',(30.3953509060134,33.6133229150267,176.741089398768));
#32484=CARTESIAN_POINT('Ctrl Pts',(32.4850094306167,34.2231678761279,176.629959609548));
#32485=CARTESIAN_POINT('Ctrl Pts',(34.1307925861515,32.7983937039596,176.518829820329));
#32486=CARTESIAN_POINT('Ctrl Pts',(33.8264974732807,30.6429382732709,176.407700031109));
#32487=CARTESIAN_POINT('Ctrl Pts',(31.8506116809161,29.7294510176109,176.29657024189));
#32488=CARTESIAN_POINT('Ctrl Pts',(30.0114444578766,30.8939455678262,176.185440452669));
#32489=CARTESIAN_POINT('Ctrl Pts',(29.9921817021251,33.0706891395728,176.07431066345));
#32490=CARTESIAN_POINT('Ctrl Pts',(31.8104524786453,34.2675496219881,175.96318087423));
#32491=CARTESIAN_POINT('Ctrl Pts',(33.8021950911818,33.3891732808794,175.85205108501));
#32492=CARTESIAN_POINT('Ctrl Pts',(34.1445883002461,31.2394406180825,175.740921295791));
#32493=CARTESIAN_POINT('Ctrl Pts',(32.5242775540239,29.7857636536858,175.629791506571));
#32494=CARTESIAN_POINT('Ctrl Pts',(30.4241536759089,30.3585317810463,175.518661717351));
#32495=CARTESIAN_POINT('Ctrl Pts',(29.766227264262,32.4335538214098,175.407531928132));
#32496=CARTESIAN_POINT('Ctrl Pts',(31.1526254361051,34.1117921061154,175.296402138912));
#32497=CARTESIAN_POINT('Ctrl Pts',(33.3145316194307,33.8573411567355,175.185272349692));
#32498=CARTESIAN_POINT('Ctrl Pts',(34.2733927201549,31.9030717227376,175.074142560472));
#32499=CARTESIAN_POINT('Ctrl Pts',(33.1516694573109,30.0375099969467,174.963012771253));
#32500=CARTESIAN_POINT('Ctrl Pts',(30.9759507964711,29.9679978396324,174.851882982033));
#32501=CARTESIAN_POINT('Ctrl Pts',(29.7374308613498,31.7581520233406,174.740753192813));
#32502=CARTESIAN_POINT('Ctrl Pts',(30.5695896653805,33.7696428525554,174.629623403593));
#32503=CARTESIAN_POINT('Ctrl Pts',(32.7108444955008,34.1615757340891,174.518493614374));
#32504=CARTESIAN_POINT('Ctrl Pts',(34.2015421521264,32.5752579450972,174.407363825154));
#32505=CARTESIAN_POINT('Ctrl Pts',(33.6774123058563,30.462470323165,174.296234035934));
#32506=CARTESIAN_POINT('Ctrl Pts',(31.6181329080456,29.7568131876572,174.185104246715));
#32507=CARTESIAN_POINT('Ctrl Pts',(29.9083341316153,31.1040962964574,174.073974457495));
#32508=CARTESIAN_POINT('Ctrl Pts',(30.1128052747589,33.2713007590689,173.962844668275));
#32509=CARTESIAN_POINT('Ctrl Pts',(32.0444165646686,34.275024553663,173.851714879055));
#32510=CARTESIAN_POINT('Ctrl Pts',(33.9353782962711,33.1966705483588,173.740585089836));
#32511=CARTESIAN_POINT('Ctrl Pts',(34.05510279943,31.0231366345483,173.629455300616));
#32512=CARTESIAN_POINT('Ctrl Pts',(32.2940195072124,29.7436174791571,173.518325511396));
#32513=CARTESIAN_POINT('Ctrl Pts',(30.2638527505027,30.5291151373919,173.407195722177));
#32514=CARTESIAN_POINT('Ctrl Pts',(29.8225891288001,32.6607506708034,173.296065932957));
#32515=CARTESIAN_POINT('Ctrl Pts',(31.374068323382,34.1876743558384,173.184936143737));
#32516=CARTESIAN_POINT('Ctrl Pts',(33.4983934004583,33.7124621947505,173.073806354517));
#32517=CARTESIAN_POINT('Ctrl Pts',(34.2514050868349,31.6700232039062,172.962676565298));
#32518=CARTESIAN_POINT('Ctrl Pts',(32.9439552532118,29.9295753983976,172.851546776078));
#32519=CARTESIAN_POINT('Ctrl Pts',(30.7726078086176,30.0839577354556,172.740416986858));
#32520=CARTESIAN_POINT('Ctrl Pts',(29.7245563870626,31.9918811744116,172.629287197638));
#32521=CARTESIAN_POINT('Ctrl Pts',(30.7589662839094,33.9072348745011,172.518157408419));
#32522=CARTESIAN_POINT('Ctrl Pts',(32.9291567792721,34.0771079005481,172.407027619199));
#32523=CARTESIAN_POINT('Ctrl Pts',(34.2489930665307,32.3460343013108,172.295897829979));
#32524=CARTESIAN_POINT('Ctrl Pts',(33.5105752886146,30.2982738620995,172.184768040759));
#32525=CARTESIAN_POINT('Ctrl Pts',(31.3896953880653,29.8079147298433,172.07363825154));
#32526=CARTESIAN_POINT('Ctrl Pts',(29.8273596498807,31.3237282646596,171.96250846232));
#32527=CARTESIAN_POINT('Ctrl Pts',(30.2534007988218,33.4584583577978,171.8513786731));
#32528=CARTESIAN_POINT('Ctrl Pts',(32.2779105956015,34.2584231782018,171.74024888388));
#32529=CARTESIAN_POINT('Ctrl Pts',(34.0480796291017,32.991503597495,171.629119094661));
#32530=CARTESIAN_POINT('Ctrl Pts',(33.9438683965466,30.8171706767696,171.517989305441));
#32531=CARTESIAN_POINT('Ctrl Pts',(32.0606498878471,29.7253503254147,171.406859516221));
#32532=CARTESIAN_POINT('Ctrl Pts',(30.1219252595105,30.7152646886918,171.295729727001));
#32533=CARTESIAN_POINT('Ctrl Pts',(29.9019942667975,32.8809548765038,171.184599937782));
#32534=CARTESIAN_POINT('Ctrl Pts',(31.6021353691866,34.2404047148974,171.073470148562));
#32535=CARTESIAN_POINT('Ctrl Pts',(33.6663978670339,33.5494604543942,170.962340359343));
#32536=CARTESIAN_POINT('Ctrl Pts',(34.2055911083041,31.4404667892284,170.851210570123));
#32537=CARTESIAN_POINT('Ctrl Pts',(32.7262512858941,29.8435518506758,170.740080780903));
#32538=CARTESIAN_POINT('Ctrl Pts',(30.5822541625009,30.2201948726783,170.628950991683));
#32539=CARTESIAN_POINT('Ctrl Pts',(29.7357626547736,32.2256962460227,170.517821202463));
#32540=CARTESIAN_POINT('Ctrl Pts',(30.9614766107659,34.0246428625811,170.406691413244));
#32541=CARTESIAN_POINT('Ctrl Pts',(33.1376359102681,33.9706582876428,170.295561624024));
#32542=CARTESIAN_POINT('Ctrl Pts',(34.2726431618406,32.1131486187531,170.184431834804));
#32543=CARTESIAN_POINT('Ctrl Pts',(33.3277520374855,30.1520865610262,170.073302045585));
#32544=CARTESIAN_POINT('Ctrl Pts',(31.1677166472949,29.8822148428614,169.962172256365));
#32545=CARTESIAN_POINT('Ctrl Pts',(29.7693779557629,31.5505171340862,169.851042467145));
#32546=CARTESIAN_POINT('Ctrl Pts',(30.4124803690279,33.6301812697564,169.739912677925));
#32547=CARTESIAN_POINT('Ctrl Pts',(32.5084635326252,34.2179211859256,169.628782888706));
#32548=CARTESIAN_POINT('Ctrl Pts',(34.139106385221,32.7758436850889,169.517653099486));
#32549=CARTESIAN_POINT('Ctrl Pts',(33.812062271706,30.6237224573342,169.406523310266));
#32550=CARTESIAN_POINT('Ctrl Pts',(31.8266384181214,29.7311555115167,169.295393521046));
#32551=CARTESIAN_POINT('Ctrl Pts',(29.9998732042468,30.9150104369695,169.184263731827));
#32552=CARTESIAN_POINT('Ctrl Pts',(30.0036023433679,33.0918360442771,169.073133942607));
#32553=CARTESIAN_POINT('Ctrl Pts',(31.8344129678195,34.2694251443491,168.962004153387));
#32554=CARTESIAN_POINT('Ctrl Pts',(33.8167670483817,33.3700609631672,168.850874364168));
#32555=CARTESIAN_POINT('Ctrl Pts',(34.136435628333,31.2168318462613,168.739744574948));
#32556=CARTESIAN_POINT('Ctrl Pts',(32.5008614898121,29.7803497304012,168.628614785728));
#32557=CARTESIAN_POINT('Ctrl Pts',(30.4069043476383,30.3752674704802,168.517484996508));
#32558=CARTESIAN_POINT('Ctrl Pts',(29.7709310696827,32.4571228014599,168.406355207289));
#32559=CARTESIAN_POINT('Ctrl Pts',(31.174977504363,34.1206243031067,168.295225418069));
#32560=CARTESIAN_POINT('Ctrl Pts',(33.3340755783122,33.8433534371718,168.184095628849));
#32561=CARTESIAN_POINT('Ctrl Pts',(34.2722421539831,31.8790655011488,168.072965839629));
#32562=CARTESIAN_POINT('Ctrl Pts',(33.1308773445499,30.0254554962531,167.96183605041));
#32563=CARTESIAN_POINT('Ctrl Pts',(30.9545458679356,29.9789272300114,167.85070626119));
#32564=CARTESIAN_POINT('Ctrl Pts',(29.7350026455872,31.7820628007198,167.73957647197));
#32565=CARTESIAN_POINT('Ctrl Pts',(30.5883605000415,33.7846522234216,167.628446682751));
#32566=CARTESIAN_POINT('Ctrl Pts',(32.7336353922418,34.1539471004548,167.517316893531));
#32567=CARTESIAN_POINT('Ctrl Pts',(34.2074953819074,32.5519733254443,167.406187104311));
#32568=CARTESIAN_POINT('Ctrl Pts',(33.6610790232724,30.4448387839772,167.295057315091));
#32569=CARTESIAN_POINT('Ctrl Pts',(31.5944622027923,29.7609724796875,167.183927525872));
#32570=CARTESIAN_POINT('Ctrl Pts',(29.8989870456498,31.1262367102264,167.072797736652));
#32571=CARTESIAN_POINT('Ctrl Pts',(30.1263404979045,33.2911660829048,166.961667947432));
#32572=CARTESIAN_POINT('Ctrl Pts',(32.0684379754575,34.2744211169802,166.850538158213));
#32573=CARTESIAN_POINT('Ctrl Pts',(33.9479197413089,33.17617736513,166.739408368993));
#32574=CARTESIAN_POINT('Ctrl Pts',(34.0446498759119,31.0014543723761,166.628278579773));
#32575=CARTESIAN_POINT('Ctrl Pts',(32.2702131488022,29.7407004085991,166.517148790554));
#32576=CARTESIAN_POINT('Ctrl Pts',(30.2483285384032,30.5474071466291,166.406019001334));
#32577=CARTESIAN_POINT('Ctrl Pts',(29.8298635841167,32.6839708172891,166.294889212114));
#32578=CARTESIAN_POINT('Ctrl Pts',(31.3968549159023,34.1936355725642,166.183759422894));
#32579=CARTESIAN_POINT('Ctrl Pts',(33.5171186103713,33.697623646563,166.072629633675));
#32580=CARTESIAN_POINT('Ctrl Pts',(34.2462980579166,31.6440163859826,165.961499844455));
#32581=CARTESIAN_POINT('Ctrl Pts',(33.3653042902582,30.4993465649714,165.887413318308));
#32582=CARTESIAN_POINT('Ctrl Pts',(32.78009369465,30.2399657611251,165.850370055235));
#32583=CARTESIAN_POINT('Ctrl Pts',(31.5367004230119,30.2652167256666,179.149629944765));
#32584=CARTESIAN_POINT('Ctrl Pts',(30.9598857617967,30.419263627372,179.112586681692));
#32585=CARTESIAN_POINT('Ctrl Pts',(29.9820799715705,31.3460285348007,179.038500155545));
#32586=CARTESIAN_POINT('Ctrl Pts',(30.3558660607915,33.3439005601231,178.927370366326));
#32587=CARTESIAN_POINT('Ctrl Pts',(32.237345288275,34.1085936397198,178.816240577106));
#32588=CARTESIAN_POINT('Ctrl Pts',(33.9001510125,32.9451030198579,178.705110787886));
#32589=CARTESIAN_POINT('Ctrl Pts',(33.8246745499582,30.9158930660159,178.593980998666));
#32590=CARTESIAN_POINT('Ctrl Pts',(32.0789243854297,29.8792247290074,178.482851209447));
#32591=CARTESIAN_POINT('Ctrl Pts',(30.2611160484258,30.7832809215223,178.371721420227));
#32592=CARTESIAN_POINT('Ctrl Pts',(30.0346306842325,32.8009565784611,178.260591631007));
#32593=CARTESIAN_POINT('Ctrl Pts',(31.6068716377727,34.0855605873852,178.149461841787));
#32594=CARTESIAN_POINT('Ctrl Pts',(33.5388789556032,33.4615042046052,178.038332052568));
#32595=CARTESIAN_POINT('Ctrl Pts',(34.0625309861015,31.4998841970782,177.927202263348));
#32596=CARTESIAN_POINT('Ctrl Pts',(32.6985720917375,29.9959700663885,177.816072474128));
#32597=CARTESIAN_POINT('Ctrl Pts',(30.695290017998,30.3261197862762,177.704942684909));
#32598=CARTESIAN_POINT('Ctrl Pts',(29.8860631805284,32.1881878081835,177.593812895689));
#32599=CARTESIAN_POINT('Ctrl Pts',(31.0114889801843,33.8780277587213,177.482683106469));
#32600=CARTESIAN_POINT('Ctrl Pts',(33.041589058059,33.8491173803483,177.371553317249));
#32601=CARTESIAN_POINT('Ctrl Pts',(34.1184382666087,32.1279146762995,177.26042352803));
#32602=CARTESIAN_POINT('Ctrl Pts',(33.2565156777848,30.2896459223494,177.14929373881));
#32603=CARTESIAN_POINT('Ctrl Pts',(31.2446436010262,30.0166746355706,177.03816394959));
#32604=CARTESIAN_POINT('Ctrl Pts',(29.9240654923951,31.5588212320646,176.92703416037));
#32605=CARTESIAN_POINT('Ctrl Pts',(30.5033601407615,33.50472984374,176.815904371151));
#32606=CARTESIAN_POINT('Ctrl Pts',(32.452363353887,34.0735260248864,176.704774581931));
#32607=CARTESIAN_POINT('Ctrl Pts',(33.9873685331922,32.7446536723755,176.593644792711));
#32608=CARTESIAN_POINT('Ctrl Pts',(33.7035555820612,30.7342823553878,176.482515003492));
#32609=CARTESIAN_POINT('Ctrl Pts',(31.8606670369967,29.8822821000979,176.371385214272));
#32610=CARTESIAN_POINT('Ctrl Pts',(30.1452945084351,30.9683943013571,176.260255425052));
#32611=CARTESIAN_POINT('Ctrl Pts',(30.1273283324253,32.998620850592,176.149125635832));
#32612=CARTESIAN_POINT('Ctrl Pts',(31.8232109582448,34.1149204270184,176.037995846613));
#32613=CARTESIAN_POINT('Ctrl Pts',(33.680888997909,33.2956677639645,175.926866057393));
#32614=CARTESIAN_POINT('Ctrl Pts',(34.0002356551555,31.2906340142769,175.815736268173));
#32615=CARTESIAN_POINT('Ctrl Pts',(32.4889883324627,29.934804321962,175.704606478953));
#32616=CARTESIAN_POINT('Ctrl Pts',(30.5302241907544,30.4690193180765,175.593476689734));
#32617=CARTESIAN_POINT('Ctrl Pts',(29.9165829306144,32.4043712314915,175.482346900514));
#32618=CARTESIAN_POINT('Ctrl Pts',(31.2096623786579,33.9696469790697,175.371217111294));
#32619=CARTESIAN_POINT('Ctrl Pts',(33.2260502468995,33.7323231713349,175.260087322075));
#32620=CARTESIAN_POINT('Ctrl Pts',(34.1203702251398,31.9095959834572,175.148957532855));
#32621=CARTESIAN_POINT('Ctrl Pts',(33.0741503677897,30.1696055711286,175.037827743635));
#32622=CARTESIAN_POINT('Ctrl Pts',(31.0448797425142,30.1047722903021,174.926697954415));
#32623=CARTESIAN_POINT('Ctrl Pts',(29.8897248190418,31.7744308565025,174.815568165196));
#32624=CARTESIAN_POINT('Ctrl Pts',(30.6658708562009,33.6505278566363,174.704438375976));
#32625=CARTESIAN_POINT('Ctrl Pts',(32.6629974177368,34.0160796616058,174.593308586756));
#32626=CARTESIAN_POINT('Ctrl Pts',(34.0533559324676,32.5365372237472,174.482178797536));
#32627=CARTESIAN_POINT('Ctrl Pts',(33.5645053655219,30.5659617372191,174.371049008317));
#32628=CARTESIAN_POINT('Ctrl Pts',(31.6438364544047,29.9078025172906,174.259919219097));
#32629=CARTESIAN_POINT('Ctrl Pts',(30.0491245577835,31.1643997446009,174.148789429877));
#32630=CARTESIAN_POINT('Ctrl Pts',(30.2398327095156,33.1857292639449,174.037659640658));
#32631=CARTESIAN_POINT('Ctrl Pts',(32.0414268772797,34.1218922196251,173.926529851438));
#32632=CARTESIAN_POINT('Ctrl Pts',(33.805107616213,33.1161224268672,173.815400062218));
#32633=CARTESIAN_POINT('Ctrl Pts',(33.9167734403653,31.0888894928842,173.704270272998));
#32634=CARTESIAN_POINT('Ctrl Pts',(32.2742289984375,29.8954950144316,173.593140483778));
#32635=CARTESIAN_POINT('Ctrl Pts',(30.3807131510295,30.6281206763649,173.482010694559));
#32636=CARTESIAN_POINT('Ctrl Pts',(29.9691510673645,32.6162754178773,173.370880905339));
#32637=CARTESIAN_POINT('Ctrl Pts',(31.416199903208,34.040421580177,173.25975111612));
#32638=CARTESIAN_POINT('Ctrl Pts',(33.3975362565871,33.5971960397494,173.1486213269));
#32639=CARTESIAN_POINT('Ctrl Pts',(34.0998625835872,31.6922340046129,173.03749153768));
#32640=CARTESIAN_POINT('Ctrl Pts',(32.8804174461499,30.0689360708715,172.92636174846));
#32641=CARTESIAN_POINT('Ctrl Pts',(30.8552238097257,30.2129269035522,172.815231959241));
#32642=CARTESIAN_POINT('Ctrl Pts',(29.8777169280598,31.9924276541012,172.704102170021));
#32643=CARTESIAN_POINT('Ctrl Pts',(30.8425004986319,33.7788585334981,172.592972380801));
#32644=CARTESIAN_POINT('Ctrl Pts',(32.8666150602968,33.9372973739551,172.481842591581));
#32645=CARTESIAN_POINT('Ctrl Pts',(34.097612916827,32.3227426668835,172.370712802362));
#32646=CARTESIAN_POINT('Ctrl Pts',(33.408898179542,30.4128173710787,172.259583013142));
#32647=CARTESIAN_POINT('Ctrl Pts',(31.4307751072047,29.9554644049837,172.148453223922));
#32648=CARTESIAN_POINT('Ctrl Pts',(29.9736004837668,31.3692482433824,172.037323434702));
#32649=CARTESIAN_POINT('Ctrl Pts',(30.3709647221978,33.3602892492196,171.926193645483));
#32650=CARTESIAN_POINT('Ctrl Pts',(32.2592043807214,34.1064082858936,171.815063856263));
#32651=CARTESIAN_POINT('Ctrl Pts',(33.9102230009633,32.9247653023644,171.703934067043));
#32652=CARTESIAN_POINT('Ctrl Pts',(33.8130262462293,30.8967871427735,171.592804277824));
#32653=CARTESIAN_POINT('Ctrl Pts',(32.0565675323973,29.8784574262709,171.481674488604));
#32654=CARTESIAN_POINT('Ctrl Pts',(30.2483388263645,30.8017404660741,171.370544699384));
#32655=CARTESIAN_POINT('Ctrl Pts',(30.0432114304686,32.8216576367426,171.259414910164));
#32656=CARTESIAN_POINT('Ctrl Pts',(31.6289157129194,34.0896026487704,171.148285120945));
#32657=CARTESIAN_POINT('Ctrl Pts',(33.5542323106648,33.4451659774406,171.037155331725));
#32658=CARTESIAN_POINT('Ctrl Pts',(34.0571323526374,31.4781290757296,170.926025542505));
#32659=CARTESIAN_POINT('Ctrl Pts',(32.6773671741476,29.9887027844564,170.814895753285));
#32660=CARTESIAN_POINT('Ctrl Pts',(30.6776829036191,30.3399938932386,170.703765964066));
#32661=CARTESIAN_POINT('Ctrl Pts',(29.8881688997665,32.2105045889123,170.592636174846));
#32662=CARTESIAN_POINT('Ctrl Pts',(31.031379816993,33.8883637676406,170.481506385626));
#32663=CARTESIAN_POINT('Ctrl Pts',(33.061061421459,33.8380129046766,170.370376596406));
#32664=CARTESIAN_POINT('Ctrl Pts',(34.1196711197376,32.1055325637725,170.259246807187));
#32665=CARTESIAN_POINT('Ctrl Pts',(33.2383807961085,30.2764699649568,170.148117017967));
#32666=CARTESIAN_POINT('Ctrl Pts',(31.2237377975614,30.0247633633077,170.036987228747));
#32667=CARTESIAN_POINT('Ctrl Pts',(29.919521548473,31.5807719110101,169.925857439528));
#32668=CARTESIAN_POINT('Ctrl Pts',(30.5193366163728,33.5204534594166,169.814727650308));
#32669=CARTESIAN_POINT('Ctrl Pts',(32.4742387558426,34.0686324903965,169.703597861088));
#32670=CARTESIAN_POINT('Ctrl Pts',(33.9951227288701,32.7236214995502,169.592468071869));
#32671=CARTESIAN_POINT('Ctrl Pts',(33.6900920166414,30.716359959665,169.481338282649));
#32672=CARTESIAN_POINT('Ctrl Pts',(31.8383074190659,29.8838718641958,169.370208493429));
#32673=CARTESIAN_POINT('Ctrl Pts',(30.134502118081,30.9880412901646,169.259078704209));
#32674=CARTESIAN_POINT('Ctrl Pts',(30.1379802481407,33.0183443531313,169.14794891499));
#32675=CARTESIAN_POINT('Ctrl Pts',(31.8455586623499,34.1166697076136,169.03681912577));
#32676=CARTESIAN_POINT('Ctrl Pts',(33.6944801139071,33.2778418999811,168.92568933655));
#32677=CARTESIAN_POINT('Ctrl Pts',(33.9926317411346,31.2695470431734,168.81455954733));
#32678=CARTESIAN_POINT('Ctrl Pts',(32.4671484079726,29.9297548108802,168.703429758111));
#32679=CARTESIAN_POINT('Ctrl Pts',(30.5141359180401,30.4846285250817,168.592299968891));
#32680=CARTESIAN_POINT('Ctrl Pts',(29.9209701220004,32.4263537790259,168.481170179671));
#32681=CARTESIAN_POINT('Ctrl Pts',(31.2305099249636,33.977884679207,168.370040390452));
#32682=CARTESIAN_POINT('Ctrl Pts',(33.2442786982033,33.719276967827,168.258910601232));
#32683=CARTESIAN_POINT('Ctrl Pts',(34.1192971037951,31.8872056251949,168.147780812012));
#32684=CARTESIAN_POINT('Ctrl Pts',(33.0547577760807,30.158362461162,168.036651022792));
#32685=CARTESIAN_POINT('Ctrl Pts',(31.0249155837767,30.1149660213425,167.925521233573));
#32686=CARTESIAN_POINT('Ctrl Pts',(29.8874600469425,31.796732194923,167.814391444353));
#32687=CARTESIAN_POINT('Ctrl Pts',(30.6833782224221,33.6645269439038,167.703261655133));
#32688=CARTESIAN_POINT('Ctrl Pts',(32.6842542548971,34.0089645127478,167.592131865913));
#32689=CARTESIAN_POINT('Ctrl Pts',(34.0589084492235,32.5148198962578,167.481002076694));
#32690=CARTESIAN_POINT('Ctrl Pts',(33.5492714792853,30.5495169802769,167.369872287474));
#32691=CARTESIAN_POINT('Ctrl Pts',(31.6217590288099,29.9116818465859,167.258742498254));
#32692=CARTESIAN_POINT('Ctrl Pts',(30.0404066259465,31.1850498829213,167.147612709034));
#32693=CARTESIAN_POINT('Ctrl Pts',(30.2524568742251,33.2042574490671,167.036482919815));
#32694=CARTESIAN_POINT('Ctrl Pts',(32.063831402354,34.1213294003798,166.925353130595));
#32695=CARTESIAN_POINT('Ctrl Pts',(33.8168048942076,33.0970086436869,166.814223341375));
#32696=CARTESIAN_POINT('Ctrl Pts',(33.9070241051109,31.0686666678897,166.703093552156));
#32697=CARTESIAN_POINT('Ctrl Pts',(32.2520250505256,29.8927742924459,166.591963762936));
#32698=CARTESIAN_POINT('Ctrl Pts',(30.3662338765896,30.6451814469923,166.480833973716));
#32699=CARTESIAN_POINT('Ctrl Pts',(29.9759358777146,32.6379326119006,166.369704184496));
#32700=CARTESIAN_POINT('Ctrl Pts',(31.4374527258656,34.0459815462748,166.258574395277));
#32701=CARTESIAN_POINT('Ctrl Pts',(33.4150010690707,33.5833562770537,166.147444606057));
#32702=CARTESIAN_POINT('Ctrl Pts',(34.0950993097536,31.6679777105344,166.036314816837));
#32703=CARTESIAN_POINT('Ctrl Pts',(33.2734053996274,30.600355832198,165.962228290691));
#32704=CARTESIAN_POINT('Ctrl Pts',(32.727585440162,30.3584339994357,165.925185027618));
#32705=CARTESIAN_POINT('Ctrl Pts',(31.5701357431129,30.3904122513355,179.224444917147));
#32706=CARTESIAN_POINT('Ctrl Pts',(31.0349485380721,30.5333419240925,179.187401654074));
#32707=CARTESIAN_POINT('Ctrl Pts',(30.1277088593139,31.393224229254,179.113315127928));
#32708=CARTESIAN_POINT('Ctrl Pts',(30.4745196216338,33.2469141874962,179.002185338708));
#32709=CARTESIAN_POINT('Ctrl Pts',(32.2202165964262,33.9564210351918,178.891055549488));
#32710=CARTESIAN_POINT('Ctrl Pts',(33.7630212578038,32.8768969960087,178.779925760269));
#32711=CARTESIAN_POINT('Ctrl Pts',(33.6929917669636,30.9941306992059,178.668795971049));
#32712=CARTESIAN_POINT('Ctrl Pts',(32.0732285846526,30.0322764552985,178.557666181829));
#32713=CARTESIAN_POINT('Ctrl Pts',(30.3866075110284,30.871088883978,178.446536392609));
#32714=CARTESIAN_POINT('Ctrl Pts',(30.1764671016465,32.7431532889309,178.33540660339));
#32715=CARTESIAN_POINT('Ctrl Pts',(31.6352428543348,33.9350502280134,178.22427681417));
#32716=CARTESIAN_POINT('Ctrl Pts',(33.4278214173861,33.3560306334278,178.11314702495));
#32717=CARTESIAN_POINT('Ctrl Pts',(33.9136826228311,31.5359764639154,178.002017235731));
#32718=CARTESIAN_POINT('Ctrl Pts',(32.6481576673327,30.1405965362806,177.890887446511));
#32719=CARTESIAN_POINT('Ctrl Pts',(30.7894480920692,30.4469200708791,177.779757657291));
#32720=CARTESIAN_POINT('Ctrl Pts',(30.0386213906866,32.1746067044695,177.668627868071));
#32721=CARTESIAN_POINT('Ctrl Pts',(31.0828276647257,33.7424945910037,177.557498078852));
#32722=CARTESIAN_POINT('Ctrl Pts',(32.9664198472509,33.7156706115897,177.446368289632));
#32723=CARTESIAN_POINT('Ctrl Pts',(33.9655551968274,32.1186833530691,177.335238500412));
#32724=CARTESIAN_POINT('Ctrl Pts',(33.1658356815461,30.4130784461693,177.224108711192));
#32725=CARTESIAN_POINT('Ctrl Pts',(31.2991560250483,30.1598069018577,177.112978921973));
#32726=CARTESIAN_POINT('Ctrl Pts',(30.0738811585818,31.5906601416176,177.001849132753));
#32727=CARTESIAN_POINT('Ctrl Pts',(30.6113693755095,33.3961367724532,176.890719343533));
#32728=CARTESIAN_POINT('Ctrl Pts',(32.4197172771573,33.923884173645,176.779589554314));
#32729=CARTESIAN_POINT('Ctrl Pts',(33.8439444802329,32.6909136407913,176.668459765094));
#32730=CARTESIAN_POINT('Ctrl Pts',(33.5806136908418,30.8256264375046,176.557329975874));
#32731=CARTESIAN_POINT('Ctrl Pts',(31.8707223930774,30.035113182585,176.446200186654));
#32732=CARTESIAN_POINT('Ctrl Pts',(30.2791445589935,31.0428430348879,176.335070397435));
#32733=CARTESIAN_POINT('Ctrl Pts',(30.2624749627256,32.9265525616111,176.223940608215));
#32734=CARTESIAN_POINT('Ctrl Pts',(31.8359694378442,33.9622912320486,176.112810818995));
#32735=CARTESIAN_POINT('Ctrl Pts',(33.5595829046363,33.2021622470496,176.001681029775));
#32736=CARTESIAN_POINT('Ctrl Pts',(33.8558830100649,31.3418274104712,175.890551240556));
#32737=CARTESIAN_POINT('Ctrl Pts',(32.4536991109015,30.0838449902383,175.779421451336));
#32738=CARTESIAN_POINT('Ctrl Pts',(30.6362947056,30.5795068551068,175.668291662116));
#32739=CARTESIAN_POINT('Ctrl Pts',(30.0669385969668,32.3751886415732,175.557161872896));
#32740=CARTESIAN_POINT('Ctrl Pts',(31.2666993212108,33.827501852024,175.446032083677));
#32741=CARTESIAN_POINT('Ctrl Pts',(33.1375688743684,33.6073051859344,175.334902294457));
#32742=CARTESIAN_POINT('Ctrl Pts',(33.9673477301245,31.9161202441767,175.223772505237));
#32743=CARTESIAN_POINT('Ctrl Pts',(32.9966312782686,30.3017011453104,175.112642716018));
#32744=CARTESIAN_POINT('Ctrl Pts',(31.1138086885573,30.2415467409718,175.001512926798));
#32745=CARTESIAN_POINT('Ctrl Pts',(30.0420187767338,31.7907096896643,174.890383137578));
#32746=CARTESIAN_POINT('Ctrl Pts',(30.7621520470214,33.5314128607172,174.779253348358));
#32747=CARTESIAN_POINT('Ctrl Pts',(32.6151503399728,33.8705835891225,174.668123559139));
#32748=CARTESIAN_POINT('Ctrl Pts',(33.9051697128089,32.4978165023973,174.556993769919));
#32749=CARTESIAN_POINT('Ctrl Pts',(33.4515984251874,30.6694531512732,174.445863980699));
#32750=CARTESIAN_POINT('Ctrl Pts',(31.6695400007639,30.0587918469241,174.334734191479));
#32751=CARTESIAN_POINT('Ctrl Pts',(30.1899149839517,31.2247031927443,174.22360440226));
#32752=CARTESIAN_POINT('Ctrl Pts',(30.3668601442724,33.100157768821,174.11247461304));
#32753=CARTESIAN_POINT('Ctrl Pts',(32.0384371898907,33.968759885587,174.00134482382));
#32754=CARTESIAN_POINT('Ctrl Pts',(33.674836936155,33.0355743053757,173.890215034601));
#32755=CARTESIAN_POINT('Ctrl Pts',(33.7784440813005,31.1546423512202,173.779085245381));
#32756=CARTESIAN_POINT('Ctrl Pts',(32.2544384896628,30.047372549706,173.667955456161));
#32757=CARTESIAN_POINT('Ctrl Pts',(30.4975735515562,30.727126215338,173.556825666941));
#32758=CARTESIAN_POINT('Ctrl Pts',(30.115713005929,32.5718001649512,173.445695877722));
#32759=CARTESIAN_POINT('Ctrl Pts',(31.458331483034,33.8931688045157,173.334566088502));
#32760=CARTESIAN_POINT('Ctrl Pts',(33.2966791127159,33.4819298847482,173.223436299282));
#32761=CARTESIAN_POINT('Ctrl Pts',(33.9483200803396,31.7144448053196,173.112306510062));
#32762=CARTESIAN_POINT('Ctrl Pts',(32.8168796390879,30.2082967433453,173.001176720843));
#32763=CARTESIAN_POINT('Ctrl Pts',(30.9378398108339,30.3418960716488,172.890046931623));
#32764=CARTESIAN_POINT('Ctrl Pts',(30.030877469057,31.9929741337908,172.778917142403));
#32765=CARTESIAN_POINT('Ctrl Pts',(30.9260347133546,33.6504821924952,172.667787353184));
#32766=CARTESIAN_POINT('Ctrl Pts',(32.8040733413214,33.797486847362,172.556657563964));
#32767=CARTESIAN_POINT('Ctrl Pts',(33.9462327671232,32.2994510324562,172.445527774744));
#32768=CARTESIAN_POINT('Ctrl Pts',(33.3072210704694,30.5273608800578,172.334397985524));
#32769=CARTESIAN_POINT('Ctrl Pts',(31.4718548263441,30.1030140801241,172.223268196305));
#32770=CARTESIAN_POINT('Ctrl Pts',(30.1198413176528,31.4147682221052,172.112138407085));
#32771=CARTESIAN_POINT('Ctrl Pts',(30.4885286455738,33.2621201406413,172.001008617865));
#32772=CARTESIAN_POINT('Ctrl Pts',(32.2404981658413,33.9543933935854,171.889878828646));
#32773=CARTESIAN_POINT('Ctrl Pts',(33.7723663728249,32.858027007234,171.778749039426));
#32774=CARTESIAN_POINT('Ctrl Pts',(33.6821840959121,30.9764036087774,171.667619250206));
#32775=CARTESIAN_POINT('Ctrl Pts',(32.0524851769474,30.0315645271271,171.556489460986));
#32776=CARTESIAN_POINT('Ctrl Pts',(30.3747523932185,30.8882162434563,171.445359671767));
#32777=CARTESIAN_POINT('Ctrl Pts',(30.1844285941397,32.7623603969814,171.334229882547));
#32778=CARTESIAN_POINT('Ctrl Pts',(31.6556960566522,33.9388005826434,171.223100093327));
#32779=CARTESIAN_POINT('Ctrl Pts',(33.4420667542958,33.340871500487,171.111970304107));
#32780=CARTESIAN_POINT('Ctrl Pts',(33.9086735969707,31.5157913622307,171.000840514888));
#32781=CARTESIAN_POINT('Ctrl Pts',(32.6284830624013,30.133853718237,170.889710725668));
#32782=CARTESIAN_POINT('Ctrl Pts',(30.7731116447372,30.4597929137989,170.778580936448));
#32783=CARTESIAN_POINT('Ctrl Pts',(30.0405751447595,32.1953129318018,170.667451147229));
#32784=CARTESIAN_POINT('Ctrl Pts',(31.1012830232201,33.7520846727002,170.556321358009));
#32785=CARTESIAN_POINT('Ctrl Pts',(32.98448693265,33.7053675217104,170.445191568789));
#32786=CARTESIAN_POINT('Ctrl Pts',(33.9666990776347,32.0979165087919,170.334061779569));
#32787=CARTESIAN_POINT('Ctrl Pts',(33.1490095547316,30.4008533688874,170.22293199035));
#32788=CARTESIAN_POINT('Ctrl Pts',(31.2797589478278,30.167311883754,170.11180220113));
#32789=CARTESIAN_POINT('Ctrl Pts',(30.0696651411831,31.611026687934,170.00067241191));
#32790=CARTESIAN_POINT('Ctrl Pts',(30.6261928637177,33.4107256490767,169.88954262269));
#32791=CARTESIAN_POINT('Ctrl Pts',(32.4400139790599,33.9193437948674,169.778412833471));
#32792=CARTESIAN_POINT('Ctrl Pts',(33.8511390725192,32.6713993140116,169.667283044251));
#32793=CARTESIAN_POINT('Ctrl Pts',(33.5681217615767,30.8089974619958,169.556153255031));
#32794=CARTESIAN_POINT('Ctrl Pts',(31.8499764200105,30.0365882168748,169.445023465812));
#32795=CARTESIAN_POINT('Ctrl Pts',(30.2691310319151,31.0610721433597,169.333893676592));
#32796=CARTESIAN_POINT('Ctrl Pts',(30.2723581529136,32.9448526619855,169.222763887372));
#32797=CARTESIAN_POINT('Ctrl Pts',(31.8567043568802,33.9639142708781,169.111634098152));
#32798=CARTESIAN_POINT('Ctrl Pts',(33.5721931794324,33.1856228367951,169.000504308933));
#32799=CARTESIAN_POINT('Ctrl Pts',(33.8488278539362,31.3222622400855,168.889374519713));
#32800=CARTESIAN_POINT('Ctrl Pts',(32.433435326133,30.0791598913592,168.778244730493));
#32801=CARTESIAN_POINT('Ctrl Pts',(30.6213674884419,30.5939895796832,168.667114941273));
#32802=CARTESIAN_POINT('Ctrl Pts',(30.0710091743181,32.3955847565919,168.555985152054));
#32803=CARTESIAN_POINT('Ctrl Pts',(31.2860423455642,33.8351450553073,168.444855362834));
#32804=CARTESIAN_POINT('Ctrl Pts',(33.1544818180945,33.5952004984823,168.333725573614));
#32805=CARTESIAN_POINT('Ctrl Pts',(33.966352053607,31.895345749241,168.222595784395));
#32806=CARTESIAN_POINT('Ctrl Pts',(32.9786382076115,30.291269426071,168.111465995175));
#32807=CARTESIAN_POINT('Ctrl Pts',(31.0952852996177,30.2510048126737,168.000336205955));
#32808=CARTESIAN_POINT('Ctrl Pts',(30.039917448298,31.8114015891261,167.889206416735));
#32809=CARTESIAN_POINT('Ctrl Pts',(30.7783959448026,33.544401664386,167.778076627515));
#32810=CARTESIAN_POINT('Ctrl Pts',(32.6348731175525,33.8639819250408,167.666946838296));
#32811=CARTESIAN_POINT('Ctrl Pts',(33.9103215165394,32.4776664670713,167.555817049076));
#32812=CARTESIAN_POINT('Ctrl Pts',(33.4374639352983,30.6541951765766,167.444687259857));
#32813=CARTESIAN_POINT('Ctrl Pts',(31.6490558548275,30.0623912134843,167.333557470637));
#32814=CARTESIAN_POINT('Ctrl Pts',(30.1818262062432,31.2438630556162,167.222427681417));
#32815=CARTESIAN_POINT('Ctrl Pts',(30.3785732505457,33.1173488152295,167.111297892197));
#32816=CARTESIAN_POINT('Ctrl Pts',(32.0592248292506,33.9682376837793,167.000168102978));
#32817=CARTESIAN_POINT('Ctrl Pts',(33.6856900471062,33.0178399222439,166.889038313758));
#32818=CARTESIAN_POINT('Ctrl Pts',(33.76939833431,31.1358789634033,166.777908524538));
#32819=CARTESIAN_POINT('Ctrl Pts',(32.2338369522489,30.0448481762927,166.666778735318));
#32820=CARTESIAN_POINT('Ctrl Pts',(30.484139214776,30.7429557473555,166.555648946099));
#32821=CARTESIAN_POINT('Ctrl Pts',(30.1220081713125,32.5918944065121,166.444519156879));
#32822=CARTESIAN_POINT('Ctrl Pts',(31.4780505358289,33.8983275199854,166.333389367659));
#32823=CARTESIAN_POINT('Ctrl Pts',(33.3128835277701,33.4690889075443,166.222259578439));
#32824=CARTESIAN_POINT('Ctrl Pts',(33.9439005615907,31.6919390350863,166.11112978922));
#32825=CARTESIAN_POINT('Ctrl Pts',(33.1815065089967,30.7013650994246,166.037043263073));
#32826=CARTESIAN_POINT('Ctrl Pts',(32.6750771856741,30.4769022377462,166.));
#32827=CARTESIAN_POINT('Ctrl Pts',(30.3361333853116,32.0009462961084,178.37851963661));
#32828=CARTESIAN_POINT('Ctrl Pts',(30.3350134449002,32.216507009066,178.364148625537));
#32829=CARTESIAN_POINT('Ctrl Pts',(30.373884681584,32.431680346969,178.349777614463));
#32830=CARTESIAN_POINT('Ctrl Pts',(30.4546197953249,32.6297920446191,178.33540660339));
#32831=CARTESIAN_POINT('Ctrl Pts',(30.6627256858759,33.140452268625,178.298363340316));
#32832=CARTESIAN_POINT('Ctrl Pts',(31.1489842701054,33.5377512483192,178.261320077243));
#32833=CARTESIAN_POINT('Ctrl Pts',(31.690876656062,33.639897472402,178.22427681417));
#32834=CARTESIAN_POINT('Ctrl Pts',(32.2327690420186,33.7420436964848,178.187233551097));
#32835=CARTESIAN_POINT('Ctrl Pts',(32.8302952297023,33.5490371649563,178.150190288023));
#32836=CARTESIAN_POINT('Ctrl Pts',(33.2100351911184,33.1491915376066,178.11314702495));
#32837=CARTESIAN_POINT('Ctrl Pts',(33.5897751525344,32.749345910257,178.076103761877));
#32838=CARTESIAN_POINT('Ctrl Pts',(33.7517288876827,32.1426611870862,178.039060498804));
#32839=CARTESIAN_POINT('Ctrl Pts',(33.6217849293405,31.6067555042284,178.002017235731));
#32840=CARTESIAN_POINT('Ctrl Pts',(33.4918409709983,31.0708498213705,177.964973972657));
#32841=CARTESIAN_POINT('Ctrl Pts',(33.0699993191655,30.6057231788256,177.927930709584));
#32842=CARTESIAN_POINT('Ctrl Pts',(32.5492935640385,30.4242137799862,177.890887446511));
#32843=CARTESIAN_POINT('Ctrl Pts',(32.0285878089115,30.2427043811468,177.853844183437));
#32844=CARTESIAN_POINT('Ctrl Pts',(31.4090179504904,30.344812226013,177.816800920364));
#32845=CARTESIAN_POINT('Ctrl Pts',(30.974095237716,30.6838139207111,177.779757657291));
#32846=CARTESIAN_POINT('Ctrl Pts',(30.5778854104528,30.9926407512105,177.746011650397));
#32847=CARTESIAN_POINT('Ctrl Pts',(30.3349144418051,31.4980660345814,177.712265643504));
#32848=CARTESIAN_POINT('Ctrl Pts',(30.3317667672262,32.0008552724323,177.67851963661));
#32849=CARTESIAN_POINT('Ctrl Pts',(31.4698297828098,30.0148256743287,179.));
#32850=CARTESIAN_POINT('Ctrl Pts',(31.4011717602422,30.0402471946251,179.));
#32851=CARTESIAN_POINT('Ctrl Pts',(31.3342170200572,30.0695594652625,179.));
#32852=CARTESIAN_POINT('Ctrl Pts',(31.2691543791405,30.1024681435714,179.));
#32853=CARTESIAN_POINT('Ctrl Pts',(31.2022750866749,30.1362956840811,179.));
#32854=CARTESIAN_POINT('Ctrl Pts',(31.1373942576578,30.173923959486,179.));
#32855=CARTESIAN_POINT('Ctrl Pts',(31.0747481851605,30.215077936283,179.));
#32856=CARTESIAN_POINT('Ctrl Pts',(31.0218169218836,30.2498499801463,179.));
#32857=CARTESIAN_POINT('Ctrl Pts',(30.9704813835458,30.287140070486,179.));
#32858=CARTESIAN_POINT('Ctrl Pts',(30.920906837578,30.3268003233183,179.));
#32859=CARTESIAN_POINT('Ctrl Pts',(30.8988714689694,30.3444288920366,179.));
#32860=CARTESIAN_POINT('Ctrl Pts',(30.8771843246632,30.3625259150697,179.));
#32861=CARTESIAN_POINT('Ctrl Pts',(30.8558614729043,30.381079129876,179.));
#32862=CARTESIAN_POINT('Ctrl Pts',(30.8441499657732,30.391269422899,179.));
#32863=CARTESIAN_POINT('Ctrl Pts',(30.8325483731912,30.401597342812,179.));
#32864=CARTESIAN_POINT('Ctrl Pts',(30.8210594917678,30.412060899429,179.));
#32865=CARTESIAN_POINT('Ctrl Pts',(30.8104646293746,30.4217102237116,179.));
#32866=CARTESIAN_POINT('Ctrl Pts',(30.7999641824858,30.4314764150215,179.));
#32867=CARTESIAN_POINT('Ctrl Pts',(30.7895762380615,30.4413424485534,179.));
#32868=CARTESIAN_POINT('Ctrl Pts',(30.7364925281002,30.4917591278393,179.));
#32869=CARTESIAN_POINT('Ctrl Pts',(30.6862488525372,30.5448645642236,179.));
#32870=CARTESIAN_POINT('Ctrl Pts',(30.6390638156957,30.6003988925952,179.));
#32871=CARTESIAN_POINT('Ctrl Pts',(30.5922436254276,30.6555038155712,179.));
#32872=CARTESIAN_POINT('Ctrl Pts',(30.5484344479305,30.7130010983928,179.));
#32873=CARTESIAN_POINT('Ctrl Pts',(30.5078946509714,30.7726610952581,179.));
#32874=CARTESIAN_POINT('Ctrl Pts',(30.4742099869881,30.8222328025285,179.));
#32875=CARTESIAN_POINT('Ctrl Pts',(30.4427831503197,30.8732983012023,179.));
#32876=CARTESIAN_POINT('Ctrl Pts',(30.4137899491081,30.9257323179221,179.));
#32877=CARTESIAN_POINT('Ctrl Pts',(30.4016832698065,30.9476271690731,179.));
#32878=CARTESIAN_POINT('Ctrl Pts',(30.3900012514895,30.9697606799659,179.));
#32879=CARTESIAN_POINT('Ctrl Pts',(30.3787581361903,30.9921238118577,179.));
#32880=CARTESIAN_POINT('Ctrl Pts',(30.3735598930403,31.0024633835934,179.));
#32881=CARTESIAN_POINT('Ctrl Pts',(30.3684554850874,31.0128520405776,179.));
#32882=CARTESIAN_POINT('Ctrl Pts',(30.3634463850541,31.0232888874584,179.));
#32883=CARTESIAN_POINT('Ctrl Pts',(30.3582116938596,31.0341957709509,179.));
#32884=CARTESIAN_POINT('Ctrl Pts',(30.3530846911292,31.0451478442412,179.));
#32885=CARTESIAN_POINT('Ctrl Pts',(30.348068454379,31.056139759175,179.));
#32886=CARTESIAN_POINT('Ctrl Pts',(30.3195275799257,31.118680440517,179.));
#32887=CARTESIAN_POINT('Ctrl Pts',(30.2945477318953,31.1825532780501,179.));
#32888=CARTESIAN_POINT('Ctrl Pts',(30.2733523356296,31.2475534440222,179.));
#32889=CARTESIAN_POINT('Ctrl Pts',(30.2541560446554,31.3064229307604,179.));
#32890=CARTESIAN_POINT('Ctrl Pts',(30.2380643124207,31.3662177179318,179.));
#32891=CARTESIAN_POINT('Ctrl Pts',(30.2252797771608,31.4267904453086,179.));
#32892=CARTESIAN_POINT('Ctrl Pts',(30.2101450523644,31.4984982970514,179.));
#32893=CARTESIAN_POINT('Ctrl Pts',(30.1996446092358,31.5712979137807,179.));
#32894=CARTESIAN_POINT('Ctrl Pts',(30.1937033974617,31.6447666213231,179.));
#32895=CARTESIAN_POINT('Ctrl Pts',(30.1923961005744,31.660932584822,179.));
#32896=CARTESIAN_POINT('Ctrl Pts',(30.1913097719617,31.6771308619873,179.));
#32897=CARTESIAN_POINT('Ctrl Pts',(30.1904439810637,31.6933567855583,179.));
#32898=CARTESIAN_POINT('Ctrl Pts',(30.1895460489563,31.7101850725971,179.));
#32899=CARTESIAN_POINT('Ctrl Pts',(30.1888853223853,31.7270493233257,179.));
#32900=CARTESIAN_POINT('Ctrl Pts',(30.1884618847505,31.7439099359327,179.));
#32901=CARTESIAN_POINT('Ctrl Pts',(30.1867401602096,31.8124662665857,179.));
#32902=CARTESIAN_POINT('Ctrl Pts',(30.1889297506264,31.881048937226,179.));
#32903=CARTESIAN_POINT('Ctrl Pts',(30.1949101630748,31.9493199653033,179.));
#32904=CARTESIAN_POINT('Ctrl Pts',(30.200889360023,32.017577117506,179.));
#32905=CARTESIAN_POINT('Ctrl Pts',(30.2106582916318,32.0855238245582,179.));
#32906=CARTESIAN_POINT('Ctrl Pts',(30.2241461415959,32.1528072679591,179.));
#32907=CARTESIAN_POINT('Ctrl Pts',(30.23390407838,32.2014842319721,179.));
#32908=CARTESIAN_POINT('Ctrl Pts',(30.2456095327489,32.2498137804381,179.));
#32909=CARTESIAN_POINT('Ctrl Pts',(30.2592498872082,32.2976526714744,179.));
#32910=CARTESIAN_POINT('Ctrl Pts',(30.2694853722893,32.3335501444441,179.));
#32911=CARTESIAN_POINT('Ctrl Pts',(30.2808105985582,32.3691711861731,179.));
#32912=CARTESIAN_POINT('Ctrl Pts',(30.293224150216,32.404451098837,179.));
#32913=CARTESIAN_POINT('Ctrl Pts',(30.2973533131521,32.4161863790998,179.));
#32914=CARTESIAN_POINT('Ctrl Pts',(30.3015996987641,32.4278747200823,179.));
#32915=CARTESIAN_POINT('Ctrl Pts',(30.3059626641326,32.4395135673061,179.));
#32916=CARTESIAN_POINT('Ctrl Pts',(30.3290856800155,32.5011975887183,179.));
#32917=CARTESIAN_POINT('Ctrl Pts',(30.3554815681533,32.561497971648,179.));
#32918=CARTESIAN_POINT('Ctrl Pts',(30.3851004076594,32.6200808955868,179.));
#32919=CARTESIAN_POINT('Ctrl Pts',(30.4059270031276,32.6612736930956,179.));
#32920=CARTESIAN_POINT('Ctrl Pts',(30.4283479615027,32.7016168064163,179.));
#32921=CARTESIAN_POINT('Ctrl Pts',(30.4523563217739,32.7409828457338,179.));
#32922=CARTESIAN_POINT('Ctrl Pts',(30.4600693931975,32.7536298182672,179.));
#32923=CARTESIAN_POINT('Ctrl Pts',(30.4679474569151,32.7661775460074,179.));
#32924=CARTESIAN_POINT('Ctrl Pts',(30.4759869702196,32.7786161898381,179.));
#32925=CARTESIAN_POINT('Ctrl Pts',(30.5102319100181,32.8315995724167,179.));
#32926=CARTESIAN_POINT('Ctrl Pts',(30.5473331969222,32.8824994972081,179.));
#32927=CARTESIAN_POINT('Ctrl Pts',(30.5872566572931,32.9310009671585,179.));
#32928=CARTESIAN_POINT('Ctrl Pts',(30.6240225851301,32.9756664727941,179.));
#32929=CARTESIAN_POINT('Ctrl Pts',(30.6631825179533,33.0182979966642,179.));
#32930=CARTESIAN_POINT('Ctrl Pts',(30.704731170499,33.0586167056725,179.));
#32931=CARTESIAN_POINT('Ctrl Pts',(30.7125728682978,33.066226269697,179.));
#32932=CARTESIAN_POINT('Ctrl Pts',(30.7204997080418,33.0737533451809,179.));
#32933=CARTESIAN_POINT('Ctrl Pts',(30.728510082833,33.081197258918,179.));
#32934=CARTESIAN_POINT('Origin',(32.,32.,172.));
#32935=CARTESIAN_POINT('Origin',(-32.,-32.,166.));
#32936=CARTESIAN_POINT('Ctrl Pts',(-31.3249228143252,-33.5230977622534,
166.));
#32937=CARTESIAN_POINT('Ctrl Pts',(-31.2652496657111,-33.5045147077491,
166.));
#32938=CARTESIAN_POINT('Ctrl Pts',(-31.2068892780268,-33.4823562231994,
166.));
#32939=CARTESIAN_POINT('Ctrl Pts',(-31.1499979698121,-33.4569214879221,
166.));
#32940=CARTESIAN_POINT('Ctrl Pts',(-31.1139308831639,-33.440796761142,166.));
#32941=CARTESIAN_POINT('Ctrl Pts',(-31.0784541858883,-33.4233541702623,
166.));
#32942=CARTESIAN_POINT('Ctrl Pts',(-31.0436086065906,-33.4046595162816,
166.));
#32943=CARTESIAN_POINT('Ctrl Pts',(-31.020037064781,-33.3920133836358,166.));
#32944=CARTESIAN_POINT('Ctrl Pts',(-30.9967543373406,-33.3787941494722,
166.));
#32945=CARTESIAN_POINT('Ctrl Pts',(-30.9737734827442,-33.3650202765066,
166.));
#32946=CARTESIAN_POINT('Ctrl Pts',(-30.9613024215807,-33.3575455844106,
166.));
#32947=CARTESIAN_POINT('Ctrl Pts',(-30.9489201683257,-33.3499073220363,
166.));
#32948=CARTESIAN_POINT('Ctrl Pts',(-30.9366413906613,-33.3421166398709,
166.));
#32949=CARTESIAN_POINT('Ctrl Pts',(-30.8809436659781,-33.3067773510422,
166.));
#32950=CARTESIAN_POINT('Ctrl Pts',(-30.82730918088,-33.2682678880975,166.));
#32951=CARTESIAN_POINT('Ctrl Pts',(-30.7759194947972,-33.2268911757215,
166.));
#32952=CARTESIAN_POINT('Ctrl Pts',(-30.738836022715,-33.1970331969088,166.));
#32953=CARTESIAN_POINT('Ctrl Pts',(-30.7029215593492,-33.1656809490029,
166.));
#32954=CARTESIAN_POINT('Ctrl Pts',(-30.6682496155875,-33.1329323650887,
166.));
#32955=CARTESIAN_POINT('Ctrl Pts',(-30.6588709943895,-33.124074004986,166.));
#32956=CARTESIAN_POINT('Ctrl Pts',(-30.6495833196648,-33.1151134090585,
166.));
#32957=CARTESIAN_POINT('Ctrl Pts',(-30.640388127734,-33.1060523678756,166.));
#32958=CARTESIAN_POINT('Ctrl Pts',(-30.6306794907576,-33.0964853724138,
166.));
#32959=CARTESIAN_POINT('Ctrl Pts',(-30.6210793827335,-33.0868116833964,
166.));
#32960=CARTESIAN_POINT('Ctrl Pts',(-30.6115938499237,-33.0770385931226,
166.));
#32961=CARTESIAN_POINT('Ctrl Pts',(-30.564337834939,-33.0283499944233,166.));
#32962=CARTESIAN_POINT('Ctrl Pts',(-30.5198880169309,-32.9771627809512,
166.));
#32963=CARTESIAN_POINT('Ctrl Pts',(-30.4784278661767,-32.9237844624066,
166.));
#32964=CARTESIAN_POINT('Ctrl Pts',(-30.4363632851573,-32.8696279635937,
166.));
#32965=CARTESIAN_POINT('Ctrl Pts',(-30.3973752864255,-32.8132154260561,
166.));
#32966=CARTESIAN_POINT('Ctrl Pts',(-30.361679837689,-32.7548210768249,166.));
#32967=CARTESIAN_POINT('Ctrl Pts',(-30.3395645388112,-32.7186425573852,
166.));
#32968=CARTESIAN_POINT('Ctrl Pts',(-30.3187136102408,-32.6817024296689,
166.));
#32969=CARTESIAN_POINT('Ctrl Pts',(-30.2991853292908,-32.6440586298174,
166.));
#32970=CARTESIAN_POINT('Ctrl Pts',(-30.2832062943298,-32.6132565538216,
166.));
#32971=CARTESIAN_POINT('Ctrl Pts',(-30.2681128991308,-32.5819832290257,
166.));
#32972=CARTESIAN_POINT('Ctrl Pts',(-30.2539403906387,-32.5502681863268,
166.));
#32973=CARTESIAN_POINT('Ctrl Pts',(-30.2481177635283,-32.5372383922343,
166.));
#32974=CARTESIAN_POINT('Ctrl Pts',(-30.2424496988302,-32.5241314966566,
166.));
#32975=CARTESIAN_POINT('Ctrl Pts',(-30.2369478542267,-32.5109721386666,
166.));
#32976=CARTESIAN_POINT('Ctrl Pts',(-30.2097573184397,-32.4459375875024,
166.));
#32977=CARTESIAN_POINT('Ctrl Pts',(-30.1865718984384,-32.379512851388,166.));
#32978=CARTESIAN_POINT('Ctrl Pts',(-30.167602992408,-32.3119935916337,166.));
#32979=CARTESIAN_POINT('Ctrl Pts',(-30.1654998512031,-32.3045075227436,
166.));
#32980=CARTESIAN_POINT('Ctrl Pts',(-30.1634485787457,-32.297007960316,166.));
#32981=CARTESIAN_POINT('Ctrl Pts',(-30.1614494913157,-32.2894952795695,
166.));
#32982=CARTESIAN_POINT('Ctrl Pts',(-30.144109446168,-32.2243304341649,166.));
#32983=CARTESIAN_POINT('Ctrl Pts',(-30.130691802039,-32.1581806460084,166.));
#32984=CARTESIAN_POINT('Ctrl Pts',(-30.1210426074296,-32.0913500757851,
166.));
#32985=CARTESIAN_POINT('Ctrl Pts',(-30.1106636454464,-32.0194651179478,
166.));
#32986=CARTESIAN_POINT('Ctrl Pts',(-30.1046440842174,-31.9467917171052,
166.));
#32987=CARTESIAN_POINT('Ctrl Pts',(-30.102852468024,-31.873685883042,166.));
#32988=CARTESIAN_POINT('Ctrl Pts',(-30.1025311821446,-31.8605760036622,
166.));
#32989=CARTESIAN_POINT('Ctrl Pts',(-30.1023460194269,-31.8474521833933,
166.));
#32990=CARTESIAN_POINT('Ctrl Pts',(-30.1022964301738,-31.8343164404446,
166.));
#32991=CARTESIAN_POINT('Ctrl Pts',(-30.102251899601,-31.8225206959586,166.));
#32992=CARTESIAN_POINT('Ctrl Pts',(-30.102316746396,-31.8107240263089,166.));
#32993=CARTESIAN_POINT('Ctrl Pts',(-30.1024900270227,-31.7989311721439,
166.));
#32994=CARTESIAN_POINT('Ctrl Pts',(-30.1035341466453,-31.7278721583389,
166.));
#32995=CARTESIAN_POINT('Ctrl Pts',(-30.1085110510928,-31.6569165693418,
166.));
#32996=CARTESIAN_POINT('Ctrl Pts',(-30.1172407253237,-31.5863996593262,
166.));
#32997=CARTESIAN_POINT('Ctrl Pts',(-30.1261541825071,-31.51439818006,166.));
#32998=CARTESIAN_POINT('Ctrl Pts',(-30.1389800306763,-31.442853110017,166.));
#32999=CARTESIAN_POINT('Ctrl Pts',(-30.1555793421879,-31.372105161476,166.));
#33000=CARTESIAN_POINT('Ctrl Pts',(-30.1722789678255,-31.3009296639604,
166.));
#33001=CARTESIAN_POINT('Ctrl Pts',(-30.1927978814359,-31.230559881898,166.));
#33002=CARTESIAN_POINT('Ctrl Pts',(-30.2170470200302,-31.1613418292143,
166.));
#33003=CARTESIAN_POINT('Ctrl Pts',(-30.2230312117698,-31.1442602286663,
166.));
#33004=CARTESIAN_POINT('Ctrl Pts',(-30.2292428199321,-31.1272488082428,
166.));
#33005=CARTESIAN_POINT('Ctrl Pts',(-30.2356809841796,-31.1103128783636,
166.));
#33006=CARTESIAN_POINT('Ctrl Pts',(-30.2407433191753,-31.0969961397381,
166.));
#33007=CARTESIAN_POINT('Ctrl Pts',(-30.2459464874926,-31.083724508723,166.));
#33008=CARTESIAN_POINT('Ctrl Pts',(-30.2512816614537,-31.0705206906996,
166.));
#33009=CARTESIAN_POINT('Ctrl Pts',(-30.2795038863081,-31.0006745856034,
166.));
#33010=CARTESIAN_POINT('Ctrl Pts',(-30.3114625623906,-30.932599286949,166.));
#33011=CARTESIAN_POINT('Ctrl Pts',(-30.3469997430835,-30.8666517028784,
166.));
#33012=CARTESIAN_POINT('Ctrl Pts',(-30.3825752356235,-30.8006330221788,
166.));
#33013=CARTESIAN_POINT('Ctrl Pts',(-30.4217371239017,-30.7367455318663,
166.));
#33014=CARTESIAN_POINT('Ctrl Pts',(-30.4643787139105,-30.6753517285781,
166.));
#33015=CARTESIAN_POINT('Ctrl Pts',(-30.5060510273331,-30.6153534543042,
166.));
#33016=CARTESIAN_POINT('Ctrl Pts',(-30.5510469857941,-30.5577358065873,
166.));
#33017=CARTESIAN_POINT('Ctrl Pts',(-30.5993123466261,-30.5028567349083,
166.));
#33018=CARTESIAN_POINT('Ctrl Pts',(-30.6096397636154,-30.4911141715577,
166.));
#33019=CARTESIAN_POINT('Ctrl Pts',(-30.620117024632,-30.479497094178,166.));
#33020=CARTESIAN_POINT('Ctrl Pts',(-30.6307438541099,-30.4680091959517,
166.));
#33021=CARTESIAN_POINT('Ctrl Pts',(-30.6398545489831,-30.4581602814009,
166.));
#33022=CARTESIAN_POINT('Ctrl Pts',(-30.649075180594,-30.4484063167597,166.));
#33023=CARTESIAN_POINT('Ctrl Pts',(-30.6584038878141,-30.4387477190139,
166.));
#33024=CARTESIAN_POINT('Ctrl Pts',(-31.6163320011535,-29.981387499008,166.));
#33025=CARTESIAN_POINT('Ctrl Pts',(-31.6906427498098,-29.9743675630937,
166.));
#33026=CARTESIAN_POINT('Ctrl Pts',(-31.7652022960126,-29.9717511873187,
166.));
#33027=CARTESIAN_POINT('Ctrl Pts',(-31.8396884569134,-29.9733742829586,
166.));
#33028=CARTESIAN_POINT('Ctrl Pts',(-31.9122243289139,-29.9749548806987,
166.));
#33029=CARTESIAN_POINT('Ctrl Pts',(-31.9846913912953,-29.9805565001925,
166.));
#33030=CARTESIAN_POINT('Ctrl Pts',(-32.0567789152228,-29.9900714754047,
166.));
#33031=CARTESIAN_POINT('Ctrl Pts',(-32.0728687041251,-29.9921951985434,
166.));
#33032=CARTESIAN_POINT('Ctrl Pts',(-32.088941631761,-29.9945143667354,166.));
#33033=CARTESIAN_POINT('Ctrl Pts',(-32.1049872983986,-29.9970269692978,
166.));
#33034=CARTESIAN_POINT('Ctrl Pts',(-32.1786235674407,-30.0085577260099,
166.));
#33035=CARTESIAN_POINT('Ctrl Pts',(-32.2515406107965,-30.0241342606475,
166.));
#33036=CARTESIAN_POINT('Ctrl Pts',(-32.3234063396469,-30.0436165375461,
166.));
#33037=CARTESIAN_POINT('Ctrl Pts',(-32.3738567729472,-30.0572932834295,
166.));
#33038=CARTESIAN_POINT('Ctrl Pts',(-32.423788826305,-30.0728959391103,166.));
#33039=CARTESIAN_POINT('Ctrl Pts',(-32.4730796706315,-30.090389199647,166.));
#33040=CARTESIAN_POINT('Ctrl Pts',(-32.4918010193241,-30.0970333834656,
166.));
#33041=CARTESIAN_POINT('Ctrl Pts',(-32.5104297849499,-30.1039504059982,
166.));
#33042=CARTESIAN_POINT('Ctrl Pts',(-32.5289589042585,-30.1111386947073,
166.));
#33043=CARTESIAN_POINT('Ctrl Pts',(-32.546660933288,-30.1180061174533,166.));
#33044=CARTESIAN_POINT('Ctrl Pts',(-32.5642774893601,-30.1251235901428,
166.));
#33045=CARTESIAN_POINT('Ctrl Pts',(-32.5817714522529,-30.1324764898979,
166.));
#33046=CARTESIAN_POINT('Ctrl Pts',(-32.6487029901528,-30.1606085313138,
166.));
#33047=CARTESIAN_POINT('Ctrl Pts',(-32.7139143733596,-30.192208709252,166.));
#33048=CARTESIAN_POINT('Ctrl Pts',(-32.7770972324966,-30.2271493585151,
166.));
#33049=CARTESIAN_POINT('Ctrl Pts',(-32.8389246041363,-30.2613404118613,
166.));
#33050=CARTESIAN_POINT('Ctrl Pts',(-32.89881025273,-30.2987307725668,166.));
#33051=CARTESIAN_POINT('Ctrl Pts',(-32.9564328602487,-30.3392376279317,
166.));
#33052=CARTESIAN_POINT('Ctrl Pts',(-33.0127911310432,-30.3788556949021,
166.));
#33053=CARTESIAN_POINT('Ctrl Pts',(-33.0669851431482,-30.4214555217774,
166.));
#33054=CARTESIAN_POINT('Ctrl Pts',(-33.1186738211267,-30.4669868293286,
166.));
#33055=CARTESIAN_POINT('Ctrl Pts',(-33.1354927563908,-30.4818022230307,
166.));
#33056=CARTESIAN_POINT('Ctrl Pts',(-33.1520460717911,-30.4969281821769,
166.));
#33057=CARTESIAN_POINT('Ctrl Pts',(-33.1683209144445,-30.5123634761981,
166.));
#33058=CARTESIAN_POINT('Ctrl Pts',(-33.1774555438763,-30.5210268896673,
166.));
#33059=CARTESIAN_POINT('Ctrl Pts',(-33.1865032709774,-30.5297887184969,
166.));
#33060=CARTESIAN_POINT('Ctrl Pts',(-33.1954493554731,-30.538636114803,166.));
#33061=CARTESIAN_POINT('Ctrl Pts',(-33.2440184737772,-30.5866694458182,
166.));
#33062=CARTESIAN_POINT('Ctrl Pts',(-33.2896825812191,-30.6373038648715,
166.));
#33063=CARTESIAN_POINT('Ctrl Pts',(-33.3321491427106,-30.6904579124732,
166.));
#33064=CARTESIAN_POINT('Ctrl Pts',(-33.3382530454572,-30.698097973871,166.));
#33065=CARTESIAN_POINT('Ctrl Pts',(-33.3442908157837,-30.7057901395772,
166.));
#33066=CARTESIAN_POINT('Ctrl Pts',(-33.3502615092167,-30.7135342161227,
166.));
#33067=CARTESIAN_POINT('Ctrl Pts',(-33.3926204742275,-30.7684744121174,
166.));
#33068=CARTESIAN_POINT('Ctrl Pts',(-33.4316074125864,-30.8260259901118,
166.));
#33069=CARTESIAN_POINT('Ctrl Pts',(-33.4671552055421,-30.8858271868844,
166.));
#33070=CARTESIAN_POINT('Ctrl Pts',(-33.5003164101228,-30.9416134834574,
166.));
#33071=CARTESIAN_POINT('Ctrl Pts',(-33.5304843566103,-30.999358447659,166.));
#33072=CARTESIAN_POINT('Ctrl Pts',(-33.557564843168,-31.0587738345715,166.));
#33073=CARTESIAN_POINT('Ctrl Pts',(-33.5634601879376,-31.0717083950244,
166.));
#33074=CARTESIAN_POINT('Ctrl Pts',(-33.569209065161,-31.0847221124707,166.));
#33075=CARTESIAN_POINT('Ctrl Pts',(-33.5748102571412,-31.097811985643,166.));
#33076=CARTESIAN_POINT('Ctrl Pts',(-33.5793367581237,-31.1083903275362,
166.));
#33077=CARTESIAN_POINT('Ctrl Pts',(-33.5837665821197,-31.1190180990339,
166.));
#33078=CARTESIAN_POINT('Ctrl Pts',(-33.588094067069,-31.1296806929919,166.));
#33079=CARTESIAN_POINT('Ctrl Pts',(-33.6138045316752,-31.1930293233811,
166.));
#33080=CARTESIAN_POINT('Ctrl Pts',(-33.6359574101316,-31.2577224771475,
166.));
#33081=CARTESIAN_POINT('Ctrl Pts',(-33.6545065508599,-31.3234105339755,
166.));
#33082=CARTESIAN_POINT('Ctrl Pts',(-33.6729704001367,-31.3887965482564,
166.));
#33083=CARTESIAN_POINT('Ctrl Pts',(-33.6878635838304,-31.455169472032,166.));
#33084=CARTESIAN_POINT('Ctrl Pts',(-33.699089518876,-31.5221871118774,166.));
#33085=CARTESIAN_POINT('Ctrl Pts',(-33.7100754114707,-31.5877717237873,
166.));
#33086=CARTESIAN_POINT('Ctrl Pts',(-33.7175490812715,-31.6539747381941,
166.));
#33087=CARTESIAN_POINT('Ctrl Pts',(-33.7213721137454,-31.7204625720356,
166.));
#33088=CARTESIAN_POINT('Ctrl Pts',(-33.7221759623023,-31.7344426126579,
166.));
#33089=CARTESIAN_POINT('Ctrl Pts',(-33.722818243567,-31.7484351706062,166.));
#33090=CARTESIAN_POINT('Ctrl Pts',(-33.7232974015415,-31.7624370101449,
166.));
#33091=CARTESIAN_POINT('Ctrl Pts',(-33.7237537916425,-31.7757735323356,
166.));
#33092=CARTESIAN_POINT('Ctrl Pts',(-33.7240620939902,-31.7891203356115,
166.));
#33093=CARTESIAN_POINT('Ctrl Pts',(-33.7242209861537,-31.8024529385825,
166.));
#33094=CARTESIAN_POINT('Ctrl Pts',(-33.7249995905293,-31.8677854432606,
166.));
#33095=CARTESIAN_POINT('Ctrl Pts',(-33.7221998286388,-31.9328937570084,
166.));
#33096=CARTESIAN_POINT('Ctrl Pts',(-33.7157435098322,-31.9974682783476,
166.));
#33097=CARTESIAN_POINT('Ctrl Pts',(-33.7094097670054,-32.0608168247216,
166.));
#33098=CARTESIAN_POINT('Ctrl Pts',(-33.6995568373319,-32.1236525228668,
166.));
#33099=CARTESIAN_POINT('Ctrl Pts',(-33.6860642400599,-32.1856659078437,
166.));
#33100=CARTESIAN_POINT('Ctrl Pts',(-33.6730092582277,-32.2456679665956,
166.));
#33101=CARTESIAN_POINT('Ctrl Pts',(-33.6565466410315,-32.304900812395,166.));
#33102=CARTESIAN_POINT('Ctrl Pts',(-33.6365261352111,-32.3630572331293,
166.));
#33103=CARTESIAN_POINT('Ctrl Pts',(-33.6332193402308,-32.3726629524795,
166.));
#33104=CARTESIAN_POINT('Ctrl Pts',(-33.6298153922485,-32.3822392325952,
166.));
#33105=CARTESIAN_POINT('Ctrl Pts',(-33.6263135082516,-32.3917845978604,
166.));
#33106=CARTESIAN_POINT('Ctrl Pts',(-33.6225506586299,-32.4020412979991,
166.));
#33107=CARTESIAN_POINT('Ctrl Pts',(-33.6186747312615,-32.4122623041161,
166.));
#33108=CARTESIAN_POINT('Ctrl Pts',(-33.6146867820778,-32.422446252051,166.));
#33109=CARTESIAN_POINT('Origin',(-32.,-32.,180.545925280538));
#33110=CARTESIAN_POINT('Ctrl Pts',(-34.0565967959177,-31.9984978779484,
178.795925280538));
#33111=CARTESIAN_POINT('Ctrl Pts',(-34.0574113092882,-31.9004036992395,
178.790592107115));
#33112=CARTESIAN_POINT('Ctrl Pts',(-34.0064252722628,-31.1217950158479,
178.748215670618));
#33113=CARTESIAN_POINT('Ctrl Pts',(-33.0117514577367,-29.791988463957,178.668795971049));
#33114=CARTESIAN_POINT('Ctrl Pts',(-30.6939036549736,-29.9525600728975,
178.557666181829));
#33115=CARTESIAN_POINT('Ctrl Pts',(-29.5714224639719,-31.9866392256298,
178.446536392609));
#33116=CARTESIAN_POINT('Ctrl Pts',(-30.6715287627672,-34.0330871086906,
178.33540660339));
#33117=CARTESIAN_POINT('Ctrl Pts',(-32.9874475184943,-34.2188064189366,
178.22427681417));
#33118=CARTESIAN_POINT('Ctrl Pts',(-34.0018726081791,-32.893590431192,178.144449706553));
#33119=CARTESIAN_POINT('Ctrl Pts',(-34.0573014417229,-32.1072447535499,
178.101665862009));
#33120=CARTESIAN_POINT('Ctrl Pts',(-34.0563934268478,-32.0016074868405,
178.095925280538));
#33121=CARTESIAN_POINT('Ctrl Pts',(-34.0526600126176,-32.0021813586275,
178.854074719462));
#33122=CARTESIAN_POINT('Ctrl Pts',(-34.0491237063947,-31.5321172985515,
178.828629953495));
#33123=CARTESIAN_POINT('Ctrl Pts',(-33.6567303178001,-30.3707973172003,
178.766141924455));
#33124=CARTESIAN_POINT('Ctrl Pts',(-31.7283973144122,-29.5870608054774,
178.666610632341));
#33125=CARTESIAN_POINT('Ctrl Pts',(-29.8255893685038,-30.9184850177167,
178.555480843121));
#33126=CARTESIAN_POINT('Ctrl Pts',(-29.9119598065434,-33.2405821817579,
178.444351053901));
#33127=CARTESIAN_POINT('Ctrl Pts',(-31.909683998457,-34.4268788699842,178.333221264681));
#33128=CARTESIAN_POINT('Ctrl Pts',(-33.720863198688,-33.5261195206734,178.236462486535));
#33129=CARTESIAN_POINT('Ctrl Pts',(-34.0499397495798,-32.4182643041283,
178.176746971462));
#33130=CARTESIAN_POINT('Ctrl Pts',(-34.0521188940875,-31.9988328896354,
178.154074719462));
#33131=CARTESIAN_POINT('Ctrl Pts',(-30.7309291201476,-30.9206413469516,
179.));
#33132=CARTESIAN_POINT('Ctrl Pts',(-30.3720428517593,-31.3426068457263,
178.962956736927));
#33133=CARTESIAN_POINT('Ctrl Pts',(-30.1149439884831,-32.5658740604652,
178.88887021078));
#33134=CARTESIAN_POINT('Ctrl Pts',(-31.4545463871115,-33.8932420431011,
178.777740421561));
#33135=CARTESIAN_POINT('Ctrl Pts',(-33.2939138023212,-33.4838688004809,
178.666610632341));
#33136=CARTESIAN_POINT('Ctrl Pts',(-33.9488255585344,-31.7184482261547,
178.555480843121));
#33137=CARTESIAN_POINT('Ctrl Pts',(-32.8203323657814,-30.2097348976529,
178.444351053901));
#33138=CARTESIAN_POINT('Ctrl Pts',(-30.9410115533208,-30.3399270380568,
178.333221264682));
#33139=CARTESIAN_POINT('Ctrl Pts',(-30.0308990509683,-31.9891670275699,
178.222091475462));
#33140=CARTESIAN_POINT('Ctrl Pts',(-30.9228698959826,-33.6484356360037,
178.110961686242));
#33141=CARTESIAN_POINT('Ctrl Pts',(-32.8006266289385,-33.7990176391037,
177.999831897022));
#33142=CARTESIAN_POINT('Ctrl Pts',(-33.9456545763016,-32.3031858052012,
177.888702107803));
#33143=CARTESIAN_POINT('Ctrl Pts',(-33.3100425086012,-30.5298680560717,
177.777572318583));
#33144=CARTESIAN_POINT('Ctrl Pts',(-31.4754927844203,-30.1020057762959,
177.666442529363));
#33145=CARTESIAN_POINT('Ctrl Pts',(-30.1209668471194,-31.4111639574702,
177.555312740144));
#33146=CARTESIAN_POINT('Ctrl Pts',(-30.4861114426254,-33.2592201050247,
177.444182950924));
#33147=CARTESIAN_POINT('Ctrl Pts',(-32.2367505420768,-33.9548508793836,
177.333053161704));
#33148=CARTESIAN_POINT('Ctrl Pts',(-33.770718057041,-32.8614237158023,177.221923372484));
#33149=CARTESIAN_POINT('Ctrl Pts',(-33.6841436362607,-30.9796307189992,
177.110793583265));
#33150=CARTESIAN_POINT('Ctrl Pts',(-32.0562592098835,-30.0316687161759,
176.999663794045));
#33151=CARTESIAN_POINT('Ctrl Pts',(-30.3768869713417,-30.8851021127453,
176.888534004825));
#33152=CARTESIAN_POINT('Ctrl Pts',(-30.1829701714511,-32.7588779877096,
176.777404215605));
#33153=CARTESIAN_POINT('Ctrl Pts',(-31.6519793673763,-33.9381369469389,
176.666274426386));
#33154=CARTESIAN_POINT('Ctrl Pts',(-33.4394932713683,-33.3436339959878,
176.555144637166));
#33155=CARTESIAN_POINT('Ctrl Pts',(-33.9095985444435,-31.5194517803416,
176.444014847946));
#33156=CARTESIAN_POINT('Ctrl Pts',(-32.6320599381888,-30.1350620853103,
176.332885058727));
#33157=CARTESIAN_POINT('Ctrl Pts',(-30.7760669310012,-30.457443344749,176.221755269507));
#33158=CARTESIAN_POINT('Ctrl Pts',(-30.0402041955143,-32.1915557270597,
176.110625480287));
#33159=CARTESIAN_POINT('Ctrl Pts',(-31.0979253272145,-33.7503583851451,
175.999495691067));
#33160=CARTESIAN_POINT('Ctrl Pts',(-32.9812154168446,-33.7072520310685,
175.888365901848));
#33161=CARTESIAN_POINT('Ctrl Pts',(-33.966507797822,-32.1016871324977,175.777236112628));
#33162=CARTESIAN_POINT('Ctrl Pts',(-33.1520735681191,-30.4030592730345,
175.666106323408));
#33163=CARTESIAN_POINT('Ctrl Pts',(-31.2832741025925,-30.1659342487801,
175.554976534188));
#33164=CARTESIAN_POINT('Ctrl Pts',(-30.0704144058039,-31.6073263104316,
175.443846744969));
#33165=CARTESIAN_POINT('Ctrl Pts',(-30.6234905193395,-33.4080890744052,
175.332716955749));
#33166=CARTESIAN_POINT('Ctrl Pts',(-32.4363331819517,-33.9201839875743,
175.221587166529));
#33167=CARTESIAN_POINT('Ctrl Pts',(-33.8498484482781,-32.6749473388432,
175.11045737731));
#33168=CARTESIAN_POINT('Ctrl Pts',(-33.5704024755114,-30.8120062051021,
174.99932758809));
#33169=CARTESIAN_POINT('Ctrl Pts',(-31.8537411874624,-30.0363041091952,
174.88819779887));
#33170=CARTESIAN_POINT('Ctrl Pts',(-30.270934378537,-31.0577551971577,174.77706800965));
#33171=CARTESIAN_POINT('Ctrl Pts',(-30.2705496754386,-32.9415385104621,
174.665938220431));
#33172=CARTESIAN_POINT('Ctrl Pts',(-31.8529391542711,-33.9636359895515,
174.554808431211));
#33173=CARTESIAN_POINT('Ctrl Pts',(-33.5699171243061,-33.188635105749,174.443678641991));
#33174=CARTESIAN_POINT('Ctrl Pts',(-33.8501239672185,-31.3258082633759,
174.332548852771));
#33175=CARTESIAN_POINT('Ctrl Pts',(-32.4371174190915,-30.0799943870563,
174.221419063552));
#33176=CARTESIAN_POINT('Ctrl Pts',(-30.6240657493529,-30.5913488261089,
174.110289274332));
#33177=CARTESIAN_POINT('Ctrl Pts',(-30.070254184421,-32.3918855433208,173.999159485112));
#33178=CARTESIAN_POINT('Ctrl Pts',(-31.2825250626851,-33.8337728611072,
173.888029695892));
#33179=CARTESIAN_POINT('Ctrl Pts',(-33.151421222888,-33.5974111428469,173.776899906673));
#33180=CARTESIAN_POINT('Ctrl Pts',(-33.9665491665471,-31.8991160698556,
173.665770117453));
#33181=CARTESIAN_POINT('Ctrl Pts',(-32.98191263932,-30.2931488756918,173.554640328233));
#33182=CARTESIAN_POINT('Ctrl Pts',(-31.0986403129863,-30.2492733204651,
173.443510539014));
#33183=CARTESIAN_POINT('Ctrl Pts',(-30.0402825973689,-31.8076438365085,
173.332380749794));
#33184=CARTESIAN_POINT('Ctrl Pts',(-30.7754369963891,-33.5420566273636,
173.221250960574));
#33185=CARTESIAN_POINT('Ctrl Pts',(-32.6312981764812,-33.8651959157632,
173.110121171355));
#33186=CARTESIAN_POINT('Ctrl Pts',(-33.9094021116014,-32.4813281292638,
172.998991382135));
#33187=CARTESIAN_POINT('Ctrl Pts',(-33.4400419407876,-30.6569540586483,
172.887861592915));
#33188=CARTESIAN_POINT('Ctrl Pts',(-31.6527710023696,-30.0617210688312,
172.776731803695));
#33189=CARTESIAN_POINT('Ctrl Pts',(-30.1832802770412,-31.24037993706,172.665602014476));
#33190=CARTESIAN_POINT('Ctrl Pts',(-30.3764317406597,-33.1142348491549,
172.554472225256));
#33191=CARTESIAN_POINT('Ctrl Pts',(-32.0554552683619,-33.968354110677,172.443342436036));
#33192=CARTESIAN_POINT('Ctrl Pts',(-33.6837267358465,-33.021057036019,172.332212646816));
#33193=CARTESIAN_POINT('Ctrl Pts',(-33.7710697539406,-31.1392996348988,
172.221082857597));
#33194=CARTESIAN_POINT('Ctrl Pts',(-32.2375489396799,-30.0452458740124,
172.109953068377));
#33195=CARTESIAN_POINT('Ctrl Pts',(-30.4866259119352,-30.7401618908041,
171.998823279157));
#33196=CARTESIAN_POINT('Ctrl Pts',(-30.1207264377287,-32.5880680827564,
171.887693489937));
#33197=CARTESIAN_POINT('Ctrl Pts',(-31.4747177478399,-33.8977807427029,
171.776563700718));
#33198=CARTESIAN_POINT('Ctrl Pts',(-33.3094416786791,-33.4706650475028,
171.665433911498));
#33199=CARTESIAN_POINT('Ctrl Pts',(-33.9457787854949,-31.6976126495265,
171.554304122278));
#33200=CARTESIAN_POINT('Ctrl Pts',(-32.8013602489181,-30.2013018754492,
171.443174333058));
#33201=CARTESIAN_POINT('Ctrl Pts',(-30.9235455029214,-30.3511401188919,
171.332044543839));
#33202=CARTESIAN_POINT('Ctrl Pts',(-30.0308902389882,-32.0099970443839,
171.220914754619));
#33203=CARTESIAN_POINT('Ctrl Pts',(-30.9403428742268,-33.6597047832692,
171.109784965399));
#33204=CARTESIAN_POINT('Ctrl Pts',(-32.81958221947,-33.7904687032553,170.99865517618));
#33205=CARTESIAN_POINT('Ctrl Pts',(-33.9487488054533,-32.2826150828469,
170.88752538696));
#33206=CARTESIAN_POINT('Ctrl Pts',(-33.2944416179866,-30.5161152034498,
170.77639559774));
#33207=CARTESIAN_POINT('Ctrl Pts',(-31.4554754993733,-30.107650597795,170.66526580852));
#33208=CARTESIAN_POINT('Ctrl Pts',(-30.1148522986113,-31.4310436433634,
170.554136019301));
#33209=CARTESIAN_POINT('Ctrl Pts',(-30.4994958305847,-33.2751393764509,
170.443006230081));
#33210=CARTESIAN_POINT('Ctrl Pts',(-32.2573845061169,-33.9522413805212,
170.331876440861));
#33211=CARTESIAN_POINT('Ctrl Pts',(-33.7797176728697,-32.8426732443147,
170.220746651642));
#33212=CARTESIAN_POINT('Ctrl Pts',(-33.6732725256466,-30.9618996933222,
170.109616862422));
#33213=CARTESIAN_POINT('Ctrl Pts',(-32.0354665088367,-30.0311842852721,
169.998487073202));
#33214=CARTESIAN_POINT('Ctrl Pts',(-30.3652019277577,-30.9023076684237,
169.887357283982));
#33215=CARTESIAN_POINT('Ctrl Pts',(-30.191086813748,-32.7780271694562,169.776227494763));
#33216=CARTESIAN_POINT('Ctrl Pts',(-31.6724694309494,-33.9417046423557,
169.665097705543));
#33217=CARTESIAN_POINT('Ctrl Pts',(-33.453604473025,-33.3283550834814,169.553967916323));
#33218=CARTESIAN_POINT('Ctrl Pts',(-33.9044164650717,-31.4993093576157,
169.442838127103));
#33219=CARTESIAN_POINT('Ctrl Pts',(-32.6123271608224,-30.1284902778966,
169.331708337884));
#33220=CARTESIAN_POINT('Ctrl Pts',(-30.759842679398,-30.4704566001679,169.220578548664));
#33221=CARTESIAN_POINT('Ctrl Pts',(-30.0423367288465,-32.2122444547597,
169.109448759444));
#33222=CARTESIAN_POINT('Ctrl Pts',(-31.1164629740721,-33.7597884860473,
168.998318970225));
#33223=CARTESIAN_POINT('Ctrl Pts',(-32.9991927238842,-33.6967931790227,
168.887189181005));
#33224=CARTESIAN_POINT('Ctrl Pts',(-33.9674721285561,-32.0809111554984,
168.776059391785));
#33225=CARTESIAN_POINT('Ctrl Pts',(-33.135142377592,-30.3909801199351,168.664929602566));
#33226=CARTESIAN_POINT('Ctrl Pts',(-31.263942632616,-30.1736066294559,168.553799813346));
#33227=CARTESIAN_POINT('Ctrl Pts',(-30.0663746083578,-31.627728545404,168.442670024126));
#33228=CARTESIAN_POINT('Ctrl Pts',(-30.6384395726302,-33.4225492592449,
168.331540234906));
#33229=CARTESIAN_POINT('Ctrl Pts',(-32.4565898757574,-33.9154683184132,
168.220410445686));
#33230=CARTESIAN_POINT('Ctrl Pts',(-33.8568740735902,-32.6553715439732,
168.109280656467));
#33231=CARTESIAN_POINT('Ctrl Pts',(-33.557767261349,-30.7954858417039,167.998150867247));
#33232=CARTESIAN_POINT('Ctrl Pts',(-31.8330087343896,-30.0379584306098,
167.887021078027));
#33233=CARTESIAN_POINT('Ctrl Pts',(-30.2610788239753,-31.0760701946845,
167.775891288807));
#33234=CARTESIAN_POINT('Ctrl Pts',(-30.2805906728734,-32.9597524800475,
167.664761499588));
#33235=CARTESIAN_POINT('Ctrl Pts',(-31.8736873796365,-33.9650797382332,
167.553631710368));
#33236=CARTESIAN_POINT('Ctrl Pts',(-33.5823838477932,-33.1719872601882,
167.442501921148));
#33237=CARTESIAN_POINT('Ctrl Pts',(-33.8429001430549,-31.3063048942249,
167.331372131929));
#33238=CARTESIAN_POINT('Ctrl Pts',(-32.4168134709511,-30.0754844752405,
167.220242342709));
#33239=CARTESIAN_POINT('Ctrl Pts',(-30.6092651408375,-30.6059603865314,
167.109112553489));
#33240=CARTESIAN_POINT('Ctrl Pts',(-30.0744991966179,-32.4122450279571,
166.99798276427));
#33241=CARTESIAN_POINT('Ctrl Pts',(-31.3019369679044,-33.8412499466342,
166.88685297505));
#33242=CARTESIAN_POINT('Ctrl Pts',(-33.1682217075247,-33.5851578807299,
166.77572318583));
#33243=CARTESIAN_POINT('Ctrl Pts',(-33.9653885654801,-31.8783566947692,
166.66459339661));
#33244=CARTESIAN_POINT('Ctrl Pts',(-32.9638002744564,-30.2828614116132,
166.553463607391));
#33245=CARTESIAN_POINT('Ctrl Pts',(-31.0802600234891,-30.2589149518813,
166.442333818171));
#33246=CARTESIAN_POINT('Ctrl Pts',(-30.0382367488593,-31.8283047073915,
166.331204028951));
#33247=CARTESIAN_POINT('Ctrl Pts',(-30.7920439879536,-33.5550031292294,
166.220074239731));
#33248=CARTESIAN_POINT('Ctrl Pts',(-32.6504510705939,-33.8582230624016,
166.108944450512));
#33249=CARTESIAN_POINT('Ctrl Pts',(-33.9154261036092,-32.461549476428,165.997814661292));
#33250=CARTESIAN_POINT('Ctrl Pts',(-33.423606114718,-30.6409579664333,165.886684872072));
#33251=CARTESIAN_POINT('Ctrl Pts',(-32.2331222331378,-30.2598665970074,
165.812598345926));
#33252=CARTESIAN_POINT('Ctrl Pts',(-31.6889203620497,-30.3633004372052,
165.775555082853));
#33253=CARTESIAN_POINT('Ctrl Pts',(-30.6322193753411,-30.8366876301903,
179.074814972382));
#33254=CARTESIAN_POINT('Ctrl Pts',(-30.2454185337564,-31.2914740748732,
179.037771709309));
#33255=CARTESIAN_POINT('Ctrl Pts',(-29.9683222348862,-32.6098883743919,
178.963685183163));
#33256=CARTESIAN_POINT('Ctrl Pts',(-31.4121203983139,-34.0405005153411,
178.852555393943));
#33257=CARTESIAN_POINT('Ctrl Pts',(-33.3945558572736,-33.5992857665047,
178.741425604723));
#33258=CARTESIAN_POINT('Ctrl Pts',(-34.1004073784384,-31.6965488159742,
178.630295815504));
#33259=CARTESIAN_POINT('Ctrl Pts',(-32.8841387297665,-30.0704860864209,
178.519166026284));
#33260=CARTESIAN_POINT('Ctrl Pts',(-30.8586422538717,-30.2108047163371,
178.408036237064));
#33261=CARTESIAN_POINT('Ctrl Pts',(-29.8777401886362,-31.9883244269232,
178.296906447844));
#33262=CARTESIAN_POINT('Ctrl Pts',(-30.8390895182441,-33.776652793566,178.185776658625));
#33263=CARTESIAN_POINT('Ctrl Pts',(-32.8629002587904,-33.9389472323813,
178.074646869405));
#33264=CARTESIAN_POINT('Ctrl Pts',(-34.09698975368,-32.3267679344073,177.963517080185));
#33265=CARTESIAN_POINT('Ctrl Pts',(-33.4119390722704,-30.415519558032,177.852387290965));
#33266=CARTESIAN_POINT('Ctrl Pts',(-31.4346960297071,-29.954377674162,177.741257501746));
#33267=CARTESIAN_POINT('Ctrl Pts',(-29.9748135581674,-31.3653636350345,
177.630127712526));
#33268=CARTESIAN_POINT('Ctrl Pts',(-30.3683595065151,-33.3571636456066,
177.518997923306));
#33269=CARTESIAN_POINT('Ctrl Pts',(-32.2551652626115,-34.1069013554461,
177.407868134087));
#33270=CARTESIAN_POINT('Ctrl Pts',(-33.9084464773441,-32.9284262107039,
177.296738344867));
#33271=CARTESIAN_POINT('Ctrl Pts',(-33.8151382018061,-30.9002652612182,
177.185608555647));
#33272=CARTESIAN_POINT('Ctrl Pts',(-32.0606351138136,-29.8785697192598,
177.074478766427));
#33273=CARTESIAN_POINT('Ctrl Pts',(-30.2506394343487,-30.7983841148121,
176.963348977208));
#33274=CARTESIAN_POINT('Ctrl Pts',(-30.0416395700409,-32.8179043618037,
176.852219187988));
#33275=CARTESIAN_POINT('Ctrl Pts',(-31.624909935417,-34.0888873947425,176.741089398768));
#33276=CARTESIAN_POINT('Ctrl Pts',(-33.5514586593724,-33.4481433429146,
176.629959609548));
#33277=CARTESIAN_POINT('Ctrl Pts',(-34.0581292435536,-31.4820742052332,
176.518829820329));
#33278=CARTESIAN_POINT('Ctrl Pts',(-32.681222263313,-29.9900051396649,176.407700031109));
#33279=CARTESIAN_POINT('Ctrl Pts',(-30.6808680553363,-30.3374615720942,
176.296570241889));
#33280=CARTESIAN_POINT('Ctrl Pts',(-29.8877690976764,-32.2064551446055,
176.18544045267));
#33281=CARTESIAN_POINT('Ctrl Pts',(-31.0277609556569,-33.8865032075191,
176.07431066345));
#33282=CARTESIAN_POINT('Ctrl Pts',(-33.0575354435149,-33.8400439932689,
175.96318087423));
#33283=CARTESIAN_POINT('Ctrl Pts',(-34.1194649619683,-32.1095964707848,
175.85205108501));
#33284=CARTESIAN_POINT('Ctrl Pts',(-33.2416831318658,-30.2788474467825,
175.740921295791));
#33285=CARTESIAN_POINT('Ctrl Pts',(-31.227526364974,-30.0232785743529,175.629791506571));
#33286=CARTESIAN_POINT('Ctrl Pts',(-29.9203290917295,-31.5767837140291,
175.518661717351));
#33287=CARTESIAN_POINT('Ctrl Pts',(-30.5164240806426,-33.517611809034,175.407531928132));
#33288=CARTESIAN_POINT('Ctrl Pts',(-32.4702716622405,-34.0695380342269,
175.296402138912));
#33289=CARTESIAN_POINT('Ctrl Pts',(-33.9937317184398,-32.7274454937002,
175.185272349692));
#33290=CARTESIAN_POINT('Ctrl Pts',(-33.692550127043,-30.7196027261572,175.074142560472));
#33291=CARTESIAN_POINT('Ctrl Pts',(-31.8423650143184,-29.8835656583048,
174.963012771252));
#33292=CARTESIAN_POINT('Ctrl Pts',(-30.1364457310092,-30.9844663481972,
174.851882982033));
#33293=CARTESIAN_POINT('Ctrl Pts',(-30.136031105276,-33.0147724232156,174.740753192813));
#33294=CARTESIAN_POINT('Ctrl Pts',(-31.8415005980932,-34.1163697812558,
174.629623403593));
#33295=CARTESIAN_POINT('Ctrl Pts',(-33.692027024681,-33.2810884665653,174.518493614374));
#33296=CARTESIAN_POINT('Ctrl Pts',(-33.9940286675499,-31.2733688801001,
174.407363825154));
#33297=CARTESIAN_POINT('Ctrl Pts',(-32.4711168982175,-29.930654214581,174.296234035934));
#33298=CARTESIAN_POINT('Ctrl Pts',(-30.5170440526865,-30.4817823707567,
174.185104246715));
#33299=CARTESIAN_POINT('Ctrl Pts',(-29.9201564081492,-32.4223668368314,
174.073974457495));
#33300=CARTESIAN_POINT('Ctrl Pts',(-31.2267190639093,-33.9764057542155,
173.962844668275));
#33301=CARTESIAN_POINT('Ctrl Pts',(-33.240980046497,-33.7216595585696,173.851714879055));
#33302=CARTESIAN_POINT('Ctrl Pts',(-34.1195095483989,-31.8912692055412,
173.740585089835));
#33303=CARTESIAN_POINT('Ctrl Pts',(-33.05828689673,-30.1603880964652,173.629455300616));
#33304=CARTESIAN_POINT('Ctrl Pts',(-31.0285315538174,-30.1130998517438,
173.518325511396));
#33305=CARTESIAN_POINT('Ctrl Pts',(-29.8878535977144,-31.7926821601266,
173.407195722177));
#33306=CARTESIAN_POINT('Ctrl Pts',(-30.6801891237093,-33.661999507293,173.296065932957));
#33307=CARTESIAN_POINT('Ctrl Pts',(-32.6804012509324,-34.0102729290192,
173.184936143737));
#33308=CARTESIAN_POINT('Ctrl Pts',(-34.0579175319466,-32.518766366609,173.073806354517));
#33309=CARTESIAN_POINT('Ctrl Pts',(-33.5520500049095,-30.5524904512653,
172.962676565297));
#33310=CARTESIAN_POINT('Ctrl Pts',(-31.6257631446607,-29.9109595773362,
172.851546776078));
#33311=CARTESIAN_POINT('Ctrl Pts',(-30.0419737959887,-31.181295843529,172.740416986858));
#33312=CARTESIAN_POINT('Ctrl Pts',(-30.2501487953179,-33.2009012752471,
172.629287197638));
#33313=CARTESIAN_POINT('Ctrl Pts',(-32.059768640826,-34.1214548830912,172.518157408419));
#33314=CARTESIAN_POINT('Ctrl Pts',(-33.814688874414,-33.1004759881503,172.407027619199));
#33315=CARTESIAN_POINT('Ctrl Pts',(-33.9088255296197,-31.0723534030195,
172.295897829979));
#33316=CARTESIAN_POINT('Ctrl Pts',(-32.2560257604683,-29.8932029235367,
172.184768040759));
#33317=CARTESIAN_POINT('Ctrl Pts',(-30.3689139918201,-30.6421702811702,
172.07363825154));
#33318=CARTESIAN_POINT('Ctrl Pts',(-29.9745544494668,-32.6338086724266,
171.96250846232));
#33319=CARTESIAN_POINT('Ctrl Pts',(-31.4338607099192,-34.045392240047,171.8513786731));
#33320=CARTESIAN_POINT('Ctrl Pts',(-33.4112915091286,-33.5850550109315,
171.74024888388));
#33321=CARTESIAN_POINT('Ctrl Pts',(-34.0971236240025,-31.6740926250174,
171.629119094661));
#33322=CARTESIAN_POINT('Ctrl Pts',(-32.8636909405481,-30.0613971343689,
171.517989305441));
#33323=CARTESIAN_POINT('Ctrl Pts',(-30.8398176746423,-30.2228899630735,
171.406859516221));
#33324=CARTESIAN_POINT('Ctrl Pts',(-29.8777306912504,-32.0107746256172,
171.295729727001));
#33325=CARTESIAN_POINT('Ctrl Pts',(-30.8579215641739,-33.7887984676421,
171.184599937782));
#33326=CARTESIAN_POINT('Ctrl Pts',(-32.8833302362405,-33.9297333507925,
171.073470148562));
#33327=CARTESIAN_POINT('Ctrl Pts',(-34.1003246554173,-32.3045971983844,
170.962340359343));
#33328=CARTESIAN_POINT('Ctrl Pts',(-33.3951247270286,-30.4006969932339,
170.851210570123));
#33329=CARTESIAN_POINT('Ctrl Pts',(-31.413121777961,-29.9604615561569,170.740080780903));
#33330=CARTESIAN_POINT('Ctrl Pts',(-29.9682234132741,-31.3867895850116,
170.628950991683));
#33331=CARTESIAN_POINT('Ctrl Pts',(-30.3827849470592,-33.3743211356737,
170.517821202464));
#33332=CARTESIAN_POINT('Ctrl Pts',(-32.2774041593287,-34.1040888868593,
170.406691413244));
#33333=CARTESIAN_POINT('Ctrl Pts',(-33.9181460933034,-32.9082173066851,
170.295561624024));
#33334=CARTESIAN_POINT('Ctrl Pts',(-33.803421524115,-30.8811550966393,170.184431834804));
#33335=CARTESIAN_POINT('Ctrl Pts',(-32.0382251333486,-29.8780476087814,
170.073302045585));
#33336=CARTESIAN_POINT('Ctrl Pts',(-30.2380455150758,-30.8169279377514,
169.962172256365));
#33337=CARTESIAN_POINT('Ctrl Pts',(-30.050387533805,-32.838542988209,169.851042467145));
#33338=CARTESIAN_POINT('Ctrl Pts',(-31.6469937389289,-34.0927325894777,
169.739912677925));
#33339=CARTESIAN_POINT('Ctrl Pts',(-33.5666674459918,-33.4316760195965,
169.628782888706));
#33340=CARTESIAN_POINT('Ctrl Pts',(-34.0525440962835,-31.4603650824602,
169.517653099486));
#33341=CARTESIAN_POINT('Ctrl Pts',(-32.6599546485714,-29.9829221697599,
169.406523310266));
#33342=CARTESIAN_POINT('Ctrl Pts',(-30.6633818633947,-30.3514870129961,
169.295393521047));
#33343=CARTESIAN_POINT('Ctrl Pts',(-29.8900675018235,-32.2287530645612,
169.184263731827));
#33344=CARTESIAN_POINT('Ctrl Pts',(-31.0477404813091,-33.89666679216,169.073133942607));
#33345=CARTESIAN_POINT('Ctrl Pts',(-33.0769110454948,-33.8287716400761,
168.962004153387));
#33346=CARTESIAN_POINT('Ctrl Pts',(-34.1205042994196,-32.0872045151823,
168.850874364168));
#33347=CARTESIAN_POINT('Ctrl Pts',(-33.2234350145046,-30.2658287637176,
168.739744574948));
#33348=CARTESIAN_POINT('Ctrl Pts',(-31.2066912717576,-30.0315477213328,
168.628614785728));
#33349=CARTESIAN_POINT('Ctrl Pts',(-29.915975074344,-31.598772857534,168.517484996508));
#33350=CARTESIAN_POINT('Ctrl Pts',(-30.5325358879284,-33.5331967231367,
168.406355207289));
#33351=CARTESIAN_POINT('Ctrl Pts',(-32.4921039442249,-34.0644555750725,
168.295225418069));
#33352=CARTESIAN_POINT('Ctrl Pts',(-34.0013038047043,-32.7063470717282,
168.184095628849));
#33353=CARTESIAN_POINT('Ctrl Pts',(-33.6789321318671,-30.7017973905159,
168.07296583963));
#33354=CARTESIAN_POINT('Ctrl Pts',(-31.8200199679818,-29.8853486546794,
167.96183605041));
#33355=CARTESIAN_POINT('Ctrl Pts',(-30.12582360045,-31.0042059066059,167.85070626119));
#33356=CARTESIAN_POINT('Ctrl Pts',(-30.1468531026612,-33.0344030956174,
167.73957647197));
#33357=CARTESIAN_POINT('Ctrl Pts',(-31.8638626435088,-34.1179258263161,
167.628446682751));
#33358=CARTESIAN_POINT('Ctrl Pts',(-33.7054634237896,-33.263145733057,167.517316893531));
#33359=CARTESIAN_POINT('Ctrl Pts',(-33.9862429663067,-31.2523485172001,
167.406187104311));
#33360=CARTESIAN_POINT('Ctrl Pts',(-32.4492336864037,-29.9257935168071,
167.295057315092));
#33361=CARTESIAN_POINT('Ctrl Pts',(-30.5010922363758,-30.4975304346034,
167.183927525872));
#33362=CARTESIAN_POINT('Ctrl Pts',(-29.9247316021171,-32.4443099048315,
167.072797736652));
#33363=CARTESIAN_POINT('Ctrl Pts',(-31.2476408487112,-33.9844644157726,
166.961667947432));
#33364=CARTESIAN_POINT('Ctrl Pts',(-33.2590872915183,-33.7084532240939,
166.850538158213));
#33365=CARTESIAN_POINT('Ctrl Pts',(-34.1182586744898,-31.8688951431669,
166.739408368993));
#33366=CARTESIAN_POINT('Ctrl Pts',(-33.0387657319783,-30.1493004619863,
166.628278579773));
#33367=CARTESIAN_POINT('Ctrl Pts',(-31.008721624956,-30.1234914199773,166.517148790553));
#33368=CARTESIAN_POINT('Ctrl Pts',(-29.8856486208318,-31.8149500565308,
166.406019001334));
#33369=CARTESIAN_POINT('Ctrl Pts',(-30.698087825552,-33.6759530024763,166.294889212114));
#33370=CARTESIAN_POINT('Ctrl Pts',(-32.7010438784557,-34.0027577193661,
166.183759422894));
#33371=CARTESIAN_POINT('Ctrl Pts',(-34.0644100767541,-32.4974493081529,
166.072629633674));
#33372=CARTESIAN_POINT('Ctrl Pts',(-33.5343357820042,-30.535250165203,165.961499844455));
#33373=CARTESIAN_POINT('Ctrl Pts',(-32.2512547397669,-30.12451708512,165.887413318308));
#33374=CARTESIAN_POINT('Ctrl Pts',(-31.664724241751,-30.2359961244728,165.850370055235));
#33375=CARTESIAN_POINT('Ctrl Pts',(-30.5335096305347,-30.7527339134291,
179.149629944765));
#33376=CARTESIAN_POINT('Ctrl Pts',(-30.1187942157535,-31.24034130402,179.112586681692));
#33377=CARTESIAN_POINT('Ctrl Pts',(-29.8217004812893,-32.6539026883187,
179.038500155545));
#33378=CARTESIAN_POINT('Ctrl Pts',(-31.3696944095162,-34.187758987581,178.927370366326));
#33379=CARTESIAN_POINT('Ctrl Pts',(-33.4951979122261,-33.7147027325285,
178.816240577106));
#33380=CARTESIAN_POINT('Ctrl Pts',(-34.2519891983425,-31.6746494057936,
178.705110787886));
#33381=CARTESIAN_POINT('Ctrl Pts',(-32.9479450937516,-29.9312372751889,
178.593980998666));
#33382=CARTESIAN_POINT('Ctrl Pts',(-30.7762729544227,-30.0816823946173,
178.482851209447));
#33383=CARTESIAN_POINT('Ctrl Pts',(-29.724581326304,-31.9874818262765,178.371721420227));
#33384=CARTESIAN_POINT('Ctrl Pts',(-30.7553091405056,-33.9048699511283,
178.260591631007));
#33385=CARTESIAN_POINT('Ctrl Pts',(-32.9251738886423,-34.078876825659,178.149461841787));
#33386=CARTESIAN_POINT('Ctrl Pts',(-34.2483249310584,-32.3503500636134,
178.038332052568));
#33387=CARTESIAN_POINT('Ctrl Pts',(-33.5138356359396,-30.3011710599924,
177.927202263348));
#33388=CARTESIAN_POINT('Ctrl Pts',(-31.3938992749938,-29.8067495720281,
177.816072474128));
#33389=CARTESIAN_POINT('Ctrl Pts',(-29.8286602692153,-31.3195633125989,
177.704942684908));
#33390=CARTESIAN_POINT('Ctrl Pts',(-30.2506075704047,-33.4551071861885,
177.593812895689));
#33391=CARTESIAN_POINT('Ctrl Pts',(-32.2735799831462,-34.2589518315086,
177.482683106469));
#33392=CARTESIAN_POINT('Ctrl Pts',(-34.0461748976471,-32.9954287056055,
177.371553317249));
#33393=CARTESIAN_POINT('Ctrl Pts',(-33.9461327673516,-30.8208998034373,
177.26042352803));
#33394=CARTESIAN_POINT('Ctrl Pts',(-32.0650110177436,-29.7254707223437,
177.14929373881));
#33395=CARTESIAN_POINT('Ctrl Pts',(-30.1243918973557,-30.7116661168789,
177.03816394959));
#33396=CARTESIAN_POINT('Ctrl Pts',(-29.9003089686307,-32.8769307358977,
176.92703416037));
#33397=CARTESIAN_POINT('Ctrl Pts',(-31.5978405034577,-34.2396378425461,
176.815904371151));
#33398=CARTESIAN_POINT('Ctrl Pts',(-33.6634240473765,-33.5526526898415,
176.704774581931));
#33399=CARTESIAN_POINT('Ctrl Pts',(-34.2066599426637,-31.4446966301247,
176.593644792711));
#33400=CARTESIAN_POINT('Ctrl Pts',(-32.7303845884373,-29.8449481940195,
176.482515003492));
#33401=CARTESIAN_POINT('Ctrl Pts',(-30.5856691796714,-30.2174797994394,
176.371385214272));
#33402=CARTESIAN_POINT('Ctrl Pts',(-29.7353339998384,-32.2213545621514,
176.260255425052));
#33403=CARTESIAN_POINT('Ctrl Pts',(-30.9575965840992,-34.0226480298931,
176.149125635832));
#33404=CARTESIAN_POINT('Ctrl Pts',(-33.1338554701853,-33.9728359554694,
176.037995846613));
#33405=CARTESIAN_POINT('Ctrl Pts',(-34.2724221261146,-32.1175058090718,
175.926866057393));
#33406=CARTESIAN_POINT('Ctrl Pts',(-33.3312926956126,-30.1546356205304,
175.815736268173));
#33407=CARTESIAN_POINT('Ctrl Pts',(-31.1717786273556,-29.8806228999258,
175.704606478953));
#33408=CARTESIAN_POINT('Ctrl Pts',(-29.7702437776551,-31.5462411176266,
175.593476689734));
#33409=CARTESIAN_POINT('Ctrl Pts',(-30.4093576419459,-33.6271345436629,
175.482346900514));
#33410=CARTESIAN_POINT('Ctrl Pts',(-32.5042101425294,-34.2188920808795,
175.371217111294));
#33411=CARTESIAN_POINT('Ctrl Pts',(-34.1376149886015,-32.7799436485572,
175.260087322074));
#33412=CARTESIAN_POINT('Ctrl Pts',(-33.8146977785746,-30.6271992472123,
175.148957532855));
#33413=CARTESIAN_POINT('Ctrl Pts',(-31.8309888411744,-29.7308272074143,
175.037827743635));
#33414=CARTESIAN_POINT('Ctrl Pts',(-30.0019570834814,-30.9111774992366,
174.926697954415));
#33415=CARTESIAN_POINT('Ctrl Pts',(-30.0015125351133,-33.0880063359691,
174.815568165196));
#33416=CARTESIAN_POINT('Ctrl Pts',(-31.8300620419152,-34.2691035729601,
174.704438375976));
#33417=CARTESIAN_POINT('Ctrl Pts',(-33.814136925056,-33.3735418273816,174.593308586756));
#33418=CARTESIAN_POINT('Ctrl Pts',(-34.1379333678812,-31.2209294968243,
174.482178797536));
#33419=CARTESIAN_POINT('Ctrl Pts',(-32.5051163773435,-29.7813140421056,
174.371049008317));
#33420=CARTESIAN_POINT('Ctrl Pts',(-30.41002235602,-30.3722159154045,174.259919219097));
#33421=CARTESIAN_POINT('Ctrl Pts',(-29.7700586318775,-32.452848130342,174.148789429877));
#33422=CARTESIAN_POINT('Ctrl Pts',(-31.1709130651335,-34.1190386473239,
174.037659640657));
#33423=CARTESIAN_POINT('Ctrl Pts',(-33.330538870106,-33.8459079742922,173.926529851438));
#33424=CARTESIAN_POINT('Ctrl Pts',(-34.2724699302506,-31.8834223412267,
173.815400062218));
#33425=CARTESIAN_POINT('Ctrl Pts',(-33.1346611541401,-30.0276273172385,
173.704270272998));
#33426=CARTESIAN_POINT('Ctrl Pts',(-30.9584227946484,-29.9769263830225,
173.593140483779));
#33427=CARTESIAN_POINT('Ctrl Pts',(-29.73542459806,-31.7777204837445,173.482010694559));
#33428=CARTESIAN_POINT('Ctrl Pts',(-30.5849412510295,-33.7819423872226,
173.370880905339));
#33429=CARTESIAN_POINT('Ctrl Pts',(-32.7295043253836,-34.155349942275,173.259751116119));
#33430=CARTESIAN_POINT('Ctrl Pts',(-34.2064329522917,-32.5562046039542,
173.1486213269));
#33431=CARTESIAN_POINT('Ctrl Pts',(-33.6640580690314,-30.4480268438822,
173.03749153768));
#33432=CARTESIAN_POINT('Ctrl Pts',(-31.5987552869518,-29.7601980858412,
172.92636174846));
#33433=CARTESIAN_POINT('Ctrl Pts',(-29.9006673149363,-31.122211749998,172.815231959241));
#33434=CARTESIAN_POINT('Ctrl Pts',(-30.123865849976,-33.2875677013394,172.704102170021));
#33435=CARTESIAN_POINT('Ctrl Pts',(-32.0640820132901,-34.2745556555053,
172.592972380801));
#33436=CARTESIAN_POINT('Ctrl Pts',(-33.9456510129815,-33.1798949402817,
172.481842591581));
#33437=CARTESIAN_POINT('Ctrl Pts',(-34.0465813052989,-31.0054071711401,
172.370712802362));
#33438=CARTESIAN_POINT('Ctrl Pts',(-32.2745025812568,-29.741159973061,172.259583013142));
#33439=CARTESIAN_POINT('Ctrl Pts',(-30.251202071705,-30.5441786715364,172.148453223922));
#33440=CARTESIAN_POINT('Ctrl Pts',(-29.828382461205,-32.6795492620968,172.037323434702));
#33441=CARTESIAN_POINT('Ctrl Pts',(-31.3930036719987,-34.1930037373911,
171.926193645483));
#33442=CARTESIAN_POINT('Ctrl Pts',(-33.513141339578,-33.6994449743603,171.815063856263));
#33443=CARTESIAN_POINT('Ctrl Pts',(-34.2484684625102,-31.6505726005082,
171.703934067043));
#33444=CARTESIAN_POINT('Ctrl Pts',(-32.9260216321781,-29.9214923932887,
171.592804277823));
#33445=CARTESIAN_POINT('Ctrl Pts',(-30.7560898463631,-30.0946398072549,
171.481674488604));
#33446=CARTESIAN_POINT('Ctrl Pts',(-29.7245711435126,-32.0115522068506,
171.370544699384));
#33447=CARTESIAN_POINT('Ctrl Pts',(-30.775500254121,-33.917892152015,171.259414910165));
#33448=CARTESIAN_POINT('Ctrl Pts',(-32.947078253011,-34.0689979983296,171.148285120944));
#33449=CARTESIAN_POINT('Ctrl Pts',(-34.2519005053813,-32.326579313922,171.037155331725));
#33450=CARTESIAN_POINT('Ctrl Pts',(-33.4958078360707,-30.2852787830181,
170.926025542505));
#33451=CARTESIAN_POINT('Ctrl Pts',(-31.3707680565487,-29.8132725145188,
170.814895753286));
#33452=CARTESIAN_POINT('Ctrl Pts',(-29.821594527937,-31.3425355266598,170.703765964066));
#33453=CARTESIAN_POINT('Ctrl Pts',(-30.2660740635338,-33.4735028948964,
170.592636174846));
#33454=CARTESIAN_POINT('Ctrl Pts',(-32.2974238125406,-34.2559363931974,
170.481506385626));
#33455=CARTESIAN_POINT('Ctrl Pts',(-34.0565745137372,-32.9737613690555,
170.370376596407));
#33456=CARTESIAN_POINT('Ctrl Pts',(-33.9335705225834,-30.8004104999564,
170.259246807187));
#33457=CARTESIAN_POINT('Ctrl Pts',(-32.0409837578605,-29.7249109322907,
170.148117017967));
#33458=CARTESIAN_POINT('Ctrl Pts',(-30.1108891023939,-30.731548207079,170.036987228747));
#33459=CARTESIAN_POINT('Ctrl Pts',(-29.9096882538619,-32.8990588069617,
169.925857439528));
#33460=CARTESIAN_POINT('Ctrl Pts',(-31.6215180469084,-34.2437605365997,
169.814727650308));
#33461=CARTESIAN_POINT('Ctrl Pts',(-33.6797304189587,-33.5349969557116,
169.703597861088));
#33462=CARTESIAN_POINT('Ctrl Pts',(-34.2006717274953,-31.4214208073048,
169.592468071868));
#33463=CARTESIAN_POINT('Ctrl Pts',(-32.7075821363205,-29.837354061623,169.481338282649));
#33464=CARTESIAN_POINT('Ctrl Pts',(-30.5669210473915,-30.2325174258244,
169.370208493429));
#33465=CARTESIAN_POINT('Ctrl Pts',(-29.7377982748005,-32.2452616743627,
169.259078704209));
#33466=CARTESIAN_POINT('Ctrl Pts',(-30.9790179885462,-34.0335450982727,
169.14794891499));
#33467=CARTESIAN_POINT('Ctrl Pts',(-33.1546293671055,-33.9607501011295,
169.03681912577));
#33468=CARTESIAN_POINT('Ctrl Pts',(-34.2735364702832,-32.0934978748662,
168.92568933655));
#33469=CARTESIAN_POINT('Ctrl Pts',(-33.3117276514171,-30.1406774075,168.81455954733));
#33470=CARTESIAN_POINT('Ctrl Pts',(-31.1494399108992,-29.8894888132097,
168.703429758111));
#33471=CARTESIAN_POINT('Ctrl Pts',(-29.7655755403302,-31.569817169664,168.592299968891));
#33472=CARTESIAN_POINT('Ctrl Pts',(-30.4266322032265,-33.6438441870286,
168.481170179671));
#33473=CARTESIAN_POINT('Ctrl Pts',(-32.5276180126925,-34.2134428317317,
168.370040390452));
#33474=CARTESIAN_POINT('Ctrl Pts',(-34.1457335358184,-32.7573225994832,
168.258910601232));
#33475=CARTESIAN_POINT('Ctrl Pts',(-33.8000970023852,-30.6081089393279,
168.147780812012));
#33476=CARTESIAN_POINT('Ctrl Pts',(-31.807031201574,-29.7327388787489,168.036651022792));
#33477=CARTESIAN_POINT('Ctrl Pts',(-29.9905683769247,-30.9323416185274,
167.925521233573));
#33478=CARTESIAN_POINT('Ctrl Pts',(-30.013115532449,-33.1090537111873,167.814391444353));
#33479=CARTESIAN_POINT('Ctrl Pts',(-31.8540379073811,-34.2707719143989,
167.703261655133));
#33480=CARTESIAN_POINT('Ctrl Pts',(-33.8285429997859,-33.3543042059258,
167.592131865913));
#33481=CARTESIAN_POINT('Ctrl Pts',(-34.1295857895586,-31.1983921401753,
167.481002076694));
#33482=CARTESIAN_POINT('Ctrl Pts',(-32.4816539018563,-29.7761025583737,
167.369872287474));
#33483=CARTESIAN_POINT('Ctrl Pts',(-30.3929193319141,-30.3891004826755,
167.258742498254));
#33484=CARTESIAN_POINT('Ctrl Pts',(-29.7749640076164,-32.4763747817059,
167.147612709034));
#33485=CARTESIAN_POINT('Ctrl Pts',(-31.1933447295181,-34.1276788849111,
167.036482919815));
#33486=CARTESIAN_POINT('Ctrl Pts',(-33.349952875512,-33.8317485674581,166.925353130595));
#33487=CARTESIAN_POINT('Ctrl Pts',(-34.2711287834995,-31.8594335915646,
166.814223341375));
#33488=CARTESIAN_POINT('Ctrl Pts',(-33.1137311895003,-30.0157395123594,
166.703093552156));
#33489=CARTESIAN_POINT('Ctrl Pts',(-30.9371832264228,-29.9880678880733,
166.591963762936));
#33490=CARTESIAN_POINT('Ctrl Pts',(-29.7330604928044,-31.8015954056701,
166.480833973716));
#33491=CARTESIAN_POINT('Ctrl Pts',(-30.6041316631504,-33.7969028757232,
166.369704184496));
#33492=CARTESIAN_POINT('Ctrl Pts',(-32.7516366863175,-34.1472923763307,
166.258574395277));
#33493=CARTESIAN_POINT('Ctrl Pts',(-34.213394049899,-32.5333491398779,166.147444606057));
#33494=CARTESIAN_POINT('Ctrl Pts',(-33.6450654492904,-30.4295423639727,
166.036314816837));
#33495=CARTESIAN_POINT('Ctrl Pts',(-32.2693872463961,-29.9891675732325,
165.962228290691));
#33496=CARTESIAN_POINT('Ctrl Pts',(-31.6405281214523,-30.1086918117404,
165.925185027618));
#33497=CARTESIAN_POINT('Ctrl Pts',(-30.4347998857282,-30.6687801966679,
179.224444917147));
#33498=CARTESIAN_POINT('Ctrl Pts',(-29.9921698977506,-31.1892085331669,
179.187401654074));
#33499=CARTESIAN_POINT('Ctrl Pts',(-29.6750787276925,-32.6979170022453,
179.113315127928));
#33500=CARTESIAN_POINT('Ctrl Pts',(-31.3272684207187,-34.3350174598211,
179.002185338708));
#33501=CARTESIAN_POINT('Ctrl Pts',(-33.5958399671785,-33.8301196985523,
178.891055549488));
#33502=CARTESIAN_POINT('Ctrl Pts',(-34.4035710182465,-31.6527499956131,
178.779925760269));
#33503=CARTESIAN_POINT('Ctrl Pts',(-33.0117514577367,-29.791988463957,178.668795971049));
#33504=CARTESIAN_POINT('Ctrl Pts',(-30.6939036549736,-29.9525600728975,
178.557666181829));
#33505=CARTESIAN_POINT('Ctrl Pts',(-29.5714224639719,-31.9866392256298,
178.446536392609));
#33506=CARTESIAN_POINT('Ctrl Pts',(-30.6715287627672,-34.0330871086906,
178.33540660339));
#33507=CARTESIAN_POINT('Ctrl Pts',(-32.9874475184943,-34.2188064189366,
178.22427681417));
#33508=CARTESIAN_POINT('Ctrl Pts',(-34.3996601084368,-32.3739321928194,
178.11314702495));
#33509=CARTESIAN_POINT('Ctrl Pts',(-33.6157321996089,-30.1868225619527,
178.002017235731));
#33510=CARTESIAN_POINT('Ctrl Pts',(-31.3531025202806,-29.6591214698943,
177.890887446511));
#33511=CARTESIAN_POINT('Ctrl Pts',(-29.6825069802633,-31.2737629901632,
177.779757657291));
#33512=CARTESIAN_POINT('Ctrl Pts',(-30.1328556342944,-33.5530507267704,
177.668627868071));
#33513=CARTESIAN_POINT('Ctrl Pts',(-32.2919947036809,-34.4110023075711,
177.557498078851));
#33514=CARTESIAN_POINT('Ctrl Pts',(-34.1839033179502,-33.062431200507,177.446368289632));
#33515=CARTESIAN_POINT('Ctrl Pts',(-34.0771273328971,-30.7415343456564,
177.335238500412));
#33516=CARTESIAN_POINT('Ctrl Pts',(-32.0693869216736,-29.5723717254276,
177.224108711192));
#33517=CARTESIAN_POINT('Ctrl Pts',(-29.9981443603627,-30.6249481189457,
177.112978921973));
#33518=CARTESIAN_POINT('Ctrl Pts',(-29.7589783672204,-32.9359571099918,
177.001849132753));
#33519=CARTESIAN_POINT('Ctrl Pts',(-31.5707710714985,-34.3903882903498,
176.890719343533));
#33520=CARTESIAN_POINT('Ctrl Pts',(-33.7753894353805,-33.6571620367683,
176.779589554314));
#33521=CARTESIAN_POINT('Ctrl Pts',(-34.3551906417739,-31.4073190550162,
176.668459765094));
#33522=CARTESIAN_POINT('Ctrl Pts',(-32.7795469135615,-29.6998912483741,
176.557329975874));
#33523=CARTESIAN_POINT('Ctrl Pts',(-30.4904703040065,-30.0974980267845,
176.446200186654));
#33524=CARTESIAN_POINT('Ctrl Pts',(-29.5828989020006,-32.2362539796973,
176.335070397435));
#33525=CARTESIAN_POINT('Ctrl Pts',(-30.8874322125415,-34.1587928522671,
176.223940608215));
#33526=CARTESIAN_POINT('Ctrl Pts',(-33.2101754968556,-34.1056279176698,
176.112810818995));
#33527=CARTESIAN_POINT('Ctrl Pts',(-34.4253792902609,-32.1254151473588,
176.001681029775));
#33528=CARTESIAN_POINT('Ctrl Pts',(-33.4209022593593,-30.0304237942783,
175.890551240556));
#33529=CARTESIAN_POINT('Ctrl Pts',(-31.116030889737,-29.7379672254987,175.779421451336));
#33530=CARTESIAN_POINT('Ctrl Pts',(-29.6201584635808,-31.5156985212241,
175.668291662116));
#33531=CARTESIAN_POINT('Ctrl Pts',(-30.302291203249,-33.7366572782917,175.557161872896));
#33532=CARTESIAN_POINT('Ctrl Pts',(-32.5381486228183,-34.368246127532,175.446032083677));
#33533=CARTESIAN_POINT('Ctrl Pts',(-34.2814982587632,-32.8324418034142,
175.334902294457));
#33534=CARTESIAN_POINT('Ctrl Pts',(-33.9368454301063,-30.5347957682674,
175.223772505237));
#33535=CARTESIAN_POINT('Ctrl Pts',(-31.8196126680302,-29.5780887565239,
175.112642716018));
#33536=CARTESIAN_POINT('Ctrl Pts',(-29.8674684359538,-30.837888650276,175.001512926798));
#33537=CARTESIAN_POINT('Ctrl Pts',(-29.8669939649505,-33.1612402487227,
174.890383137578));
#33538=CARTESIAN_POINT('Ctrl Pts',(-31.8186234857374,-34.4218373646645,
174.779253348358));
#33539=CARTESIAN_POINT('Ctrl Pts',(-33.936246825431,-33.4659951881979,174.668123559139));
#33540=CARTESIAN_POINT('Ctrl Pts',(-34.2818380682126,-31.1684901135484,
174.556993769919));
#33541=CARTESIAN_POINT('Ctrl Pts',(-32.5391158564695,-29.6319738696303,
174.445863980699));
#33542=CARTESIAN_POINT('Ctrl Pts',(-30.3030006593535,-30.2626494600523,
174.334734191479));
#33543=CARTESIAN_POINT('Ctrl Pts',(-29.6199608556057,-32.4833294238526,
174.22360440226));
#33544=CARTESIAN_POINT('Ctrl Pts',(-31.1151070663578,-34.2616715404322,
174.11247461304));
#33545=CARTESIAN_POINT('Ctrl Pts',(-33.420097693715,-33.9701563900148,174.00134482382));
#33546=CARTESIAN_POINT('Ctrl Pts',(-34.4254303121024,-31.8755754769123,
173.890215034601));
#33547=CARTESIAN_POINT('Ctrl Pts',(-33.2110354115502,-29.8948665380118,
173.779085245381));
#33548=CARTESIAN_POINT('Ctrl Pts',(-30.8883140354794,-29.8407529143012,
173.667955456161));
#33549=CARTESIAN_POINT('Ctrl Pts',(-29.5829955984056,-31.7627588073625,
173.556825666941));
#33550=CARTESIAN_POINT('Ctrl Pts',(-30.4896933783496,-33.9018852671521,
173.445695877722));
#33551=CARTESIAN_POINT('Ctrl Pts',(-32.7786073998349,-34.3004269555309,
173.334566088502));
#33552=CARTESIAN_POINT('Ctrl Pts',(-34.3549483726368,-32.5936428412994,
173.223436299282));
#33553=CARTESIAN_POINT('Ctrl Pts',(-33.7760661331533,-30.3435632364992,
173.112306510063));
#33554=CARTESIAN_POINT('Ctrl Pts',(-31.571747429243,-29.6094365943462,173.001176720843));
#33555=CARTESIAN_POINT('Ctrl Pts',(-29.7593608338838,-31.063127656467,172.890046931623));
#33556=CARTESIAN_POINT('Ctrl Pts',(-29.9975829046342,-33.3742341274316,
172.778917142403));
#33557=CARTESIAN_POINT('Ctrl Pts',(-32.0683953857542,-34.4276564279194,
172.667787353184));
#33558=CARTESIAN_POINT('Ctrl Pts',(-34.076613151549,-33.2593138924131,172.556657563964));
#33559=CARTESIAN_POINT('Ctrl Pts',(-34.184337080978,-30.9384609392607,172.445527774744));
#33560=CARTESIAN_POINT('Ctrl Pts',(-32.2929794020452,-29.5891170225852,
172.334397985524));
#33561=CARTESIAN_POINT('Ctrl Pts',(-30.1334901515899,-30.4461870619026,
172.223268196305));
#33562=CARTESIAN_POINT('Ctrl Pts',(-29.6822104729431,-32.7252898517669,
172.112138407085));
#33563=CARTESIAN_POINT('Ctrl Pts',(-31.352146634078,-34.3406152347352,172.001008617865));
#33564=CARTESIAN_POINT('Ctrl Pts',(-33.6149911700275,-33.813834937789,171.889878828645));
#33565=CARTESIAN_POINT('Ctrl Pts',(-34.3998133010178,-31.6270525759992,
171.778749039426));
#33566=CARTESIAN_POINT('Ctrl Pts',(-32.9883523238082,-29.7815876522084,
171.667619250206));
#33567=CARTESIAN_POINT('Ctrl Pts',(-30.6723620180839,-29.9663896514365,
171.556489460986));
#33568=CARTESIAN_POINT('Ctrl Pts',(-29.5714115957749,-32.0123297880839,
171.445359671767));
#33569=CARTESIAN_POINT('Ctrl Pts',(-30.6930789440682,-34.046985836388,171.334229882547));
#33570=CARTESIAN_POINT('Ctrl Pts',(-33.0108262697815,-34.2082626458667,
171.223100093327));
#33571=CARTESIAN_POINT('Ctrl Pts',(-34.4034763553453,-32.3485614294596,
171.111970304107));
#33572=CARTESIAN_POINT('Ctrl Pts',(-33.5964909451128,-30.1698605728022,
171.000840514888));
#33573=CARTESIAN_POINT('Ctrl Pts',(-31.3284143351364,-29.6660834728807,
170.889710725668));
#33574=CARTESIAN_POINT('Ctrl Pts',(-29.6749656425999,-31.298281468308,170.778580936448));
#33575=CARTESIAN_POINT('Ctrl Pts',(-30.1493631800083,-33.5726846541191,
170.667451147229));
#33576=CARTESIAN_POINT('Ctrl Pts',(-32.3174434657525,-34.4077838995354,
170.556321358009));
#33577=CARTESIAN_POINT('Ctrl Pts',(-34.195002934171,-33.0393054314259,170.445191568789));
#33578=CARTESIAN_POINT('Ctrl Pts',(-34.0637195210518,-30.7196659032736,
170.334061779569));
#33579=CARTESIAN_POINT('Ctrl Pts',(-32.0437423823724,-29.5717742558001,
170.22293199035));
#33580=CARTESIAN_POINT('Ctrl Pts',(-29.983732689712,-30.6461684764067,170.11180220113));
#33581=CARTESIAN_POINT('Ctrl Pts',(-29.7689889739188,-32.9595746257144,
170.00067241191));
#33582=CARTESIAN_POINT('Ctrl Pts',(-31.5960423548879,-34.3947884837217,
169.88954262269));
#33583=CARTESIAN_POINT('Ctrl Pts',(-33.7927933919256,-33.6383178918267,
169.778412833471));
#33584=CARTESIAN_POINT('Ctrl Pts',(-34.3487993587072,-31.3824765321494,
169.667283044251));
#33585=CARTESIAN_POINT('Ctrl Pts',(-32.7552096240695,-29.6917859534862,
169.556153255031));
#33586=CARTESIAN_POINT('Ctrl Pts',(-30.4704602313883,-30.1135478386525,
169.445023465812));
#33587=CARTESIAN_POINT('Ctrl Pts',(-29.5855290477775,-32.2617702841642,
169.333893676592));
#33588=CARTESIAN_POINT('Ctrl Pts',(-30.9102954957832,-34.1704234043853,
169.222763887372));
#33589=CARTESIAN_POINT('Ctrl Pts',(-33.2323476887161,-34.0927285621829,
169.111634098152));
#33590=CARTESIAN_POINT('Ctrl Pts',(-34.4265686411468,-32.09979123455,169.000504308932));
#33591=CARTESIAN_POINT('Ctrl Pts',(-33.4000202883296,-30.0155260512825,
168.889374519713));
#33592=CARTESIAN_POINT('Ctrl Pts',(-31.0921885500407,-29.7474299050867,
168.778244730493));
#33593=CARTESIAN_POINT('Ctrl Pts',(-29.6151760063164,-31.540861481794,168.667114941273));
#33594=CARTESIAN_POINT('Ctrl Pts',(-30.3207285185246,-33.7544916509204,
168.555985152054));
#33595=CARTESIAN_POINT('Ctrl Pts',(-32.56313208116,-34.3624300883911,168.444855362834));
#33596=CARTESIAN_POINT('Ctrl Pts',(-34.2901632669325,-32.8082981272383,
168.333725573614));
#33597=CARTESIAN_POINT('Ctrl Pts',(-33.9212618729032,-30.5144204881399,
168.222595784395));
#33598=CARTESIAN_POINT('Ctrl Pts',(-31.7940424351662,-29.5801291028184,
168.111465995175));
#33599=CARTESIAN_POINT('Ctrl Pts',(-29.8553131533993,-30.8604773304489,
168.000336205955));
#33600=CARTESIAN_POINT('Ctrl Pts',(-29.8793779622368,-33.1837043267573,
167.889206416735));
#33601=CARTESIAN_POINT('Ctrl Pts',(-31.8442131712534,-34.4236180024818,
167.778076627516));
#33602=CARTESIAN_POINT('Ctrl Pts',(-33.9516225757822,-33.4454626787946,
167.666946838296));
#33603=CARTESIAN_POINT('Ctrl Pts',(-34.2729286128104,-31.1444357631505,
167.555817049076));
#33604=CARTESIAN_POINT('Ctrl Pts',(-32.514074117309,-29.6264115999403,167.444687259856));
#33605=CARTESIAN_POINT('Ctrl Pts',(-30.2847464274524,-30.2806705307475,
167.333557470637));
#33606=CARTESIAN_POINT('Ctrl Pts',(-29.6251964131156,-32.5084396585803,
167.222427681417));
#33607=CARTESIAN_POINT('Ctrl Pts',(-31.139048610325,-34.2708933540495,167.111297892197));
#33608=CARTESIAN_POINT('Ctrl Pts',(-33.4408184595056,-33.9550439108221,
167.000168102978));
#33609=CARTESIAN_POINT('Ctrl Pts',(-34.4239988925092,-31.8499720399622,
166.889038313758));
#33610=CARTESIAN_POINT('Ctrl Pts',(-33.1886966470223,-29.8821785627325,
166.777908524538));
#33611=CARTESIAN_POINT('Ctrl Pts',(-30.8656448278897,-29.8526443561693,
166.666778735318));
#33612=CARTESIAN_POINT('Ctrl Pts',(-29.580472364777,-31.7882407548095,166.555648946099));
#33613=CARTESIAN_POINT('Ctrl Pts',(-30.5101755007489,-33.9178527489701,
166.444519156879));
#33614=CARTESIAN_POINT('Ctrl Pts',(-32.8022294941794,-34.2918270332952,
166.333389367659));
#33615=CARTESIAN_POINT('Ctrl Pts',(-34.3623780230438,-32.5692489716029,
166.222259578439));
#33616=CARTESIAN_POINT('Ctrl Pts',(-33.7557951165766,-30.3238345627424,
166.11112978922));
#33617=CARTESIAN_POINT('Ctrl Pts',(-32.2875197530252,-29.8538180613451,
166.037043263073));
#33618=CARTESIAN_POINT('Ctrl Pts',(-31.6163320011535,-29.981387499008,166.));
#33619=CARTESIAN_POINT('Ctrl Pts',(-30.7309291201476,-30.9206413469516,
179.));
#33620=CARTESIAN_POINT('Ctrl Pts',(-30.6856062030546,-30.962922818334,179.));
#33621=CARTESIAN_POINT('Ctrl Pts',(-30.6430136434112,-31.0077738784331,
179.));
#33622=CARTESIAN_POINT('Ctrl Pts',(-30.6031497132239,-31.0548493830004,
179.));
#33623=CARTESIAN_POINT('Ctrl Pts',(-30.5606495403132,-31.1050380391255,
179.));
#33624=CARTESIAN_POINT('Ctrl Pts',(-30.5212500994078,-31.1577553100502,
179.));
#33625=CARTESIAN_POINT('Ctrl Pts',(-30.4849781474539,-31.2126376829455,
179.));
#33626=CARTESIAN_POINT('Ctrl Pts',(-30.4532401894943,-31.260659759229,179.));
#33627=CARTESIAN_POINT('Ctrl Pts',(-30.4238969592621,-31.3103407178797,
179.));
#33628=CARTESIAN_POINT('Ctrl Pts',(-30.3969892820085,-31.3614645973307,
179.));
#33629=CARTESIAN_POINT('Ctrl Pts',(-30.3834951193651,-31.3871031516275,
179.));
#33630=CARTESIAN_POINT('Ctrl Pts',(-30.3706138609554,-31.4131049574139,
179.));
#33631=CARTESIAN_POINT('Ctrl Pts',(-30.3583529950348,-31.4394446156991,
179.));
#33632=CARTESIAN_POINT('Ctrl Pts',(-30.3527381728228,-31.4515067734091,
179.));
#33633=CARTESIAN_POINT('Ctrl Pts',(-30.3472528660996,-31.4636414961716,
179.));
#33634=CARTESIAN_POINT('Ctrl Pts',(-30.3419063336923,-31.4758263198916,
179.));
#33635=CARTESIAN_POINT('Ctrl Pts',(-30.314994749283,-31.5371582051345,179.));
#33636=CARTESIAN_POINT('Ctrl Pts',(-30.2915439633216,-31.5998656461968,
179.));
#33637=CARTESIAN_POINT('Ctrl Pts',(-30.2715772012624,-31.6635906893212,
179.));
#33638=CARTESIAN_POINT('Ctrl Pts',(-30.2512551602859,-31.7284496250744,
179.));
#33639=CARTESIAN_POINT('Ctrl Pts',(-30.2345416753266,-31.7943635399902,
179.));
#33640=CARTESIAN_POINT('Ctrl Pts',(-30.2215005522,-31.860991549714,179.));
#33641=CARTESIAN_POINT('Ctrl Pts',(-30.210592869978,-31.9167196607127,179.));
#33642=CARTESIAN_POINT('Ctrl Pts',(-30.2022548395526,-31.9729482768223,
179.));
#33643=CARTESIAN_POINT('Ctrl Pts',(-30.1965486177622,-32.0294902235943,
179.));
#33644=CARTESIAN_POINT('Ctrl Pts',(-30.1939214710931,-32.0555221572595,
179.));
#33645=CARTESIAN_POINT('Ctrl Pts',(-30.1918525198042,-32.0816206201513,
179.));
#33646=CARTESIAN_POINT('Ctrl Pts',(-30.1903496283998,-32.107767746287,179.));
#33647=CARTESIAN_POINT('Ctrl Pts',(-30.1896917076954,-32.1192141725515,
179.));
#33648=CARTESIAN_POINT('Ctrl Pts',(-30.189142383326,-32.1306697639313,179.));
#33649=CARTESIAN_POINT('Ctrl Pts',(-30.1887026532007,-32.1421188060292,
179.));
#33650=CARTESIAN_POINT('Ctrl Pts',(-30.1860090542042,-32.2122507495274,
179.));
#33651=CARTESIAN_POINT('Ctrl Pts',(-30.1874155654491,-32.2822683610148,
179.));
#33652=CARTESIAN_POINT('Ctrl Pts',(-30.1929765281086,-32.3518105278729,
179.));
#33653=CARTESIAN_POINT('Ctrl Pts',(-30.1979467071931,-32.4139646987207,
179.));
#33654=CARTESIAN_POINT('Ctrl Pts',(-30.2062358596473,-32.4757400430717,
179.));
#33655=CARTESIAN_POINT('Ctrl Pts',(-30.2179158795994,-32.5368908724721,
179.));
#33656=CARTESIAN_POINT('Ctrl Pts',(-30.2306456144363,-32.6035374917853,
179.));
#33657=CARTESIAN_POINT('Ctrl Pts',(-30.2474020092586,-32.6694431322195,
179.));
#33658=CARTESIAN_POINT('Ctrl Pts',(-30.2679400111633,-32.7343943852058,
179.));
#33659=CARTESIAN_POINT('Ctrl Pts',(-30.2758707783801,-32.7594753677795,
179.));
#33660=CARTESIAN_POINT('Ctrl Pts',(-30.2843659849015,-32.7844139919257,
179.));
#33661=CARTESIAN_POINT('Ctrl Pts',(-30.2934135323341,-32.8091976483089,
179.));
#33662=CARTESIAN_POINT('Ctrl Pts',(-30.2973812067702,-32.8200661715852,
179.));
#33663=CARTESIAN_POINT('Ctrl Pts',(-30.3014550058364,-32.8309043340832,
179.));
#33664=CARTESIAN_POINT('Ctrl Pts',(-30.3056288188997,-32.8416985210892,
179.));
#33665=CARTESIAN_POINT('Ctrl Pts',(-30.3308503323267,-32.9069256235929,
179.));
#33666=CARTESIAN_POINT('Ctrl Pts',(-30.3597622632288,-32.9706662212829,
179.));
#33667=CARTESIAN_POINT('Ctrl Pts',(-30.3920521450586,-33.0327016892519,
179.));
#33668=CARTESIAN_POINT('Ctrl Pts',(-30.425088851225,-33.096171959536,179.));
#33669=CARTESIAN_POINT('Ctrl Pts',(-30.4616618729745,-33.1578581320537,
179.));
#33670=CARTESIAN_POINT('Ctrl Pts',(-30.5014926867972,-33.2175223280988,
179.));
#33671=CARTESIAN_POINT('Ctrl Pts',(-30.5319855016706,-33.2631987557176,
179.));
#33672=CARTESIAN_POINT('Ctrl Pts',(-30.5643888576175,-33.3076901760244,
179.));
#33673=CARTESIAN_POINT('Ctrl Pts',(-30.5985973406978,-33.3508837471854,
179.));
#33674=CARTESIAN_POINT('Ctrl Pts',(-30.619899662223,-33.3777812666846,179.));
#33675=CARTESIAN_POINT('Ctrl Pts',(-30.6419023011681,-33.4041753823072,
179.));
#33676=CARTESIAN_POINT('Ctrl Pts',(-30.664582713691,-33.4300371526971,179.));
#33677=CARTESIAN_POINT('Ctrl Pts',(-30.6772410834679,-33.4444710988324,
179.));
#33678=CARTESIAN_POINT('Ctrl Pts',(-30.6901150229931,-33.4587437314971,
179.));
#33679=CARTESIAN_POINT('Ctrl Pts',(-30.7031769988168,-33.4728246891271,
179.));
#33680=CARTESIAN_POINT('Ctrl Pts',(-30.7540414798183,-33.5276571747721,
179.));
#33681=CARTESIAN_POINT('Ctrl Pts',(-30.8078024741205,-33.5796445815827,
179.));
#33682=CARTESIAN_POINT('Ctrl Pts',(-30.8641753039031,-33.6285232274692,
179.));
#33683=CARTESIAN_POINT('Ctrl Pts',(-30.9063225983237,-33.6650674755938,
179.));
#33684=CARTESIAN_POINT('Ctrl Pts',(-30.9499310243967,-33.6998737756725,
179.));
#33685=CARTESIAN_POINT('Ctrl Pts',(-30.994897985227,-33.7328221880585,179.));
#33686=CARTESIAN_POINT('Ctrl Pts',(-31.0089818323205,-33.7431417736709,
179.));
#33687=CARTESIAN_POINT('Ctrl Pts',(-31.0231990403432,-33.7532790290714,
179.));
#33688=CARTESIAN_POINT('Ctrl Pts',(-31.0375466996756,-33.7632300412436,
179.));
#33689=CARTESIAN_POINT('Ctrl Pts',(-31.0513257036538,-33.7727866548438,
179.));
#33690=CARTESIAN_POINT('Ctrl Pts',(-31.065217962404,-33.7821665362252,179.));
#33691=CARTESIAN_POINT('Ctrl Pts',(-31.0792155749848,-33.7913635116716,
179.));
#33692=CARTESIAN_POINT('Ctrl Pts',(-31.1421637728842,-33.8327229240097,
179.));
#33693=CARTESIAN_POINT('Ctrl Pts',(-31.2072699803896,-33.870407069935,179.));
#33694=CARTESIAN_POINT('Ctrl Pts',(-31.2742731852794,-33.9041370162845,
179.));
#33695=CARTESIAN_POINT('Ctrl Pts',(-31.3254578858164,-33.9299038017072,
179.));
#33696=CARTESIAN_POINT('Ctrl Pts',(-31.3777505811556,-33.9533626457797,
179.));
#33697=CARTESIAN_POINT('Ctrl Pts',(-31.4310487463576,-33.9743739898132,
179.));
#33698=CARTESIAN_POINT('Ctrl Pts',(-31.4435331568518,-33.979295627227,179.));
#33699=CARTESIAN_POINT('Ctrl Pts',(-31.4560727789483,-33.9840829100841,
179.));
#33700=CARTESIAN_POINT('Ctrl Pts',(-31.4686656554564,-33.9887364314851,
179.));
#33701=CARTESIAN_POINT('Ctrl Pts',(-33.6673324974466,-32.0013033571361,
177.87148036339));
#33702=CARTESIAN_POINT('Ctrl Pts',(-33.668068719752,-32.0869545002621,177.877220944861));
#33703=CARTESIAN_POINT('Ctrl Pts',(-33.6620385737897,-32.1725016588414,
177.882961526332));
#33704=CARTESIAN_POINT('Ctrl Pts',(-33.6488812404577,-32.2569381526634,
177.888702107803));
#33705=CARTESIAN_POINT('Ctrl Pts',(-33.5639785938473,-32.801796416502,177.925745370876));
#33706=CARTESIAN_POINT('Ctrl Pts',(-33.1823026113929,-33.3004070278029,
177.962788633949));
#33707=CARTESIAN_POINT('Ctrl Pts',(-32.678505164673,-33.5246153329366,177.999831897022));
#33708=CARTESIAN_POINT('Ctrl Pts',(-32.1747077179532,-33.7488236380704,
178.036875160096));
#33709=CARTESIAN_POINT('Ctrl Pts',(-31.5487888069679,-33.698629637037,178.073918423169));
#33710=CARTESIAN_POINT('Ctrl Pts',(-31.0871675439728,-33.3969878684481,
178.110961686242));
#33711=CARTESIAN_POINT('Ctrl Pts',(-30.6255462809778,-33.0953460998591,
178.148004949315));
#33712=CARTESIAN_POINT('Ctrl Pts',(-30.3282226659731,-32.5422565637145,
178.185048212389));
#33713=CARTESIAN_POINT('Ctrl Pts',(-30.3312462755294,-31.9908384640567,
178.222091475462));
#33714=CARTESIAN_POINT('Ctrl Pts',(-30.3342698850858,-31.4394203643989,
178.259134738535));
#33715=CARTESIAN_POINT('Ctrl Pts',(-30.6376407192033,-30.8896737012279,
178.296178001608));
#33716=CARTESIAN_POINT('Ctrl Pts',(-31.1025462716722,-30.593101679575,178.333221264682));
#33717=CARTESIAN_POINT('Ctrl Pts',(-31.567451824141,-30.2965296579222,178.370264527755));
#33718=CARTESIAN_POINT('Ctrl Pts',(-32.1938920949612,-30.2531322777876,
178.407307790828));
#33719=CARTESIAN_POINT('Ctrl Pts',(-32.6951944291635,-30.4828858091372,
178.444351053901));
#33720=CARTESIAN_POINT('Ctrl Pts',(-33.1964967633658,-30.7126393404869,
178.481394316975));
#33721=CARTESIAN_POINT('Ctrl Pts',(-33.5726611609501,-31.2155437833208,
178.518437580048));
#33722=CARTESIAN_POINT('Ctrl Pts',(-33.6515914003734,-31.7612327671255,
178.555480843121));
#33723=CARTESIAN_POINT('Ctrl Pts',(-33.6629551037905,-31.839796417955,178.560814016544));
#33724=CARTESIAN_POINT('Ctrl Pts',(-33.6681578008391,-31.9192468976437,
178.566147189967));
#33725=CARTESIAN_POINT('Ctrl Pts',(-33.6674973899495,-31.9987820730806,
178.57148036339));
#33726=CARTESIAN_POINT('Ctrl Pts',(-32.5301702171889,-33.9851743256717,
179.));
#33727=CARTESIAN_POINT('Ctrl Pts',(-33.190239790753,-33.8088929660697,178.962956736927));
#33728=CARTESIAN_POINT('Ctrl Pts',(-34.3091776399806,-32.7483617530395,
178.88887021078));
#33729=CARTESIAN_POINT('Ctrl Pts',(-33.8814412030322,-30.4621270434605,
178.777740421561));
#33730=CARTESIAN_POINT('Ctrl Pts',(-31.7283973144122,-29.5870608054774,
178.666610632341));
#33731=CARTESIAN_POINT('Ctrl Pts',(-29.8255893685038,-30.9184850177167,
178.555480843121));
#33732=CARTESIAN_POINT('Ctrl Pts',(-29.9119598065434,-33.2405821817579,
178.444351053901));
#33733=CARTESIAN_POINT('Ctrl Pts',(-31.909683998457,-34.4268788699842,178.333221264681));
#33734=CARTESIAN_POINT('Ctrl Pts',(-33.9898669711731,-33.392335043116,178.222091475462));
#33735=CARTESIAN_POINT('Ctrl Pts',(-34.2490422451154,-31.0834368136807,
178.110961686242));
#33736=CARTESIAN_POINT('Ctrl Pts',(-32.4498708176529,-29.6134185829238,
177.999831897022));
#33737=CARTESIAN_POINT('Ctrl Pts',(-30.23900588914,-30.3275485827783,177.888702107803));
#33738=CARTESIAN_POINT('Ctrl Pts',(-29.6397721844782,-32.5723003600472,
177.777572318583));
#33739=CARTESIAN_POINT('Ctrl Pts',(-31.2005990238776,-34.293282975036,177.666442529363));
#33740=CARTESIAN_POINT('Ctrl Pts',(-33.4930261959862,-33.9154808666257,
177.555312740144));
#33741=CARTESIAN_POINT('Ctrl Pts',(-34.4190533459356,-31.7846499751686,
177.444182950924));
#33742=CARTESIAN_POINT('Ctrl Pts',(-33.1311884386701,-29.8509058112995,
177.333053161704));
#33743=CARTESIAN_POINT('Ctrl Pts',(-30.8080724679209,-29.8839889892312,
177.221923372484));
#33744=CARTESIAN_POINT('Ctrl Pts',(-29.5757954873418,-31.853622670774,177.110793583265));
#33745=CARTESIAN_POINT('Ctrl Pts',(-30.562124266553,-33.9572192112968,176.999663794045));
#33746=CARTESIAN_POINT('Ctrl Pts',(-32.8643812849987,-34.2695899967097,
176.888534004825));
#33747=CARTESIAN_POINT('Ctrl Pts',(-34.3755659443455,-32.5048566092284,
176.777404215605));
#33748=CARTESIAN_POINT('Ctrl Pts',(-33.7126584039828,-30.278083938033,176.666274426386));
#33749=CARTESIAN_POINT('Ctrl Pts',(-31.4823444699111,-29.6271901683823,
176.555144637166));
#33750=CARTESIAN_POINT('Ctrl Pts',(-29.7257832609726,-31.1478662270158,
176.444014847946));
#33751=CARTESIAN_POINT('Ctrl Pts',(-30.0505605498502,-33.4484058724806,
176.332885058726));
#33752=CARTESIAN_POINT('Ctrl Pts',(-32.1594436821683,-34.4233801713471,
176.221755269507));
#33753=CARTESIAN_POINT('Ctrl Pts',(-34.1224056859289,-33.1805032175714,
176.110625480287));
#33754=CARTESIAN_POINT('Ctrl Pts',(-34.1429650223268,-30.8572425212406,
175.999495691067));
#33755=CARTESIAN_POINT('Ctrl Pts',(-32.2023060098439,-29.5798210767118,
175.888365901848));
#33756=CARTESIAN_POINT('Ctrl Pts',(-30.0764987310374,-30.5173211370632,
175.777236112628));
#33757=CARTESIAN_POINT('Ctrl Pts',(-29.7110589540984,-32.8117528137747,
175.666106323408));
#33758=CARTESIAN_POINT('Ctrl Pts',(-31.4404331998289,-34.3632771184206,
175.554976534188));
#33759=CARTESIAN_POINT('Ctrl Pts',(-33.6819169128305,-33.7519558329571,
175.443846744969));
#33760=CARTESIAN_POINT('Ctrl Pts',(-34.3841285068372,-31.5372635683431,
175.332716955749));
#33761=CARTESIAN_POINT('Ctrl Pts',(-32.9044115461845,-29.7460626678129,
175.221587166529));
#33762=CARTESIAN_POINT('Ctrl Pts',(-30.5969869463981,-30.0176407707682,
175.110457377309));
#33763=CARTESIAN_POINT('Ctrl Pts',(-29.5735846782254,-32.1034525425256,
174.99932758809));
#33764=CARTESIAN_POINT('Ctrl Pts',(-30.7708113991622,-34.0945856692598,
174.88819779887));
#33765=CARTESIAN_POINT('Ctrl Pts',(-33.0929781975906,-34.168776706323,174.77706800965));
#33766=CARTESIAN_POINT('Ctrl Pts',(-34.414863202439,-32.2581268211635,174.665938220431));
#33767=CARTESIAN_POINT('Ctrl Pts',(-33.5266915925162,-30.1112420685439,
174.554808431211));
#33768=CARTESIAN_POINT('Ctrl Pts',(-31.2413083934035,-29.6929280920661,
174.443678641991));
#33769=CARTESIAN_POINT('Ctrl Pts',(-29.65027152498,-31.3860213065764,174.332548852771));
#33770=CARTESIAN_POINT('Ctrl Pts',(-30.2096806751507,-33.6410211629863,
174.221419063552));
#33771=CARTESIAN_POINT('Ctrl Pts',(-32.4075706562188,-34.3941762471646,
174.110289274332));
#33772=CARTESIAN_POINT('Ctrl Pts',(-34.2324563926352,-32.9562071936981,
173.999159485112));
#33773=CARTESIAN_POINT('Ctrl Pts',(-34.0142222484933,-30.6431276861944,
173.888029695892));
#33774=CARTESIAN_POINT('Ctrl Pts',(-31.9525937458611,-29.571843005618,173.776899906673));
#33775=CARTESIAN_POINT('Ctrl Pts',(-29.9343509329174,-30.722781274034,173.665770117453));
#33776=CARTESIAN_POINT('Ctrl Pts',(-29.8065677451363,-33.0426162695937,
173.554640328234));
#33777=CARTESIAN_POINT('Ctrl Pts',(-31.6861899702242,-34.4082601619239,
173.443510539014));
#33778=CARTESIAN_POINT('Ctrl Pts',(-33.8530077314349,-33.5698904705553,
173.332380749794));
#33779=CARTESIAN_POINT('Ctrl Pts',(-34.3239729118684,-31.2947740452877,
173.221250960574));
#33780=CARTESIAN_POINT('Ctrl Pts',(-32.6680632857967,-29.6650727659158,
173.110121171355));
#33781=CARTESIAN_POINT('Ctrl Pts',(-30.4007493854086,-30.1722715699463,
172.998991382135));
#33782=CARTESIAN_POINT('Ctrl Pts',(-29.5970523043438,-32.3521876122724,
172.887861592915));
#33783=CARTESIAN_POINT('Ctrl Pts',(-30.9925068954609,-34.2097853711626,
172.776731803695));
#33784=CARTESIAN_POINT('Ctrl Pts',(-33.3100082500444,-34.0450115224891,
172.665602014476));
#33785=CARTESIAN_POINT('Ctrl Pts',(-34.4286042606353,-32.0086653056602,
172.554472225256));
#33786=CARTESIAN_POINT('Ctrl Pts',(-33.3245679890092,-29.9643886950623,
172.443342436036));
#33787=CARTESIAN_POINT('Ctrl Pts',(-31.0083014581836,-29.7830814754581,
172.332212646816));
#33788=CARTESIAN_POINT('Ctrl Pts',(-29.5996266783055,-31.6306740480343,
172.221082857597));
#33789=CARTESIAN_POINT('Ctrl Pts',(-30.3877475314776,-33.8162697266764,
172.109953068377));
#33790=CARTESIAN_POINT('Ctrl Pts',(-32.6513843596913,-34.3396350480892,
171.998823279157));
#33791=CARTESIAN_POINT('Ctrl Pts',(-34.3188812858848,-32.7217917457764,
171.887693489937));
#33792=CARTESIAN_POINT('Ctrl Pts',(-33.864163206457,-30.4433724652345,171.776563700718));
#33793=CARTESIAN_POINT('Ctrl Pts',(-31.7033831764878,-29.5895618235874,
171.665433911498));
#33794=CARTESIAN_POINT('Ctrl Pts',(-29.8140636467216,-30.9417580608795,
171.554304122278));
#33795=CARTESIAN_POINT('Ctrl Pts',(-29.925289361983,-33.2624458446987,171.443174333059));
#33796=CARTESIAN_POINT('Ctrl Pts',(-31.9352677538577,-34.4277568821048,
171.332044543839));
#33797=CARTESIAN_POINT('Ctrl Pts',(-34.0044883954098,-33.3712111489356,
171.220914754619));
#33798=CARTESIAN_POINT('Ctrl Pts',(-34.2392229952543,-31.0597478424262,
171.109784965399));
#33799=CARTESIAN_POINT('Ctrl Pts',(-32.4246449932043,-29.6087931139184,
170.99865517618));
#33800=CARTESIAN_POINT('Ctrl Pts',(-30.2214364984569,-30.3462449959935,
170.88752538696));
#33801=CARTESIAN_POINT('Ctrl Pts',(-29.6459500326037,-32.5971955235092,
170.77639559774));
#33802=CARTESIAN_POINT('Ctrl Pts',(-31.2248645683027,-34.3015991842251,
170.66526580852));
#33803=CARTESIAN_POINT('Ctrl Pts',(-33.5131746450974,-33.8996042313419,
170.554136019301));
#33804=CARTESIAN_POINT('Ctrl Pts',(-34.4166436963946,-31.7591120862848,
170.443006230081));
#33805=CARTESIAN_POINT('Ctrl Pts',(-33.1084266441611,-29.8390779475391,
170.331876440861));
#33806=CARTESIAN_POINT('Ctrl Pts',(-30.7857895475778,-29.8966962369818,
170.220746651642));
#33807=CARTESIAN_POINT('Ctrl Pts',(-29.5743846894872,-31.8792353209593,
170.109616862422));
#33808=CARTESIAN_POINT('Ctrl Pts',(-30.5828766588753,-33.9722969295563,
169.998487073202));
#33809=CARTESIAN_POINT('Ctrl Pts',(-32.888304541998,-34.2603337768931,169.887357283982));
#33810=CARTESIAN_POINT('Ctrl Pts',(-34.3807657415457,-32.4797376639163,
169.776227494763));
#33811=CARTESIAN_POINT('Ctrl Pts',(-33.6943759527602,-30.2600908434617,
169.665097705543));
#33812=CARTESIAN_POINT('Ctrl Pts',(-31.4573116667505,-29.6327900145418,
169.553967916323));
#33813=CARTESIAN_POINT('Ctrl Pts',(-29.7169098581211,-31.1719340929902,
169.442838127103));
#33814=CARTESIAN_POINT('Ctrl Pts',(-30.065967388257,-33.4689151095322,169.331708337884));
#33815=CARTESIAN_POINT('Ctrl Pts',(-32.1850305909512,-34.4215609475536,
169.220578548664));
#33816=CARTESIAN_POINT('Ctrl Pts',(-34.1347558033771,-33.1580204671043,
169.109448759444));
#33817=CARTESIAN_POINT('Ctrl Pts',(-34.1307756550211,-30.8346722133795,
168.998318970225));
#33818=CARTESIAN_POINT('Ctrl Pts',(-32.1767327344769,-29.5778193124972,
168.887189181005));
#33819=CARTESIAN_POINT('Ctrl Pts',(-30.0609459319521,-30.5377199094004,
168.776059391785));
#33820=CARTESIAN_POINT('Ctrl Pts',(-29.719760384286,-32.8358833873742,168.664929602565));
#33821=CARTESIAN_POINT('Ctrl Pts',(-31.4654254048604,-34.3690554541617,
168.553799813346));
#33822=CARTESIAN_POINT('Ctrl Pts',(-33.7003272974666,-33.7340936603098,
168.442670024126));
#33823=CARTESIAN_POINT('Ctrl Pts',(-34.3791080871609,-31.5121081546712,
168.331540234906));
#33824=CARTESIAN_POINT('Ctrl Pts',(-32.8805549549265,-29.7366359735545,
168.220410445687));
#33825=CARTESIAN_POINT('Ctrl Pts',(-30.576127479021,-30.0325700070413,168.109280656467));
#33826=CARTESIAN_POINT('Ctrl Pts',(-29.5748126892805,-32.1290746285719,
167.998150867247));
#33827=CARTESIAN_POINT('Ctrl Pts',(-30.7930030339464,-34.1074515612365,
167.887021078027));
#33828=CARTESIAN_POINT('Ctrl Pts',(-33.1158238969359,-34.1571116561114,
167.775891288808));
#33829=CARTESIAN_POINT('Ctrl Pts',(-34.4174548619641,-32.2326066036682,
167.664761499588));
#33830=CARTESIAN_POINT('Ctrl Pts',(-33.5066572885625,-30.0952224134444,
167.553631710368));
#33831=CARTESIAN_POINT('Ctrl Pts',(-31.2169834359616,-29.7010702107005,
167.442501921148));
#33832=CARTESIAN_POINT('Ctrl Pts',(-29.643917581989,-31.4108732197425,167.331372131929));
#33833=CARTESIAN_POINT('Ctrl Pts',(-30.2271133546761,-33.6598394847521,
167.220242342709));
#33834=CARTESIAN_POINT('Ctrl Pts',(-32.4328346425493,-34.389736993149,167.109112553489));
#33835=CARTESIAN_POINT('Ctrl Pts',(-34.2424326326234,-32.932576501644,166.99798276427));
#33836=CARTESIAN_POINT('Ctrl Pts',(-33.9997759672129,-30.6219252261187,
166.886852975049));
#33837=CARTESIAN_POINT('Ctrl Pts',(-31.9269554466752,-29.5724870533531,
166.77572318583));
#33838=CARTESIAN_POINT('Ctrl Pts',(-29.9209653227032,-30.7446538702704,
166.66459339661));
#33839=CARTESIAN_POINT('Ctrl Pts',(-29.8177242538605,-33.0657579476906,
166.553463607391));
#33840=CARTESIAN_POINT('Ctrl Pts',(-31.7115987445193,-34.4113736221389,
166.442333818171));
#33841=CARTESIAN_POINT('Ctrl Pts',(-33.8695768792418,-33.5503671474171,
166.331204028951));
#33842=CARTESIAN_POINT('Ctrl Pts',(-34.3162088044827,-31.2699910786138,
166.220074239731));
#33843=CARTESIAN_POINT('Ctrl Pts',(-32.6437429613104,-29.6587100617298,
166.108944450512));
#33844=CARTESIAN_POINT('Ctrl Pts',(-30.3807636536437,-30.1881093063979,
165.997814661292));
#33845=CARTESIAN_POINT('Ctrl Pts',(-29.6025035271829,-32.3799438764187,
165.886684872072));
#33846=CARTESIAN_POINT('Ctrl Pts',(-30.5427968191103,-33.6016627022545,
165.812598345926));
#33847=CARTESIAN_POINT('Ctrl Pts',(-31.1673980508611,-33.878502477185,165.775555082853));
#33848=CARTESIAN_POINT('Ctrl Pts',(-32.4967348970879,-33.8599788000027,
179.074814972382));
#33849=CARTESIAN_POINT('Ctrl Pts',(-33.1151770144777,-33.6948146693492,
179.037771709309));
#33850=CARTESIAN_POINT('Ctrl Pts',(-34.1635487625758,-32.7011661280252,
178.963685183163));
#33851=CARTESIAN_POINT('Ctrl Pts',(-33.7627876332259,-30.5591133940879,
178.852555393943));
#33852=CARTESIAN_POINT('Ctrl Pts',(-31.7455260071196,-29.73923343181,178.741425604723));
#33853=CARTESIAN_POINT('Ctrl Pts',(-29.9627191301121,-30.9866910361882,
178.630295815504));
#33854=CARTESIAN_POINT('Ctrl Pts',(-30.0436425944261,-33.1623445497413,
178.519166026284));
#33855=CARTESIAN_POINT('Ctrl Pts',(-31.9153798001522,-34.2738271344597,
178.408036237064));
#33856=CARTESIAN_POINT('Ctrl Pts',(-33.8643755026176,-33.3045270781549,
178.296906447844));
#33857=CARTESIAN_POINT('Ctrl Pts',(-34.1072058217405,-31.1412401050271,
178.185776658625));
#33858=CARTESIAN_POINT('Ctrl Pts',(-32.4214995996843,-29.7639289492925,
178.074646869405));
#33859=CARTESIAN_POINT('Ctrl Pts',(-30.3500634323281,-30.4330221583869,
177.963517080185));
#33860=CARTESIAN_POINT('Ctrl Pts',(-29.7886205542368,-32.5362080917309,
177.852387290965));
#33861=CARTESIAN_POINT('Ctrl Pts',(-31.251013450526,-34.1486564987339,177.741257501746));
#33862=CARTESIAN_POINT('Ctrl Pts',(-33.3988681177627,-33.7946805767444,
177.630127712526));
#33863=CARTESIAN_POINT('Ctrl Pts',(-34.2664951290832,-31.798231079464,177.518997923306));
#33864=CARTESIAN_POINT('Ctrl Pts',(-33.0598497509898,-29.9864389849795,
177.407868134087));
#33865=CARTESIAN_POINT('Ctrl Pts',(-30.8832416820338,-30.0174357638488,
177.296738344867));
#33866=CARTESIAN_POINT('Ctrl Pts',(-29.7286785638387,-31.8628539944121,
177.185608555647));
#33867=CARTESIAN_POINT('Ctrl Pts',(-30.6528042667765,-33.8337866820529,
177.074478766427));
#33868=CARTESIAN_POINT('Ctrl Pts',(-32.8098688585814,-34.1264577241346,
176.963348977208));
#33869=CARTESIAN_POINT('Ctrl Pts',(-34.2257502715768,-32.4730176982761,
176.852219187988));
#33870=CARTESIAN_POINT('Ctrl Pts',(-33.6046491644892,-30.3866770140909,
176.741089398768));
#33871=CARTESIAN_POINT('Ctrl Pts',(-31.5149905480751,-29.7768320261982,
176.629959609548));
#33872=CARTESIAN_POINT('Ctrl Pts',(-29.8692073202332,-31.2016062609611,
176.518829820329));
#33873=CARTESIAN_POINT('Ctrl Pts',(-30.1735024464712,-33.3570617863506,
176.407700031109));
#33874=CARTESIAN_POINT('Ctrl Pts',(-32.149388325646,-34.2705490821455,176.296570241889));
#33875=CARTESIAN_POINT('Ctrl Pts',(-33.9885556294898,-33.1060544807695,
176.18544045267));
#33876=CARTESIAN_POINT('Ctrl Pts',(-34.007818386089,-30.9293108133877,176.07431066345));
#33877=CARTESIAN_POINT('Ctrl Pts',(-32.1895475296838,-29.7324502783874,
175.96318087423));
#33878=CARTESIAN_POINT('Ctrl Pts',(-30.1978048296397,-30.6108266580862,
175.85205108501));
#33879=CARTESIAN_POINT('Ctrl Pts',(-29.8554116055311,-32.7605594153313,
175.740921295791));
#33880=CARTESIAN_POINT('Ctrl Pts',(-31.4757224229406,-34.2142364435962,
175.629791506571));
#33881=CARTESIAN_POINT('Ctrl Pts',(-33.5758463933248,-33.6414682910725,
175.518661717351));
#33882=CARTESIAN_POINT('Ctrl Pts',(-34.2337728338789,-31.5664461595434,
175.407531928132));
#33883=CARTESIAN_POINT('Ctrl Pts',(-32.8473746011256,-29.8882078011037,
175.296402138912));
#33884=CARTESIAN_POINT('Ctrl Pts',(-30.6854683228166,-30.1426587616615,
175.185272349692));
#33885=CARTESIAN_POINT('Ctrl Pts',(-29.7266071799636,-32.0969282815195,
175.074142560472));
#33886=CARTESIAN_POINT('Ctrl Pts',(-30.8483304920893,-33.9624900892745,
174.963012771253));
#33887=CARTESIAN_POINT('Ctrl Pts',(-33.0240492485192,-34.0320022496441,
174.851882982033));
#33888=CARTESIAN_POINT('Ctrl Pts',(-34.2625692380559,-32.2418479872864,
174.740753192813));
#33889=CARTESIAN_POINT('Ctrl Pts',(-33.4304103974656,-30.2303570696963,
174.629623403593));
#33890=CARTESIAN_POINT('Ctrl Pts',(-31.2891554732695,-29.8384241709418,
174.518493614374));
#33891=CARTESIAN_POINT('Ctrl Pts',(-29.7984577511493,-31.4247420296276,
174.407363825154));
#33892=CARTESIAN_POINT('Ctrl Pts',(-30.3225876204458,-33.5375297443853,
174.296234035934));
#33893=CARTESIAN_POINT('Ctrl Pts',(-32.3818671087304,-34.2431869108974,
174.185104246714));
#33894=CARTESIAN_POINT('Ctrl Pts',(-34.0916659602814,-32.8959037429052,
174.073974457495));
#33895=CARTESIAN_POINT('Ctrl Pts',(-33.8871948081556,-30.7286991850778,
173.962844668275));
#33896=CARTESIAN_POINT('Ctrl Pts',(-31.9555834333813,-29.7249753463838,
173.851714879055));
#33897=CARTESIAN_POINT('Ctrl Pts',(-30.0646216186988,-30.8033293990645,
173.740585089835));
#33898=CARTESIAN_POINT('Ctrl Pts',(-29.9448971102786,-32.976863408369,173.629455300616));
#33899=CARTESIAN_POINT('Ctrl Pts',(-31.7059804798686,-34.2563826199768,
173.518325511396));
#33900=CARTESIAN_POINT('Ctrl Pts',(-33.7361473257739,-33.4708849272324,
173.407195722177));
#33901=CARTESIAN_POINT('Ctrl Pts',(-34.1774109668647,-31.3392493001677,
173.296065932957));
#33902=CARTESIAN_POINT('Ctrl Pts',(-32.6259317041196,-29.8123255480467,
173.184936143737));
#33903=CARTESIAN_POINT('Ctrl Pts',(-30.5016065337109,-30.2875377300117,
173.073806354517));
#33904=CARTESIAN_POINT('Ctrl Pts',(-29.7485948142495,-32.3299768105901,
172.962676565298));
#33905=CARTESIAN_POINT('Ctrl Pts',(-31.0560447053144,-34.0704246925659,
172.851546776078));
#33906=CARTESIAN_POINT('Ctrl Pts',(-33.2273922453066,-33.9160423487263,
172.740416986858));
#33907=CARTESIAN_POINT('Ctrl Pts',(-34.2754437129089,-32.0081188259464,
172.629287197638));
#33908=CARTESIAN_POINT('Ctrl Pts',(-33.2410337706164,-30.0927650417054,
172.518157408419));
#33909=CARTESIAN_POINT('Ctrl Pts',(-31.0708431799067,-29.9228920081938,
172.407027619199));
#33910=CARTESIAN_POINT('Ctrl Pts',(-29.7510068346601,-31.6539656834849,
172.295897829979));
#33911=CARTESIAN_POINT('Ctrl Pts',(-30.4894246450174,-33.7017262126649,
172.18476804076));
#33912=CARTESIAN_POINT('Ctrl Pts',(-32.6103046387472,-34.1920853664661,
172.07363825154));
#33913=CARTESIAN_POINT('Ctrl Pts',(-34.1726404455737,-32.6762717650536,
171.96250846232));
#33914=CARTESIAN_POINT('Ctrl Pts',(-33.7465992779157,-30.5415415781258,
171.8513786731));
#33915=CARTESIAN_POINT('Ctrl Pts',(-31.7220893921897,-29.7415767225744,
171.74024888388));
#33916=CARTESIAN_POINT('Ctrl Pts',(-29.9519202809166,-31.0084963589422,
171.629119094661));
#33917=CARTESIAN_POINT('Ctrl Pts',(-30.056131518049,-33.1828293751969,171.517989305441));
#33918=CARTESIAN_POINT('Ctrl Pts',(-31.9393501094869,-34.2746497745218,
171.406859516221));
#33919=CARTESIAN_POINT('Ctrl Pts',(-33.8780748230019,-33.284735367754,171.295729727002));
#33920=CARTESIAN_POINT('Ctrl Pts',(-34.0980058253788,-31.1190450847926,
171.184599937782));
#33921=CARTESIAN_POINT('Ctrl Pts',(-32.3978646482948,-29.7595951866708,
171.073470148562));
#33922=CARTESIAN_POINT('Ctrl Pts',(-30.3336020597539,-30.4505394775294,
170.962340359343));
#33923=CARTESIAN_POINT('Ctrl Pts',(-29.794408794793,-32.5595332353534,170.851210570123));
#33924=CARTESIAN_POINT('Ctrl Pts',(-31.273748682197,-34.1564482440673,170.740080780903));
#33925=CARTESIAN_POINT('Ctrl Pts',(-33.4177458997867,-33.7798052055182,
170.628950991683));
#33926=CARTESIAN_POINT('Ctrl Pts',(-34.2642374447057,-31.7743037440626,
170.517821202464));
#33927=CARTESIAN_POINT('Ctrl Pts',(-33.0385234348626,-29.975357048467,170.406691413244));
#33928=CARTESIAN_POINT('Ctrl Pts',(-30.8623640397511,-30.0293416257758,
170.295561624024));
#33929=CARTESIAN_POINT('Ctrl Pts',(-29.727356738311,-31.8868513762745,170.184431834804));
#33930=CARTESIAN_POINT('Ctrl Pts',(-30.6722479041788,-33.847913520161,170.073302045585));
#33931=CARTESIAN_POINT('Ctrl Pts',(-32.8322833892703,-34.1177852501839,
169.962172256365));
#33932=CARTESIAN_POINT('Ctrl Pts',(-34.2306221422391,-32.4494828856631,
169.851042467145));
#33933=CARTESIAN_POINT('Ctrl Pts',(-33.5875197007206,-30.3698186586225,
169.739912677925));
#33934=CARTESIAN_POINT('Ctrl Pts',(-31.4915364450367,-29.7820787166299,
169.628782888706));
#33935=CARTESIAN_POINT('Ctrl Pts',(-29.8608935207979,-31.2241562808234,
169.517653099486));
#33936=CARTESIAN_POINT('Ctrl Pts',(-30.1879376486804,-33.3762776031315,
169.406523310266));
#33937=CARTESIAN_POINT('Ctrl Pts',(-32.1733615894941,-34.2688445881649,
169.295393521047));
#33938=CARTESIAN_POINT('Ctrl Pts',(-34.0001268836281,-33.0849896107005,
169.184263731827));
#33939=CARTESIAN_POINT('Ctrl Pts',(-33.9963977443443,-30.9081639077541,
169.073133942607));
#33940=CARTESIAN_POINT('Ctrl Pts',(-32.1655870394568,-29.730574755944,168.962004153387));
#33941=CARTESIAN_POINT('Ctrl Pts',(-30.1832328717994,-30.6299389766382,
168.850874364168));
#33942=CARTESIAN_POINT('Ctrl Pts',(-29.8635642778024,-32.7831681881461,
168.739744574948));
#33943=CARTESIAN_POINT('Ctrl Pts',(-31.4991384881812,-34.2196503671186,
168.628614785728));
#33944=CARTESIAN_POINT('Ctrl Pts',(-33.5930957223536,-33.6247326009035,
168.517484996508));
#33945=CARTESIAN_POINT('Ctrl Pts',(-34.2290690282512,-31.5428771784569,
168.406355207289));
#33946=CARTESIAN_POINT('Ctrl Pts',(-32.825022531886,-29.8793756037254,168.295225418069));
#33947=CARTESIAN_POINT('Ctrl Pts',(-30.6659243630751,-30.1566464818375,
168.184095628849));
#33948=CARTESIAN_POINT('Ctrl Pts',(-29.7277577461881,-32.1209345041679,
168.072965839629));
#33949=CARTESIAN_POINT('Ctrl Pts',(-30.8691226057602,-33.9745445904889,
167.96183605041));
#33950=CARTESIAN_POINT('Ctrl Pts',(-33.0454541780027,-34.0210728588022,
167.85070626119));
#33951=CARTESIAN_POINT('Ctrl Pts',(-34.2649974539114,-32.2179372088228,
167.73957647197));
#33952=CARTESIAN_POINT('Ctrl Pts',(-33.4116395620055,-30.2153476982354,
167.628446682751));
#33953=CARTESIAN_POINT('Ctrl Pts',(-31.266364575479,-29.8460528047858,167.517316893531));
#33954=CARTESIAN_POINT('Ctrl Pts',(-29.7925045211951,-31.4480266505451,
167.406187104311));
#33955=CARTESIAN_POINT('Ctrl Pts',(-30.3389209035863,-33.5551612838846,
167.295057315091));
#33956=CARTESIAN_POINT('Ctrl Pts',(-32.4055378153131,-34.2390276195696,
167.183927525872));
#33957=CARTESIAN_POINT('Ctrl Pts',(-34.1010130461478,-32.8737633264784,
167.072797736652));
#33958=CARTESIAN_POINT('Ctrl Pts',(-33.8736595852923,-30.7088338635598,
166.961667947432));
#33959=CARTESIAN_POINT('Ctrl Pts',(-31.9315620200791,-29.7255787770841,
166.850538158213));
#33960=CARTESIAN_POINT('Ctrl Pts',(-30.0520801754102,-30.8238225944352,
166.739408368993));
#33961=CARTESIAN_POINT('Ctrl Pts',(-29.9553500309319,-32.9985456506286,
166.628278579773));
#33962=CARTESIAN_POINT('Ctrl Pts',(-31.7297868433258,-34.2592997290284,
166.517148790554));
#33963=CARTESIAN_POINT('Ctrl Pts',(-33.7516715360443,-33.4525928474522,
166.406019001334));
#33964=CARTESIAN_POINT('Ctrl Pts',(-34.1701365048935,-31.3160292776143,
166.294889212114));
#33965=CARTESIAN_POINT('Ctrl Pts',(-32.603145147106,-29.8063641094246,166.183759422894));
#33966=CARTESIAN_POINT('Ctrl Pts',(-30.4828812072222,-30.3023766555707,
166.072629633674));
#33967=CARTESIAN_POINT('Ctrl Pts',(-29.7537022543286,-32.3559826188516,
165.961499844455));
#33968=CARTESIAN_POINT('Ctrl Pts',(-30.6346957097411,-33.5006534350279,
165.887413318308));
#33969=CARTESIAN_POINT('Ctrl Pts',(-31.2199063053492,-33.7600342388745,
165.850370055235));
#33970=CARTESIAN_POINT('Ctrl Pts',(-32.463299576987,-33.7347832743337,179.149629944765));
#33971=CARTESIAN_POINT('Ctrl Pts',(-33.0401142382023,-33.5807363726286,
179.112586681692));
#33972=CARTESIAN_POINT('Ctrl Pts',(-34.017919885171,-32.653970503011,179.038500155545));
#33973=CARTESIAN_POINT('Ctrl Pts',(-33.6441340634195,-30.6560997447152,
178.927370366326));
#33974=CARTESIAN_POINT('Ctrl Pts',(-31.7626546998272,-29.8914060581426,
178.816240577106));
#33975=CARTESIAN_POINT('Ctrl Pts',(-30.0998488917205,-31.0548970546596,
178.705110787886));
#33976=CARTESIAN_POINT('Ctrl Pts',(-30.1753253823088,-33.0841069177247,
178.593980998666));
#33977=CARTESIAN_POINT('Ctrl Pts',(-31.9210756018475,-34.1207753989353,
178.482851209446));
#33978=CARTESIAN_POINT('Ctrl Pts',(-33.738884034062,-33.2167191131938,178.371721420227));
#33979=CARTESIAN_POINT('Ctrl Pts',(-33.9653693983657,-31.1990433963734,
178.260591631007));
#33980=CARTESIAN_POINT('Ctrl Pts',(-32.3931283817158,-29.9144393156612,
178.149461841787));
#33981=CARTESIAN_POINT('Ctrl Pts',(-30.4611209755161,-30.5384957339954,
178.038332052568));
#33982=CARTESIAN_POINT('Ctrl Pts',(-29.9374689239953,-32.5001158234147,
177.927202263348));
#33983=CARTESIAN_POINT('Ctrl Pts',(-31.3014278771744,-34.0040300224318,
177.816072474128));
#33984=CARTESIAN_POINT('Ctrl Pts',(-33.3047100395391,-33.6738802868631,
177.704942684909));
#33985=CARTESIAN_POINT('Ctrl Pts',(-34.1139369122308,-31.8118121837595,
177.593812895689));
#33986=CARTESIAN_POINT('Ctrl Pts',(-32.9885110633096,-30.1219721586597,
177.482683106469));
#33987=CARTESIAN_POINT('Ctrl Pts',(-30.9584108961468,-30.1508825384663,
177.371553317249));
#33988=CARTESIAN_POINT('Ctrl Pts',(-29.8815616403355,-31.8720853180504,
177.260423528029));
#33989=CARTESIAN_POINT('Ctrl Pts',(-30.743484267,-33.710354152809,177.14929373881));
#33990=CARTESIAN_POINT('Ctrl Pts',(-32.755356432164,-33.9833254515596,177.03816394959));
#33991=CARTESIAN_POINT('Ctrl Pts',(-34.0759345988082,-32.4411787873238,
176.927034160371));
#33992=CARTESIAN_POINT('Ctrl Pts',(-33.4966399249956,-30.4952700901487,
176.815904371151));
#33993=CARTESIAN_POINT('Ctrl Pts',(-31.547636626239,-29.9264738840141,176.704774581931));
#33994=CARTESIAN_POINT('Ctrl Pts',(-30.0126313794938,-31.2553462949064,
176.593644792711));
#33995=CARTESIAN_POINT('Ctrl Pts',(-30.2964443430921,-33.2657177002206,
176.482515003491));
#33996=CARTESIAN_POINT('Ctrl Pts',(-32.1393329691236,-34.1177179929438,
176.371385214272));
#33997=CARTESIAN_POINT('Ctrl Pts',(-33.8547055730506,-33.0316057439677,
176.260255425052));
#33998=CARTESIAN_POINT('Ctrl Pts',(-33.872671749851,-31.0013791055347,176.149125635832));
#33999=CARTESIAN_POINT('Ctrl Pts',(-32.1767890495237,-29.8850794800629,
176.037995846613));
#34000=CARTESIAN_POINT('Ctrl Pts',(-30.319110928242,-30.7043321791094,175.926866057393));
#34001=CARTESIAN_POINT('Ctrl Pts',(-29.9997642569639,-32.7093660168879,
175.815736268173));
#34002=CARTESIAN_POINT('Ctrl Pts',(-31.5110116460523,-34.0651957687719,
175.704606478954));
#34003=CARTESIAN_POINT('Ctrl Pts',(-33.4697758738191,-33.5309807491879,
175.593476689734));
#34004=CARTESIAN_POINT('Ctrl Pts',(-34.0834171609207,-31.5956287507438,
175.482346900514));
#34005=CARTESIAN_POINT('Ctrl Pts',(-32.7903376560667,-30.0303529343944,
175.371217111294));
#34006=CARTESIAN_POINT('Ctrl Pts',(-30.7739496992351,-30.2676767525548,
175.260087322075));
#34007=CARTESIAN_POINT('Ctrl Pts',(-29.8796296817018,-32.0904040205134,
175.148957532855));
#34008=CARTESIAN_POINT('Ctrl Pts',(-30.9258495850164,-33.8303945092891,
175.037827743635));
#34009=CARTESIAN_POINT('Ctrl Pts',(-32.9551202994478,-33.8952277929652,
174.926697954415));
#34010=CARTESIAN_POINT('Ctrl Pts',(-34.1102752736729,-32.2255691534092,
174.815568165196));
#34011=CARTESIAN_POINT('Ctrl Pts',(-33.334129202415,-30.3494720708486,174.704438375976));
#34012=CARTESIAN_POINT('Ctrl Pts',(-31.3370025531356,-29.9839202498175,
174.593308586756));
#34013=CARTESIAN_POINT('Ctrl Pts',(-29.9466439773186,-31.4634627526788,
174.482178797536));
#34014=CARTESIAN_POINT('Ctrl Pts',(-30.4354945657408,-33.4340383257844,
174.371049008317));
#34015=CARTESIAN_POINT('Ctrl Pts',(-32.3561635612421,-34.0921975746302,
174.259919219097));
#34016=CARTESIAN_POINT('Ctrl Pts',(-33.9508755279276,-32.8356002921123,
174.148789429877));
#34017=CARTESIAN_POINT('Ctrl Pts',(-33.7601673678179,-30.8142706839612,
174.037659640658));
#34018=CARTESIAN_POINT('Ctrl Pts',(-31.9585731209015,-29.8781076871497,
173.926529851438));
#34019=CARTESIAN_POINT('Ctrl Pts',(-30.1948923044803,-30.883877524095,173.815400062218));
#34020=CARTESIAN_POINT('Ctrl Pts',(-30.0832264754209,-32.9111105471442,
173.704270272998));
#34021=CARTESIAN_POINT('Ctrl Pts',(-31.725770989513,-34.1045050780296,173.593140483779));
#34022=CARTESIAN_POINT('Ctrl Pts',(-33.619286920113,-33.3718793839095,173.482010694559));
#34023=CARTESIAN_POINT('Ctrl Pts',(-34.0308490218611,-31.3837245550478,
173.370880905339));
#34024=CARTESIAN_POINT('Ctrl Pts',(-32.5838001224424,-29.9595783301775,
173.25975111612));
#34025=CARTESIAN_POINT('Ctrl Pts',(-30.6024636820132,-30.4028038900771,
173.1486213269));
#34026=CARTESIAN_POINT('Ctrl Pts',(-29.9001373241552,-32.3077660089076,
173.03749153768));
#34027=CARTESIAN_POINT('Ctrl Pts',(-31.1195825151679,-33.9310640139692,
172.92636174846));
#34028=CARTESIAN_POINT('Ctrl Pts',(-33.1447762405689,-33.7870731749634,
172.815231959241));
#34029=CARTESIAN_POINT('Ctrl Pts',(-34.1222831651826,-32.0075723462327,
172.704102170021));
#34030=CARTESIAN_POINT('Ctrl Pts',(-33.1574995522237,-30.2211413883485,
172.592972380801));
#34031=CARTESIAN_POINT('Ctrl Pts',(-31.1333849016297,-30.0627025409294,
172.481842591581));
#34032=CARTESIAN_POINT('Ctrl Pts',(-29.9023869910147,-31.6772573189356,
172.370712802361));
#34033=CARTESIAN_POINT('Ctrl Pts',(-30.5911017585573,-33.5871826986533,
172.259583013142));
#34034=CARTESIAN_POINT('Ctrl Pts',(-32.569224917803,-34.0445356848432,172.148453223922));
#34035=CARTESIAN_POINT('Ctrl Pts',(-34.0263996052626,-32.6307517843307,
172.037323434703));
#34036=CARTESIAN_POINT('Ctrl Pts',(-33.6290353493745,-30.6397106910171,
171.926193645483));
#34037=CARTESIAN_POINT('Ctrl Pts',(-31.7407956078916,-29.8935916215613,
171.815063856263));
#34038=CARTESIAN_POINT('Ctrl Pts',(-30.0897769151117,-31.0752346570049,
171.703934067043));
#34039=CARTESIAN_POINT('Ctrl Pts',(-30.1869736741148,-33.1032129056951,
171.592804277824));
#34040=CARTESIAN_POINT('Ctrl Pts',(-31.9434324651163,-34.1215426669389,
171.481674488604));
#34041=CARTESIAN_POINT('Ctrl Pts',(-33.7516612505939,-33.1982595865724,
171.370544699384));
#34042=CARTESIAN_POINT('Ctrl Pts',(-33.9567886555033,-31.1783423271589,
171.259414910164));
#34043=CARTESIAN_POINT('Ctrl Pts',(-32.3710843033854,-29.9103972594232,
171.148285120945));
#34044=CARTESIAN_POINT('Ctrl Pts',(-30.4457676210508,-30.5548339590653,
171.037155331725));
#34045=CARTESIAN_POINT('Ctrl Pts',(-29.9428675569823,-32.5218709471976,
170.926025542505));
#34046=CARTESIAN_POINT('Ctrl Pts',(-31.3226327960912,-34.0112973039095,
170.814895753286));
#34047=CARTESIAN_POINT('Ctrl Pts',(-33.3223171544759,-33.6600061796944,
170.703765964066));
#34048=CARTESIAN_POINT('Ctrl Pts',(-34.1118311930168,-31.7894954018404,
170.592636174846));
#34049=CARTESIAN_POINT('Ctrl Pts',(-32.9686202255643,-30.1116361493947,
170.481506385626));
#34050=CARTESIAN_POINT('Ctrl Pts',(-30.9389385319243,-30.1619870145698,
170.370376596406));
#34051=CARTESIAN_POINT('Ctrl Pts',(-29.8803287871347,-31.8944674315897,
170.259246807187));
#34052=CARTESIAN_POINT('Ctrl Pts',(-30.7616191494823,-33.7235301107657,
170.148117017967));
#34053=CARTESIAN_POINT('Ctrl Pts',(-32.7762622365426,-33.9752367234746,
170.036987228747));
#34054=CARTESIAN_POINT('Ctrl Pts',(-34.0804785429325,-32.4192281074099,
169.925857439528));
#34055=CARTESIAN_POINT('Ctrl Pts',(-33.4806634486809,-30.4795464737831,
169.814727650308));
#34056=CARTESIAN_POINT('Ctrl Pts',(-31.5257612233229,-29.9313674187181,
169.703597861088));
#34057=CARTESIAN_POINT('Ctrl Pts',(-30.0048771834747,-31.2763784686564,
169.592468071869));
#34058=CARTESIAN_POINT('Ctrl Pts',(-30.3099079091038,-33.2836400967308,
169.481338282649));
#34059=CARTESIAN_POINT('Ctrl Pts',(-32.161692588037,-34.1161282287762,169.370208493429));
#34060=CARTESIAN_POINT('Ctrl Pts',(-33.865497963879,-33.0119587542968,169.259078704209));
#34061=CARTESIAN_POINT('Ctrl Pts',(-33.8620198336676,-30.9816556021287,
169.14794891499));
#34062=CARTESIAN_POINT('Ctrl Pts',(-32.1544413444366,-29.8833301993908,
169.03681912577));
#34063=CARTESIAN_POINT('Ctrl Pts',(-30.3055198116467,-30.722158043876,168.92568933655));
#34064=CARTESIAN_POINT('Ctrl Pts',(-30.0073681713189,-32.7304529889181,
168.81455954733));
#34065=CARTESIAN_POINT('Ctrl Pts',(-31.5328515715021,-34.0702452800755,
168.703429758111));
#34066=CARTESIAN_POINT('Ctrl Pts',(-33.4858641472406,-33.5153715414972,
168.592299968891));
#34067=CARTESIAN_POINT('Ctrl Pts',(-34.0790299693416,-31.5736462022427,
168.481170179671));
#34068=CARTESIAN_POINT('Ctrl Pts',(-32.7694901088454,-30.0221152338963,
168.370040390451));
#34069=CARTESIAN_POINT('Ctrl Pts',(-30.7557212471292,-30.2807229566338,
168.258910601232));
#34070=CARTESIAN_POINT('Ctrl Pts',(-29.8807028030956,-32.1127943797639,
168.147780812012));
#34071=CARTESIAN_POINT('Ctrl Pts',(-30.9452421775741,-33.8416376197414,
168.036651022792));
#34072=CARTESIAN_POINT('Ctrl Pts',(-32.9750844590695,-33.885034061493,167.925521233573));
#34073=CARTESIAN_POINT('Ctrl Pts',(-34.1125400458588,-32.2032678139773,
167.814391444353));
#34074=CARTESIAN_POINT('Ctrl Pts',(-33.3166218354486,-30.3354729830266,
167.703261655133));
#34075=CARTESIAN_POINT('Ctrl Pts',(-31.3157457149963,-29.9910353988711,
167.592131865913));
#34076=CARTESIAN_POINT('Ctrl Pts',(-29.9410914604013,-31.4851800813478,
167.481002076694));
#34077=CARTESIAN_POINT('Ctrl Pts',(-30.4507284524965,-33.4504830830171,
167.369872287474));
#34078=CARTESIAN_POINT('Ctrl Pts',(-32.3782409880768,-34.0883182459902,
167.258742498254));
#34079=CARTESIAN_POINT('Ctrl Pts',(-33.9595934596722,-32.8149501513129,
167.147612709035));
#34080=CARTESIAN_POINT('Ctrl Pts',(-33.7475432033717,-30.7957425010009,
167.036482919815));
#34081=CARTESIAN_POINT('Ctrl Pts',(-31.936168593483,-29.8786705008151,166.925353130595));
#34082=CARTESIAN_POINT('Ctrl Pts',(-30.1831950281172,-30.9029913185999,
166.814223341375));
#34083=CARTESIAN_POINT('Ctrl Pts',(-30.0929758080031,-32.9313333535665,
166.703093552156));
#34084=CARTESIAN_POINT('Ctrl Pts',(-31.7479749421323,-34.1072258359179,
166.591963762936));
#34085=CARTESIAN_POINT('Ctrl Pts',(-33.6337661928468,-33.3548185474873,
166.480833973716));
#34086=CARTESIAN_POINT('Ctrl Pts',(-34.0240642053043,-31.3620674766148,
166.369704184496));
#34087=CARTESIAN_POINT('Ctrl Pts',(-32.5625473329016,-29.9540181571193,
166.258574395277));
#34088=CARTESIAN_POINT('Ctrl Pts',(-30.5849987608006,-30.4166440047433,
166.147444606057));
#34089=CARTESIAN_POINT('Ctrl Pts',(-29.9049009814742,-32.3320213612846,
166.036314816837));
#34090=CARTESIAN_POINT('Ctrl Pts',(-30.7265946003719,-33.3996441678013,
165.962228290691));
#34091=CARTESIAN_POINT('Ctrl Pts',(-31.2724145598372,-33.6415660005639,
165.925185027618));
#34092=CARTESIAN_POINT('Ctrl Pts',(-32.4298642568861,-33.6095877486648,
179.224444917147));
#34093=CARTESIAN_POINT('Ctrl Pts',(-32.965051461927,-33.4666580759081,179.187401654074));
#34094=CARTESIAN_POINT('Ctrl Pts',(-33.8722910077662,-32.6067748779967,
179.113315127928));
#34095=CARTESIAN_POINT('Ctrl Pts',(-33.5254804936132,-30.7530860953427,
179.002185338708));
#34096=CARTESIAN_POINT('Ctrl Pts',(-31.7797833925347,-30.0435786844751,
178.891055549488));
#34097=CARTESIAN_POINT('Ctrl Pts',(-30.2369786533288,-31.1231030731311,
178.779925760269));
#34098=CARTESIAN_POINT('Ctrl Pts',(-30.3070081701916,-33.0058692857081,
178.668795971049));
#34099=CARTESIAN_POINT('Ctrl Pts',(-31.9267714035427,-33.9677236634109,
178.557666181829));
#34100=CARTESIAN_POINT('Ctrl Pts',(-33.6133925655065,-33.1289111482327,
178.446536392609));
#34101=CARTESIAN_POINT('Ctrl Pts',(-33.8235329749908,-31.2568466877197,
178.33540660339));
#34102=CARTESIAN_POINT('Ctrl Pts',(-32.3647571637473,-30.0649496820299,
178.22427681417));
#34103=CARTESIAN_POINT('Ctrl Pts',(-30.5721785187041,-30.643969309604,178.11314702495));
#34104=CARTESIAN_POINT('Ctrl Pts',(-30.0863172937539,-32.4640235550984,
178.00201723573));
#34105=CARTESIAN_POINT('Ctrl Pts',(-31.3518423038228,-33.8594035461297,
177.890887446511));
#34106=CARTESIAN_POINT('Ctrl Pts',(-33.2105519613155,-33.5530799969818,
177.779757657291));
#34107=CARTESIAN_POINT('Ctrl Pts',(-33.9613786953784,-31.8253932880549,
177.668627868071));
#34108=CARTESIAN_POINT('Ctrl Pts',(-32.9171723756293,-30.2575053323397,
177.557498078851));
#34109=CARTESIAN_POINT('Ctrl Pts',(-31.0335801102598,-30.2843293130839,
177.446368289632));
#34110=CARTESIAN_POINT('Ctrl Pts',(-30.0344447168324,-31.8813166416885,
177.335238500412));
#34111=CARTESIAN_POINT('Ctrl Pts',(-30.8341642672234,-33.5869216235651,
177.224108711192));
#34112=CARTESIAN_POINT('Ctrl Pts',(-32.7008440057466,-33.8401931789845,
177.112978921973));
#34113=CARTESIAN_POINT('Ctrl Pts',(-33.9261189260395,-32.4093398763715,
177.001849132753));
#34114=CARTESIAN_POINT('Ctrl Pts',(-33.388630685502,-30.6038631662066,176.890719343533));
#34115=CARTESIAN_POINT('Ctrl Pts',(-31.5802827044029,-30.0761157418299,
176.779589554313));
#34116=CARTESIAN_POINT('Ctrl Pts',(-30.1560554387543,-31.3090863288518,
176.668459765094));
#34117=CARTESIAN_POINT('Ctrl Pts',(-30.4193862397131,-33.1743736140907,
176.557329975874));
#34118=CARTESIAN_POINT('Ctrl Pts',(-32.1292776126013,-33.9648869037422,
176.446200186654));
#34119=CARTESIAN_POINT('Ctrl Pts',(-33.7208555166115,-32.9571570071658,
176.335070397434));
#34120=CARTESIAN_POINT('Ctrl Pts',(-33.7375251136131,-31.0734473976818,
176.223940608215));
#34121=CARTESIAN_POINT('Ctrl Pts',(-32.1640305693636,-30.0377086817384,
176.112810818995));
#34122=CARTESIAN_POINT('Ctrl Pts',(-30.4404170268443,-30.7978377001325,
176.001681029775));
#34123=CARTESIAN_POINT('Ctrl Pts',(-30.1441169083966,-32.6581726184444,
175.890551240556));
#34124=CARTESIAN_POINT('Ctrl Pts',(-31.5463008691641,-33.9161550939476,
175.779421451336));
#34125=CARTESIAN_POINT('Ctrl Pts',(-33.3637053543134,-33.4204932073033,
175.668291662116));
#34126=CARTESIAN_POINT('Ctrl Pts',(-33.9330614879624,-31.6248113419441,
175.557161872897));
#34127=CARTESIAN_POINT('Ctrl Pts',(-32.7333007110078,-30.1724980676852,
175.446032083677));
#34128=CARTESIAN_POINT('Ctrl Pts',(-30.8624310756536,-30.3926947434481,
175.334902294457));
#34129=CARTESIAN_POINT('Ctrl Pts',(-30.0326521834401,-32.0838797595073,
175.223772505237));
#34130=CARTESIAN_POINT('Ctrl Pts',(-31.0033686779435,-33.6982989293037,
175.112642716018));
#34131=CARTESIAN_POINT('Ctrl Pts',(-32.8861913503764,-33.7584533362862,
175.001512926798));
#34132=CARTESIAN_POINT('Ctrl Pts',(-33.9579813092899,-32.209290319532,174.890383137578));
#34133=CARTESIAN_POINT('Ctrl Pts',(-33.2378480073643,-30.4685870720011,
174.779253348358));
#34134=CARTESIAN_POINT('Ctrl Pts',(-31.3848496330017,-30.1294163286931,
174.668123559139));
#34135=CARTESIAN_POINT('Ctrl Pts',(-30.0948302034879,-31.50218347573,174.556993769919));
#34136=CARTESIAN_POINT('Ctrl Pts',(-30.5484015110359,-33.3305469071834,
174.445863980699));
#34137=CARTESIAN_POINT('Ctrl Pts',(-32.3304600137538,-33.9412082383629,
174.33473419148));
#34138=CARTESIAN_POINT('Ctrl Pts',(-33.8100850955738,-32.7752968413194,
174.22360440226));
#34139=CARTESIAN_POINT('Ctrl Pts',(-33.6331399274802,-30.8998421828445,
174.11247461304));
#34140=CARTESIAN_POINT('Ctrl Pts',(-31.9615628084217,-30.0312400279156,
174.00134482382));
#34141=CARTESIAN_POINT('Ctrl Pts',(-30.3251629902618,-30.9644256491254,
173.890215034601));
#34142=CARTESIAN_POINT('Ctrl Pts',(-30.2215558405631,-32.8453576859195,
173.779085245381));
#34143=CARTESIAN_POINT('Ctrl Pts',(-31.7455614991574,-33.9526275360824,
173.667955456161));
#34144=CARTESIAN_POINT('Ctrl Pts',(-33.5024265144521,-33.2728738405865,
173.556825666942));
#34145=CARTESIAN_POINT('Ctrl Pts',(-33.8842870768574,-31.4281998099279,
173.445695877722));
#34146=CARTESIAN_POINT('Ctrl Pts',(-32.5416685407652,-30.1068311123084,
173.334566088502));
#34147=CARTESIAN_POINT('Ctrl Pts',(-30.7033208303155,-30.5180700501426,
173.223436299282));
#34148=CARTESIAN_POINT('Ctrl Pts',(-30.0516798340609,-32.2855552072252,
173.112306510062));
#34149=CARTESIAN_POINT('Ctrl Pts',(-31.1831203250215,-33.7917033353726,
173.001176720843));
#34150=CARTESIAN_POINT('Ctrl Pts',(-33.0621602358311,-33.6581040012006,
172.890046931623));
#34151=CARTESIAN_POINT('Ctrl Pts',(-33.9691226174563,-32.007025866519,172.778917142403));
#34152=CARTESIAN_POINT('Ctrl Pts',(-33.073965333831,-30.3495177349915,172.667787353183));
#34153=CARTESIAN_POINT('Ctrl Pts',(-31.1959266233527,-30.202513073665,172.556657563964));
#34154=CARTESIAN_POINT('Ctrl Pts',(-30.0537671473693,-31.7005489543862,
172.445527774744));
#34155=CARTESIAN_POINT('Ctrl Pts',(-30.6927788720971,-33.4726391846419,
172.334397985525));
#34156=CARTESIAN_POINT('Ctrl Pts',(-32.5281451968589,-33.8969860032201,
172.223268196305));
#34157=CARTESIAN_POINT('Ctrl Pts',(-33.8801587649515,-32.585231803608,172.112138407085));
#34158=CARTESIAN_POINT('Ctrl Pts',(-33.5114714208333,-30.7378798039084,
172.001008617865));
#34159=CARTESIAN_POINT('Ctrl Pts',(-31.7595018235935,-30.0456065205483,
171.889878828645));
#34160=CARTESIAN_POINT('Ctrl Pts',(-30.2276335493068,-31.1419729550677,
171.778749039426));
#34161=CARTESIAN_POINT('Ctrl Pts',(-30.3178158301807,-33.0235964361933,
171.667619250206));
#34162=CARTESIAN_POINT('Ctrl Pts',(-31.9475148207455,-33.9684355593559,
171.556489460986));
#34163=CARTESIAN_POINT('Ctrl Pts',(-33.625247678186,-33.1117838053908,171.445359671767));
#34164=CARTESIAN_POINT('Ctrl Pts',(-33.8155714856278,-31.2376395695253,
171.334229882547));
#34165=CARTESIAN_POINT('Ctrl Pts',(-32.3443039584759,-30.0611993321757,
171.223100093327));
#34166=CARTESIAN_POINT('Ctrl Pts',(-30.5579331823478,-30.6591284406011,
171.111970304108));
#34167=CARTESIAN_POINT('Ctrl Pts',(-30.0913263191716,-32.4842086590419,
171.000840514888));
#34168=CARTESIAN_POINT('Ctrl Pts',(-31.3715169099854,-33.8661463637517,
170.889710725668));
#34169=CARTESIAN_POINT('Ctrl Pts',(-33.2268884091652,-33.5402071538707,
170.778580936448));
#34170=CARTESIAN_POINT('Ctrl Pts',(-33.9594249413278,-31.8046870596182,
170.667451147228));
#34171=CARTESIAN_POINT('Ctrl Pts',(-32.8987170162659,-30.2479152503225,
170.556321358009));
#34172=CARTESIAN_POINT('Ctrl Pts',(-31.0155130240976,-30.2946324033638,
170.445191568789));
#34173=CARTESIAN_POINT('Ctrl Pts',(-30.0333008359585,-31.902083486905,170.334061779569));
#34174=CARTESIAN_POINT('Ctrl Pts',(-30.8509903947858,-33.5991467013704,
170.22293199035));
#34175=CARTESIAN_POINT('Ctrl Pts',(-32.7202410838149,-33.8326881967655,
170.11180220113));
#34176=CARTESIAN_POINT('Ctrl Pts',(-33.9303349436258,-32.3889733291566,
170.00067241191));
#34177=CARTESIAN_POINT('Ctrl Pts',(-33.3738071966412,-30.5892742889438,
169.88954262269));
#34178=CARTESIAN_POINT('Ctrl Pts',(-31.5599860016091,-30.0806561208062,
169.778412833471));
#34179=CARTESIAN_POINT('Ctrl Pts',(-30.1488608461515,-31.3286006564895,
169.667283044251));
#34180=CARTESIAN_POINT('Ctrl Pts',(-30.4318781695273,-33.1910025903301,
169.556153255031));
#34181=CARTESIAN_POINT('Ctrl Pts',(-32.1500235865798,-33.9634118693876,
169.445023465812));
#34182=CARTESIAN_POINT('Ctrl Pts',(-33.7308690441301,-32.938927897893,169.333893676592));
#34183=CARTESIAN_POINT('Ctrl Pts',(-33.7276419229907,-31.0551472965034,
169.222763887372));
#34184=CARTESIAN_POINT('Ctrl Pts',(-32.1432956494165,-30.0360856428375,
169.111634098152));
#34185=CARTESIAN_POINT('Ctrl Pts',(-30.427806751494,-30.8143771111138,169.000504308933));
#34186=CARTESIAN_POINT('Ctrl Pts',(-30.1511720648354,-32.6777377896899,
168.889374519713));
#34187=CARTESIAN_POINT('Ctrl Pts',(-31.5665646548229,-33.9208401930324,
168.778244730493));
#34188=CARTESIAN_POINT('Ctrl Pts',(-33.3786325721277,-33.4060104820908,
168.667114941273));
#34189=CARTESIAN_POINT('Ctrl Pts',(-33.9289909104319,-31.6044152260286,
168.555985152054));
#34190=CARTESIAN_POINT('Ctrl Pts',(-32.7139576858049,-30.1648548640671,
168.444855362834));
#34191=CARTESIAN_POINT('Ctrl Pts',(-30.8455181311833,-30.4047994314301,
168.333725573614));
#34192=CARTESIAN_POINT('Ctrl Pts',(-30.0336478600031,-32.1046542553599,
168.222595784394));
#34193=CARTESIAN_POINT('Ctrl Pts',(-31.0213617493879,-33.7087306489938,
168.111465995175));
#34194=CARTESIAN_POINT('Ctrl Pts',(-32.9047147401363,-33.7489952641838,
168.000336205955));
#34195=CARTESIAN_POINT('Ctrl Pts',(-33.9600826378061,-32.1885984191319,
167.889206416735));
#34196=CARTESIAN_POINT('Ctrl Pts',(-33.2216041088917,-30.4555982678176,
167.778076627516));
#34197=CARTESIAN_POINT('Ctrl Pts',(-31.3651268545137,-30.1360179929564,
167.666946838296));
#34198=CARTESIAN_POINT('Ctrl Pts',(-30.0896783996075,-31.5223335121504,
167.555817049076));
#34199=CARTESIAN_POINT('Ctrl Pts',(-30.5625360014067,-33.3458048821496,
167.444687259856));
#34200=CARTESIAN_POINT('Ctrl Pts',(-32.3509441608406,-33.9376088724108,
167.333557470637));
#34201=CARTESIAN_POINT('Ctrl Pts',(-33.8181738731966,-32.7561369761474,
167.222427681417));
#34202=CARTESIAN_POINT('Ctrl Pts',(-33.6214268214511,-30.8826511384421,
167.111297892197));
#34203=CARTESIAN_POINT('Ctrl Pts',(-31.9407751668869,-30.0317622245461,
167.000168102978));
#34204=CARTESIAN_POINT('Ctrl Pts',(-30.3143098808242,-30.9821600427646,
166.889038313758));
#34205=CARTESIAN_POINT('Ctrl Pts',(-30.2306015850745,-32.8641210565045,
166.777908524538));
#34206=CARTESIAN_POINT('Ctrl Pts',(-31.7661630409388,-33.9551519428074,
166.666778735318));
#34207=CARTESIAN_POINT('Ctrl Pts',(-33.5158608496493,-33.2570442475225,
166.555648946099));
#34208=CARTESIAN_POINT('Ctrl Pts',(-33.8779919057151,-31.4081056756153,
166.444519156879));
#34209=CARTESIAN_POINT('Ctrl Pts',(-32.5219495186972,-30.1016722048141,
166.333389367659));
#34210=CARTESIAN_POINT('Ctrl Pts',(-30.6871163143791,-30.5309113539161,
166.222259578439));
#34211=CARTESIAN_POINT('Ctrl Pts',(-30.0560997086199,-32.3080601037175,
166.11112978922));
#34212=CARTESIAN_POINT('Ctrl Pts',(-30.8184934910027,-33.2986349005748,
166.037043263073));
#34213=CARTESIAN_POINT('Ctrl Pts',(-31.3249228143252,-33.5230977622534,
166.));
#34214=CARTESIAN_POINT('Ctrl Pts',(-33.6638666881858,-31.9990537019747,
178.37851963661));
#34215=CARTESIAN_POINT('Ctrl Pts',(-33.6649866280482,-31.7834929812639,
178.364148625536));
#34216=CARTESIAN_POINT('Ctrl Pts',(-33.6261153890564,-31.5683196357392,
178.349777614463));
#34217=CARTESIAN_POINT('Ctrl Pts',(-33.5453802715361,-31.3702079301903,
178.33540660339));
#34218=CARTESIAN_POINT('Ctrl Pts',(-33.3372743712429,-30.8595476858231,
178.298363340316));
#34219=CARTESIAN_POINT('Ctrl Pts',(-32.8510157674951,-30.4622486839265,
178.261320077243));
#34220=CARTESIAN_POINT('Ctrl Pts',(-32.309123358114,-30.3601024542406,178.22427681417));
#34221=CARTESIAN_POINT('Ctrl Pts',(-31.7672309487329,-30.2579562245546,
178.187233551097));
#34222=CARTESIAN_POINT('Ctrl Pts',(-31.1697047337185,-30.4509627670793,
178.150190288024));
#34223=CARTESIAN_POINT('Ctrl Pts',(-30.7899647553863,-30.8508084125907,
178.11314702495));
#34224=CARTESIAN_POINT('Ctrl Pts',(-30.410224777054,-31.2506540581021,178.076103761877));
#34225=CARTESIAN_POINT('Ctrl Pts',(-30.2482710354039,-31.8573388066003,
178.039060498804));
#34226=CARTESIAN_POINT('Ctrl Pts',(-30.3782149995904,-32.3932445126879,
178.002017235731));
#34227=CARTESIAN_POINT('Ctrl Pts',(-30.5081589637769,-32.9291502187755,
177.964973972657));
#34228=CARTESIAN_POINT('Ctrl Pts',(-30.9300006337998,-33.3942768824526,
177.927930709584));
#34229=CARTESIAN_POINT('Ctrl Pts',(-31.4507064117268,-33.5757862894332,
177.890887446511));
#34230=CARTESIAN_POINT('Ctrl Pts',(-31.9714121896537,-33.7572956964137,
177.853844183438));
#34231=CARTESIAN_POINT('Ctrl Pts',(-32.5909820754846,-33.6551878466978,
177.816800920364));
#34232=CARTESIAN_POINT('Ctrl Pts',(-33.0259048074106,-33.3161861370186,
177.779757657291));
#34233=CARTESIAN_POINT('Ctrl Pts',(-33.4221146521209,-33.0073592928715,
177.746011650397));
#34234=CARTESIAN_POINT('Ctrl Pts',(-33.6650856313621,-32.5019339874448,
177.712265643504));
#34235=CARTESIAN_POINT('Ctrl Pts',(-33.6682333060465,-31.9991447275653,
177.67851963661));
#34236=CARTESIAN_POINT('Ctrl Pts',(-32.5301702171889,-33.9851743256717,
179.));
#34237=CARTESIAN_POINT('Ctrl Pts',(-32.5988282168344,-33.9597528138625,
179.));
#34238=CARTESIAN_POINT('Ctrl Pts',(-32.6657829343011,-33.9304405480476,
179.));
#34239=CARTESIAN_POINT('Ctrl Pts',(-32.7308455531179,-33.8975318719722,
179.));
#34240=CARTESIAN_POINT('Ctrl Pts',(-32.7977248428542,-33.8637043236487,
179.));
#34241=CARTESIAN_POINT('Ctrl Pts',(-32.8626056686009,-33.8260760354227,
179.));
#34242=CARTESIAN_POINT('Ctrl Pts',(-32.9252517375558,-33.7849220422036,
179.));
#34243=CARTESIAN_POINT('Ctrl Pts',(-32.9781830025095,-33.7501499813973,
179.));
#34244=CARTESIAN_POINT('Ctrl Pts',(-33.0295185420485,-33.7128598710975,
179.));
#34245=CARTESIAN_POINT('Ctrl Pts',(-33.0790930888641,-33.6731995961689,
179.));
#34246=CARTESIAN_POINT('Ctrl Pts',(-33.1011284696503,-33.6555710081884,
179.));
#34247=CARTESIAN_POINT('Ctrl Pts',(-33.1228156256912,-33.6374739649692,
179.));
#34248=CARTESIAN_POINT('Ctrl Pts',(-33.1441384887267,-33.6189207291506,
179.));
#34249=CARTESIAN_POINT('Ctrl Pts',(-33.1558499891621,-33.6087304358017,
179.));
#34250=CARTESIAN_POINT('Ctrl Pts',(-33.1674515751521,-33.5984025156165,
179.));
#34251=CARTESIAN_POINT('Ctrl Pts',(-33.1789404500937,-33.5879389587906,
179.));
#34252=CARTESIAN_POINT('Ctrl Pts',(-33.1895353200388,-33.5782896219933,
179.));
#34253=CARTESIAN_POINT('Ctrl Pts',(-33.2000357743432,-33.568523417913,179.));
#34254=CARTESIAN_POINT('Ctrl Pts',(-33.2104237260108,-33.5586573714086,
179.));
#34255=CARTESIAN_POINT('Ctrl Pts',(-33.2635074325071,-33.5082406642775,
179.));
#34256=CARTESIAN_POINT('Ctrl Pts',(-33.3137511044884,-33.4551351988,179.));
#34257=CARTESIAN_POINT('Ctrl Pts',(-33.3609361378531,-33.3996008414489,
179.));
#34258=CARTESIAN_POINT('Ctrl Pts',(-33.4077563290928,-33.3444958845135,
179.));
#34259=CARTESIAN_POINT('Ctrl Pts',(-33.4515655070966,-33.2869985673899,
179.));
#34260=CARTESIAN_POINT('Ctrl Pts',(-33.4921053042421,-33.2273385372884,
179.));
#34261=CARTESIAN_POINT('Ctrl Pts',(-33.5257899646654,-33.1777668078692,
179.));
#34262=CARTESIAN_POINT('Ctrl Pts',(-33.5572167980499,-33.1267012881111,
179.));
#34263=CARTESIAN_POINT('Ctrl Pts',(-33.586209996391,-33.0742672521662,179.));
#34264=CARTESIAN_POINT('Ctrl Pts',(-33.5983166726236,-33.0523723963699,
179.));
#34265=CARTESIAN_POINT('Ctrl Pts',(-33.6099986880749,-33.0302388812303,
179.));
#34266=CARTESIAN_POINT('Ctrl Pts',(-33.6212418007289,-33.0078757455458,
179.));
#34267=CARTESIAN_POINT('Ctrl Pts',(-33.6264400400048,-32.9975361773298,
179.));
#34268=CARTESIAN_POINT('Ctrl Pts',(-33.6315444442265,-32.9871475240125,
179.));
#34269=CARTESIAN_POINT('Ctrl Pts',(-33.6365535406754,-32.9767106809501,
179.));
#34270=CARTESIAN_POINT('Ctrl Pts',(-33.6417882346349,-32.965803787882,179.));
#34271=CARTESIAN_POINT('Ctrl Pts',(-33.646915240041,-32.9548517050336,179.));
#34272=CARTESIAN_POINT('Ctrl Pts',(-33.6519314793551,-32.9438597806135,
179.));
#34273=CARTESIAN_POINT('Ctrl Pts',(-33.6804723551455,-32.8813190743342,
179.));
#34274=CARTESIAN_POINT('Ctrl Pts',(-33.7054522044227,-32.8174462149676,
179.));
#34275=CARTESIAN_POINT('Ctrl Pts',(-33.726647601974,-32.752446031535,179.));
#34276=CARTESIAN_POINT('Ctrl Pts',(-33.7458438908687,-32.6935765389313,
179.));
#34277=CARTESIAN_POINT('Ctrl Pts',(-33.7619356221037,-32.633781749793,179.));
#34278=CARTESIAN_POINT('Ctrl Pts',(-33.7747201576386,-32.5732090252637,
179.));
#34279=CARTESIAN_POINT('Ctrl Pts',(-33.7898548837777,-32.5015011720726,
179.));
#34280=CARTESIAN_POINT('Ctrl Pts',(-33.800355329414,-32.4287015605003,179.));
#34281=CARTESIAN_POINT('Ctrl Pts',(-33.8062965446138,-32.355232863435,179.));
#34282=CARTESIAN_POINT('Ctrl Pts',(-33.8076038423758,-32.3390669007456,
179.));
#34283=CARTESIAN_POINT('Ctrl Pts',(-33.8086901718668,-32.3228686246414,
179.));
#34284=CARTESIAN_POINT('Ctrl Pts',(-33.8095559636441,-32.3066427023709,
179.));
#34285=CARTESIAN_POINT('Ctrl Pts',(-33.8104538965015,-32.2898144197184,
179.));
#34286=CARTESIAN_POINT('Ctrl Pts',(-33.8111146239095,-32.2729501736476,
179.));
#34287=CARTESIAN_POINT('Ctrl Pts',(-33.8115380624634,-32.2560895659403,
179.));
#34288=CARTESIAN_POINT('Ctrl Pts',(-33.8132597908656,-32.1875332502793,
179.));
#34289=CARTESIAN_POINT('Ctrl Pts',(-33.8110702051067,-32.1189505986289,
179.));
#34290=CARTESIAN_POINT('Ctrl Pts',(-33.8050897978935,-32.0506795924014,
179.));
#34291=CARTESIAN_POINT('Ctrl Pts',(-33.7991106060521,-31.9824224605892,
179.));
#34292=CARTESIAN_POINT('Ctrl Pts',(-33.7893416799664,-31.9144757768024,
179.));
#34293=CARTESIAN_POINT('Ctrl Pts',(-33.775853835733,-31.8471923584511,179.));
#34294=CARTESIAN_POINT('Ctrl Pts',(-33.7660958992626,-31.7985153934433,
179.));
#34295=CARTESIAN_POINT('Ctrl Pts',(-33.7543904437871,-31.7501858451891,
179.));
#34296=CARTESIAN_POINT('Ctrl Pts',(-33.7407500867331,-31.7023469553251,
179.));
#34297=CARTESIAN_POINT('Ctrl Pts',(-33.7305145998785,-31.6664494838438,
179.));
#34298=CARTESIAN_POINT('Ctrl Pts',(-33.7191893710348,-31.6308284441348,
179.));
#34299=CARTESIAN_POINT('Ctrl Pts',(-33.706775815965,-31.595548533918,179.));
#34300=CARTESIAN_POINT('Ctrl Pts',(-33.7026466613343,-31.5838132812991,
179.));
#34301=CARTESIAN_POINT('Ctrl Pts',(-33.6984002845091,-31.5721249678948,
179.));
#34302=CARTESIAN_POINT('Ctrl Pts',(-33.6940373283514,-31.560486148014,179.));
#34303=CARTESIAN_POINT('Ctrl Pts',(-33.6709143145649,-31.4988021468828,
179.));
#34304=CARTESIAN_POINT('Ctrl Pts',(-33.6445184276946,-31.4385017846299,
179.));
#34305=CARTESIAN_POINT('Ctrl Pts',(-33.6148995884413,-31.3799188808691,
179.));
#34306=CARTESIAN_POINT('Ctrl Pts',(-33.5940729902705,-31.3387260918518,
179.));
#34307=CARTESIAN_POINT('Ctrl Pts',(-33.5716520282499,-31.2983829870109,
179.));
#34308=CARTESIAN_POINT('Ctrl Pts',(-33.5476436633208,-31.2590169558985,
179.));
#34309=CARTESIAN_POINT('Ctrl Pts',(-33.5399305936275,-31.2463699912919,
179.));
#34310=CARTESIAN_POINT('Ctrl Pts',(-33.5320525316577,-31.2338222713431,
179.));
#34311=CARTESIAN_POINT('Ctrl Pts',(-33.524013020168,-31.2213836352321,179.));
#34312=CARTESIAN_POINT('Ctrl Pts',(-33.4897680757568,-31.1684002664396,
179.));
#34313=CARTESIAN_POINT('Ctrl Pts',(-33.4526667826938,-31.1175003544769,
179.));
#34314=CARTESIAN_POINT('Ctrl Pts',(-33.4127433144394,-31.0689988956573,
179.));
#34315=CARTESIAN_POINT('Ctrl Pts',(-33.3759774110677,-31.0243334388139,
179.));
#34316=CARTESIAN_POINT('Ctrl Pts',(-33.336817505376,-30.9817019587916,179.));
#34317=CARTESIAN_POINT('Ctrl Pts',(-33.2952688824592,-30.9413832873573,
179.));
#34318=CARTESIAN_POINT('Ctrl Pts',(-33.2874271850203,-30.933773725347,179.));
#34319=CARTESIAN_POINT('Ctrl Pts',(-33.2795003456115,-30.9262466517635,
179.));
#34320=CARTESIAN_POINT('Ctrl Pts',(-33.2714899711316,-30.9188027398162,
179.));
#34321=CARTESIAN_POINT('Origin',(-32.,-32.,172.));
#34322=CARTESIAN_POINT('Origin',(-32.,32.,166.));
#34323=CARTESIAN_POINT('Ctrl Pts',(-31.3249228143257,30.4769022377464,166.));
#34324=CARTESIAN_POINT('Ctrl Pts',(-31.2652496529217,30.4954852962336,166.));
#34325=CARTESIAN_POINT('Ctrl Pts',(-31.2068892521994,30.5176437837123,166.));
#34326=CARTESIAN_POINT('Ctrl Pts',(-31.149997930983,30.543078521238,166.));
#34327=CARTESIAN_POINT('Ctrl Pts',(-31.1139308250343,30.5592032543871,166.));
#34328=CARTESIAN_POINT('Ctrl Pts',(-31.0784541088344,30.57664585217,166.));
#34329=CARTESIAN_POINT('Ctrl Pts',(-31.0436085110974,30.5953405136239,166.));
#34330=CARTESIAN_POINT('Ctrl Pts',(-31.0200367372352,30.6079867691293,166.));
#34331=CARTESIAN_POINT('Ctrl Pts',(-30.9967537833441,30.6212061370888,166.));
#34332=CARTESIAN_POINT('Ctrl Pts',(-30.9737727083008,30.6349801542912,166.));
#34333=CARTESIAN_POINT('Ctrl Pts',(-30.9613018107735,30.6424547548808,166.));
#34334=CARTESIAN_POINT('Ctrl Pts',(-30.9489197191831,30.6500929212155,166.));
#34335=CARTESIAN_POINT('Ctrl Pts',(-30.9366411005164,30.6578835033087,166.));
#34336=CARTESIAN_POINT('Ctrl Pts',(-30.8809433698913,30.6932227995781,166.));
#34337=CARTESIAN_POINT('Ctrl Pts',(-30.8273088794392,30.7317322690669,166.));
#34338=CARTESIAN_POINT('Ctrl Pts',(-30.7759191889064,30.7731089876249,166.));
#34339=CARTESIAN_POINT('Ctrl Pts',(-30.7388357321088,30.8029669560067,166.));
#34340=CARTESIAN_POINT('Ctrl Pts',(-30.7029212833327,30.8343191918032,166.));
#34341=CARTESIAN_POINT('Ctrl Pts',(-30.6682493534813,30.8670677622712,166.));
#34342=CARTESIAN_POINT('Ctrl Pts',(-30.6588706375682,30.8759262117518,166.));
#34343=CARTESIAN_POINT('Ctrl Pts',(-30.6495828699885,30.884886899106,166.));
#34344=CARTESIAN_POINT('Ctrl Pts',(-30.6403875871116,30.893948033715,166.));
#34345=CARTESIAN_POINT('Ctrl Pts',(-30.6306791049162,30.9035148806733,166.));
#34346=CARTESIAN_POINT('Ctrl Pts',(-30.6210791487639,30.9131884173309,166.));
#34347=CARTESIAN_POINT('Ctrl Pts',(-30.611593764049,30.9229613523084,166.));
#34348=CARTESIAN_POINT('Ctrl Pts',(-30.5643377407046,30.9716499461109,166.));
#34349=CARTESIAN_POINT('Ctrl Pts',(-30.5198879151527,31.0228371550682,166.));
#34350=CARTESIAN_POINT('Ctrl Pts',(-30.4784277579538,31.0762154699866,166.));
#34351=CARTESIAN_POINT('Ctrl Pts',(-30.4363631767253,31.1303719569714,166.));
#34352=CARTESIAN_POINT('Ctrl Pts',(-30.3973751779897,31.1867844829168,166.));
#34353=CARTESIAN_POINT('Ctrl Pts',(-30.3616797296655,31.2451788214444,166.));
#34354=CARTESIAN_POINT('Ctrl Pts',(-30.3395644350503,31.2813573276974,166.));
#34355=CARTESIAN_POINT('Ctrl Pts',(-30.3187135104441,31.3182974422918,166.));
#34356=CARTESIAN_POINT('Ctrl Pts',(-30.299185233179,31.3559412292716,166.));
#34357=CARTESIAN_POINT('Ctrl Pts',(-30.2832061926244,31.3867433113299,166.));
#34358=CARTESIAN_POINT('Ctrl Pts',(-30.2681127925988,31.4180166428631,166.));
#34359=CARTESIAN_POINT('Ctrl Pts',(-30.2539402801135,31.4497316930281,166.));
#34360=CARTESIAN_POINT('Ctrl Pts',(-30.2481176636228,31.4627614627521,166.));
#34361=CARTESIAN_POINT('Ctrl Pts',(-30.2424496090511,31.475868333721,166.));
#34362=CARTESIAN_POINT('Ctrl Pts',(-30.2369477740253,31.4890276669845,166.));
#34363=CARTESIAN_POINT('Ctrl Pts',(-30.2097572377756,31.5540622102674,166.));
#34364=CARTESIAN_POINT('Ctrl Pts',(-30.1865718180333,31.6204869404992,166.));
#34365=CARTESIAN_POINT('Ctrl Pts',(-30.167602913195,31.6880061970132,166.));
#34366=CARTESIAN_POINT('Ctrl Pts',(-30.1654997751652,31.6954922547127,166.));
#34367=CARTESIAN_POINT('Ctrl Pts',(-30.1634485057444,31.7029918059433,166.));
#34368=CARTESIAN_POINT('Ctrl Pts',(-30.1614494212112,31.7105044754886,166.));
#34369=CARTESIAN_POINT('Ctrl Pts',(-30.1441093782497,31.7756693099455,166.));
#34370=CARTESIAN_POINT('Ctrl Pts',(-30.1306917361854,31.8418190894582,166.));
#34371=CARTESIAN_POINT('Ctrl Pts',(-30.121042543408,31.908649652992,166.));
#34372=CARTESIAN_POINT('Ctrl Pts',(-30.1106635819057,31.980534613952,166.));
#34373=CARTESIAN_POINT('Ctrl Pts',(-30.104644022139,32.0532080204044,166.));
#34374=CARTESIAN_POINT('Ctrl Pts',(-30.102852408182,32.1263138620071,166.));
#34375=CARTESIAN_POINT('Ctrl Pts',(-30.1025311237508,32.1394237000121,166.));
#34376=CARTESIAN_POINT('Ctrl Pts',(-30.1023459616189,32.1525474788775,166.));
#34377=CARTESIAN_POINT('Ctrl Pts',(-30.1022963720935,32.1656831804107,166.));
#34378=CARTESIAN_POINT('Ctrl Pts',(-30.1022518409735,32.1774789678619,166.));
#34379=CARTESIAN_POINT('Ctrl Pts',(-30.1023166880166,32.1892756806987,166.));
#34380=CARTESIAN_POINT('Ctrl Pts',(-30.1024899696769,32.201068577993,166.));
#34381=CARTESIAN_POINT('Ctrl Pts',(-30.103534091715,32.272127592208,166.));
#34382=CARTESIAN_POINT('Ctrl Pts',(-30.1085109983323,32.3430831832316,166.));
#34383=CARTESIAN_POINT('Ctrl Pts',(-30.1172406743503,32.4136000964793,166.));
#34384=CARTESIAN_POINT('Ctrl Pts',(-30.1261541338587,32.485601583085,166.));
#34385=CARTESIAN_POINT('Ctrl Pts',(-30.1389799843928,32.5571466616736,166.));
#34386=CARTESIAN_POINT('Ctrl Pts',(-30.1555792981318,32.627894619499,166.));
#34387=CARTESIAN_POINT('Ctrl Pts',(-30.1722789267301,32.6990701294235,166.));
#34388=CARTESIAN_POINT('Ctrl Pts',(-30.1927978434914,32.7694399245741,166.));
#34389=CARTESIAN_POINT('Ctrl Pts',(-30.2170469852316,32.838657990524,166.));
#34390=CARTESIAN_POINT('Ctrl Pts',(-30.2230311731062,32.8557395810976,166.));
#34391=CARTESIAN_POINT('Ctrl Pts',(-30.2292427770505,32.8727509916663,166.));
#34392=CARTESIAN_POINT('Ctrl Pts',(-30.2356809367261,32.8896869118155,166.));
#34393=CARTESIAN_POINT('Ctrl Pts',(-30.2407432797558,32.9030036733807,166.));
#34394=CARTESIAN_POINT('Ctrl Pts',(-30.2459464565493,32.9162753272425,166.));
#34395=CARTESIAN_POINT('Ctrl Pts',(-30.2512816393884,32.9294791679086,166.));
#34396=CARTESIAN_POINT('Ctrl Pts',(-30.2795038677291,32.9993252851818,166.));
#34397=CARTESIAN_POINT('Ctrl Pts',(-30.311462547048,33.0674005959196,166.));
#34398=CARTESIAN_POINT('Ctrl Pts',(-30.3469997305368,33.1333481914682,166.));
#34399=CARTESIAN_POINT('Ctrl Pts',(-30.382575226724,33.1993668852328,166.));
#34400=CARTESIAN_POINT('Ctrl Pts',(-30.4217371183794,33.2632543879031,166.));
#34401=CARTESIAN_POINT('Ctrl Pts',(-30.4643787112962,33.3246482023152,166.));
#34402=CARTESIAN_POINT('Ctrl Pts',(-30.5060510266821,33.3846464861954,166.));
#34403=CARTESIAN_POINT('Ctrl Pts',(-30.5510469865186,33.4422641424414,166.));
#34404=CARTESIAN_POINT('Ctrl Pts',(-30.5993123479533,33.4971432210983,166.));
#34405=CARTESIAN_POINT('Ctrl Pts',(-30.609639774304,33.5088857964396,166.));
#34406=CARTESIAN_POINT('Ctrl Pts',(-30.6201170449146,33.5205028855144,166.));
#34407=CARTESIAN_POINT('Ctrl Pts',(-30.6307438842162,33.5319907951258,166.));
#34408=CARTESIAN_POINT('Ctrl Pts',(-30.6398545795245,33.5418397108032,166.));
#34409=CARTESIAN_POINT('Ctrl Pts',(-30.6490752115469,33.5515936765095,166.));
#34410=CARTESIAN_POINT('Ctrl Pts',(-30.6584039191552,33.5612522752607,166.));
#34411=CARTESIAN_POINT('Ctrl Pts',(-31.6163320011529,34.0186125009919,166.));
#34412=CARTESIAN_POINT('Ctrl Pts',(-31.6906427588626,34.0256324377615,166.));
#34413=CARTESIAN_POINT('Ctrl Pts',(-31.7652023131977,34.0282488164819,166.));
#34414=CARTESIAN_POINT('Ctrl Pts',(-31.8396884813956,34.0266257252458,166.));
#34415=CARTESIAN_POINT('Ctrl Pts',(-31.9122243505307,34.0250451320115,166.));
#34416=CARTESIAN_POINT('Ctrl Pts',(-31.9846914092729,34.0194435195122,166.));
#34417=CARTESIAN_POINT('Ctrl Pts',(-32.0567789289828,34.0099285531527,166.));
#34418=CARTESIAN_POINT('Ctrl Pts',(-32.0728687183824,34.0078048318001,166.));
#34419=CARTESIAN_POINT('Ctrl Pts',(-32.0889416464922,34.0054856654506,166.));
#34420=CARTESIAN_POINT('Ctrl Pts',(-32.1049873135507,34.0029730647847,166.));
#34421=CARTESIAN_POINT('Ctrl Pts',(-32.1786235791049,33.9914423176246,166.));
#34422=CARTESIAN_POINT('Ctrl Pts',(-32.2515406184048,33.9758657941873,166.));
#34423=CARTESIAN_POINT('Ctrl Pts',(-32.3234063428329,33.9563835294395,166.));
#34424=CARTESIAN_POINT('Ctrl Pts',(-32.3738567719135,33.9427067923884,166.));
#34425=CARTESIAN_POINT('Ctrl Pts',(-32.4237888208937,33.9271041460939,166.));
#34426=CARTESIAN_POINT('Ctrl Pts',(-32.4730796607622,33.9096108952537,166.));
#34427=CARTESIAN_POINT('Ctrl Pts',(-32.4918010174038,33.902966711696,166.));
#34428=CARTESIAN_POINT('Ctrl Pts',(-32.5104297908714,33.8960496891882,166.));
#34429=CARTESIAN_POINT('Ctrl Pts',(-32.5289589179083,33.8888614002562,166.));
#34430=CARTESIAN_POINT('Ctrl Pts',(-32.5466609278563,33.8819939875644,166.));
#34431=CARTESIAN_POINT('Ctrl Pts',(-32.5642774649958,33.8748765254527,166.));
#34432=CARTESIAN_POINT('Ctrl Pts',(-32.5817714091896,33.8675236367515,166.));
#34433=CARTESIAN_POINT('Ctrl Pts',(-32.6487029413755,33.8393916099592,166.));
#34434=CARTESIAN_POINT('Ctrl Pts',(-32.7139143188879,33.8077914467863,166.));
#34435=CARTESIAN_POINT('Ctrl Pts',(-32.7770971725608,33.7728508117707,166.));
#34436=CARTESIAN_POINT('Ctrl Pts',(-32.8389245367741,33.7386597735164,166.));
#34437=CARTESIAN_POINT('Ctrl Pts',(-32.8988101782919,33.7012694276233,166.));
#34438=CARTESIAN_POINT('Ctrl Pts',(-32.9564327793223,33.660762586154,166.));
#34439=CARTESIAN_POINT('Ctrl Pts',(-33.0127910447732,33.6211445320697,166.));
#34440=CARTESIAN_POINT('Ctrl Pts',(-33.0669850520193,33.5785447170987,166.));
#34441=CARTESIAN_POINT('Ctrl Pts',(-33.1186737258448,33.53301341985,166.));
#34442=CARTESIAN_POINT('Ctrl Pts',(-33.1354926710747,33.5181980195313,166.));
#34443=CARTESIAN_POINT('Ctrl Pts',(-33.1520459961584,33.5030720531806,166.));
#34444=CARTESIAN_POINT('Ctrl Pts',(-33.1683208481947,33.4876367513471,166.));
#34445=CARTESIAN_POINT('Ctrl Pts',(-33.177455472586,33.4789733432682,166.));
#34446=CARTESIAN_POINT('Ctrl Pts',(-33.1865031947452,33.4702115198622,166.));
#34447=CARTESIAN_POINT('Ctrl Pts',(-33.195449274418,33.4613641289918,166.));
#34448=CARTESIAN_POINT('Ctrl Pts',(-33.2440183877757,33.4133308064843,166.));
#34449=CARTESIAN_POINT('Ctrl Pts',(-33.2896824911655,33.3626963940901,166.));
#34450=CARTESIAN_POINT('Ctrl Pts',(-33.3321490497204,33.3095423506968,166.));
#34451=CARTESIAN_POINT('Ctrl Pts',(-33.3382529548252,33.3019022864239,166.));
#34452=CARTESIAN_POINT('Ctrl Pts',(-33.3442907274727,33.2942101177445,166.));
#34453=CARTESIAN_POINT('Ctrl Pts',(-33.3502614231889,33.2864660381261,166.));
#34454=CARTESIAN_POINT('Ctrl Pts',(-33.392620387346,33.2315258424474,166.));
#34455=CARTESIAN_POINT('Ctrl Pts',(-33.4316073256674,33.1739742618556,166.));
#34456=CARTESIAN_POINT('Ctrl Pts',(-33.4671551192539,33.1141730601304,166.));
#34457=CARTESIAN_POINT('Ctrl Pts',(-33.5003163244037,33.0583867589698,166.));
#34458=CARTESIAN_POINT('Ctrl Pts',(-33.5304842720454,33.0006417881322,166.));
#34459=CARTESIAN_POINT('Ctrl Pts',(-33.557564760225,32.9412263929792,166.));
#34460=CARTESIAN_POINT('Ctrl Pts',(-33.563460103192,32.9282918354623,166.));
#34461=CARTESIAN_POINT('Ctrl Pts',(-33.569208978742,32.9152781209338,166.));
#34462=CARTESIAN_POINT('Ctrl Pts',(-33.5748101691781,32.9021882506626,166.));
#34463=CARTESIAN_POINT('Ctrl Pts',(-33.5793366711509,32.8916099058836,166.));
#34464=CARTESIAN_POINT('Ctrl Pts',(-33.5837664961298,32.8809821314316,166.));
#34465=CARTESIAN_POINT('Ctrl Pts',(-33.5880939820481,32.8703195344679,166.));
#34466=CARTESIAN_POINT('Ctrl Pts',(-33.6138044493615,32.8069708937352,166.));
#34467=CARTESIAN_POINT('Ctrl Pts',(-33.6359573309018,32.7422777280778,166.));
#34468=CARTESIAN_POINT('Ctrl Pts',(-33.654506474946,32.6765896583697,166.));
#34469=CARTESIAN_POINT('Ctrl Pts',(-33.672970327122,32.6112036326896,166.));
#34470=CARTESIAN_POINT('Ctrl Pts',(-33.6878635141003,32.5448306965761,166.));
#34471=CARTESIAN_POINT('Ctrl Pts',(-33.6990894526804,32.4778130439757,166.));
#34472=CARTESIAN_POINT('Ctrl Pts',(-33.7100753481424,32.4122284231156,166.));
#34473=CARTESIAN_POINT('Ctrl Pts',(-33.7175490214282,32.3460253994248,166.));
#34474=CARTESIAN_POINT('Ctrl Pts',(-33.7213720579008,32.2795375564111,166.));
#34475=CARTESIAN_POINT('Ctrl Pts',(-33.7221759064895,32.2655575279288,166.));
#34476=CARTESIAN_POINT('Ctrl Pts',(-33.7228181881339,32.2515649821506,166.));
#34477=CARTESIAN_POINT('Ctrl Pts',(-33.72329734684,32.2375631548068,166.));
#34478=CARTESIAN_POINT('Ctrl Pts',(-33.7237537386745,32.2242266139311,166.));
#34479=CARTESIAN_POINT('Ctrl Pts',(-33.7240620424032,32.2108797919198,166.));
#34480=CARTESIAN_POINT('Ctrl Pts',(-33.7242209355861,32.1975471702555,166.));
#34481=CARTESIAN_POINT('Ctrl Pts',(-33.7249995439963,32.1322146546463,166.));
#34482=CARTESIAN_POINT('Ctrl Pts',(-33.7221997863358,32.0671063303133,166.));
#34483=CARTESIAN_POINT('Ctrl Pts',(-33.715743471838,32.0025317991948,166.));
#34484=CARTESIAN_POINT('Ctrl Pts',(-33.7094097335377,31.9391832462227,166.));
#34485=CARTESIAN_POINT('Ctrl Pts',(-33.6995568087996,31.8763475422056,166.));
#34486=CARTESIAN_POINT('Ctrl Pts',(-33.6860642167824,31.8143341524862,166.));
#34487=CARTESIAN_POINT('Ctrl Pts',(-33.67300924081,31.7543320927102,166.));
#34488=CARTESIAN_POINT('Ctrl Pts',(-33.6565466301776,31.6950992468525,166.));
#34489=CARTESIAN_POINT('Ctrl Pts',(-33.6365261315778,31.6369428273527,166.));
#34490=CARTESIAN_POINT('Ctrl Pts',(-33.6332193297538,31.627337084862,166.));
#34491=CARTESIAN_POINT('Ctrl Pts',(-33.6298153744735,31.6177607817841,166.));
#34492=CARTESIAN_POINT('Ctrl Pts',(-33.6263134827184,31.6082153937475,166.));
#34493=CARTESIAN_POINT('Ctrl Pts',(-33.6225506333734,31.5979586926172,166.));
#34494=CARTESIAN_POINT('Ctrl Pts',(-33.6186747062679,31.5877376855654,166.));
#34495=CARTESIAN_POINT('Ctrl Pts',(-33.6146867573338,31.577553736751,166.));
#34496=CARTESIAN_POINT('Origin',(-32.,32.,180.545925280538));
#34497=CARTESIAN_POINT('Ctrl Pts',(-34.0565967526292,32.0015021117824,178.795925280538));
#34498=CARTESIAN_POINT('Ctrl Pts',(-34.0574112680809,32.0995962853728,178.790592107115));
#34499=CARTESIAN_POINT('Ctrl Pts',(-34.0064252466113,32.8782049323825,178.748215670618));
#34500=CARTESIAN_POINT('Ctrl Pts',(-33.0117514203349,34.2080115215553,178.668795971049));
#34501=CARTESIAN_POINT('Ctrl Pts',(-30.6939036908508,34.0474398623436,178.557666181829));
#34502=CARTESIAN_POINT('Ctrl Pts',(-29.5714225144095,32.0133607849434,178.446536392609));
#34503=CARTESIAN_POINT('Ctrl Pts',(-30.6715287936437,29.9669129302815,178.33540660339));
#34504=CARTESIAN_POINT('Ctrl Pts',(-32.9874474959699,29.7811936333636,178.22427681417));
#34505=CARTESIAN_POINT('Ctrl Pts',(-34.0018725639557,31.1064095882227,178.144449706553));
#34506=CARTESIAN_POINT('Ctrl Pts',(-34.0573013963354,31.8927552482639,178.101665862009));
#34507=CARTESIAN_POINT('Ctrl Pts',(-34.0563933814841,31.9983925126321,178.095925280538));
#34508=CARTESIAN_POINT('Ctrl Pts',(-34.0526600320705,31.9978184065947,178.854074719462));
#34509=CARTESIAN_POINT('Ctrl Pts',(-34.0491237090593,32.4678825338461,178.828629953495));
#34510=CARTESIAN_POINT('Ctrl Pts',(-33.6567302575586,33.6292028150091,178.766141924454));
#34511=CARTESIAN_POINT('Ctrl Pts',(-31.7283973209264,34.4129390290683,178.666610632341));
#34512=CARTESIAN_POINT('Ctrl Pts',(-29.8255894209646,33.0815150230766,178.555480843121));
#34513=CARTESIAN_POINT('Ctrl Pts',(-29.9119598436444,30.7594178093493,178.444351053902));
#34514=CARTESIAN_POINT('Ctrl Pts',(-31.9096840054244,29.5731212000867,178.333221264681));
#34515=CARTESIAN_POINT('Ctrl Pts',(-33.7208631602512,30.4738805049478,178.236462486535));
#34516=CARTESIAN_POINT('Ctrl Pts',(-34.0499397056807,31.5817357019626,178.176746971462));
#34517=CARTESIAN_POINT('Ctrl Pts',(-34.0521188506995,32.0011671092335,178.154074719462));
#34518=CARTESIAN_POINT('Ctrl Pts',(-30.7309291201472,33.079358653048,179.));
#34519=CARTESIAN_POINT('Ctrl Pts',(-30.3720428517591,32.6573931542732,178.962956736927));
#34520=CARTESIAN_POINT('Ctrl Pts',(-30.1149436779728,31.4341262709582,178.88887021078));
#34521=CARTESIAN_POINT('Ctrl Pts',(-31.4545465157447,30.1067578728411,178.777740421561));
#34522=CARTESIAN_POINT('Ctrl Pts',(-33.2939137175247,30.5161313123725,178.666610632341));
#34523=CARTESIAN_POINT('Ctrl Pts',(-33.9488255415399,32.2815517198011,178.555480843121));
#34524=CARTESIAN_POINT('Ctrl Pts',(-32.8203323354559,33.7902650906004,178.444351053901));
#34525=CARTESIAN_POINT('Ctrl Pts',(-30.9410115824103,33.6600729094363,178.333221264682));
#34526=CARTESIAN_POINT('Ctrl Pts',(-30.0308990918633,32.0108329810029,178.222091475462));
#34527=CARTESIAN_POINT('Ctrl Pts',(-30.9228699210173,30.3515643955951,178.110961686242));
#34528=CARTESIAN_POINT('Ctrl Pts',(-32.8006266106757,30.2009824033015,177.999831897022));
#34529=CARTESIAN_POINT('Ctrl Pts',(-33.9456545335462,31.6968142000849,177.888702107803));
#34530=CARTESIAN_POINT('Ctrl Pts',(-33.3100424795202,33.4701319121845,177.777572318583));
#34531=CARTESIAN_POINT('Ctrl Pts',(-31.4754927960691,33.8979941813415,177.666442529363));
#34532=CARTESIAN_POINT('Ctrl Pts',(-30.1209668886363,32.5888360297234,177.555312740143));
#34533=CARTESIAN_POINT('Ctrl Pts',(-30.4861114761055,30.7407799227021,177.444182950924));
#34534=CARTESIAN_POINT('Ctrl Pts',(-32.2367505368386,30.0451491638923,177.333053161704));
#34535=CARTESIAN_POINT('Ctrl Pts',(-33.7707180178967,31.1385763032121,177.221923372484));
#34536=CARTESIAN_POINT('Ctrl Pts',(-33.6841435990266,33.020369258459,177.110793583264));
#34537=CARTESIAN_POINT('Ctrl Pts',(-32.0562592086395,33.9683312403004,176.999663794045));
#34538=CARTESIAN_POINT('Ctrl Pts',(-30.3768870072247,33.1148978626103,176.888534004825));
#34539=CARTESIAN_POINT('Ctrl Pts',(-30.1829702116221,31.2411220290648,176.777404215605));
#34540=CARTESIAN_POINT('Ctrl Pts',(-31.6519793750709,30.0618630959102,176.666274426386));
#34541=CARTESIAN_POINT('Ctrl Pts',(-33.4394932395446,30.656366033717,176.555144637166));
#34542=CARTESIAN_POINT('Ctrl Pts',(-33.9095985022262,32.4805482090353,176.444014847946));
#34543=CARTESIAN_POINT('Ctrl Pts',(-32.6320599242147,33.8649378734601,176.332885058727));
#34544=CARTESIAN_POINT('Ctrl Pts',(-30.7760669580592,33.542556621148,176.221755269507));
#34545=CARTESIAN_POINT('Ctrl Pts',(-30.0402042388412,31.8084442771746,176.110625480287));
#34546=CARTESIAN_POINT('Ctrl Pts',(-31.0979253471581,30.2496416535512,175.999495691067));
#34547=CARTESIAN_POINT('Ctrl Pts',(-32.9812153951526,30.2927480066755,175.888365901848));
#34548=CARTESIAN_POINT('Ctrl Pts',(-33.9665077543468,31.898312869751,175.777236112628));
#34549=CARTESIAN_POINT('Ctrl Pts',(-33.1520735426487,33.5969406916609,175.666106323408));
#34550=CARTESIAN_POINT('Ctrl Pts',(-31.2832741184371,33.8340657106725,175.554976534188));
#34551=CARTESIAN_POINT('Ctrl Pts',(-30.0704144484628,32.3926736808866,175.443846744969));
#34552=CARTESIAN_POINT('Ctrl Pts',(-30.6234905497716,30.5919109567242,175.332716955749));
#34553=CARTESIAN_POINT('Ctrl Pts',(-32.4363331723059,30.0798160548769,175.221587166529));
#34554=CARTESIAN_POINT('Ctrl Pts',(-33.8498484073821,31.3250526760791,175.110457377309));
#34555=CARTESIAN_POINT('Ctrl Pts',(-33.5704024407928,33.1879937686345,174.99932758809));
#34556=CARTESIAN_POINT('Ctrl Pts',(-31.8537411906952,33.9636958473916,174.88819779887));
#34557=CARTESIAN_POINT('Ctrl Pts',(-30.2709344167626,32.9422447820107,174.77706800965));
#34558=CARTESIAN_POINT('Ctrl Pts',(-30.2705497136734,31.0584615103527,174.66593822043));
#34559=CARTESIAN_POINT('Ctrl Pts',(-31.8529391575229,30.0363640538602,174.554808431211));
#34560=CARTESIAN_POINT('Ctrl Pts',(-33.569917089599,30.8113649205297,174.443678641991));
#34561=CARTESIAN_POINT('Ctrl Pts',(-33.850123926316,32.6741917217198,174.332548852772));
#34562=CARTESIAN_POINT('Ctrl Pts',(-32.4371174094271,33.9200055704967,174.221419063552));
#34563=CARTESIAN_POINT('Ctrl Pts',(-30.6240657797714,33.4086511427483,174.110289274332));
#34564=CARTESIAN_POINT('Ctrl Pts',(-30.0702542270837,31.6081144653424,173.999159485112));
#34565=CARTESIAN_POINT('Ctrl Pts',(-31.2825250785475,30.1662271794333,173.888029695893));
#34566=CARTESIAN_POINT('Ctrl Pts',(-33.1514211974331,30.4025888924688,173.776899906673));
#34567=CARTESIAN_POINT('Ctrl Pts',(-33.9665491230709,32.1008839279147,173.665770117453));
#34568=CARTESIAN_POINT('Ctrl Pts',(-32.9819126176114,33.7068510865737,173.554640328233));
#34569=CARTESIAN_POINT('Ctrl Pts',(-31.0986403329129,33.7507266408298,173.443510539014));
#34570=CARTESIAN_POINT('Ctrl Pts',(-30.0402826406939,32.1923561592382,173.332380749794));
#34571=CARTESIAN_POINT('Ctrl Pts',(-30.7754370234621,30.4579434067276,173.221250960574));
#34572=CARTESIAN_POINT('Ctrl Pts',(-32.6312981625253,30.1348041254724,173.110121171354));
#34573=CARTESIAN_POINT('Ctrl Pts',(-33.9094020693888,31.518671881378,172.998991382135));
#34574=CARTESIAN_POINT('Ctrl Pts',(-33.4400419089509,33.3430459116603,172.887861592915));
#34575=CARTESIAN_POINT('Ctrl Pts',(-31.6527710100454,33.9382788883175,172.776731803695));
#34576=CARTESIAN_POINT('Ctrl Pts',(-30.1832803172047,32.7596200461458,172.665602014475));
#34577=CARTESIAN_POINT('Ctrl Pts',(-30.3764317765537,30.8857651754778,172.554472225256));
#34578=CARTESIAN_POINT('Ctrl Pts',(-32.0554552671365,30.031645932839,172.443342436036));
#34579=CARTESIAN_POINT('Ctrl Pts',(-33.6837266986233,30.9789429865549,172.332212646816));
#34580=CARTESIAN_POINT('Ctrl Pts',(-33.7710697147857,32.8607003460735,172.221082857597));
#34581=CARTESIAN_POINT('Ctrl Pts',(-32.2375489344276,33.9547540827722,172.109953068377));
#34582=CARTESIAN_POINT('Ctrl Pts',(-30.4866259453921,33.2598380813431,171.998823279157));
#34583=CARTESIAN_POINT('Ctrl Pts',(-30.1207264792757,31.4119319302438,171.887693489937));
#34584=CARTESIAN_POINT('Ctrl Pts',(-31.4747177594533,30.1022192992527,171.776563700718));
#34585=CARTESIAN_POINT('Ctrl Pts',(-33.3094416497307,30.5293349850108,171.665433911498));
#34586=CARTESIAN_POINT('Ctrl Pts',(-33.9457787424778,32.302387343789,171.554304122278));
#34587=CARTESIAN_POINT('Ctrl Pts',(-32.8013602312011,33.7986980847857,171.443174333058));
#34588=CARTESIAN_POINT('Ctrl Pts',(-30.9235455267189,33.648859844655,171.332044543839));
#34589=CARTESIAN_POINT('Ctrl Pts',(-30.030890282521,31.9900029558365,171.220914754619));
#34590=CARTESIAN_POINT('Ctrl Pts',(-30.9403428976541,30.340295253423,171.109784965399));
#34591=CARTESIAN_POINT('Ctrl Pts',(-32.8195822013514,30.2095313363283,170.99865517618));
#34592=CARTESIAN_POINT('Ctrl Pts',(-33.9487487623708,31.7173849234018,170.88752538696));
#34593=CARTESIAN_POINT('Ctrl Pts',(-33.2944415893687,33.4838847637451,170.77639559774));
#34594=CARTESIAN_POINT('Ctrl Pts',(-31.4554755114109,33.8923493603691,170.66526580852));
#34595=CARTESIAN_POINT('Ctrl Pts',(-30.1148523402876,32.5689563440575,170.554136019301));
#34596=CARTESIAN_POINT('Ctrl Pts',(-30.499495863758,30.7248606517391,170.443006230081));
#34597=CARTESIAN_POINT('Ctrl Pts',(-32.2573845004273,30.0477586626387,170.331876440861));
#34598=CARTESIAN_POINT('Ctrl Pts',(-33.7797176335243,31.1573267743156,170.220746651641));
#34599=CARTESIAN_POINT('Ctrl Pts',(-33.6732724886538,33.0381002837283,170.109616862422));
#34600=CARTESIAN_POINT('Ctrl Pts',(-32.035466508052,33.9688156712016,169.998487073202));
#34601=CARTESIAN_POINT('Ctrl Pts',(-30.3652019638992,33.0976923073081,169.887357283983));
#34602=CARTESIAN_POINT('Ctrl Pts',(-30.1910868537395,31.2219728477436,169.776227494763));
#34603=CARTESIAN_POINT('Ctrl Pts',(-31.672469438191,30.0582954005711,169.665097705543));
#34604=CARTESIAN_POINT('Ctrl Pts',(-33.4536044408894,30.6716449458862,169.553967916323));
#34605=CARTESIAN_POINT('Ctrl Pts',(-33.904416422969,32.5006906313158,169.442838127104));
#34606=CARTESIAN_POINT('Ctrl Pts',(-32.6123271472845,33.8715096807286,169.331708337884));
#34607=CARTESIAN_POINT('Ctrl Pts',(-30.7598427068146,33.5295433660167,169.220578548664));
#34608=CARTESIAN_POINT('Ctrl Pts',(-30.0423367721263,31.7877555499318,169.109448759444));
#34609=CARTESIAN_POINT('Ctrl Pts',(-31.1164629936058,30.2402115528575,168.998318970225));
#34610=CARTESIAN_POINT('Ctrl Pts',(-32.9991927017948,30.3032068584901,168.887189181005));
#34611=CARTESIAN_POINT('Ctrl Pts',(-33.9674720850595,31.9190888462911,168.776059391785));
#34612=CARTESIAN_POINT('Ctrl Pts',(-33.1351423524959,33.6090198444933,168.664929602565));
#34613=CARTESIAN_POINT('Ctrl Pts',(-31.263942648888,33.8263933301663,168.553799813346));
#34614=CARTESIAN_POINT('Ctrl Pts',(-30.0663746511061,32.3722714463651,168.442670024126));
#34615=CARTESIAN_POINT('Ctrl Pts',(-30.6384396027317,30.5774507722043,168.331540234906));
#34616=CARTESIAN_POINT('Ctrl Pts',(-32.4565898656643,30.0845317239336,168.220410445686));
#34617=CARTESIAN_POINT('Ctrl Pts',(-33.856874032538,31.3446284705168,168.109280656467));
#34618=CARTESIAN_POINT('Ctrl Pts',(-33.5577672269115,33.2045141316663,167.998150867247));
#34619=CARTESIAN_POINT('Ctrl Pts',(-31.8330087380771,33.9620415260158,167.887021078027));
#34620=CARTESIAN_POINT('Ctrl Pts',(-30.2610788624257,32.9239297848845,167.775891288808));
#34621=CARTESIAN_POINT('Ctrl Pts',(-30.2805907108729,31.0402475411786,167.664761499588));
#34622=CARTESIAN_POINT('Ctrl Pts',(-31.873687382455,30.0349203051936,167.553631710368));
#34623=CARTESIAN_POINT('Ctrl Pts',(-33.5823838127623,30.8280127657554,167.442501921148));
#34624=CARTESIAN_POINT('Ctrl Pts',(-33.8429001024036,32.6936950903751,167.331372131929));
#34625=CARTESIAN_POINT('Ctrl Pts',(-32.4168134615631,33.9245154823387,167.220242342709));
#34626=CARTESIAN_POINT('Ctrl Pts',(-30.6092651719059,33.3940395824034,167.109112553489));
#34627=CARTESIAN_POINT('Ctrl Pts',(-30.0744992385868,31.5877549816332,166.997982764269));
#34628=CARTESIAN_POINT('Ctrl Pts',(-31.301936984442,30.1587500931461,166.88685297505));
#34629=CARTESIAN_POINT('Ctrl Pts',(-33.1682216796882,30.4148421561058,166.77572318583));
#34630=CARTESIAN_POINT('Ctrl Pts',(-33.9653885256372,32.1216432990863,166.66459339661));
#34631=CARTESIAN_POINT('Ctrl Pts',(-32.9638002467904,33.7171385570736,166.553463607391));
#34632=CARTESIAN_POINT('Ctrl Pts',(-31.080260054756,33.7410849968787,166.442333818171));
#34633=CARTESIAN_POINT('Ctrl Pts',(-30.038236774059,32.1716953131642,166.331204028951));
#34634=CARTESIAN_POINT('Ctrl Pts',(-30.7920440433359,30.4449968588325,166.220074239731));
#34635=CARTESIAN_POINT('Ctrl Pts',(-32.6504510143993,30.1417770670916,166.108944450512));
#34636=CARTESIAN_POINT('Ctrl Pts',(-33.9154261131066,31.5384503702043,165.997814661292));
#34637=CARTESIAN_POINT('Ctrl Pts',(-33.4236059800711,33.3590424673056,165.886684872072));
#34638=CARTESIAN_POINT('Ctrl Pts',(-32.2331222331372,33.7401334029927,165.812598345926));
#34639=CARTESIAN_POINT('Ctrl Pts',(-31.6889203620492,33.6366995627947,165.775555082853));
#34640=CARTESIAN_POINT('Ctrl Pts',(-30.6322193753407,33.1633123698092,179.074814972382));
#34641=CARTESIAN_POINT('Ctrl Pts',(-30.2454185337562,32.7085259251263,179.037771709309));
#34642=CARTESIAN_POINT('Ctrl Pts',(-29.9683219002241,31.3901119828099,178.963685183163));
#34643=CARTESIAN_POINT('Ctrl Pts',(-31.4121205369524,29.959499394063,178.852555393943));
#34644=CARTESIAN_POINT('Ctrl Pts',(-33.3945557658816,30.4007143551266,178.741425604723));
#34645=CARTESIAN_POINT('Ctrl Pts',(-34.100407360122,32.303451125778,178.630295815503));
#34646=CARTESIAN_POINT('Ctrl Pts',(-32.8841386970822,33.9295139009187,178.519166026284));
#34647=CARTESIAN_POINT('Ctrl Pts',(-30.8586422852238,33.7891952270721,178.408036237064));
#34648=CARTESIAN_POINT('Ctrl Pts',(-29.877740232712,32.0116755823164,178.296906447845));
#34649=CARTESIAN_POINT('Ctrl Pts',(-30.8390895452261,30.2233472404906,178.185776658624));
#34650=CARTESIAN_POINT('Ctrl Pts',(-32.8629002391071,30.0610528133222,178.074646869405));
#34651=CARTESIAN_POINT('Ctrl Pts',(-34.0969897075991,31.6732320712899,177.963517080185));
#34652=CARTESIAN_POINT('Ctrl Pts',(-33.4119390409275,33.5844804077551,177.852387290965));
#34653=CARTESIAN_POINT('Ctrl Pts',(-31.434696042262,34.0456222801803,177.741257501746));
#34654=CARTESIAN_POINT('Ctrl Pts',(-29.9748136029135,32.634636351163,177.630127712526));
#34655=CARTESIAN_POINT('Ctrl Pts',(-30.3683595425993,30.6428363842767,177.518997923306));
#34656=CARTESIAN_POINT('Ctrl Pts',(-32.2551652569659,29.8930986911959,177.407868134087));
#34657=CARTESIAN_POINT('Ctrl Pts',(-33.908446435155,31.0715738097895,177.296738344867));
#34658=CARTESIAN_POINT('Ctrl Pts',(-33.815138161676,33.0997347144866,177.185608555647));
#34659=CARTESIAN_POINT('Ctrl Pts',(-32.0606351124727,34.1214302338311,177.074478766427));
#34660=CARTESIAN_POINT('Ctrl Pts',(-30.2506394730227,33.2016158586267,176.963348977208));
#34661=CARTESIAN_POINT('Ctrl Pts',(-30.0416396133364,31.1820956562754,176.852219187988));
#34662=CARTESIAN_POINT('Ctrl Pts',(-31.6249099437101,29.9111126514394,176.741089398768));
#34663=CARTESIAN_POINT('Ctrl Pts',(-33.5514586250734,30.5518566891006,176.629959609548));
#34664=CARTESIAN_POINT('Ctrl Pts',(-34.0581291980526,32.5179257833176,176.518829820329));
#34665=CARTESIAN_POINT('Ctrl Pts',(-32.681222248252,34.0099948158986,176.407700031109));
#34666=CARTESIAN_POINT('Ctrl Pts',(-30.6808680844989,33.6625383911503,176.296570241889));
#34667=CARTESIAN_POINT('Ctrl Pts',(-29.8877691443733,31.793544859958,176.18544045267));
#34668=CARTESIAN_POINT('Ctrl Pts',(-31.0277609771516,30.1134968341871,176.07431066345));
#34669=CARTESIAN_POINT('Ctrl Pts',(-33.0575354201357,30.1599560474108,175.96318087423));
#34670=CARTESIAN_POINT('Ctrl Pts',(-34.1194649151115,31.8904035316389,175.85205108501));
#34671=CARTESIAN_POINT('Ctrl Pts',(-33.2416831044143,33.7211525151669,175.740921295791));
#34672=CARTESIAN_POINT('Ctrl Pts',(-31.2275263820511,33.9767213819458,175.629791506571));
#34673=CARTESIAN_POINT('Ctrl Pts',(-29.9203291377064,32.4232162766138,175.518661717351));
#34674=CARTESIAN_POINT('Ctrl Pts',(-30.5164241134418,30.4823882245166,175.407531928131));
#34675=CARTESIAN_POINT('Ctrl Pts',(-32.4702716518446,29.9304620115263,175.296402138912));
#34676=CARTESIAN_POINT('Ctrl Pts',(-33.9937316743629,31.2725545223828,175.185272349692));
#34677=CARTESIAN_POINT('Ctrl Pts',(-33.692550089624,33.2803972455365,175.074142560472));
#34678=CARTESIAN_POINT('Ctrl Pts',(-31.8423650178026,34.1164342949053,174.963012771252));
#34679=CARTESIAN_POINT('Ctrl Pts',(-30.1364457722081,33.0155336293509,174.851882982033));
#34680=CARTESIAN_POINT('Ctrl Pts',(-30.1360311464846,30.9852275992181,174.740753192813));
#34681=CARTESIAN_POINT('Ctrl Pts',(-31.841500601598,29.8836302655325,174.629623403593));
#34682=CARTESIAN_POINT('Ctrl Pts',(-33.6920269872744,30.7189115617574,174.518493614374));
#34683=CARTESIAN_POINT('Ctrl Pts',(-33.9940286234659,32.7266311038364,174.407363825154));
#34684=CARTESIAN_POINT('Ctrl Pts',(-32.4711168878014,34.0693457396704,174.296234035934));
#34685=CARTESIAN_POINT('Ctrl Pts',(-30.5170440854709,33.5182175956782,174.185104246715));
#34686=CARTESIAN_POINT('Ctrl Pts',(-29.9201564541303,31.5776331725056,174.073974457495));
#34687=CARTESIAN_POINT('Ctrl Pts',(-31.2267190810055,30.0235942894783,173.962844668275));
#34688=CARTESIAN_POINT('Ctrl Pts',(-33.2409800190622,30.278340479493,173.851714879055));
#34689=CARTESIAN_POINT('Ctrl Pts',(-34.119509501541,32.1087307920557,173.740585089836));
#34690=CARTESIAN_POINT('Ctrl Pts',(-33.058286873333,33.8396118628653,173.629455300616));
#34691=CARTESIAN_POINT('Ctrl Pts',(-31.0285315752938,33.8869001065405,173.518325511396));
#34692=CARTESIAN_POINT('Ctrl Pts',(-29.8878536444094,32.2073178352894,173.407195722176));
#34693=CARTESIAN_POINT('Ctrl Pts',(-30.680189152888,30.3380005294497,173.296065932957));
#34694=CARTESIAN_POINT('Ctrl Pts',(-32.680401235891,29.9897271154239,173.184936143737));
#34695=CARTESIAN_POINT('Ctrl Pts',(-34.0579174864506,31.4812336448605,173.073806354517));
#34696=CARTESIAN_POINT('Ctrl Pts',(-33.5520499705965,33.4475095167339,172.962676565297));
#34697=CARTESIAN_POINT('Ctrl Pts',(-31.6257631529336,34.0890403764795,172.851546776078));
#34698=CARTESIAN_POINT('Ctrl Pts',(-30.0419738392762,32.8187041383706,172.740416986858));
#34699=CARTESIAN_POINT('Ctrl Pts',(-30.2501488340038,30.7990987513016,172.629287197638));
#34700=CARTESIAN_POINT('Ctrl Pts',(-32.0597686395054,29.8785451638096,172.518157408419));
#34701=CARTESIAN_POINT('Ctrl Pts',(-33.8146888342956,30.8995240361794,172.407027619199));
#34702=CARTESIAN_POINT('Ctrl Pts',(-33.9088254874194,32.9276465764729,172.295897829979));
#34703=CARTESIAN_POINT('Ctrl Pts',(-32.2560257548074,34.1067970298866,172.184768040759));
#34704=CARTESIAN_POINT('Ctrl Pts',(-30.3689140278794,33.3578296888105,172.07363825154));
#34705=CARTESIAN_POINT('Ctrl Pts',(-29.9745544942453,31.3661913415849,171.96250846232));
#34706=CARTESIAN_POINT('Ctrl Pts',(-31.433860722436,29.954607805172,171.8513786731));
#34707=CARTESIAN_POINT('Ctrl Pts',(-33.4112914779285,30.4149450241111,171.740248883881));
#34708=CARTESIAN_POINT('Ctrl Pts',(-34.0971235776395,32.3259073677782,171.629119094661));
#34709=CARTESIAN_POINT('Ctrl Pts',(-32.8636909214531,33.938602822773,171.517989305441));
#34710=CARTESIAN_POINT('Ctrl Pts',(-30.8398177002908,33.7771099976381,171.406859516221));
#34711=CARTESIAN_POINT('Ctrl Pts',(-29.8777307381692,31.9892253746203,171.295729727002));
#34712=CARTESIAN_POINT('Ctrl Pts',(-30.8579215894234,30.211201571904,171.184599937782));
#34713=CARTESIAN_POINT('Ctrl Pts',(-32.8833302167127,30.0702666918701,171.073470148562));
#34714=CARTESIAN_POINT('Ctrl Pts',(-34.1003246089838,31.6954028083503,170.962340359342));
#34715=CARTESIAN_POINT('Ctrl Pts',(-33.3951246961849,33.5993029714094,170.851210570123));
#34716=CARTESIAN_POINT('Ctrl Pts',(-31.4131217909349,34.0395383987531,170.740080780903));
#34717=CARTESIAN_POINT('Ctrl Pts',(-29.9682234581922,32.6132104014309,170.628950991683));
#34718=CARTESIAN_POINT('Ctrl Pts',(-30.3827849828128,30.625678894709,170.517821202464));
#34719=CARTESIAN_POINT('Ctrl Pts',(-32.2774041531966,29.8959111596577,170.406691413244));
#34720=CARTESIAN_POINT('Ctrl Pts',(-33.9181460508977,31.0917827133943,170.295561624024));
#34721=CARTESIAN_POINT('Ctrl Pts',(-33.8034214842449,33.1188448786261,170.184431834804));
#34722=CARTESIAN_POINT('Ctrl Pts',(-32.0382251325028,34.1219523443068,170.073302045585));
#34723=CARTESIAN_POINT('Ctrl Pts',(-30.2380455540284,33.1830720360928,169.962172256365));
#34724=CARTESIAN_POINT('Ctrl Pts',(-30.050387576907,31.1614570303288,169.851042467145));
#34725=CARTESIAN_POINT('Ctrl Pts',(-31.6469937467338,29.9072674567879,169.739912677925));
#34726=CARTESIAN_POINT('Ctrl Pts',(-33.5666674113567,30.5683240120554,169.628782888706));
#34727=CARTESIAN_POINT('Ctrl Pts',(-34.052544050906,32.5396349056103,169.517653099486));
#34728=CARTESIAN_POINT('Ctrl Pts',(-32.6599546339806,34.0170777856472,169.406523310266));
#34729=CARTESIAN_POINT('Ctrl Pts',(-30.6633818929439,33.6485129505583,169.295393521047));
#34730=CARTESIAN_POINT('Ctrl Pts',(-29.8900675484697,31.7712469404953,169.184263731827));
#34731=CARTESIAN_POINT('Ctrl Pts',(-31.0477405023622,30.1033332497709,169.073133942607));
#34732=CARTESIAN_POINT('Ctrl Pts',(-33.0769110216873,30.1712284003545,168.962004153387));
#34733=CARTESIAN_POINT('Ctrl Pts',(-34.1205042525398,31.9127954867463,168.850874364168));
#34734=CARTESIAN_POINT('Ctrl Pts',(-33.2234349874565,33.734171197944,168.739744574948));
#34735=CARTESIAN_POINT('Ctrl Pts',(-31.2066912892952,33.9684522351487,168.628614785728));
#34736=CARTESIAN_POINT('Ctrl Pts',(-29.9159751204173,32.4012271335949,168.517484996508));
#34737=CARTESIAN_POINT('Ctrl Pts',(-30.5325359203711,30.4668033107586,168.406355207289));
#34738=CARTESIAN_POINT('Ctrl Pts',(-32.4921039333468,29.935544470568,168.295225418069));
#34739=CARTESIAN_POINT('Ctrl Pts',(-34.001303760459,31.2936529438889,168.184095628849));
#34740=CARTESIAN_POINT('Ctrl Pts',(-33.678932094751,33.298202580783,168.07296583963));
#34741=CARTESIAN_POINT('Ctrl Pts',(-31.8200199719562,34.1146512985726,167.96183605041));
#34742=CARTESIAN_POINT('Ctrl Pts',(-30.1258236418911,32.9957940713738,167.85070626119));
#34743=CARTESIAN_POINT('Ctrl Pts',(-30.1468531436163,30.9655969272596,167.73957647197));
#34744=CARTESIAN_POINT('Ctrl Pts',(-31.8638626465465,29.8820742204885,167.628446682751));
#34745=CARTESIAN_POINT('Ctrl Pts',(-33.7054633860338,30.7368542949046,167.517316893531));
#34746=CARTESIAN_POINT('Ctrl Pts',(-33.9862429224935,32.7476514662021,167.406187104311));
#34747=CARTESIAN_POINT('Ctrl Pts',(-32.4492336762855,34.0742064374725,167.295057315092));
#34748=CARTESIAN_POINT('Ctrl Pts',(-30.5010922698608,33.5024695319151,167.183927525872));
#34749=CARTESIAN_POINT('Ctrl Pts',(-29.9247316473505,31.5556901055047,167.072797736652));
#34750=CARTESIAN_POINT('Ctrl Pts',(-31.2476408665352,30.0155356271018,166.961667947432));
#34751=CARTESIAN_POINT('Ctrl Pts',(-33.2590872615167,30.2915468156069,166.850538158212));
#34752=CARTESIAN_POINT('Ctrl Pts',(-34.1182586315479,32.1311048502107,166.739408368993));
#34753=CARTESIAN_POINT('Ctrl Pts',(-33.0387657021605,33.8506995042649,166.628278579773));
#34754=CARTESIAN_POINT('Ctrl Pts',(-31.0087216586548,33.8765085247972,166.517148790553));
#34755=CARTESIAN_POINT('Ctrl Pts',(-29.8856486479917,32.1850499656236,166.406019001334));
#34756=CARTESIAN_POINT('Ctrl Pts',(-30.698087885242,30.324046984657,166.294889212114));
#34757=CARTESIAN_POINT('Ctrl Pts',(-32.7010438178903,29.9972424201992,166.183759422894));
#34758=CARTESIAN_POINT('Ctrl Pts',(-34.0644100869902,31.5025505265502,166.072629633674));
#34759=CARTESIAN_POINT('Ctrl Pts',(-33.5343356368844,33.4647503022726,165.961499844455));
#34760=CARTESIAN_POINT('Ctrl Pts',(-32.2512547397663,33.8754829148802,165.887413318308));
#34761=CARTESIAN_POINT('Ctrl Pts',(-31.6647242417504,33.7640038755271,165.850370055235));
#34762=CARTESIAN_POINT('Ctrl Pts',(-30.5335096305342,33.2472660865704,179.149629944765));
#34763=CARTESIAN_POINT('Ctrl Pts',(-30.1187942157532,32.7596586959793,179.112586681692));
#34764=CARTESIAN_POINT('Ctrl Pts',(-29.8217001224754,31.3460976946617,179.038500155545));
#34765=CARTESIAN_POINT('Ctrl Pts',(-31.36969455816,29.8122409152849,178.927370366325));
#34766=CARTESIAN_POINT('Ctrl Pts',(-33.4951978142385,30.2852973978806,178.816240577106));
#34767=CARTESIAN_POINT('Ctrl Pts',(-34.2519891787042,32.325350531755,178.705110787886));
#34768=CARTESIAN_POINT('Ctrl Pts',(-32.9479450587086,34.068762711237,178.593980998666));
#34769=CARTESIAN_POINT('Ctrl Pts',(-30.7762729880373,33.9183175447078,178.482851209447));
#34770=CARTESIAN_POINT('Ctrl Pts',(-29.7245813735608,32.01251818363,178.371721420227));
#34771=CARTESIAN_POINT('Ctrl Pts',(-30.7553091694349,30.095130085386,178.260591631007));
#34772=CARTESIAN_POINT('Ctrl Pts',(-32.9251738675385,29.9211232233429,178.149461841787));
#34773=CARTESIAN_POINT('Ctrl Pts',(-34.2483248816519,31.649649942495,178.038332052568));
#34774=CARTESIAN_POINT('Ctrl Pts',(-33.5138356023347,33.6988289033257,177.927202263348));
#34775=CARTESIAN_POINT('Ctrl Pts',(-31.3938992884549,34.1932503790191,177.816072474128));
#34776=CARTESIAN_POINT('Ctrl Pts',(-29.8286603171907,32.6804366726026,177.704942684909));
#34777=CARTESIAN_POINT('Ctrl Pts',(-30.2506076090931,30.5448928458515,177.593812895689));
#34778=CARTESIAN_POINT('Ctrl Pts',(-32.2735799770931,29.7410482184995,177.482683106469));
#34779=CARTESIAN_POINT('Ctrl Pts',(-34.0461748524134,31.0045713163668,177.371553317249));
#34780=CARTESIAN_POINT('Ctrl Pts',(-33.9461327243253,33.1791001705142,177.26042352803));
#34781=CARTESIAN_POINT('Ctrl Pts',(-32.065011016306,34.2745292273619,177.14929373881));
#34782=CARTESIAN_POINT('Ctrl Pts',(-30.1243919388208,33.2883338546431,177.03816394959));
#34783=CARTESIAN_POINT('Ctrl Pts',(-29.9003090150507,31.1230692834861,176.92703416037));
#34784=CARTESIAN_POINT('Ctrl Pts',(-31.5978405123493,29.7603622069686,176.815904371151));
#34785=CARTESIAN_POINT('Ctrl Pts',(-33.6634240106023,30.4473473444842,176.704774581931));
#34786=CARTESIAN_POINT('Ctrl Pts',(-34.206659893879,32.5553033575998,176.593644792711));
#34787=CARTESIAN_POINT('Ctrl Pts',(-32.7303845722893,34.155051758337,176.482515003492));
#34788=CARTESIAN_POINT('Ctrl Pts',(-30.5856692109386,33.7825201611525,176.371385214272));
#34789=CARTESIAN_POINT('Ctrl Pts',(-29.7353340499054,31.7786454427414,176.260255425052));
#34790=CARTESIAN_POINT('Ctrl Pts',(-30.9575966071452,29.9773520148229,176.149125635832));
#34791=CARTESIAN_POINT('Ctrl Pts',(-33.1338554451188,30.0271640881461,176.037995846612));
#34792=CARTESIAN_POINT('Ctrl Pts',(-34.2724220758763,31.8824941935268,175.926866057393));
#34793=CARTESIAN_POINT('Ctrl Pts',(-33.3312926661799,33.845364338673,175.815736268173));
#34794=CARTESIAN_POINT('Ctrl Pts',(-31.171778645665,34.1193770532191,175.704606478954));
#34795=CARTESIAN_POINT('Ctrl Pts',(-29.7702438269501,32.453758872341,175.593476689734));
#34796=CARTESIAN_POINT('Ctrl Pts',(-30.409357677112,30.372865492309,175.482346900514));
#34797=CARTESIAN_POINT('Ctrl Pts',(-32.5042101313832,29.7811079681756,175.371217111294));
#34798=CARTESIAN_POINT('Ctrl Pts',(-34.1376149413436,31.2200563686864,175.260087322074));
#34799=CARTESIAN_POINT('Ctrl Pts',(-33.8146977384552,33.3728007224386,175.148957532855));
#34800=CARTESIAN_POINT('Ctrl Pts',(-31.83098884491,34.269172742419,175.037827743635));
#34801=CARTESIAN_POINT('Ctrl Pts',(-30.0019571276536,33.0888224766912,174.926697954415));
#34802=CARTESIAN_POINT('Ctrl Pts',(-30.0015125792959,30.9119936880836,174.815568165196));
#34803=CARTESIAN_POINT('Ctrl Pts',(-31.830062045673,29.7308964772048,174.704438375976));
#34804=CARTESIAN_POINT('Ctrl Pts',(-33.8141368849498,30.6264582029851,174.593308586756));
#34805=CARTESIAN_POINT('Ctrl Pts',(-34.1379333206158,32.7790704859529,174.482178797536));
#34806=CARTESIAN_POINT('Ctrl Pts',(-32.5051163661757,34.2186859088442,174.371049008317));
#34807=CARTESIAN_POINT('Ctrl Pts',(-30.4100223911704,33.6277840486081,174.259919219097));
#34808=CARTESIAN_POINT('Ctrl Pts',(-29.7700586811768,31.5471518796688,174.148789429877));
#34809=CARTESIAN_POINT('Ctrl Pts',(-31.1709130834636,29.8809613995232,174.037659640658));
#34810=CARTESIAN_POINT('Ctrl Pts',(-33.3305388406912,30.1540920665173,173.926529851438));
#34811=CARTESIAN_POINT('Ctrl Pts',(-34.2724698800112,32.1165776561968,173.815400062218));
#34812=CARTESIAN_POINT('Ctrl Pts',(-33.1346611290545,33.9723726391569,173.704270272998));
#34813=CARTESIAN_POINT('Ctrl Pts',(-30.9584228176748,34.0230735722514,173.593140483779));
#34814=CARTESIAN_POINT('Ctrl Pts',(-29.7354246481248,32.2222795113406,173.482010694559));
#34815=CARTESIAN_POINT('Ctrl Pts',(-30.584941282314,30.2180576521719,173.370880905339));
#34816=CARTESIAN_POINT('Ctrl Pts',(-32.7295043092566,29.8446501053754,173.259751116119));
#34817=CARTESIAN_POINT('Ctrl Pts',(-34.2064329035124,31.443795408343,173.1486213269));
#34818=CARTESIAN_POINT('Ctrl Pts',(-33.6640580322421,33.5519731218075,173.03749153768));
#34819=CARTESIAN_POINT('Ctrl Pts',(-31.5987552958217,34.2398018646414,172.92636174846));
#34820=CARTESIAN_POINT('Ctrl Pts',(-29.9006673613477,32.8777882305953,172.81523195924));
#34821=CARTESIAN_POINT('Ctrl Pts',(-30.1238658914538,30.7124323271253,172.704102170021));
#34822=CARTESIAN_POINT('Ctrl Pts',(-32.0640820118742,29.7254443947803,172.592972380801));
#34823=CARTESIAN_POINT('Ctrl Pts',(-33.9456509699678,30.8201050858039,172.481842591581));
#34824=CARTESIAN_POINT('Ctrl Pts',(-34.046581260053,32.9945928068723,172.370712802362));
#34825=CARTESIAN_POINT('Ctrl Pts',(-32.2745025751873,34.258839977001,172.259583013142));
#34826=CARTESIAN_POINT('Ctrl Pts',(-30.2512021103666,33.4558212962779,172.148453223922));
#34827=CARTESIAN_POINT('Ctrl Pts',(-29.828382509215,31.3204507529258,172.037323434703));
#34828=CARTESIAN_POINT('Ctrl Pts',(-31.3930036854187,29.8069963110913,171.926193645483));
#34829=CARTESIAN_POINT('Ctrl Pts',(-33.5131413061263,30.3005550632113,171.815063856263));
#34830=CARTESIAN_POINT('Ctrl Pts',(-34.2484684128012,32.3494273917673,171.703934067043));
#34831=CARTESIAN_POINT('Ctrl Pts',(-32.9260216117051,34.0785075607603,171.592804277824));
#34832=CARTESIAN_POINT('Ctrl Pts',(-30.7560898738626,33.9053601506212,171.481674488604));
#34833=CARTESIAN_POINT('Ctrl Pts',(-29.7245711938175,31.9884477934041,171.370544699384));
#34834=CARTESIAN_POINT('Ctrl Pts',(-30.7755002811927,30.0821078903851,171.259414910164));
#34835=CARTESIAN_POINT('Ctrl Pts',(-32.9470782320738,29.9310020474118,171.148285120945));
#34836=CARTESIAN_POINT('Ctrl Pts',(-34.2519004555968,31.6734206932988,171.037155331725));
#34837=CARTESIAN_POINT('Ctrl Pts',(-33.4958078030011,33.7147211790736,170.926025542505));
#34838=CARTESIAN_POINT('Ctrl Pts',(-31.3707680704589,34.1867274371371,170.814895753285));
#34839=CARTESIAN_POINT('Ctrl Pts',(-29.8215945760967,32.6574644588044,170.703765964066));
#34840=CARTESIAN_POINT('Ctrl Pts',(-30.2660741018676,30.5264971376789,170.592636174846));
#34841=CARTESIAN_POINT('Ctrl Pts',(-32.297423805966,29.7440636566767,170.481506385626));
#34842=CARTESIAN_POINT('Ctrl Pts',(-34.0565744682711,31.0262386524729,170.370376596407));
#34843=CARTESIAN_POINT('Ctrl Pts',(-33.9335704798359,33.1995894735239,170.259246807187));
#34844=CARTESIAN_POINT('Ctrl Pts',(-32.0409837569536,34.2750890174119,170.148117017967));
#34845=CARTESIAN_POINT('Ctrl Pts',(-30.1108891441576,33.2684517648776,170.036987228747));
#34846=CARTESIAN_POINT('Ctrl Pts',(-29.9096883000745,31.1009412129138,169.925857439528));
#34847=CARTESIAN_POINT('Ctrl Pts',(-31.6215180552765,29.7562395130049,169.814727650308));
#34848=CARTESIAN_POINT('Ctrl Pts',(-33.679730381824,30.4650030782245,169.703597861088));
#34849=CARTESIAN_POINT('Ctrl Pts',(-34.200671678843,32.5785791799048,169.592468071868));
#34850=CARTESIAN_POINT('Ctrl Pts',(-32.7075821206767,34.1626458905658,169.481338282649));
#34851=CARTESIAN_POINT('Ctrl Pts',(-30.5669210790731,33.7674825350999,169.370208493429));
#34852=CARTESIAN_POINT('Ctrl Pts',(-29.7377983248131,31.7547383310587,169.259078704209));
#34853=CARTESIAN_POINT('Ctrl Pts',(-30.9790180111186,29.9664549466843,169.147948914989));
#34854=CARTESIAN_POINT('Ctrl Pts',(-33.1546293415798,30.0392499422189,169.03681912577));
#34855=CARTESIAN_POINT('Ctrl Pts',(-34.2735364200202,31.9065021272017,168.92568933655));
#34856=CARTESIAN_POINT('Ctrl Pts',(-33.311727622417,33.8593225513948,168.81455954733));
#34857=CARTESIAN_POINT('Ctrl Pts',(-31.1494399297024,34.1105111401311,168.703429758111));
#34858=CARTESIAN_POINT('Ctrl Pts',(-29.7655755897285,32.4301828208247,168.592299968891));
#34859=CARTESIAN_POINT('Ctrl Pts',(-30.4266322380106,30.3561558493129,168.481170179671));
#34860=CARTESIAN_POINT('Ctrl Pts',(-32.5276180010293,29.7865572172026,168.370040390452));
#34861=CARTESIAN_POINT('Ctrl Pts',(-34.14573348838,31.2426774172609,168.258910601232));
#34862=CARTESIAN_POINT('Ctrl Pts',(-33.8000969625905,33.3918910298997,168.147780812012));
#34863=CARTESIAN_POINT('Ctrl Pts',(-31.8070312058352,34.2672610711293,168.036651022792));
#34864=CARTESIAN_POINT('Ctrl Pts',(-29.9905684213565,33.0676583578632,167.925521233573));
#34865=CARTESIAN_POINT('Ctrl Pts',(-30.0131155763598,30.8909463133407,167.814391444353));
#34866=CARTESIAN_POINT('Ctrl Pts',(-31.8540379106381,29.7292281357834,167.703261655133));
#34867=CARTESIAN_POINT('Ctrl Pts',(-33.8285429593054,30.6456958240537,167.592131865914));
#34868=CARTESIAN_POINT('Ctrl Pts',(-34.1295857425834,32.801607842029,167.481002076694));
#34869=CARTESIAN_POINT('Ctrl Pts',(-32.481653891008,34.2238973926065,167.369872287474));
#34870=CARTESIAN_POINT('Ctrl Pts',(-30.3929193678157,33.6108994814268,167.258742498254));
#34871=CARTESIAN_POINT('Ctrl Pts',(-29.7749640561141,31.5236252293763,167.147612709035));
#34872=CARTESIAN_POINT('Ctrl Pts',(-31.1933447486284,29.8723211610575,167.036482919815));
#34873=CARTESIAN_POINT('Ctrl Pts',(-33.3499528433452,30.1682514751079,166.925353130595));
#34874=CARTESIAN_POINT('Ctrl Pts',(-34.2711287374585,32.1405664013351,166.814223341375));
#34875=CARTESIAN_POINT('Ctrl Pts',(-33.1137311575306,33.9842604514563,166.703093552156));
#34876=CARTESIAN_POINT('Ctrl Pts',(-30.9371832625537,34.0119320527157,166.591963762936));
#34877=CARTESIAN_POINT('Ctrl Pts',(-29.7330605219244,32.1984046180832,166.480833973716));
#34878=CARTESIAN_POINT('Ctrl Pts',(-30.6041317271482,30.2030971104815,166.369704184496));
#34879=CARTESIAN_POINT('Ctrl Pts',(-32.7516366213812,29.8527077733068,166.258574395277));
#34880=CARTESIAN_POINT('Ctrl Pts',(-34.2133940608738,31.4666506828962,166.147444606057));
#34881=CARTESIAN_POINT('Ctrl Pts',(-33.6450652936977,33.5704581372396,166.036314816837));
#34882=CARTESIAN_POINT('Ctrl Pts',(-32.2693872463954,34.0108324267676,165.962228290691));
#34883=CARTESIAN_POINT('Ctrl Pts',(-31.6405281214516,33.8913081882595,165.925185027618));
#34884=CARTESIAN_POINT('Ctrl Pts',(-30.4347998857278,33.3312198033316,179.224444917147));
#34885=CARTESIAN_POINT('Ctrl Pts',(-29.9921698977503,32.8107914668324,179.187401654074));
#34886=CARTESIAN_POINT('Ctrl Pts',(-29.6750783447267,31.3020834065134,179.113315127928));
#34887=CARTESIAN_POINT('Ctrl Pts',(-31.3272685793676,29.6649824365068,179.002185338708));
#34888=CARTESIAN_POINT('Ctrl Pts',(-33.5958398625953,30.1698804406347,178.891055549488));
#34889=CARTESIAN_POINT('Ctrl Pts',(-34.4035709972863,32.3472499377319,178.779925760269));
#34890=CARTESIAN_POINT('Ctrl Pts',(-33.0117514203349,34.2080115215553,178.668795971049));
#34891=CARTESIAN_POINT('Ctrl Pts',(-30.6939036908508,34.0474398623436,178.557666181829));
#34892=CARTESIAN_POINT('Ctrl Pts',(-29.5714225144095,32.0133607849434,178.446536392609));
#34893=CARTESIAN_POINT('Ctrl Pts',(-30.6715287936437,29.9669129302815,178.33540660339));
#34894=CARTESIAN_POINT('Ctrl Pts',(-32.9874474959699,29.7811936333636,178.22427681417));
#34895=CARTESIAN_POINT('Ctrl Pts',(-34.3996600557047,31.6260678137,178.11314702495));
#34896=CARTESIAN_POINT('Ctrl Pts',(-33.615732163742,33.8131773988963,178.002017235731));
#34897=CARTESIAN_POINT('Ctrl Pts',(-31.3531025346477,34.3408784778579,177.890887446511));
#34898=CARTESIAN_POINT('Ctrl Pts',(-29.6825070314679,32.7262369940422,177.779757657291));
#34899=CARTESIAN_POINT('Ctrl Pts',(-30.1328556755869,30.4469493074261,177.668627868071));
#34900=CARTESIAN_POINT('Ctrl Pts',(-32.2919946972204,29.588997745803,177.557498078852));
#34901=CARTESIAN_POINT('Ctrl Pts',(-34.1839032696717,30.9375688229442,177.446368289632));
#34902=CARTESIAN_POINT('Ctrl Pts',(-34.0771272869747,33.2584656265418,177.335238500412));
#34903=CARTESIAN_POINT('Ctrl Pts',(-32.0693869201392,34.4276282208927,177.224108711192));
#34904=CARTESIAN_POINT('Ctrl Pts',(-29.9981444046188,33.3750518506594,177.112978921973));
#34905=CARTESIAN_POINT('Ctrl Pts',(-29.758978416765,31.0640429106968,177.001849132753));
#34906=CARTESIAN_POINT('Ctrl Pts',(-31.5707710809886,29.6096117624978,176.890719343533));
#34907=CARTESIAN_POINT('Ctrl Pts',(-33.7753893961311,30.3428379998679,176.779589554313));
#34908=CARTESIAN_POINT('Ctrl Pts',(-34.3551905897055,32.592680931882,176.668459765094));
#34909=CARTESIAN_POINT('Ctrl Pts',(-32.7795468963266,34.3001087007756,176.557329975874));
#34910=CARTESIAN_POINT('Ctrl Pts',(-30.4904703373783,33.9025019311548,176.446200186654));
#34911=CARTESIAN_POINT('Ctrl Pts',(-29.5828989554375,31.7637460255249,176.335070397434));
#34912=CARTESIAN_POINT('Ctrl Pts',(-30.8874322371387,29.8412071954588,176.223940608215));
#34913=CARTESIAN_POINT('Ctrl Pts',(-33.210175470102,29.8943721288814,176.112810818995));
#34914=CARTESIAN_POINT('Ctrl Pts',(-34.425379236641,31.8745848554147,176.001681029775));
#34915=CARTESIAN_POINT('Ctrl Pts',(-33.4209022279456,33.969576162179,175.890551240556));
#34916=CARTESIAN_POINT('Ctrl Pts',(-31.1160309092789,34.2620327244924,175.779421451336));
#34917=CARTESIAN_POINT('Ctrl Pts',(-29.6201585161938,32.4843014680682,175.668291662116));
#34918=CARTESIAN_POINT('Ctrl Pts',(-30.3022912407822,30.2633427601015,175.557161872896));
#34919=CARTESIAN_POINT('Ctrl Pts',(-32.5381486109218,29.631753924825,175.446032083677));
#34920=CARTESIAN_POINT('Ctrl Pts',(-34.2814982083244,31.1675582149901,175.334902294457));
#34921=CARTESIAN_POINT('Ctrl Pts',(-33.9368453872864,33.4652041993407,175.223772505237));
#34922=CARTESIAN_POINT('Ctrl Pts',(-31.8196126720174,34.4219111899327,175.112642716018));
#34923=CARTESIAN_POINT('Ctrl Pts',(-29.867468483099,33.1621113240314,175.001512926798));
#34924=CARTESIAN_POINT('Ctrl Pts',(-29.8669940121071,30.8387597769491,174.890383137578));
#34925=CARTESIAN_POINT('Ctrl Pts',(-31.8186234897481,29.5781626888771,174.779253348358));
#34926=CARTESIAN_POINT('Ctrl Pts',(-33.9362467826252,30.5340048442128,174.668123559139));
#34927=CARTESIAN_POINT('Ctrl Pts',(-34.2818380177658,32.8315098680694,174.556993769919));
#34928=CARTESIAN_POINT('Ctrl Pts',(-32.53911584455,34.368026078018,174.445863980699));
#34929=CARTESIAN_POINT('Ctrl Pts',(-30.3030006968699,33.737350501538,174.33473419148));
#34930=CARTESIAN_POINT('Ctrl Pts',(-29.6199609082234,31.516670586832,174.22360440226));
#34931=CARTESIAN_POINT('Ctrl Pts',(-31.1151070859216,29.7383285095682,174.11247461304));
#34932=CARTESIAN_POINT('Ctrl Pts',(-33.4200976623203,30.0298436535415,174.00134482382));
#34933=CARTESIAN_POINT('Ctrl Pts',(-34.4254302584813,32.1244245203378,173.8902150346));
#34934=CARTESIAN_POINT('Ctrl Pts',(-33.2110353847761,34.1051334154486,173.779085245381));
#34935=CARTESIAN_POINT('Ctrl Pts',(-30.8883140600557,34.1592470379621,173.667955456161));
#34936=CARTESIAN_POINT('Ctrl Pts',(-29.5829956518403,32.2372411873918,173.556825666941));
#34937=CARTESIAN_POINT('Ctrl Pts',(-30.48969341174,30.098114774894,173.445695877722));
#34938=CARTESIAN_POINT('Ctrl Pts',(-32.7786073826223,29.6995730953269,173.334566088502));
#34939=CARTESIAN_POINT('Ctrl Pts',(-34.3549483205742,31.4063571718256,173.223436299282));
#34940=CARTESIAN_POINT('Ctrl Pts',(-33.7760660938876,33.6564367268812,173.112306510062));
#34941=CARTESIAN_POINT('Ctrl Pts',(-31.5717474387099,34.3905633528034,173.001176720843));
#34942=CARTESIAN_POINT('Ctrl Pts',(-29.7593608834192,32.93687232282,172.890046931623));
#34943=CARTESIAN_POINT('Ctrl Pts',(-29.9975829489038,30.625765902949,172.778917142403));
#34944=CARTESIAN_POINT('Ctrl Pts',(-32.068395384243,29.5723436257509,172.667787353184));
#34945=CARTESIAN_POINT('Ctrl Pts',(-34.07661310564,30.7406861354284,172.556657563964));
#34946=CARTESIAN_POINT('Ctrl Pts',(-34.1843370326867,33.0615390372716,172.445527774744));
#34947=CARTESIAN_POINT('Ctrl Pts',(-32.2929793955673,34.4108829241154,172.334397985524));
#34948=CARTESIAN_POINT('Ctrl Pts',(-30.1334901928539,33.5538129037453,172.223268196305));
#34949=CARTESIAN_POINT('Ctrl Pts',(-29.6822105241847,31.2747101642669,172.112138407085));
#34950=CARTESIAN_POINT('Ctrl Pts',(-31.3521466484014,29.6593848170106,172.001008617865));
#34951=CARTESIAN_POINT('Ctrl Pts',(-33.6149911343242,30.1861651023115,171.889878828645));
#34952=CARTESIAN_POINT('Ctrl Pts',(-34.399813247963,32.3729474157566,171.778749039426));
#34953=CARTESIAN_POINT('Ctrl Pts',(-32.9883523019571,34.2184122987475,171.667619250206));
#34954=CARTESIAN_POINT('Ctrl Pts',(-30.6723620474344,34.0336103036043,171.556489460986));
#34955=CARTESIAN_POINT('Ctrl Pts',(-29.5714116494658,31.9876702121879,171.445359671767));
#34956=CARTESIAN_POINT('Ctrl Pts',(-30.693078972962,29.9530142088661,171.334229882547));
#34957=CARTESIAN_POINT('Ctrl Pts',(-33.0108262474351,29.7917374029535,171.223100093327));
#34958=CARTESIAN_POINT('Ctrl Pts',(-34.4034763022098,31.6514385782472,171.111970304107));
#34959=CARTESIAN_POINT('Ctrl Pts',(-33.5964909098172,33.8301393867379,171.000840514888));
#34960=CARTESIAN_POINT('Ctrl Pts',(-31.3284143499829,34.3339164755211,170.889710725668));
#34961=CARTESIAN_POINT('Ctrl Pts',(-29.6749656940012,32.7017185161778,170.778580936448));
#34962=CARTESIAN_POINT('Ctrl Pts',(-30.1493632209224,30.4273153806489,170.667451147228));
#34963=CARTESIAN_POINT('Ctrl Pts',(-32.3174434587353,29.5922161536956,170.556321358009));
#34964=CARTESIAN_POINT('Ctrl Pts',(-34.1950028856446,30.9606945915516,170.445191568789));
#34965=CARTESIAN_POINT('Ctrl Pts',(-34.063719475427,33.2803340684217,170.334061779569));
#34966=CARTESIAN_POINT('Ctrl Pts',(-32.0437423814044,34.4282256905171,170.22293199035));
#34967=CARTESIAN_POINT('Ctrl Pts',(-29.9837327342869,33.3538314936623,170.11180220113));
#34968=CARTESIAN_POINT('Ctrl Pts',(-29.768989023242,31.0404253954989,170.00067241191));
#34969=CARTESIAN_POINT('Ctrl Pts',(-31.5960423638194,29.6052115692218,169.88954262269));
#34970=CARTESIAN_POINT('Ctrl Pts',(-33.7927933522913,30.3616821443936,169.778412833471));
#34971=CARTESIAN_POINT('Ctrl Pts',(-34.3487993067801,32.6175234541993,169.667283044251));
#34972=CARTESIAN_POINT('Ctrl Pts',(-32.7552096073727,34.3082139954844,169.556153255031));
#34973=CARTESIAN_POINT('Ctrl Pts',(-30.4704602652025,33.8864521196416,169.445023465811));
#34974=CARTESIAN_POINT('Ctrl Pts',(-29.5855291011564,31.7382297216221,169.333893676592));
#34975=CARTESIAN_POINT('Ctrl Pts',(-30.9102955198749,29.8295766435978,169.222763887372));
#34976=CARTESIAN_POINT('Ctrl Pts',(-33.2323476614723,29.9072714840831,169.111634098152));
#34977=CARTESIAN_POINT('Ctrl Pts',(-34.4265685875006,31.900208767657,169.000504308933));
#34978=CARTESIAN_POINT('Ctrl Pts',(-33.4000202573775,33.9844739048455,168.889374519713));
#34979=CARTESIAN_POINT('Ctrl Pts',(-31.0921885701096,34.2525700451136,168.778244730493));
#34980=CARTESIAN_POINT('Ctrl Pts',(-29.6151760590397,32.4591385080545,168.667114941274));
#34981=CARTESIAN_POINT('Ctrl Pts',(-30.32072855565,30.2455083878672,168.555985152054));
#34982=CARTESIAN_POINT('Ctrl Pts',(-32.5631320687118,29.637569963837,168.444855362834));
#34983=CARTESIAN_POINT('Ctrl Pts',(-34.290163216301,31.1917018906329,168.333725573614));
#34984=CARTESIAN_POINT('Ctrl Pts',(-33.92126183043,33.4855794790164,168.222595784395));
#34985=CARTESIAN_POINT('Ctrl Pts',(-31.7940424397143,34.4198708436861,168.111465995175));
#34986=CARTESIAN_POINT('Ctrl Pts',(-29.8553132008219,33.1395226443526,168.000336205955));
#34987=CARTESIAN_POINT('Ctrl Pts',(-29.8793780091033,30.8162956994218,167.889206416735));
#34988=CARTESIAN_POINT('Ctrl Pts',(-31.8442131747296,29.5763820510783,167.778076627516));
#34989=CARTESIAN_POINT('Ctrl Pts',(-33.951622532577,30.5545373532029,167.666946838296));
#34990=CARTESIAN_POINT('Ctrl Pts',(-34.2729285626733,32.8555642178561,167.555817049076));
#34991=CARTESIAN_POINT('Ctrl Pts',(-32.5140741057304,34.3735883477403,167.444687259856));
#34992=CARTESIAN_POINT('Ctrl Pts',(-30.2847464657706,33.7193294309385,167.333557470637));
#34993=CARTESIAN_POINT('Ctrl Pts',(-29.6251964648778,31.4915603532478,167.222427681417));
#34994=CARTESIAN_POINT('Ctrl Pts',(-31.1390486307216,29.7291066950132,167.111297892197));
#34995=CARTESIAN_POINT('Ctrl Pts',(-33.4408184251737,30.0449561346089,167.000168102977));
#34996=CARTESIAN_POINT('Ctrl Pts',(-34.4239988433692,32.1500279524596,166.889038313758));
#34997=CARTESIAN_POINT('Ctrl Pts',(-33.1886966129007,34.1178213986476,166.777908524538));
#34998=CARTESIAN_POINT('Ctrl Pts',(-30.8656448664525,34.1473555806342,166.666778735318));
#34999=CARTESIAN_POINT('Ctrl Pts',(-29.580472395857,32.2117592705426,166.555648946099));
#35000=CARTESIAN_POINT('Ctrl Pts',(-30.5101755690543,30.0821472363061,166.444519156879));
#35001=CARTESIAN_POINT('Ctrl Pts',(-32.8022294248721,29.7081731264144,166.333389367659));
#35002=CARTESIAN_POINT('Ctrl Pts',(-34.3623780347574,31.4307508392421,166.222259578439));
#35003=CARTESIAN_POINT('Ctrl Pts',(-33.7557949505109,33.6761659722066,166.11112978922));
#35004=CARTESIAN_POINT('Ctrl Pts',(-32.2875197530244,34.146181938655,166.037043263073));
#35005=CARTESIAN_POINT('Ctrl Pts',(-31.6163320011528,34.0186125009919,166.));
#35006=CARTESIAN_POINT('Ctrl Pts',(-30.7309291201472,33.079358653048,179.));
#35007=CARTESIAN_POINT('Ctrl Pts',(-30.6856061922837,33.0370771716178,179.));
#35008=CARTESIAN_POINT('Ctrl Pts',(-30.6430136212517,32.9922261022954,179.));
#35009=CARTESIAN_POINT('Ctrl Pts',(-30.6031496794869,32.945150589125,179.));
#35010=CARTESIAN_POINT('Ctrl Pts',(-30.560649505517,32.894961937153,179.));
#35011=CARTESIAN_POINT('Ctrl Pts',(-30.5212500616914,32.8422446724269,179.));
#35012=CARTESIAN_POINT('Ctrl Pts',(-30.48497810544,32.7873623072376,179.));
#35013=CARTESIAN_POINT('Ctrl Pts',(-30.45324014372,32.7393402376969,179.));
#35014=CARTESIAN_POINT('Ctrl Pts',(-30.4238969086718,32.6896592869444,179.));
#35015=CARTESIAN_POINT('Ctrl Pts',(-30.3969892258523,32.638535416209,179.));
#35016=CARTESIAN_POINT('Ctrl Pts',(-30.3834950561993,32.6128968582681,179.));
#35017=CARTESIAN_POINT('Ctrl Pts',(-30.3706137909742,32.5868950488164,179.));
#35018=CARTESIAN_POINT('Ctrl Pts',(-30.3583529184774,32.560555386827,179.));
#35019=CARTESIAN_POINT('Ctrl Pts',(-30.3527381009956,32.5484932440519,179.));
#35020=CARTESIAN_POINT('Ctrl Pts',(-30.3472527987053,32.5363585364383,179.));
#35021=CARTESIAN_POINT('Ctrl Pts',(-30.3419062704107,32.5241737280056,179.));
#35022=CARTESIAN_POINT('Ctrl Pts',(-30.3149946729871,32.462841842872,179.));
#35023=CARTESIAN_POINT('Ctrl Pts',(-30.2915438746221,32.4001344020816,179.));
#35024=CARTESIAN_POINT('Ctrl Pts',(-30.2715771012512,32.3364093590736,179.));
#35025=CARTESIAN_POINT('Ctrl Pts',(-30.2512550505768,32.2715504292317,179.));
#35026=CARTESIAN_POINT('Ctrl Pts',(-30.2345415564051,32.2056365202545,179.));
#35027=CARTESIAN_POINT('Ctrl Pts',(-30.221500425048,32.1390085160714,179.));
#35028=CARTESIAN_POINT('Ctrl Pts',(-30.210592737675,32.0832804185613,179.));
#35029=CARTESIAN_POINT('Ctrl Pts',(-30.2022547019689,32.0270518158213,179.));
#35030=CARTESIAN_POINT('Ctrl Pts',(-30.1965484750337,31.9705098819633,179.));
#35031=CARTESIAN_POINT('Ctrl Pts',(-30.1939213248785,31.9444779431711,179.));
#35032=CARTESIAN_POINT('Ctrl Pts',(-30.1918523706069,31.9183794749991,179.));
#35033=CARTESIAN_POINT('Ctrl Pts',(-30.1903494767592,31.8922323434201,179.));
#35034=CARTESIAN_POINT('Ctrl Pts',(-30.1896915558872,31.880785930464,179.));
#35035=CARTESIAN_POINT('Ctrl Pts',(-30.1891422311578,31.8693303524252,179.));
#35036=CARTESIAN_POINT('Ctrl Pts',(-30.1887025004782,31.8578813236233,179.));
#35037=CARTESIAN_POINT('Ctrl Pts',(-30.1860088953412,31.7877493900974,179.));
#35038=CARTESIAN_POINT('Ctrl Pts',(-30.1874154015388,31.7177317874487,179.));
#35039=CARTESIAN_POINT('Ctrl Pts',(-30.1929763607359,31.6481896277696,179.));
#35040=CARTESIAN_POINT('Ctrl Pts',(-30.1979465359268,31.5860354733315,179.));
#35041=CARTESIAN_POINT('Ctrl Pts',(-30.2062356846863,31.5242601439434,179.));
#35042=CARTESIAN_POINT('Ctrl Pts',(-30.2179157014571,31.4631093275663,179.));
#35043=CARTESIAN_POINT('Ctrl Pts',(-30.2306454337487,31.39646271762,179.));
#35044=CARTESIAN_POINT('Ctrl Pts',(-30.2474018272177,31.3305570843581,179.));
#35045=CARTESIAN_POINT('Ctrl Pts',(-30.26793982867,31.2656058366414,179.));
#35046=CARTESIAN_POINT('Ctrl Pts',(-30.2758705976169,31.2405248500787,179.));
#35047=CARTESIAN_POINT('Ctrl Pts',(-30.2843658062738,31.2155862217279,179.));
#35048=CARTESIAN_POINT('Ctrl Pts',(-30.2934133562222,31.1908025609492,179.));
#35049=CARTESIAN_POINT('Ctrl Pts',(-30.2973810315899,31.1799340362157,179.));
#35050=CARTESIAN_POINT('Ctrl Pts',(-30.3014548316538,31.1690958722154,179.));
#35051=CARTESIAN_POINT('Ctrl Pts',(-30.3056286457748,31.1583016836734,179.));
#35052=CARTESIAN_POINT('Ctrl Pts',(-30.3308501602472,31.0930745857145,179.));
#35053=CARTESIAN_POINT('Ctrl Pts',(-30.3597620928403,31.0293339906667,179.));
#35054=CARTESIAN_POINT('Ctrl Pts',(-30.3920519767111,30.9672985237551,179.));
#35055=CARTESIAN_POINT('Ctrl Pts',(-30.4250886868533,30.9038282509261,179.));
#35056=CARTESIAN_POINT('Ctrl Pts',(-30.461661713349,30.8421420744079,179.));
#35057=CARTESIAN_POINT('Ctrl Pts',(-30.5014925323278,30.7824778732566,179.));
#35058=CARTESIAN_POINT('Ctrl Pts',(-30.5319853636164,30.7368014230525,179.));
#35059=CARTESIAN_POINT('Ctrl Pts',(-30.5643887377804,30.6923099804802,179.));
#35060=CARTESIAN_POINT('Ctrl Pts',(-30.5985972405943,30.6491163876609,179.));
#35061=CARTESIAN_POINT('Ctrl Pts',(-30.6198995701376,30.6222188600665,179.));
#35062=CARTESIAN_POINT('Ctrl Pts',(-30.6419022174088,30.5958247363827,179.));
#35063=CARTESIAN_POINT('Ctrl Pts',(-30.6645826385146,30.569962958019,179.));
#35064=CARTESIAN_POINT('Ctrl Pts',(-30.6772410040684,30.555529017711,179.));
#35065=CARTESIAN_POINT('Ctrl Pts',(-30.6901149391436,30.5412563906713,179.));
#35066=CARTESIAN_POINT('Ctrl Pts',(-30.7031769103107,30.5271754384393,179.));
#35067=CARTESIAN_POINT('Ctrl Pts',(-30.7540414015774,30.4723429432007,179.));
#35068=CARTESIAN_POINT('Ctrl Pts',(-30.807802406251,30.4203555265443,179.));
#35069=CARTESIAN_POINT('Ctrl Pts',(-30.8641752460904,30.3714768709713,179.));
#35070=CARTESIAN_POINT('Ctrl Pts',(-30.9063225488272,30.3349326149134,179.));
#35071=CARTESIAN_POINT('Ctrl Pts',(-30.9499309830963,30.3001263070555,179.));
#35072=CARTESIAN_POINT('Ctrl Pts',(-30.9948979518231,30.2671778872202,179.));
#35073=CARTESIAN_POINT('Ctrl Pts',(-31.0089817993794,30.2568583007477,179.));
#35074=CARTESIAN_POINT('Ctrl Pts',(-31.0231990077974,30.2467210444674,179.));
#35075=CARTESIAN_POINT('Ctrl Pts',(-31.0375466674535,30.2367700313995,179.));
#35076=CARTESIAN_POINT('Ctrl Pts',(-31.0513256752561,30.2272134145022,179.));
#35077=CARTESIAN_POINT('Ctrl Pts',(-31.0652179378318,30.217833529893,179.));
#35078=CARTESIAN_POINT('Ctrl Pts',(-31.079215554219,30.2086365513038,179.));
#35079=CARTESIAN_POINT('Ctrl Pts',(-31.14216376158,30.1672771298632,179.));
#35080=CARTESIAN_POINT('Ctrl Pts',(-31.2072699777245,30.1295929755988,179.));
#35081=CARTESIAN_POINT('Ctrl Pts',(-31.2742731900079,30.095863022087,179.));
#35082=CARTESIAN_POINT('Ctrl Pts',(-31.325457897845,30.0700962303613,179.));
#35083=CARTESIAN_POINT('Ctrl Pts',(-31.377750599829,30.0466373808211,179.));
#35084=CARTESIAN_POINT('Ctrl Pts',(-31.4310487708202,30.0256260323555,179.));
#35085=CARTESIAN_POINT('Ctrl Pts',(-31.4435331822408,30.0207043940728,179.));
#35086=CARTESIAN_POINT('Ctrl Pts',(-31.4560728052128,30.0159171103945,179.));
#35087=CARTESIAN_POINT('Ctrl Pts',(-31.4686656825472,30.0112635882184,179.));
#35088=CARTESIAN_POINT('Ctrl Pts',(-33.6673324606655,31.9986966424362,177.87148036339));
#35089=CARTESIAN_POINT('Ctrl Pts',(-33.6680686829516,31.9130455012085,177.877220944861));
#35090=CARTESIAN_POINT('Ctrl Pts',(-33.662038537116,31.8274983445442,177.882961526332));
#35091=CARTESIAN_POINT('Ctrl Pts',(-33.6488812040635,31.7430618526376,177.888702107803));
#35092=CARTESIAN_POINT('Ctrl Pts',(-33.5639785592561,31.1982036011571,177.925745370876));
#35093=CARTESIAN_POINT('Ctrl Pts',(-33.1823025849659,30.6995930022293,177.962788633949));
#35094=CARTESIAN_POINT('Ctrl Pts',(-32.6785051495444,30.475384701481,177.999831897022));
#35095=CARTESIAN_POINT('Ctrl Pts',(-32.1747077141229,30.2511764007327,178.036875160096));
#35096=CARTESIAN_POINT('Ctrl Pts',(-31.5487888175701,30.3013703981639,178.073918423169));
#35097=CARTESIAN_POINT('Ctrl Pts',(-31.0871675644347,30.6030121611142,178.110961686242));
#35098=CARTESIAN_POINT('Ctrl Pts',(-30.6255463112993,30.9046539240644,178.148004949315));
#35099=CARTESIAN_POINT('Ctrl Pts',(-30.3282227015813,31.4577434525337,178.185048212389));
#35100=CARTESIAN_POINT('Ctrl Pts',(-30.3312463118135,32.0091615381739,178.222091475462));
#35101=CARTESIAN_POINT('Ctrl Pts',(-30.3342699220457,32.5605796238141,178.259134738535));
#35102=CARTESIAN_POINT('Ctrl Pts',(-30.637640752228,33.1103262666252,178.296178001608));
#35103=CARTESIAN_POINT('Ctrl Pts',(-31.1025462928267,33.4068982848914,178.333221264682));
#35104=CARTESIAN_POINT('Ctrl Pts',(-31.5674518334255,33.7034703031577,178.370264527755));
#35105=CARTESIAN_POINT('Ctrl Pts',(-32.1938920844407,33.746867696879,178.407307790828));
#35106=CARTESIAN_POINT('Ctrl Pts',(-32.6951944109623,33.5171141652731,178.444351053901));
#35107=CARTESIAN_POINT('Ctrl Pts',(-33.1964967374839,33.2873606336673,178.481394316975));
#35108=CARTESIAN_POINT('Ctrl Pts',(-33.5726611395119,32.7844561767342,178.518437580048));
#35109=CARTESIAN_POINT('Ctrl Pts',(-33.6515913698567,32.2387672136962,178.555480843121));
#35110=CARTESIAN_POINT('Ctrl Pts',(-33.6629550719668,32.1602035658563,178.560814016544));
#35111=CARTESIAN_POINT('Ctrl Pts',(-33.668157767428,32.08075308988,178.566147189967));
#35112=CARTESIAN_POINT('Ctrl Pts',(-33.6674973548511,32.0012179185931,178.57148036339));
#35113=CARTESIAN_POINT('Ctrl Pts',(-32.5301702171895,30.0148256743285,179.));
#35114=CARTESIAN_POINT('Ctrl Pts',(-33.1902397907536,30.1911070339307,178.962956736927));
#35115=CARTESIAN_POINT('Ctrl Pts',(-34.3091777184327,31.251637720013,178.88887021078));
#35116=CARTESIAN_POINT('Ctrl Pts',(-33.8814411350113,33.5378731234361,178.77774042156));
#35117=CARTESIAN_POINT('Ctrl Pts',(-31.7283973209264,34.4129390290683,178.666610632341));
#35118=CARTESIAN_POINT('Ctrl Pts',(-29.8255894209646,33.0815150230766,178.555480843121));
#35119=CARTESIAN_POINT('Ctrl Pts',(-29.9119598436444,30.7594178093493,178.444351053902));
#35120=CARTESIAN_POINT('Ctrl Pts',(-31.9096840054244,29.5731212000867,178.333221264681));
#35121=CARTESIAN_POINT('Ctrl Pts',(-33.9898669259929,30.6076649759035,178.222091475462));
#35122=CARTESIAN_POINT('Ctrl Pts',(-34.249042199873,32.9165631725329,178.110961686242));
#35123=CARTESIAN_POINT('Ctrl Pts',(-32.4498708069788,34.3865813639729,177.999831897023));
#35124=CARTESIAN_POINT('Ctrl Pts',(-30.239005926868,33.6724513835904,177.888702107803));
#35125=CARTESIAN_POINT('Ctrl Pts',(-29.6397722337213,31.4276996511778,177.777572318583));
#35126=CARTESIAN_POINT('Ctrl Pts',(-31.2005990409054,29.7067170736135,177.666442529363));
#35127=CARTESIAN_POINT('Ctrl Pts',(-33.4930261644715,30.0845191734353,177.555312740144));
#35128=CARTESIAN_POINT('Ctrl Pts',(-34.4190532951284,32.2153500204183,177.444182950924));
#35129=CARTESIAN_POINT('Ctrl Pts',(-33.1311884148471,34.1490941434474,177.333053161704));
#35130=CARTESIAN_POINT('Ctrl Pts',(-30.8080724930038,34.1160109663009,177.221923372484));
#35131=CARTESIAN_POINT('Ctrl Pts',(-29.5757955383114,32.1463773261312,177.110793583265));
#35132=CARTESIAN_POINT('Ctrl Pts',(-30.5621242967963,30.0427808298698,176.999663794045));
#35133=CARTESIAN_POINT('Ctrl Pts',(-32.8643812668194,29.7304100510143,176.888534004825));
#35134=CARTESIAN_POINT('Ctrl Pts',(-34.3755658943906,31.4951434013914,176.777404215606));
#35135=CARTESIAN_POINT('Ctrl Pts',(-33.7126583679654,33.7219160257557,176.666274426386));
#35136=CARTESIAN_POINT('Ctrl Pts',(-31.4823444807967,34.3728097817195,176.555144637166));
#35137=CARTESIAN_POINT('Ctrl Pts',(-29.7257833087973,32.8521337550634,176.444014847946));
#35138=CARTESIAN_POINT('Ctrl Pts',(-30.0505605908462,30.5515941579779,176.332885058727));
#35139=CARTESIAN_POINT('Ctrl Pts',(-32.1594436788161,29.5766198796149,176.221755269507));
#35140=CARTESIAN_POINT('Ctrl Pts',(-34.1224056412966,30.8194968072545,176.110625480287));
#35141=CARTESIAN_POINT('Ctrl Pts',(-34.1429649772614,33.1427574547287,175.999495691067));
#35142=CARTESIAN_POINT('Ctrl Pts',(-32.2023060055888,34.4201788723936,175.888365901848));
#35143=CARTESIAN_POINT('Ctrl Pts',(-30.0764987714868,33.4826788317565,175.777236112628));
#35144=CARTESIAN_POINT('Ctrl Pts',(-29.7110590022335,31.1882472032951,175.666106323408));
#35145=CARTESIAN_POINT('Ctrl Pts',(-31.4404332115969,29.6367229312773,175.554976534189));
#35146=CARTESIAN_POINT('Ctrl Pts',(-33.6819168774615,30.2480442038859,175.443846744969));
#35147=CARTESIAN_POINT('Ctrl Pts',(-34.3841284567005,32.4627364219267,175.332716955749));
#35148=CARTESIAN_POINT('Ctrl Pts',(-32.9044115271646,34.2539372847887,175.221587166529));
#35149=CARTESIAN_POINT('Ctrl Pts',(-30.5969869759018,33.9823591875437,175.11045737731));
#35150=CARTESIAN_POINT('Ctrl Pts',(-29.5735847292512,31.8965474596491,174.99932758809));
#35151=CARTESIAN_POINT('Ctrl Pts',(-30.7708114250119,29.9054143747875,174.88819779887));
#35152=CARTESIAN_POINT('Ctrl Pts',(-33.0929781746067,29.8312233392852,174.77706800965));
#35153=CARTESIAN_POINT('Ctrl Pts',(-34.4148631516561,31.7418731842655,174.665938220431));
#35154=CARTESIAN_POINT('Ctrl Pts',(-33.5266915604102,33.8887578917373,174.554808431211));
#35155=CARTESIAN_POINT('Ctrl Pts',(-31.2413084093575,34.3070718594175,174.443678641991));
#35156=CARTESIAN_POINT('Ctrl Pts',(-29.650271574393,32.6139786805113,174.332548852772));
#35157=CARTESIAN_POINT('Ctrl Pts',(-30.2096807128004,30.3589788715227,174.221419063552));
#35158=CARTESIAN_POINT('Ctrl Pts',(-32.4075706476486,29.6058238031834,174.110289274332));
#35159=CARTESIAN_POINT('Ctrl Pts',(-34.2324563456884,31.0437928264109,173.999159485112));
#35160=CARTESIAN_POINT('Ctrl Pts',(-34.0142222061352,33.3568722852722,173.888029695893));
#35161=CARTESIAN_POINT('Ctrl Pts',(-31.9525937468572,34.4281569433195,173.776899906673));
#35162=CARTESIAN_POINT('Ctrl Pts',(-29.9343509763561,33.2772186991064,173.665770117453));
#35163=CARTESIAN_POINT('Ctrl Pts',(-29.8065677912631,30.9573837523311,173.554640328233));
#35164=CARTESIAN_POINT('Ctrl Pts',(-31.6861899768242,29.59173988872,173.443510539014));
#35165=CARTESIAN_POINT('Ctrl Pts',(-33.8530076924679,30.430109562459,173.332380749794));
#35166=CARTESIAN_POINT('Ctrl Pts',(-34.3239728629966,32.7052259398826,173.221250960574));
#35167=CARTESIAN_POINT('Ctrl Pts',(-32.6680632717471,34.3349271849826,173.110121171355));
#35168=CARTESIAN_POINT('Ctrl Pts',(-30.4007494190391,33.8277283916173,172.998991382135));
#35169=CARTESIAN_POINT('Ctrl Pts',(-29.5970523548762,31.6478123951331,172.887861592915));
#35170=CARTESIAN_POINT('Ctrl Pts',(-30.9925069166485,29.7902146753074,172.776731803695));
#35171=CARTESIAN_POINT('Ctrl Pts',(-33.3100082224966,29.9549885205165,172.665602014476));
#35172=CARTESIAN_POINT('Ctrl Pts',(-34.4286042095633,31.9913346945228,172.554472225256));
#35173=CARTESIAN_POINT('Ctrl Pts',(-33.3245679611538,34.0356112621306,172.443342436036));
#35174=CARTESIAN_POINT('Ctrl Pts',(-31.0083014790376,34.2169184779213,172.332212646816));
#35175=CARTESIAN_POINT('Ctrl Pts',(-29.5996267287836,32.3693259441983,172.221082857597));
#35176=CARTESIAN_POINT('Ctrl Pts',(-30.3877475653827,30.183730311518,172.109953068377));
#35177=CARTESIAN_POINT('Ctrl Pts',(-32.6513843459939,29.660365001112,171.998823279157));
#35178=CARTESIAN_POINT('Ctrl Pts',(-34.3188812371206,31.2782082694031,171.887693489938));
#35179=CARTESIAN_POINT('Ctrl Pts',(-33.8641631672544,33.5566275020312,171.776563700718));
#35180=CARTESIAN_POINT('Ctrl Pts',(-31.7033831827247,34.4104381257226,171.665433911498));
#35181=CARTESIAN_POINT('Ctrl Pts',(-29.81406369269,33.0582419168657,171.554304122278));
#35182=CARTESIAN_POINT('Ctrl Pts',(-29.9252894056131,30.7375541818489,171.443174333058));
#35183=CARTESIAN_POINT('Ctrl Pts',(-31.9352677552198,29.5722431689493,171.332044543839));
#35184=CARTESIAN_POINT('Ctrl Pts',(-34.0044883532572,30.6287888799007,171.220914754619));
#35185=CARTESIAN_POINT('Ctrl Pts',(-34.2392229481647,32.9402521378016,171.1097849654));
#35186=CARTESIAN_POINT('Ctrl Pts',(-32.4246449842735,34.3912068357963,170.99865517618));
#35187=CARTESIAN_POINT('Ctrl Pts',(-30.2214365358583,33.6537549692286,170.88752538696));
#35188=CARTESIAN_POINT('Ctrl Pts',(-29.645950082108,31.4028044890487,170.77639559774));
#35189=CARTESIAN_POINT('Ctrl Pts',(-31.224864584604,29.6984008641758,170.665265808521));
#35190=CARTESIAN_POINT('Ctrl Pts',(-33.513174613277,30.1003958086059,170.554136019301));
#35191=CARTESIAN_POINT('Ctrl Pts',(-34.4166436455741,32.2408879086503,170.443006230081));
#35192=CARTESIAN_POINT('Ctrl Pts',(-33.1084266208509,34.1609220070185,170.331876440861));
#35193=CARTESIAN_POINT('Ctrl Pts',(-30.7857895731111,34.1033037187868,170.220746651641));
#35194=CARTESIAN_POINT('Ctrl Pts',(-29.5743847404962,32.1207646765004,170.109616862422));
#35195=CARTESIAN_POINT('Ctrl Pts',(-30.582876688677,30.0277031119193,169.998487073202));
#35196=CARTESIAN_POINT('Ctrl Pts',(-32.8883045233183,29.7396662706405,169.887357283983));
#35197=CARTESIAN_POINT('Ctrl Pts',(-34.38076569148,31.520262346173,169.776227494762));
#35198=CARTESIAN_POINT('Ctrl Pts',(-33.6943759171282,33.7399091199497,169.665097705543));
#35199=CARTESIAN_POINT('Ctrl Pts',(-31.4573116781621,34.3672099356773,169.553967916323));
#35200=CARTESIAN_POINT('Ctrl Pts',(-29.7169099061327,32.8280658895954,169.442838127104));
#35201=CARTESIAN_POINT('Ctrl Pts',(-30.0659674289288,30.5310849213574,169.331708337884));
#35202=CARTESIAN_POINT('Ctrl Pts',(-32.1850305870609,29.5784391033703,169.220578548664));
#35203=CARTESIAN_POINT('Ctrl Pts',(-34.134755758485,30.8419795572488,169.109448759444));
#35204=CARTESIAN_POINT('Ctrl Pts',(-34.130775610212,33.1653277621151,168.998318970225));
#35205=CARTESIAN_POINT('Ctrl Pts',(-32.1767327307596,34.4221806365661,168.887189181005));
#35206=CARTESIAN_POINT('Ctrl Pts',(-30.0609459727286,33.4622800598482,168.776059391785));
#35207=CARTESIAN_POINT('Ctrl Pts',(-29.7197604322381,31.1641166302031,168.664929602565));
#35208=CARTESIAN_POINT('Ctrl Pts',(-31.4654254161029,29.6309445956577,168.553799813346));
#35209=CARTESIAN_POINT('Ctrl Pts',(-33.7003272617103,30.2659063761577,168.442670024126));
#35210=CARTESIAN_POINT('Ctrl Pts',(-34.3791080371299,32.4878918350693,168.331540234906));
#35211=CARTESIAN_POINT('Ctrl Pts',(-32.880554936408,34.2633639788494,168.220410445686));
#35212=CARTESIAN_POINT('Ctrl Pts',(-30.5761275089639,33.9674299515833,168.109280656467));
#35213=CARTESIAN_POINT('Ctrl Pts',(-29.5748127402796,31.870925374144,167.998150867247));
#35214=CARTESIAN_POINT('Ctrl Pts',(-30.7930030593313,29.8925484830768,167.887021078027));
#35215=CARTESIAN_POINT('Ctrl Pts',(-33.1158238734678,29.8428883892604,167.775891288808));
#35216=CARTESIAN_POINT('Ctrl Pts',(-34.4174548111338,31.7673934012069,167.664761499588));
#35217=CARTESIAN_POINT('Ctrl Pts',(-33.5066572568647,33.9047775465331,167.553631710368));
#35218=CARTESIAN_POINT('Ctrl Pts',(-31.2169834524517,34.2989297408903,167.442501921148));
#35219=CARTESIAN_POINT('Ctrl Pts',(-29.6439176314904,32.5891267679911,167.331372131929));
#35220=CARTESIAN_POINT('Ctrl Pts',(-30.2271133920415,30.3401605499161,167.220242342709));
#35221=CARTESIAN_POINT('Ctrl Pts',(-32.4328346333002,29.6102630575578,167.109112553489));
#35222=CARTESIAN_POINT('Ctrl Pts',(-34.2424325857273,31.0674235171078,166.997982764269));
#35223=CARTESIAN_POINT('Ctrl Pts',(-33.9997759247107,33.3780747465314,166.88685297505));
#35224=CARTESIAN_POINT('Ctrl Pts',(-31.9269554489549,34.4275128925295,166.77572318583));
#35225=CARTESIAN_POINT('Ctrl Pts',(-29.9209653652486,33.2553461090702,166.66459339661));
#35226=CARTESIAN_POINT('Ctrl Pts',(-29.8177243014505,30.9342420640658,166.553463607391));
#35227=CARTESIAN_POINT('Ctrl Pts',(-31.7115987485412,29.5886264481624,166.442333818171));
#35228=CARTESIAN_POINT('Ctrl Pts',(-33.8695768412099,30.4496328495725,166.331204028951));
#35229=CARTESIAN_POINT('Ctrl Pts',(-34.3162087590077,32.7300089698471,166.220074239731));
#35230=CARTESIAN_POINT('Ctrl Pts',(-32.6437429291296,34.3412897758451,166.108944450512));
#35231=CARTESIAN_POINT('Ctrl Pts',(-30.3807637468038,33.811890847881,165.997814661292));
#35232=CARTESIAN_POINT('Ctrl Pts',(-29.6025033676946,31.6200556152572,165.886684872072));
#35233=CARTESIAN_POINT('Ctrl Pts',(-30.5427968191108,30.398337297745,165.812598345926));
#35234=CARTESIAN_POINT('Ctrl Pts',(-31.1673980508617,30.1214975228147,165.775555082853));
#35235=CARTESIAN_POINT('Ctrl Pts',(-32.4967348970886,30.1400211999975,179.074814972382));
#35236=CARTESIAN_POINT('Ctrl Pts',(-33.1151770144782,30.3051853306512,179.037771709309));
#35237=CARTESIAN_POINT('Ctrl Pts',(-34.1635488360803,31.2988333782593,178.963685183163));
#35238=CARTESIAN_POINT('Ctrl Pts',(-33.7627875694947,33.4408867622834,178.852555393943));
#35239=CARTESIAN_POINT('Ctrl Pts',(-31.7455260132231,34.2607664131702,178.741425604723));
#35240=CARTESIAN_POINT('Ctrl Pts',(-29.9627191792645,33.0133090020325,178.630295815503));
#35241=CARTESIAN_POINT('Ctrl Pts',(-30.0436426291873,30.8376554419268,178.519166026284));
#35242=CARTESIAN_POINT('Ctrl Pts',(-31.9153798066803,29.7261729311921,178.408036237064));
#35243=CARTESIAN_POINT('Ctrl Pts',(-33.8643754602866,30.6954729396651,178.296906447845));
#35244=CARTESIAN_POINT('Ctrl Pts',(-34.1072057793514,32.858759882056,178.185776658625));
#35245=CARTESIAN_POINT('Ctrl Pts',(-32.4214995896834,34.2360710009532,178.074646869405));
#35246=CARTESIAN_POINT('Ctrl Pts',(-30.3500634676767,33.5669778101029,177.963517080185));
#35247=CARTESIAN_POINT('Ctrl Pts',(-29.7886206003743,31.4637919187861,177.852387290965));
#35248=CARTESIAN_POINT('Ctrl Pts',(-31.25101346648,29.8513435468475,177.741257501746));
#35249=CARTESIAN_POINT('Ctrl Pts',(-33.3988680882353,30.2053194607901,177.630127712526));
#35250=CARTESIAN_POINT('Ctrl Pts',(-34.2664950814802,32.2017689164012,177.518997923306));
#35251=CARTESIAN_POINT('Ctrl Pts',(-33.0598497286692,34.0135609726213,177.407868134087));
#35252=CARTESIAN_POINT('Ctrl Pts',(-30.8832417055349,33.9825641944877,177.296738344867));
#35253=CARTESIAN_POINT('Ctrl Pts',(-29.7286786115939,32.1371460026882,177.185608555647));
#35254=CARTESIAN_POINT('Ctrl Pts',(-30.6528042951125,30.1662133565176,177.074478766427));
#35255=CARTESIAN_POINT('Ctrl Pts',(-32.8098688415486,29.8735423205797,176.963348977208));
#35256=CARTESIAN_POINT('Ctrl Pts',(-34.2257502247723,31.5269823116739,176.852219187988));
#35257=CARTESIAN_POINT('Ctrl Pts',(-33.6046491307433,33.6133229519815,176.741089398768));
#35258=CARTESIAN_POINT('Ctrl Pts',(-31.5149905582741,34.2231679270505,176.629959609549));
#35259=CARTESIAN_POINT('Ctrl Pts',(-29.8692073650418,32.7983937222482,176.518829820329));
#35260=CARTESIAN_POINT('Ctrl Pts',(-30.1735024848817,30.642938242187,176.407700031109));
#35261=CARTESIAN_POINT('Ctrl Pts',(-32.1493883225051,29.7294509656026,176.296570241889));
#35262=CARTESIAN_POINT('Ctrl Pts',(-33.9885555876722,30.8939455424907,176.18544045267));
#35263=CARTESIAN_POINT('Ctrl Pts',(-34.0078183438655,33.0706891640971,176.07431066345));
#35264=CARTESIAN_POINT('Ctrl Pts',(-32.1895475256971,34.2675496739277,175.96318087423));
#35265=CARTESIAN_POINT('Ctrl Pts',(-30.1978048675381,33.3891733126998,175.85205108501));
#35266=CARTESIAN_POINT('Ctrl Pts',(-29.8554116506306,31.2394406006621,175.740921295791));
#35267=CARTESIAN_POINT('Ctrl Pts',(-31.4757224339665,29.7857636029674,175.629791506571));
#35268=CARTESIAN_POINT('Ctrl Pts',(-33.5758463601864,30.358531743447,175.518661717351));
#35269=CARTESIAN_POINT('Ctrl Pts',(-34.2337727869041,32.43355383134,175.407531928131));
#35270=CARTESIAN_POINT('Ctrl Pts',(-32.8473745833052,34.1117921544871,175.296402138912));
#35271=CARTESIAN_POINT('Ctrl Pts',(-30.6854683504597,33.8573411992795,175.185272349692));
#35272=CARTESIAN_POINT('Ctrl Pts',(-29.7266072277715,31.903071720518,175.074142560472));
#35273=CARTESIAN_POINT('Ctrl Pts',(-30.8483305163088,30.037509951995,174.963012771253));
#35274=CARTESIAN_POINT('Ctrl Pts',(-33.0240492269848,29.9679977930878,174.851882982033));
#35275=CARTESIAN_POINT('Ctrl Pts',(-34.2625691904757,31.7581520178003,174.740753192813));
#35276=CARTESIAN_POINT('Ctrl Pts',(-33.4304103673845,33.7696428930898,174.629623403593));
#35277=CARTESIAN_POINT('Ctrl Pts',(-31.2891554882174,34.1615757836016,174.518493614374));
#35278=CARTESIAN_POINT('Ctrl Pts',(-29.7984577974461,32.5752579582744,174.407363825154));
#35279=CARTESIAN_POINT('Ctrl Pts',(-30.3225876557211,30.4624702879473,174.296234035934));
#35280=CARTESIAN_POINT('Ctrl Pts',(-32.3818671007008,29.7568131362754,174.185104246715));
#35281=CARTESIAN_POINT('Ctrl Pts',(-34.0916659162954,31.1040962759357,174.073974457495));
#35282=CARTESIAN_POINT('Ctrl Pts',(-33.8871947684688,33.2713007881883,173.962844668275));
#35283=CARTESIAN_POINT('Ctrl Pts',(-31.9555834343146,34.275024605774,173.851714879055));
#35284=CARTESIAN_POINT('Ctrl Pts',(-30.0646216593981,33.1966705757697,173.740585089835));
#35285=CARTESIAN_POINT('Ctrl Pts',(-29.9448971534963,31.0231366121732,173.629455300616));
#35286=CARTESIAN_POINT('Ctrl Pts',(-31.7059804860523,29.7436174274733,173.518325511396));
#35287=CARTESIAN_POINT('Ctrl Pts',(-33.7361472892644,30.5291151036999,173.407195722177));
#35288=CARTESIAN_POINT('Ctrl Pts',(-34.177410921075,32.6607506859378,173.296065932956));
#35289=CARTESIAN_POINT('Ctrl Pts',(-32.625931690956,34.1876744059483,173.184936143737));
#35290=CARTESIAN_POINT('Ctrl Pts',(-30.5016065652205,33.7124622339759,173.073806354517));
#35291=CARTESIAN_POINT('Ctrl Pts',(-29.7485948615951,31.6700231963484,172.962676565298));
#35292=CARTESIAN_POINT('Ctrl Pts',(-31.0560447251658,29.9295753509734,172.851546776078));
#35293=CARTESIAN_POINT('Ctrl Pts',(-33.2273922194961,30.0839576915672,172.740416986858));
#35294=CARTESIAN_POINT('Ctrl Pts',(-34.2754436650579,31.991881174225,172.629287197638));
#35295=CARTESIAN_POINT('Ctrl Pts',(-33.2410337445178,33.9072349181872,172.518157408419));
#35296=CARTESIAN_POINT('Ctrl Pts',(-31.0708431994455,34.0771079481258,172.407027619199));
#35297=CARTESIAN_POINT('Ctrl Pts',(-29.7510068819548,32.3460343092375,172.295897829979));
#35298=CARTESIAN_POINT('Ctrl Pts',(-30.4894246767843,30.2982738231208,172.184768040759));
#35299=CARTESIAN_POINT('Ctrl Pts',(-32.6103046259136,29.8079146796321,172.07363825154));
#35300=CARTESIAN_POINT('Ctrl Pts',(-34.1726403998848,31.3237282491686,171.96250846232));
#35301=CARTESIAN_POINT('Ctrl Pts',(-33.7465992411855,33.4584583912043,171.8513786731));
#35302=CARTESIAN_POINT('Ctrl Pts',(-31.7220893980333,34.2584232299324,171.74024888388));
#35303=CARTESIAN_POINT('Ctrl Pts',(-29.951920323986,32.9915036202065,171.629119094661));
#35304=CARTESIAN_POINT('Ctrl Pts',(-30.0561315589275,30.8171706496765,171.517989305441));
#35305=CARTESIAN_POINT('Ctrl Pts',(-31.9393501107632,29.7253502733125,171.406859516221));
#35306=CARTESIAN_POINT('Ctrl Pts',(-33.8780747835076,30.7152646592637,171.295729727002));
#35307=CARTESIAN_POINT('Ctrl Pts',(-34.0980057812589,32.8809548966822,171.184599937782));
#35308=CARTESIAN_POINT('Ctrl Pts',(-32.3978646399272,34.2404047662152,171.073470148562));
#35309=CARTESIAN_POINT('Ctrl Pts',(-30.3336020947966,33.549460489886,170.962340359342));
#35310=CARTESIAN_POINT('Ctrl Pts',(-29.7944088411753,31.4404667764125,170.851210570123));
#35311=CARTESIAN_POINT('Ctrl Pts',(-31.2737486974702,29.8435518012811,170.740080780903));
#35312=CARTESIAN_POINT('Ctrl Pts',(-33.417745869973,30.2201948319103,170.628950991683));
#35313=CARTESIAN_POINT('Ctrl Pts',(-34.2642373970902,32.2256962511919,170.517821202463));
#35314=CARTESIAN_POINT('Ctrl Pts',(-33.0385234130226,34.0246429089565,170.406691413244));
#35315=CARTESIAN_POINT('Ctrl Pts',(-30.8623640636741,33.9706583327822,170.295561624024));
#35316=CARTESIAN_POINT('Ctrl Pts',(-29.7273567861031,32.1131486213453,170.184431834805));
#35317=CARTESIAN_POINT('Ctrl Pts',(-30.6722479321011,30.1520865186989,170.073302045584));
#35318=CARTESIAN_POINT('Ctrl Pts',(-32.8322833717686,29.882214794352,169.962172256365));
#35319=CARTESIAN_POINT('Ctrl Pts',(-34.2306220953308,31.55051712379,169.851042467145));
#35320=CARTESIAN_POINT('Ctrl Pts',(-33.5875196673356,33.6301813070964,169.739912677925));
#35321=CARTESIAN_POINT('Ctrl Pts',(-31.4915364557286,34.2179212367286,169.628782888706));
#35322=CARTESIAN_POINT('Ctrl Pts',(-29.8608935657816,32.7758437028605,169.517653099486));
#35323=CARTESIAN_POINT('Ctrl Pts',(-30.1879376867873,30.6237224258101,169.406523310266));
#35324=CARTESIAN_POINT('Ctrl Pts',(-32.1733615858492,29.7311554595474,169.295393521047));
#35325=CARTESIAN_POINT('Ctrl Pts',(-34.0001268415671,30.9150104121167,169.184263731827));
#35326=CARTESIAN_POINT('Ctrl Pts',(-33.9963977023611,33.0918360692859,169.073133942607));
#35327=CARTESIAN_POINT('Ctrl Pts',(-32.1655870359738,34.2694251963316,168.962004153387));
#35328=CARTESIAN_POINT('Ctrl Pts',(-30.1832329100044,33.3700609945497,168.850874364168));
#35329=CARTESIAN_POINT('Ctrl Pts',(-29.8635643227304,31.2168318283228,168.739744574948));
#35330=CARTESIAN_POINT('Ctrl Pts',(-31.4991384987148,29.7803496795589,168.628614785728));
#35331=CARTESIAN_POINT('Ctrl Pts',(-33.5930956888523,30.3752674332642,168.517484996508));
#35332=CARTESIAN_POINT('Ctrl Pts',(-34.2290689813755,32.4571228119305,168.406355207289));
#35333=CARTESIAN_POINT('Ctrl Pts',(-32.8250225145353,34.1206243516802,168.295225418069));
#35334=CARTESIAN_POINT('Ctrl Pts',(-30.6659243911297,33.8433534793964,168.184095628849));
#35335=CARTESIAN_POINT('Ctrl Pts',(-29.7277577939708,31.8790654983767,168.07296583963));
#35336=CARTESIAN_POINT('Ctrl Pts',(-30.8691226295443,30.0254554510298,167.96183605041));
#35337=CARTESIAN_POINT('Ctrl Pts',(-33.0454541560146,29.9789271837081,167.85070626119));
#35338=CARTESIAN_POINT('Ctrl Pts',(-34.2649974062867,31.782062795745,167.73957647197));
#35339=CARTESIAN_POINT('Ctrl Pts',(-33.4116395323068,33.7846522642661,167.628446682751));
#35340=CARTESIAN_POINT('Ctrl Pts',(-31.2663645909291,34.1539471498579,167.517316893531));
#35341=CARTESIAN_POINT('Ctrl Pts',(-29.7925045675747,32.5519733379621,167.406187104311));
#35342=CARTESIAN_POINT('Ctrl Pts',(-30.3389209385952,30.4448387485972,167.295057315091));
#35343=CARTESIAN_POINT('Ctrl Pts',(-32.4055378066472,29.7609724279394,167.183927525872));
#35344=CARTESIAN_POINT('Ctrl Pts',(-34.1010130022092,31.1262366910907,167.072797736652));
#35345=CARTESIAN_POINT('Ctrl Pts',(-33.8736595454705,33.2911661108151,166.961667947432));
#35346=CARTESIAN_POINT('Ctrl Pts',(-31.9315620222151,34.2744211722114,166.850538158213));
#35347=CARTESIAN_POINT('Ctrl Pts',(-30.0520802152725,33.1761773862083,166.739408368993));
#35348=CARTESIAN_POINT('Ctrl Pts',(-29.9553500755206,31.0014543603864,166.628278579773));
#35349=CARTESIAN_POINT('Ctrl Pts',(-31.729786847094,29.7407003368394,166.517148790553));
#35350=CARTESIAN_POINT('Ctrl Pts',(-33.7516715004109,30.5474071497272,166.406019001334));
#35351=CARTESIAN_POINT('Ctrl Pts',(-34.1701364622864,32.6839707677904,166.294889212114));
#35352=CARTESIAN_POINT('Ctrl Pts',(-32.6031451169547,34.1936357383937,166.183759422894));
#35353=CARTESIAN_POINT('Ctrl Pts',(-30.4828812945072,33.6976234889787,166.072629633674));
#35354=CARTESIAN_POINT('Ctrl Pts',(-29.7537021048984,31.6440169048818,165.961499844455));
#35355=CARTESIAN_POINT('Ctrl Pts',(-30.6346957097416,30.4993465649716,165.887413318308));
#35356=CARTESIAN_POINT('Ctrl Pts',(-31.2199063053497,30.2399657611253,165.850370055235));
#35357=CARTESIAN_POINT('Ctrl Pts',(-32.4632995769876,30.2652167256664,179.149629944765));
#35358=CARTESIAN_POINT('Ctrl Pts',(-33.0401142382028,30.4192636273717,179.112586681692));
#35359=CARTESIAN_POINT('Ctrl Pts',(-34.0179199537279,31.3460290365056,179.038500155545));
#35360=CARTESIAN_POINT('Ctrl Pts',(-33.6441340039781,33.3439004011306,178.927370366325));
#35361=CARTESIAN_POINT('Ctrl Pts',(-31.7626547055198,34.108593797272,178.816240577106));
#35362=CARTESIAN_POINT('Ctrl Pts',(-30.0998489375644,32.9451029809884,178.705110787886));
#35363=CARTESIAN_POINT('Ctrl Pts',(-30.1753254147303,30.9158930745042,178.593980998666));
#35364=CARTESIAN_POINT('Ctrl Pts',(-31.9210756079361,29.8792246622974,178.482851209446));
#35365=CARTESIAN_POINT('Ctrl Pts',(-33.7388839945804,30.7832809034267,178.371721420227));
#35366=CARTESIAN_POINT('Ctrl Pts',(-33.9653693588297,32.8009565915792,178.260591631007));
#35367=CARTESIAN_POINT('Ctrl Pts',(-32.393128372388,34.0855606379334,178.149461841787));
#35368=CARTESIAN_POINT('Ctrl Pts',(-30.4611210084854,33.4615042366153,178.038332052568));
#35369=CARTESIAN_POINT('Ctrl Pts',(-29.9374689670273,31.4998841863944,177.927202263348));
#35370=CARTESIAN_POINT('Ctrl Pts',(-31.3014278920546,29.9959700200815,177.816072474128));
#35371=CARTESIAN_POINT('Ctrl Pts',(-33.3047100119993,30.3261197481449,177.704942684909));
#35372=CARTESIAN_POINT('Ctrl Pts',(-34.1139368678319,32.188187812384,177.593812895689));
#35373=CARTESIAN_POINT('Ctrl Pts',(-32.9885110424914,33.8780278017951,177.482683106469));
#35374=CARTESIAN_POINT('Ctrl Pts',(-30.958410918066,33.8491174226745,177.371553317249));
#35375=CARTESIAN_POINT('Ctrl Pts',(-29.8815616848764,32.1279146792452,177.26042352803));
#35376=CARTESIAN_POINT('Ctrl Pts',(-30.7434842934286,30.2896458831653,177.14929373881));
#35377=CARTESIAN_POINT('Ctrl Pts',(-32.7553564162777,30.016674590145,177.03816394959));
#35378=CARTESIAN_POINT('Ctrl Pts',(-34.075934555154,31.5588212219564,176.927034160371));
#35379=CARTESIAN_POINT('Ctrl Pts',(-33.4966398935211,33.5047298782074,176.815904371151));
#35380=CARTESIAN_POINT('Ctrl Pts',(-31.5476366357516,34.0735260723815,176.704774581931));
#35381=CARTESIAN_POINT('Ctrl Pts',(-30.0126314212863,32.7446536894331,176.593644792711));
#35382=CARTESIAN_POINT('Ctrl Pts',(-30.2964443789173,30.7342823263961,176.482515003492));
#35383=CARTESIAN_POINT('Ctrl Pts',(-32.1393329661942,29.8822820515903,176.371385214272));
#35384=CARTESIAN_POINT('Ctrl Pts',(-33.8547055340479,30.9683942777269,176.260255425052));
#35385=CARTESIAN_POINT('Ctrl Pts',(-33.8726717104697,32.9986208734656,176.149125635832));
#35386=CARTESIAN_POINT('Ctrl Pts',(-32.1767890458053,34.1149204754619,176.037995846613));
#35387=CARTESIAN_POINT('Ctrl Pts',(-30.3191109635895,33.2956677936431,175.926866057393));
#35388=CARTESIAN_POINT('Ctrl Pts',(-29.9997642990276,31.290633998029,175.815736268173));
#35389=CARTESIAN_POINT('Ctrl Pts',(-31.5110116563361,29.9348042746576,175.704606478953));
#35390=CARTESIAN_POINT('Ctrl Pts',(-33.4697758429112,30.4690192830081,175.593476689734));
#35391=CARTESIAN_POINT('Ctrl Pts',(-34.0834171171077,32.4043712407533,175.482346900514));
#35392=CARTESIAN_POINT('Ctrl Pts',(-32.7903376394458,33.9696470241855,175.371217111294));
#35393=CARTESIAN_POINT('Ctrl Pts',(-30.7739497250175,33.7323232110152,175.260087322075));
#35394=CARTESIAN_POINT('Ctrl Pts',(-29.8796297262918,31.909595981387,175.148957532855));
#35395=CARTESIAN_POINT('Ctrl Pts',(-30.9258496076056,30.1696055292025,175.037827743635));
#35396=CARTESIAN_POINT('Ctrl Pts',(-32.9551202793629,30.1047722468905,174.926697954415));
#35397=CARTESIAN_POINT('Ctrl Pts',(-34.1102752292953,31.7744308513351,174.815568165196));
#35398=CARTESIAN_POINT('Ctrl Pts',(-33.3341291743586,33.6505278944423,174.704438375976));
#35399=CARTESIAN_POINT('Ctrl Pts',(-31.3370025670773,34.0160797077856,174.593308586756));
#35400=CARTESIAN_POINT('Ctrl Pts',(-29.9466440204991,32.5365372360375,174.482178797537));
#35401=CARTESIAN_POINT('Ctrl Pts',(-30.4354945986418,30.5659617043719,174.371049008317));
#35402=CARTESIAN_POINT('Ctrl Pts',(-32.3561635537529,29.9078024693675,174.259919219097));
#35403=CARTESIAN_POINT('Ctrl Pts',(-33.9508754869023,31.1643997254604,174.148789429877));
#35404=CARTESIAN_POINT('Ctrl Pts',(-33.7601673308024,33.1857292911044,174.037659640658));
#35405=CARTESIAN_POINT('Ctrl Pts',(-31.9585731217721,34.1218922682283,173.926529851438));
#35406=CARTESIAN_POINT('Ctrl Pts',(-30.19489234244,33.1161224524332,173.815400062218));
#35407=CARTESIAN_POINT('Ctrl Pts',(-30.0832265157296,31.0888894720152,173.704270272998));
#35408=CARTESIAN_POINT('Ctrl Pts',(-31.7257709952805,29.8954949662266,173.593140483779));
#35409=CARTESIAN_POINT('Ctrl Pts',(-33.619286886061,30.6281206449407,173.482010694559));
#35410=CARTESIAN_POINT('Ctrl Pts',(-34.0308489791535,32.6162754319929,173.370880905339));
#35411=CARTESIAN_POINT('Ctrl Pts',(-32.5838001101648,34.040421626914,173.25975111612));
#35412=CARTESIAN_POINT('Ctrl Pts',(-30.6024637114019,33.5971960763345,173.1486213269));
#35413=CARTESIAN_POINT('Ctrl Pts',(-29.900137368314,31.6922339975638,173.03749153768));
#35414=CARTESIAN_POINT('Ctrl Pts',(-31.1195825336831,30.0689360266394,172.92636174846));
#35415=CARTESIAN_POINT('Ctrl Pts',(-33.1447762164956,30.2129268626179,172.815231959241));
#35416=CARTESIAN_POINT('Ctrl Pts',(-34.1222831205525,31.9924276539272,172.704102170021));
#35417=CARTESIAN_POINT('Ctrl Pts',(-33.1574995278817,33.7788585742437,172.592972380801));
#35418=CARTESIAN_POINT('Ctrl Pts',(-31.1333849198533,33.9372974183303,172.481842591581));
#35419=CARTESIAN_POINT('Ctrl Pts',(-29.902387035126,32.3227426742766,172.370712802361));
#35420=CARTESIAN_POINT('Ctrl Pts',(-30.5911017881859,30.4128173347236,172.259583013142));
#35421=CARTESIAN_POINT('Ctrl Pts',(-32.5692249058332,29.9554643581522,172.148453223922));
#35422=CARTESIAN_POINT('Ctrl Pts',(-34.026399562649,31.3692482289342,172.037323434703));
#35423=CARTESIAN_POINT('Ctrl Pts',(-33.6290353151166,33.3602892803774,171.926193645483));
#35424=CARTESIAN_POINT('Ctrl Pts',(-31.7407956133418,34.1064083341423,171.815063856263));
#35425=CARTESIAN_POINT('Ctrl Pts',(-30.0897769552821,32.9247653235473,171.703934067043));
#35426=CARTESIAN_POINT('Ctrl Pts',(-30.1869737122419,30.8967871175041,171.592804277824));
#35427=CARTESIAN_POINT('Ctrl Pts',(-31.9434324663065,29.8784573776757,171.481674488604));
#35428=CARTESIAN_POINT('Ctrl Pts',(-33.7516612137581,30.8017404386267,171.370544699384));
#35429=CARTESIAN_POINT('Ctrl Pts',(-33.9567886143531,32.8216576555628,171.259414910164));
#35430=CARTESIAN_POINT('Ctrl Pts',(-32.371084295581,34.089602696634,171.148285120945));
#35431=CARTESIAN_POINT('Ctrl Pts',(-30.4457676537348,33.4451660105434,171.037155331725));
#35432=CARTESIAN_POINT('Ctrl Pts',(-29.9428676002425,31.4781290637763,170.926025542505));
#35433=CARTESIAN_POINT('Ctrl Pts',(-31.3226328103364,29.9887027383865,170.814895753285));
#35434=CARTESIAN_POINT('Ctrl Pts',(-33.322317126669,30.3399938552148,170.703765964066));
#35435=CARTESIAN_POINT('Ctrl Pts',(-34.1118311486063,32.2105045937335,170.592636174846));
#35436=CARTESIAN_POINT('Ctrl Pts',(-32.9686202051942,33.8883638108946,170.481506385626));
#35437=CARTESIAN_POINT('Ctrl Pts',(-30.9389385542372,33.8380129467777,170.370376596406));
#35438=CARTESIAN_POINT('Ctrl Pts',(-29.8803288317099,32.1055325661903,170.259246807187));
#35439=CARTESIAN_POINT('Ctrl Pts',(-30.7616191755252,30.2764699254786,170.148117017967));
#35440=CARTESIAN_POINT('Ctrl Pts',(-32.776262220219,30.0247633180635,170.036987228747));
#35441=CARTESIAN_POINT('Ctrl Pts',(-34.0804784991816,31.5807719014069,169.925857439528));
#35442=CARTESIAN_POINT('Ctrl Pts',(-33.4806634175431,33.5204534942432,169.814727650308));
#35443=CARTESIAN_POINT('Ctrl Pts',(-31.5257612332951,34.0686325377799,169.703597861088));
#35444=CARTESIAN_POINT('Ctrl Pts',(-30.0048772254305,32.7236215161257,169.592468071868));
#35445=CARTESIAN_POINT('Ctrl Pts',(-30.3099079446457,30.7163599302627,169.481338282649));
#35446=CARTESIAN_POINT('Ctrl Pts',(-32.1616925846373,29.8838718157245,169.370208493429));
#35447=CARTESIAN_POINT('Ctrl Pts',(-33.8654979246492,30.9880412669846,169.259078704209));
#35448=CARTESIAN_POINT('Ctrl Pts',(-33.8620197945103,33.0183443764568,169.14794891499));
#35449=CARTESIAN_POINT('Ctrl Pts',(-32.1544413411881,34.1166697560972,169.03681912577));
#35450=CARTESIAN_POINT('Ctrl Pts',(-30.3055198472801,33.2778419292513,168.92568933655));
#35451=CARTESIAN_POINT('Ctrl Pts',(-30.0073682132228,31.2695470264423,168.81455954733));
#35452=CARTESIAN_POINT('Ctrl Pts',(-31.5328515813266,29.9297547634601,168.703429758111));
#35453=CARTESIAN_POINT('Ctrl Pts',(-33.4858641159943,30.4846284903707,168.592299968891));
#35454=CARTESIAN_POINT('Ctrl Pts',(-34.0790299256211,32.4263537887917,168.481170179671));
#35455=CARTESIAN_POINT('Ctrl Pts',(-32.7694900926627,33.977884724511,168.370040390452));
#35456=CARTESIAN_POINT('Ctrl Pts',(-30.7557212732955,33.7192770072096,168.258910601232));
#35457=CARTESIAN_POINT('Ctrl Pts',(-29.880702847662,31.8872056226094,168.147780812012));
#35458=CARTESIAN_POINT('Ctrl Pts',(-30.9452421997572,30.1583624189827,168.036651022792));
#35459=CARTESIAN_POINT('Ctrl Pts',(-32.9750844385614,30.114965978156,167.925521233572));
#35460=CARTESIAN_POINT('Ctrl Pts',(-34.1125400014398,31.796732190283,167.814391444353));
#35461=CARTESIAN_POINT('Ctrl Pts',(-33.3166218077489,33.664526981999,167.703261655133));
#35462=CARTESIAN_POINT('Ctrl Pts',(-31.3157457294065,34.0089645588256,167.592131865914));
#35463=CARTESIAN_POINT('Ctrl Pts',(-29.9410915036591,32.514819907933,167.481002076694));
#35464=CARTESIAN_POINT('Ctrl Pts',(-30.4507284851489,30.5495169472784,167.369872287474));
#35465=CARTESIAN_POINT('Ctrl Pts',(-32.3782409799943,29.9116817983209,167.258742498254));
#35466=CARTESIAN_POINT('Ctrl Pts',(-33.9595934186911,31.1850498650737,167.147612709035));
#35467=CARTESIAN_POINT('Ctrl Pts',(-33.7475431662303,33.2042574750988,167.036482919815));
#35468=CARTESIAN_POINT('Ctrl Pts',(-31.9361685954752,34.1213294518934,166.925353130595));
#35469=CARTESIAN_POINT('Ctrl Pts',(-30.1831950652964,33.0970086633465,166.814223341375));
#35470=CARTESIAN_POINT('Ctrl Pts',(-30.0929758495906,31.0686666567071,166.703093552155));
#35471=CARTESIAN_POINT('Ctrl Pts',(-31.7479749456469,29.8927742255163,166.591963762936));
#35472=CARTESIAN_POINT('Ctrl Pts',(-33.6337661596119,30.6451814498819,166.480833973716));
#35473=CARTESIAN_POINT('Ctrl Pts',(-34.0240641655651,32.6379325657337,166.369704184496));
#35474=CARTESIAN_POINT('Ctrl Pts',(-32.5625473047798,34.0459817009423,166.258574395277));
#35475=CARTESIAN_POINT('Ctrl Pts',(-30.5849988422104,33.5833561300764,166.147444606057));
#35476=CARTESIAN_POINT('Ctrl Pts',(-29.9049008421022,31.6679781945065,166.036314816837));
#35477=CARTESIAN_POINT('Ctrl Pts',(-30.7265946003723,30.6003558321983,165.962228290691));
#35478=CARTESIAN_POINT('Ctrl Pts',(-31.2724145598377,30.3584339994358,165.925185027618));
#35479=CARTESIAN_POINT('Ctrl Pts',(-32.4298642568866,30.3904122513353,179.224444917147));
#35480=CARTESIAN_POINT('Ctrl Pts',(-32.9650514619275,30.5333419240922,179.187401654074));
#35481=CARTESIAN_POINT('Ctrl Pts',(-33.8722910713755,31.393224694752,179.113315127928));
#35482=CARTESIAN_POINT('Ctrl Pts',(-33.5254804384615,33.2469140399779,179.002185338708));
#35483=CARTESIAN_POINT('Ctrl Pts',(-31.7797833978164,33.9564211813738,178.891055549489));
#35484=CARTESIAN_POINT('Ctrl Pts',(-30.2369786958643,32.8768969599443,178.779925760268));
#35485=CARTESIAN_POINT('Ctrl Pts',(-30.3070082002733,30.9941307070816,178.668795971049));
#35486=CARTESIAN_POINT('Ctrl Pts',(-31.9267714091919,30.0322763934028,178.557666181829));
#35487=CARTESIAN_POINT('Ctrl Pts',(-33.6133925288741,30.8710888671883,178.44653639261));
#35488=CARTESIAN_POINT('Ctrl Pts',(-33.8235329383081,32.7431533011022,178.335406603389));
#35489=CARTESIAN_POINT('Ctrl Pts',(-32.3647571550926,33.9350502749137,178.22427681417));
#35490=CARTESIAN_POINT('Ctrl Pts',(-30.5721785492941,33.3560306631277,178.11314702495));
#35491=CARTESIAN_POINT('Ctrl Pts',(-30.0863173336803,31.5359764540028,178.002017235731));
#35492=CARTESIAN_POINT('Ctrl Pts',(-31.3518423176291,30.1405964933155,177.890887446511));
#35493=CARTESIAN_POINT('Ctrl Pts',(-33.2105519357631,30.4469200354998,177.779757657291));
#35494=CARTESIAN_POINT('Ctrl Pts',(-33.9613786541837,32.1746067083669,177.668627868071));
#35495=CARTESIAN_POINT('Ctrl Pts',(-32.9171723563135,33.742494630969,177.557498078851));
#35496=CARTESIAN_POINT('Ctrl Pts',(-31.0335801305971,33.7156706508613,177.446368289632));
#35497=CARTESIAN_POINT('Ctrl Pts',(-30.0344447581588,32.1186833558022,177.335238500412));
#35498=CARTESIAN_POINT('Ctrl Pts',(-30.8341642917448,30.4130784098129,177.224108711193));
#35499=CARTESIAN_POINT('Ctrl Pts',(-32.7008439910068,30.1598068597104,177.112978921972));
#35500=CARTESIAN_POINT('Ctrl Pts',(-33.9261188855358,31.590660132239,177.001849132753));
#35501=CARTESIAN_POINT('Ctrl Pts',(-33.388630656299,33.3961368044331,176.890719343533));
#35502=CARTESIAN_POINT('Ctrl Pts',(-31.580282713229,33.9238842177125,176.779589554314));
#35503=CARTESIAN_POINT('Ctrl Pts',(-30.1560554775308,32.6909136566179,176.668459765094));
#35504=CARTESIAN_POINT('Ctrl Pts',(-30.4193862729528,30.8256264106052,176.557329975874));
#35505=CARTESIAN_POINT('Ctrl Pts',(-32.1292776098832,30.035113137578,176.446200186654));
#35506=CARTESIAN_POINT('Ctrl Pts',(-33.7208554804235,31.0428430129631,176.335070397435));
#35507=CARTESIAN_POINT('Ctrl Pts',(-33.7375250770738,32.9265525828339,176.223940608215));
#35508=CARTESIAN_POINT('Ctrl Pts',(-32.1640305659136,33.962291276996,176.112810818995));
#35509=CARTESIAN_POINT('Ctrl Pts',(-30.4404170596408,33.2021622745864,176.001681029775));
#35510=CARTESIAN_POINT('Ctrl Pts',(-30.1441169474248,31.3418273953959,175.890551240556));
#35511=CARTESIAN_POINT('Ctrl Pts',(-31.5463008787057,30.0838449463477,175.779421451336));
#35512=CARTESIAN_POINT('Ctrl Pts',(-33.3637053256361,30.5795068225691,175.668291662116));
#35513=CARTESIAN_POINT('Ctrl Pts',(-33.9330614473113,32.3751886501666,175.557161872897));
#35514=CARTESIAN_POINT('Ctrl Pts',(-32.7333006955864,33.8275018938839,175.446032083677));
#35515=CARTESIAN_POINT('Ctrl Pts',(-30.8624310995753,33.607305222751,175.334902294457));
#35516=CARTESIAN_POINT('Ctrl Pts',(-30.0326522248121,31.9161202422559,175.223772505237));
#35517=CARTESIAN_POINT('Ctrl Pts',(-31.0033686989025,30.30170110641,175.112642716018));
#35518=CARTESIAN_POINT('Ctrl Pts',(-32.886191331741,30.2415467006931,175.001512926798));
#35519=CARTESIAN_POINT('Ctrl Pts',(-33.9579812681149,31.7907096848698,174.890383137578));
#35520=CARTESIAN_POINT('Ctrl Pts',(-33.2378479813328,33.5314128957948,174.779253348358));
#35521=CARTESIAN_POINT('Ctrl Pts',(-31.3848496459372,33.8705836319696,174.668123559139));
#35522=CARTESIAN_POINT('Ctrl Pts',(-30.0948302435522,32.4978165138007,174.556993769919));
#35523=CARTESIAN_POINT('Ctrl Pts',(-30.5484015415624,30.6694531207966,174.445863980699));
#35524=CARTESIAN_POINT('Ctrl Pts',(-32.3304600068051,30.0587918024595,174.334734191479));
#35525=CARTESIAN_POINT('Ctrl Pts',(-33.8100850575091,31.2247031749851,174.22360440226));
#35526=CARTESIAN_POINT('Ctrl Pts',(-33.633139893136,33.1001577940204,174.11247461304));
#35527=CARTESIAN_POINT('Ctrl Pts',(-31.9615628092294,33.9687599306827,174.00134482382));
#35528=CARTESIAN_POINT('Ctrl Pts',(-30.3251630254821,33.0355743290966,173.8902150346));
#35529=CARTESIAN_POINT('Ctrl Pts',(-30.2215558779629,31.1546423318572,173.779085245381));
#35530=CARTESIAN_POINT('Ctrl Pts',(-31.7455615045087,30.0473725049799,173.667955456161));
#35531=CARTESIAN_POINT('Ctrl Pts',(-33.5024264828575,30.7271261861816,173.556825666941));
#35532=CARTESIAN_POINT('Ctrl Pts',(-33.8842870372319,32.5718001780481,173.445695877722));
#35533=CARTESIAN_POINT('Ctrl Pts',(-32.5416685293737,33.8931688478798,173.334566088502));
#35534=CARTESIAN_POINT('Ctrl Pts',(-30.7033208575832,33.481929918693,173.223436299282));
#35535=CARTESIAN_POINT('Ctrl Pts',(-30.0516798750329,31.7144447987793,173.112306510063));
#35536=CARTESIAN_POINT('Ctrl Pts',(-31.1831203422005,30.2082967023054,173.001176720843));
#35537=CARTESIAN_POINT('Ctrl Pts',(-33.0621602134952,30.3418960336686,172.890046931623));
#35538=CARTESIAN_POINT('Ctrl Pts',(-33.969122576047,31.9929741336294,172.778917142403));
#35539=CARTESIAN_POINT('Ctrl Pts',(-33.0739653112457,33.6504822303003,172.667787353184));
#35540=CARTESIAN_POINT('Ctrl Pts',(-31.1959266402612,33.7974868885348,172.556657563964));
#35541=CARTESIAN_POINT('Ctrl Pts',(-30.0537671882971,32.2994510393159,172.445527774744));
#35542=CARTESIAN_POINT('Ctrl Pts',(-30.6927788995876,30.5273608463263,172.334397985524));
#35543=CARTESIAN_POINT('Ctrl Pts',(-32.5281451857529,30.1030140366724,172.223268196305));
#35544=CARTESIAN_POINT('Ctrl Pts',(-33.8801587254133,31.4147682086997,172.112138407085));
#35545=CARTESIAN_POINT('Ctrl Pts',(-33.5114713890477,33.2621201695506,172.001008617865));
#35546=CARTESIAN_POINT('Ctrl Pts',(-31.7595018286504,33.9543934383521,171.889878828646));
#35547=CARTESIAN_POINT('Ctrl Pts',(-30.2276335865782,32.8580270268881,171.778749039426));
#35548=CARTESIAN_POINT('Ctrl Pts',(-30.3178158655562,30.9764035853317,171.667619250206));
#35549=CARTESIAN_POINT('Ctrl Pts',(-31.9475148218499,30.0315644820389,171.556489460986));
#35550=CARTESIAN_POINT('Ctrl Pts',(-33.6252476440085,30.8882162179898,171.445359671767));
#35551=CARTESIAN_POINT('Ctrl Pts',(-33.8155714474473,32.7623604144434,171.334229882547));
#35552=CARTESIAN_POINT('Ctrl Pts',(-32.3443039512348,33.9388006270528,171.223100093327));
#35553=CARTESIAN_POINT('Ctrl Pts',(-30.5579332126731,33.3408715312008,171.111970304107));
#35554=CARTESIAN_POINT('Ctrl Pts',(-30.0913263593098,31.51579135114,171.000840514888));
#35555=CARTESIAN_POINT('Ctrl Pts',(-31.3715169232025,30.1338536754918,170.889710725668));
#35556=CARTESIAN_POINT('Ctrl Pts',(-33.2268883833651,30.4597928785192,170.778580936448));
#35557=CARTESIAN_POINT('Ctrl Pts',(-33.9594249001224,32.1953129362752,170.667451147229));
#35558=CARTESIAN_POINT('Ctrl Pts',(-32.8987169973659,33.7520847128326,170.556321358009));
#35559=CARTESIAN_POINT('Ctrl Pts',(-31.0155130448001,33.7053675607732,170.445191568789));
#35560=CARTESIAN_POINT('Ctrl Pts',(-30.0333008773168,32.0979165110352,170.334061779569));
#35561=CARTESIAN_POINT('Ctrl Pts',(-30.8509904189492,30.4008533322582,170.22293199035));
#35562=CARTESIAN_POINT('Ctrl Pts',(-32.7202410686693,30.167311841775,170.11180220113));
#35563=CARTESIAN_POINT('Ctrl Pts',(-33.9303349030323,31.6110266790238,170.00067241191));
#35564=CARTESIAN_POINT('Ctrl Pts',(-33.3738071677506,33.41072568139,169.88954262269));
#35565=CARTESIAN_POINT('Ctrl Pts',(-31.5599860108617,33.9193438388312,169.778412833471));
#35566=CARTESIAN_POINT('Ctrl Pts',(-30.1488608850795,32.6713993293909,169.667283044251));
#35567=CARTESIAN_POINT('Ctrl Pts',(-30.4318782025041,30.8089974347154,169.556153255031));
#35568=CARTESIAN_POINT('Ctrl Pts',(-32.1500235834255,30.0365881719016,169.445023465812));
#35569=CARTESIAN_POINT('Ctrl Pts',(-33.7308690077313,31.0610721218525,169.333893676592));
#35570=CARTESIAN_POINT('Ctrl Pts',(-33.7276418866593,32.9448526836276,169.222763887372));
#35571=CARTESIAN_POINT('Ctrl Pts',(-32.1432956464024,33.9639143158628,169.111634098152));
#35572=CARTESIAN_POINT('Ctrl Pts',(-30.4278067845557,33.1856228639528,169.000504308933));
#35573=CARTESIAN_POINT('Ctrl Pts',(-30.1511721037151,31.3222622245619,168.889374519713));
#35574=CARTESIAN_POINT('Ctrl Pts',(-31.5665646639384,30.0791598473613,168.778244730493));
#35575=CARTESIAN_POINT('Ctrl Pts',(-33.3786325431363,30.5939895474772,168.667114941273));
#35576=CARTESIAN_POINT('Ctrl Pts',(-33.9289908698666,32.3955847656529,168.555985152054));
#35577=CARTESIAN_POINT('Ctrl Pts',(-32.71395767079,33.8351450973418,168.444855362834));
#35578=CARTESIAN_POINT('Ctrl Pts',(-30.8455181554612,33.5952005350227,168.333725573614));
#35579=CARTESIAN_POINT('Ctrl Pts',(-30.0336479013533,31.8953457468421,168.222595784395));
#35580=CARTESIAN_POINT('Ctrl Pts',(-31.0213617699701,30.2912693869356,168.111465995175));
#35581=CARTESIAN_POINT('Ctrl Pts',(-32.9047147211083,30.2510047726038,168.000336205955));
#35582=CARTESIAN_POINT('Ctrl Pts',(-33.9600825965927,31.8114015848209,167.889206416735));
#35583=CARTESIAN_POINT('Ctrl Pts',(-33.221604083191,33.5444016997319,167.778076627516));
#35584=CARTESIAN_POINT('Ctrl Pts',(-31.3651268678839,33.8639819677932,167.666946838296));
#35585=CARTESIAN_POINT('Ctrl Pts',(-30.0896784397435,32.477666477904,167.555817049076));
#35586=CARTESIAN_POINT('Ctrl Pts',(-30.5625360317027,30.6541951459594,167.444687259856));
#35587=CARTESIAN_POINT('Ctrl Pts',(-32.3509441533413,30.0623911687024,167.333557470637));
#35588=CARTESIAN_POINT('Ctrl Pts',(-33.8181738351729,31.2438630390566,167.222427681417));
#35589=CARTESIAN_POINT('Ctrl Pts',(-33.6214267869902,33.1173488393825,167.111297892197));
#35590=CARTESIAN_POINT('Ctrl Pts',(-31.9407751687353,33.9682377315752,167.000168102977));
#35591=CARTESIAN_POINT('Ctrl Pts',(-30.3143099153202,33.0178399404847,166.889038313758));
#35592=CARTESIAN_POINT('Ctrl Pts',(-30.2306016236606,31.1358789530277,166.777908524538));
#35593=CARTESIAN_POINT('Ctrl Pts',(-31.7661630441998,30.0448481141933,166.666778735318));
#35594=CARTESIAN_POINT('Ctrl Pts',(-33.5158608188129,30.7429557500367,166.555648946099));
#35595=CARTESIAN_POINT('Ctrl Pts',(-33.8779918688439,32.591894363677,166.444519156879));
#35596=CARTESIAN_POINT('Ctrl Pts',(-32.5219494926048,33.8983276634909,166.333389367659));
#35597=CARTESIAN_POINT('Ctrl Pts',(-30.6871163899137,33.469088771174,166.222259578439));
#35598=CARTESIAN_POINT('Ctrl Pts',(-30.0560995793061,31.6919394841311,166.11112978922));
#35599=CARTESIAN_POINT('Ctrl Pts',(-30.8184934910031,30.7013650994249,166.037043263073));
#35600=CARTESIAN_POINT('Ctrl Pts',(-31.3249228143257,30.4769022377464,166.));
#35601=CARTESIAN_POINT('Ctrl Pts',(-33.6638666530066,32.0009462971081,178.37851963661));
#35602=CARTESIAN_POINT('Ctrl Pts',(-33.6649865931316,32.2165070141075,178.364148625536));
#35603=CARTESIAN_POINT('Ctrl Pts',(-33.6261153552445,32.4316803559838,178.349777614463));
#35604=CARTESIAN_POINT('Ctrl Pts',(-33.5453802395332,32.6297920577518,178.33540660339));
#35605=CARTESIAN_POINT('Ctrl Pts',(-33.3372743439029,33.1404522923727,178.298363340316));
#35606=CARTESIAN_POINT('Ctrl Pts',(-32.8510157494978,33.5377512836432,178.261320077243));
#35607=CARTESIAN_POINT('Ctrl Pts',(-32.3091233513288,33.6398975106474,178.22427681417));
#35608=CARTESIAN_POINT('Ctrl Pts',(-31.7672309531598,33.7420437376517,178.187233551097));
#35609=CARTESIAN_POINT('Ctrl Pts',(-31.169704751227,33.5490372003897,178.150190288023));
#35610=CARTESIAN_POINT('Ctrl Pts',(-30.7899647809916,33.1491915635712,178.11314702495));
#35611=CARTESIAN_POINT('Ctrl Pts',(-30.4102248107562,32.7493459267527,178.076103761877));
#35612=CARTESIAN_POINT('Ctrl Pts',(-30.2482710722182,32.1426611903778,178.039060498804));
#35613=CARTESIAN_POINT('Ctrl Pts',(-30.3782150336074,31.6067554954091,178.002017235731));
#35614=CARTESIAN_POINT('Ctrl Pts',(-30.5081589949966,31.0708498004404,177.964973972657));
#35615=CARTESIAN_POINT('Ctrl Pts',(-30.9300006563129,30.605723146878,177.927930709584));
#35616=CARTESIAN_POINT('Ctrl Pts',(-31.4507064233267,30.4242137437941,177.890887446511));
#35617=CARTESIAN_POINT('Ctrl Pts',(-31.9714121903405,30.2427043407103,177.853844183437));
#35618=CARTESIAN_POINT('Ctrl Pts',(-32.5909820630518,30.344812188105,177.816800920364));
#35619=CARTESIAN_POINT('Ctrl Pts',(-33.0259047858109,30.6838138906136,177.779757657291));
#35620=CARTESIAN_POINT('Ctrl Pts',(-33.4221146221702,30.9926407282283,177.746011650397));
#35621=CARTESIAN_POINT('Ctrl Pts',(-33.6650855963408,31.498066023098,177.712265643504));
#35622=CARTESIAN_POINT('Ctrl Pts',(-33.6682332709748,32.0008552724336,177.67851963661));
#35623=CARTESIAN_POINT('Ctrl Pts',(-32.5301702171895,30.0148256743285,179.));
#35624=CARTESIAN_POINT('Ctrl Pts',(-32.5988282278053,30.0402471901995,179.));
#35625=CARTESIAN_POINT('Ctrl Pts',(-32.6657829561446,30.0695594583225,179.));
#35626=CARTESIAN_POINT('Ctrl Pts',(-32.7308455855381,30.1024681354669,179.));
#35627=CARTESIAN_POINT('Ctrl Pts',(-32.7977248765802,30.1362956800508,179.));
#35628=CARTESIAN_POINT('Ctrl Pts',(-32.8626057038917,30.1739239621406,179.));
#35629=CARTESIAN_POINT('Ctrl Pts',(-32.9252517745416,30.2150779475002,179.));
#35630=CARTESIAN_POINT('Ctrl Pts',(-32.9781830386928,30.2498500001979,179.));
#35631=CARTESIAN_POINT('Ctrl Pts',(-33.0295185776569,30.2871401009452,179.));
#35632=CARTESIAN_POINT('Ctrl Pts',(-33.0790931240667,30.3268003652989,179.));
#35633=CARTESIAN_POINT('Ctrl Pts',(-33.1011284990253,30.3444289440612,179.));
#35634=CARTESIAN_POINT('Ctrl Pts',(-33.1228156494507,30.3625259776201,179.));
#35635=CARTESIAN_POINT('Ctrl Pts',(-33.1441385070898,30.381079203383,179.));
#35636=CARTESIAN_POINT('Ctrl Pts',(-33.15585001073,30.3912694965762,179.));
#35637=CARTESIAN_POINT('Ctrl Pts',(-33.1674515998752,30.4015974166315,179.));
#35638=CARTESIAN_POINT('Ctrl Pts',(-33.1789404779192,30.4120609733578,179.));
#35639=CARTESIAN_POINT('Ctrl Pts',(-33.1895353442403,30.4217103041569,179.));
#35640=CARTESIAN_POINT('Ctrl Pts',(-33.200035794986,30.4314765021164,179.));
#35641=CARTESIAN_POINT('Ctrl Pts',(-33.2104237431777,30.4413425424031,179.));
#35642=CARTESIAN_POINT('Ctrl Pts',(-33.2635074513343,30.4917592362081,179.));
#35643=CARTESIAN_POINT('Ctrl Pts',(-33.3137511250316,30.5448646877623,179.));
#35644=CARTESIAN_POINT('Ctrl Pts',(-33.3609361600621,30.6003990312448,179.));
#35645=CARTESIAN_POINT('Ctrl Pts',(-33.4077563508377,30.6555039719272,179.));
#35646=CARTESIAN_POINT('Ctrl Pts',(-33.4515655286,30.7130012726339,179.));
#35647=CARTESIAN_POINT('Ctrl Pts',(-33.4921053256574,30.7726612868285,179.));
#35648=CARTESIAN_POINT('Ctrl Pts',(-33.5257899877866,30.8222330056491,179.));
#35649=CARTESIAN_POINT('Ctrl Pts',(-33.5572168227446,30.8732985153182,179.));
#35650=CARTESIAN_POINT('Ctrl Pts',(-33.5862100224613,30.9257325420638,179.));
#35651=CARTESIAN_POINT('Ctrl Pts',(-33.5983167001639,30.9476273956384,179.));
#35652=CARTESIAN_POINT('Ctrl Pts',(-33.6099987169878,30.9697609087471,179.));
#35653=CARTESIAN_POINT('Ctrl Pts',(-33.6212418309088,30.9921240426179,179.));
#35654=CARTESIAN_POINT('Ctrl Pts',(-33.6264400720312,31.0024636125031,179.));
#35655=CARTESIAN_POINT('Ctrl Pts',(-33.6315444780314,31.0128522675599,179.));
#35656=CARTESIAN_POINT('Ctrl Pts',(-33.6365535761887,31.0232891124341,179.));
#35657=CARTESIAN_POINT('Ctrl Pts',(-33.6417882688336,31.0341960009366,179.));
#35658=CARTESIAN_POINT('Ctrl Pts',(-33.6469152729676,31.045148079228,179.));
#35659=CARTESIAN_POINT('Ctrl Pts',(-33.6519315110627,31.0561399991255,179.));
#35660=CARTESIAN_POINT('Ctrl Pts',(-33.6804723862136,31.1186806934698,179.));
#35661=CARTESIAN_POINT('Ctrl Pts',(-33.7054522348945,31.1825535423868,179.));
#35662=CARTESIAN_POINT('Ctrl Pts',(-33.726647631831,31.2475537174627,179.));
#35663=CARTESIAN_POINT('Ctrl Pts',(-33.7458439217222,31.3064232072617,179.));
#35664=CARTESIAN_POINT('Ctrl Pts',(-33.7619356534367,31.3662179954612,179.));
#35665=CARTESIAN_POINT('Ctrl Pts',(-33.7747201888406,31.4267907213557,179.));
#35666=CARTESIAN_POINT('Ctrl Pts',(-33.7898549143372,31.4984985738528,179.));
#35667=CARTESIAN_POINT('Ctrl Pts',(-33.8003553587734,31.5712981878921,179.));
#35668=CARTESIAN_POINT('Ctrl Pts',(-33.8062965723339,31.6447668899705,179.));
#35669=CARTESIAN_POINT('Ctrl Pts',(-33.8076038696773,31.6609328530473,179.));
#35670=CARTESIAN_POINT('Ctrl Pts',(-33.808690198748,31.6771311296592,179.));
#35671=CARTESIAN_POINT('Ctrl Pts',(-33.8095559901045,31.693357052552,179.));
#35672=CARTESIAN_POINT('Ctrl Pts',(-33.8104539226022,31.7101853372883,179.));
#35673=CARTESIAN_POINT('Ctrl Pts',(-33.8111146496093,31.7270495855728,179.));
#35674=CARTESIAN_POINT('Ctrl Pts',(-33.8115380877234,31.7439101956095,179.));
#35675=CARTESIAN_POINT('Ctrl Pts',(-33.8132598142794,31.8124665184444,179.));
#35676=CARTESIAN_POINT('Ctrl Pts',(-33.8110702262932,31.8810491791819,179.));
#35677=CARTESIAN_POINT('Ctrl Pts',(-33.8050898165763,31.9493201958655,179.));
#35678=CARTESIAN_POINT('Ctrl Pts',(-33.7991106222926,32.0175773374357,179.));
#35679=CARTESIAN_POINT('Ctrl Pts',(-33.7893416935654,32.0855240323565,179.));
#35680=CARTESIAN_POINT('Ctrl Pts',(-33.775853846591,32.1528074626958,179.));
#35681=CARTESIAN_POINT('Ctrl Pts',(-33.7660959099765,32.2014844272037,179.));
#35682=CARTESIAN_POINT('Ctrl Pts',(-33.7543904550383,32.2498139755358,179.));
#35683=CARTESIAN_POINT('Ctrl Pts',(-33.7407500992357,32.297652865938,179.));
#35684=CARTESIAN_POINT('Ctrl Pts',(-33.7305146132391,32.3335503381076,179.));
#35685=CARTESIAN_POINT('Ctrl Pts',(-33.7191893856383,32.3691713787597,179.));
#35686=CARTESIAN_POINT('Ctrl Pts',(-33.7067758322136,32.4044512901247,179.));
#35687=CARTESIAN_POINT('Ctrl Pts',(-33.7026466735928,32.4161865560207,179.));
#35688=CARTESIAN_POINT('Ctrl Pts',(-33.6984002925461,32.4278748826704,179.));
#35689=CARTESIAN_POINT('Ctrl Pts',(-33.6940373319631,32.4395137156836,179.));
#35690=CARTESIAN_POINT('Ctrl Pts',(-33.6709143171744,32.5011977265218,179.));
#35691=CARTESIAN_POINT('Ctrl Pts',(-33.6445184296985,32.5614980986713,179.));
#35692=CARTESIAN_POINT('Ctrl Pts',(-33.614899590325,32.62008101209,179.));
#35693=CARTESIAN_POINT('Ctrl Pts',(-33.5940729934507,32.6612738051671,179.));
#35694=CARTESIAN_POINT('Ctrl Pts',(-33.5716520331781,32.7016169140623,179.));
#35695=CARTESIAN_POINT('Ctrl Pts',(-33.5476436704819,32.740982949098,179.));
#35696=CARTESIAN_POINT('Ctrl Pts',(-33.539930599968,32.7536299174867,179.));
#35697=CARTESIAN_POINT('Ctrl Pts',(-33.5320525371695,32.7661776411531,179.));
#35698=CARTESIAN_POINT('Ctrl Pts',(-33.5240130248193,32.7786162809476,179.));
#35699=CARTESIAN_POINT('Ctrl Pts',(-33.4897680826177,32.8315996563409,179.));
#35700=CARTESIAN_POINT('Ctrl Pts',(-33.452666792504,32.8824995744465,179.));
#35701=CARTESIAN_POINT('Ctrl Pts',(-33.4127433280241,32.9310010385965,179.));
#35702=CARTESIAN_POINT('Ctrl Pts',(-33.3759774129278,32.9756665188152,179.));
#35703=CARTESIAN_POINT('Ctrl Pts',(-33.3368174942332,33.0182980198448,179.));
#35704=CARTESIAN_POINT('Ctrl Pts',(-33.2952688571158,33.0586167092817,179.));
#35705=CARTESIAN_POINT('Ctrl Pts',(-33.2874271595047,33.066226272256,179.));
#35706=CARTESIAN_POINT('Ctrl Pts',(-33.2795003199355,33.0737533467491,179.));
#35707=CARTESIAN_POINT('Ctrl Pts',(-33.2714899453066,33.081197259553,179.));
#35708=CARTESIAN_POINT('Origin',(-32.,32.,172.));
#35709=CARTESIAN_POINT('Origin',(32.,-32.,166.));
#35710=CARTESIAN_POINT('Ctrl Pts',(32.6750771856743,-33.5230977622536,166.));
#35711=CARTESIAN_POINT('Ctrl Pts',(32.7347503760542,-33.5045146947429,166.));
#35712=CARTESIAN_POINT('Ctrl Pts',(32.7931108063168,-33.4823562006339,166.));
#35713=CARTESIAN_POINT('Ctrl Pts',(32.8500021569922,-33.4569214580247,166.));
#35714=CARTESIAN_POINT('Ctrl Pts',(32.8860693067434,-33.4407967104194,166.));
#35715=CARTESIAN_POINT('Ctrl Pts',(32.9215460658915,-33.4233540969668,166.));
#35716=CARTESIAN_POINT('Ctrl Pts',(32.9563917054758,-33.404659418548,166.));
#35717=CARTESIAN_POINT('Ctrl Pts',(32.9799640056803,-33.3920128843712,166.));
#35718=CARTESIAN_POINT('Ctrl Pts',(33.0032474732066,-33.3787932129342,166.));
#35719=CARTESIAN_POINT('Ctrl Pts',(33.0262290482675,-33.3650188685718,166.));
#35720=CARTESIAN_POINT('Ctrl Pts',(33.0386995738435,-33.3575444760113,166.));
#35721=CARTESIAN_POINT('Ctrl Pts',(33.0510812979663,-33.349906528008,166.));
#35722=CARTESIAN_POINT('Ctrl Pts',(33.0633595552273,-33.3421161734122,166.));
#35723=CARTESIAN_POINT('Ctrl Pts',(33.1190572993812,-33.3067768603548,166.));
#35724=CARTESIAN_POINT('Ctrl Pts',(33.1726918020315,-33.2682673761069,166.));
#35725=CARTESIAN_POINT('Ctrl Pts',(33.2240815027149,-33.2268906436069,166.));
#35726=CARTESIAN_POINT('Ctrl Pts',(33.2611649249809,-33.1970326988656,166.));
#35727=CARTESIAN_POINT('Ctrl Pts',(33.2970793407966,-33.1656804905069,166.));
#35728=CARTESIAN_POINT('Ctrl Pts',(33.331751239224,-33.1329319505001,166.));
#35729=CARTESIAN_POINT('Ctrl Pts',(33.341130169451,-33.1240732988055,166.));
#35730=CARTESIAN_POINT('Ctrl Pts',(33.3504181471357,-33.1151124046011,166.));
#35731=CARTESIAN_POINT('Ctrl Pts',(33.3596136357983,-33.1060510586182,166.));
#35732=CARTESIAN_POINT('Ctrl Pts',(33.3693217679516,-33.0964845475258,166.));
#35733=CARTESIAN_POINT('Ctrl Pts',(33.3789213806408,-33.0868113554555,166.));
#35734=CARTESIAN_POINT('Ctrl Pts',(33.3884064304342,-33.0770387717059,166.));
#35735=CARTESIAN_POINT('Ctrl Pts',(33.4356624727154,-33.0283501890489,166.));
#35736=CARTESIAN_POINT('Ctrl Pts',(33.4801123153581,-32.9771629903732,166.));
#35737=CARTESIAN_POINT('Ctrl Pts',(33.5215724871592,-32.9237846837232,166.));
#35738=CARTESIAN_POINT('Ctrl Pts',(33.5636370688758,-32.8696282235729,166.));
#35739=CARTESIAN_POINT('Ctrl Pts',(33.6026250676343,-32.8132157239265,166.));
#35740=CARTESIAN_POINT('Ctrl Pts',(33.6383205150387,-32.7548214096818,166.));
#35741=CARTESIAN_POINT('Ctrl Pts',(33.6604358000209,-32.7186429333,166.));
#35742=CARTESIAN_POINT('Ctrl Pts',(33.6812867156679,-32.6817028484279,166.));
#35743=CARTESIAN_POINT('Ctrl Pts',(33.7008149846047,-32.6440590906012,166.));
#35744=CARTESIAN_POINT('Ctrl Pts',(33.7167940378195,-32.6132569948568,166.));
#35745=CARTESIAN_POINT('Ctrl Pts',(33.7318874487696,-32.5819836481081,166.));
#35746=CARTESIAN_POINT('Ctrl Pts',(33.7460599702932,-32.5502685810769,166.));
#35747=CARTESIAN_POINT('Ctrl Pts',(33.7518825626391,-32.5372388667638,166.));
#35748=CARTESIAN_POINT('Ctrl Pts',(33.7575505941886,-32.5241320517516,166.));
#35749=CARTESIAN_POINT('Ctrl Pts',(33.7630524074403,-32.5109727747132,166.));
#35750=CARTESIAN_POINT('Ctrl Pts',(33.7902429447907,-32.4459382492855,166.));
#35751=CARTESIAN_POINT('Ctrl Pts',(33.8134283639949,-32.3795135323734,166.));
#35752=CARTESIAN_POINT('Ctrl Pts',(33.8323972661765,-32.3119942831838,166.));
#35753=CARTESIAN_POINT('Ctrl Pts',(33.8345003970993,-32.3045082505449,166.));
#35754=CARTESIAN_POINT('Ctrl Pts',(33.8365516597232,-32.2970087243888,166.));
#35755=CARTESIAN_POINT('Ctrl Pts',(33.8385507377717,-32.289496079926,166.));
#35756=CARTESIAN_POINT('Ctrl Pts',(33.8558907757732,-32.2243312702931,166.));
#35757=CARTESIAN_POINT('Ctrl Pts',(33.8693084131536,-32.1581815103793,166.));
#35758=CARTESIAN_POINT('Ctrl Pts',(33.8789576017747,-32.0913509620122,166.));
#35759=CARTESIAN_POINT('Ctrl Pts',(33.8893365621853,-32.0194659939633,166.));
#35760=CARTESIAN_POINT('Ctrl Pts',(33.8953561186344,-31.9467925747811,166.));
#35761=CARTESIAN_POINT('Ctrl Pts',(33.8971477275179,-31.8736867160727,166.));
#35762=CARTESIAN_POINT('Ctrl Pts',(33.8974690086716,-31.860576971616,166.));
#35763=CARTESIAN_POINT('Ctrl Pts',(33.8976541694756,-31.8474532863635,166.));
#35764=CARTESIAN_POINT('Ctrl Pts',(33.8977037596136,-31.8343176784703,166.));
#35765=CARTESIAN_POINT('Ctrl Pts',(33.8977482919681,-31.822521793821,166.));
#35766=CARTESIAN_POINT('Ctrl Pts',(33.8976834443603,-31.8107249832838,166.));
#35767=CARTESIAN_POINT('Ctrl Pts',(33.8975101603586,-31.7989319884199,166.));
#35768=CARTESIAN_POINT('Ctrl Pts',(33.8964660328365,-31.7278729732675,166.));
#35769=CARTESIAN_POINT('Ctrl Pts',(33.8914891212925,-31.6569173776407,166.));
#35770=CARTESIAN_POINT('Ctrl Pts',(33.8827594412152,-31.5864004570563,166.));
#35771=CARTESIAN_POINT('Ctrl Pts',(33.8738459764261,-31.5143989537815,166.));
#35772=CARTESIAN_POINT('Ctrl Pts',(33.8610201205185,-31.4428538557896,166.));
#35773=CARTESIAN_POINT('Ctrl Pts',(33.8444208017163,-31.372105876886,166.));
#35774=CARTESIAN_POINT('Ctrl Pts',(33.8277211663871,-31.3009303387787,166.));
#35775=CARTESIAN_POINT('Ctrl Pts',(33.8072022424601,-31.230560513906,166.));
#35776=CARTESIAN_POINT('Ctrl Pts',(33.7829530935618,-31.1613424178325,166.));
#35777=CARTESIAN_POINT('Ctrl Pts',(33.776968914429,-31.1442608498207,166.));
#35778=CARTESIAN_POINT('Ctrl Pts',(33.7707573200257,-31.1272494615429,166.));
#35779=CARTESIAN_POINT('Ctrl Pts',(33.7643191706925,-31.1103135634024,166.));
#35780=CARTESIAN_POINT('Ctrl Pts',(33.7592568095487,-31.0969967501004,166.));
#35781=CARTESIAN_POINT('Ctrl Pts',(33.7540536136439,-31.0837250447109,166.));
#35782=CARTESIAN_POINT('Ctrl Pts',(33.7487184107884,-31.0705211529768,166.));
#35783=CARTESIAN_POINT('Ctrl Pts',(33.7204961745858,-31.0006750081532,166.));
#35784=CARTESIAN_POINT('Ctrl Pts',(33.6885374879799,-30.9325996700734,166.));
#35785=CARTESIAN_POINT('Ctrl Pts',(33.6530002982109,-30.8666520485507,166.));
#35786=CARTESIAN_POINT('Ctrl Pts',(33.6174247937608,-30.8006333251176,166.));
#35787=CARTESIAN_POINT('Ctrl Pts',(33.5782628944527,-30.7367457943838,166.));
#35788=CARTESIAN_POINT('Ctrl Pts',(33.535621294945,-30.6753519547081,166.));
#35789=CARTESIAN_POINT('Ctrl Pts',(33.493948975091,-30.6153536489791,166.));
#35790=CARTESIAN_POINT('Ctrl Pts',(33.4489530121136,-30.5577359733306,166.));
#35791=CARTESIAN_POINT('Ctrl Pts',(33.4006876492858,-30.5028568787942,166.));
#35792=CARTESIAN_POINT('Ctrl Pts',(33.3903602016106,-30.4911142761474,166.));
#35793=CARTESIAN_POINT('Ctrl Pts',(33.3798829091455,-30.4794971604396,166.));
#35794=CARTESIAN_POINT('Ctrl Pts',(33.3692560474651,-30.4680092249008,166.));
#35795=CARTESIAN_POINT('Ctrl Pts',(33.3601453511699,-30.4581603066688,166.));
#35796=CARTESIAN_POINT('Ctrl Pts',(33.3509247182145,-30.4484063385474,166.));
#35797=CARTESIAN_POINT('Ctrl Pts',(33.3415960097258,-30.4387477375165,166.));
#35798=CARTESIAN_POINT('Ctrl Pts',(32.3836679988471,-29.9813874990081,166.));
#35799=CARTESIAN_POINT('Ctrl Pts',(32.3093572584666,-29.9743675638755,166.));
#35800=CARTESIAN_POINT('Ctrl Pts',(32.2347977196974,-29.9717511907948,166.));
#35801=CARTESIAN_POINT('Ctrl Pts',(32.1603115654658,-29.9733742904635,166.));
#35802=CARTESIAN_POINT('Ctrl Pts',(32.087775690845,-29.9749548923253,166.));
#35803=CARTESIAN_POINT('Ctrl Pts',(32.0153086251354,-29.9805565182174,166.));
#35804=CARTESIAN_POINT('Ctrl Pts',(31.9432210973507,-29.9900715015274,166.));
#35805=CARTESIAN_POINT('Ctrl Pts',(31.927131309006,-29.9921952262863,166.));
#35806=CARTESIAN_POINT('Ctrl Pts',(31.9110583819063,-29.9945143961476,166.));
#35807=CARTESIAN_POINT('Ctrl Pts',(31.8950127157556,-29.9970270004263,166.));
#35808=CARTESIAN_POINT('Ctrl Pts',(31.8213764435297,-30.0085577658633,166.));
#35809=CARTESIAN_POINT('Ctrl Pts',(31.7484593964697,-30.0241343107327,166.));
#35810=CARTESIAN_POINT('Ctrl Pts',(31.6765936635792,-30.0436165987319,166.));
#35811=CARTESIAN_POINT('Ctrl Pts',(31.6261432264039,-30.0572933526897,166.));
#35812=CARTESIAN_POINT('Ctrl Pts',(31.5762111690267,-30.0728960169528,166.));
#35813=CARTESIAN_POINT('Ctrl Pts',(31.5269203206072,-30.0903892863566,166.));
#35814=CARTESIAN_POINT('Ctrl Pts',(31.5081989792638,-30.097033470383,166.));
#35815=CARTESIAN_POINT('Ctrl Pts',(31.4895702208887,-30.103950492905,166.));
#35816=CARTESIAN_POINT('Ctrl Pts',(31.4710411087259,-30.1111387813751,166.));
#35817=CARTESIAN_POINT('Ctrl Pts',(31.4533390621205,-30.1180062133595,166.));
#35818=CARTESIAN_POINT('Ctrl Pts',(31.4357224886101,-30.1251236957699,166.));
#35819=CARTESIAN_POINT('Ctrl Pts',(31.4182285084939,-30.1324766056846,166.));
#35820=CARTESIAN_POINT('Ctrl Pts',(31.3512969653627,-30.1606086604728,166.));
#35821=CARTESIAN_POINT('Ctrl Pts',(31.2860855769426,-30.1922088519133,166.));
#35822=CARTESIAN_POINT('Ctrl Pts',(31.2229027128029,-30.2271495142053,166.));
#35823=CARTESIAN_POINT('Ctrl Pts',(31.1610753343667,-30.2613405813522,166.));
#35824=CARTESIAN_POINT('Ctrl Pts',(31.101189679297,-30.2987309556031,166.));
#35825=CARTESIAN_POINT('Ctrl Pts',(31.0435670658395,-30.3392378236749,166.));
#35826=CARTESIAN_POINT('Ctrl Pts',(30.9872087901503,-30.3788559024312,166.));
#35827=CARTESIAN_POINT('Ctrl Pts',(30.9330147735939,-30.4214557401947,166.));
#35828=CARTESIAN_POINT('Ctrl Pts',(30.8813260918099,-30.4669870571697,166.));
#35829=CARTESIAN_POINT('Ctrl Pts',(30.8645071656146,-30.4818024448589,166.));
#35830=CARTESIAN_POINT('Ctrl Pts',(30.847953859026,-30.4969283974564,166.));
#35831=CARTESIAN_POINT('Ctrl Pts',(30.8316790249109,-30.5123636843746,166.));
#35832=CARTESIAN_POINT('Ctrl Pts',(30.8225443903146,-30.5210271033005,166.));
#35833=CARTESIAN_POINT('Ctrl Pts',(30.8134966581499,-30.5297889376287,166.));
#35834=CARTESIAN_POINT('Ctrl Pts',(30.8045505687119,-30.5386363394549,166.));
#35835=CARTESIAN_POINT('Ctrl Pts',(30.7559814459807,-30.5866696782818,166.));
#35836=CARTESIAN_POINT('Ctrl Pts',(30.7103173349291,-30.6373041034516,166.));
#35837=CARTESIAN_POINT('Ctrl Pts',(30.6678507708474,-30.6904581549245,166.));
#35838=CARTESIAN_POINT('Ctrl Pts',(30.661746870727,-30.6980982131255,166.));
#35839=CARTESIAN_POINT('Ctrl Pts',(30.655709102983,-30.7057903755372,166.));
#35840=CARTESIAN_POINT('Ctrl Pts',(30.6497384120877,-30.7135344486893,166.));
#35841=CARTESIAN_POINT('Ctrl Pts',(30.6073794462891,-30.7684746449824,166.));
#35842=CARTESIAN_POINT('Ctrl Pts',(30.5683925078902,-30.8260262206115,166.));
#35843=CARTESIAN_POINT('Ctrl Pts',(30.5328447155065,-30.885827412865,166.));
#35844=CARTESIAN_POINT('Ctrl Pts',(30.4996835114472,-30.9416137052429,166.));
#35845=CARTESIAN_POINT('Ctrl Pts',(30.4695155660164,-30.9993586633756,166.));
#35846=CARTESIAN_POINT('Ctrl Pts',(30.4424350809432,-31.0587740427515,166.));
#35847=CARTESIAN_POINT('Ctrl Pts',(30.4365397345137,-31.0717086059145,166.));
#35848=CARTESIAN_POINT('Ctrl Pts',(30.4307908557492,-31.0847223260546,166.));
#35849=CARTESIAN_POINT('Ctrl Pts',(30.4251896623469,-31.0978122019056,166.));
#35850=CARTESIAN_POINT('Ctrl Pts',(30.4206631621282,-31.1083905414929,166.));
#35851=CARTESIAN_POINT('Ctrl Pts',(30.4162333388954,-31.1190183106247,166.));
#35852=CARTESIAN_POINT('Ctrl Pts',(30.4119058547031,-31.1296809021722,166.));
#35853=CARTESIAN_POINT('Ctrl Pts',(30.386195392612,-31.1930295231227,166.));
#35854=CARTESIAN_POINT('Ctrl Pts',(30.3640425170158,-31.2577226660332,166.));
#35855=CARTESIAN_POINT('Ctrl Pts',(30.3454933793611,-31.3234107110985,166.));
#35856=CARTESIAN_POINT('Ctrl Pts',(30.3270295327823,-31.3887967149504,166.));
#35857=CARTESIAN_POINT('Ctrl Pts',(30.312136352138,-31.4551696274359,166.));
#35858=CARTESIAN_POINT('Ctrl Pts',(30.3009104203693,-31.5221872556072,166.));
#35859=CARTESIAN_POINT('Ctrl Pts',(30.2899245304527,-31.5877718592491,166.));
#35860=CARTESIAN_POINT('Ctrl Pts',(30.282450863886,-31.6539748650791,166.));
#35861=CARTESIAN_POINT('Ctrl Pts',(30.278627835107,-31.7204626904435,166.));
#35862=CARTESIAN_POINT('Ctrl Pts',(30.2778239865627,-31.7344427425749,166.));
#35863=CARTESIAN_POINT('Ctrl Pts',(30.2771817056382,-31.7484353120607,166.));
#35864=CARTESIAN_POINT('Ctrl Pts',(30.2767025483352,-31.7624371631597,166.));
#35865=CARTESIAN_POINT('Ctrl Pts',(30.2762461598509,-31.7757736678089,166.));
#35866=CARTESIAN_POINT('Ctrl Pts',(30.2759378587872,-31.7891204534951,166.));
#35867=CARTESIAN_POINT('Ctrl Pts',(30.2757789675672,-31.8024530389158,166.));
#35868=CARTESIAN_POINT('Ctrl Pts',(30.2750003669087,-31.8677855336075,166.));
#35869=CARTESIAN_POINT('Ctrl Pts',(30.2778001326965,-31.9328938376842,166.));
#35870=CARTESIAN_POINT('Ctrl Pts',(30.2842564554748,-31.9974683500875,166.));
#35871=CARTESIAN_POINT('Ctrl Pts',(30.2905902024686,-32.060816890404,166.));
#35872=CARTESIAN_POINT('Ctrl Pts',(30.3004431366813,-32.1236525831547,166.));
#35873=CARTESIAN_POINT('Ctrl Pts',(30.3139357387833,-32.1856659637692,166.));
#35874=CARTESIAN_POINT('Ctrl Pts',(30.3269907260027,-32.2456680215814,166.));
#35875=CARTESIAN_POINT('Ctrl Pts',(30.3434533492307,-32.3049008673228,166.));
#35876=CARTESIAN_POINT('Ctrl Pts',(30.363473861685,-32.3630572891802,166.));
#35877=CARTESIAN_POINT('Ctrl Pts',(30.3667806503312,-32.3726629871331,166.));
#35878=CARTESIAN_POINT('Ctrl Pts',(30.3701845915591,-32.3822392460162,166.));
#35879=CARTESIAN_POINT('Ctrl Pts',(30.3736864683761,-32.3917845902246,166.));
#35880=CARTESIAN_POINT('Ctrl Pts',(30.3774493182508,-32.4020412894562,166.));
#35881=CARTESIAN_POINT('Ctrl Pts',(30.3813252458597,-32.4122622947181,166.));
#35882=CARTESIAN_POINT('Ctrl Pts',(30.3853131952719,-32.4224462418484,166.));
#35883=CARTESIAN_POINT('Origin',(32.,-32.,180.545925280538));
#35884=CARTESIAN_POINT('Ctrl Pts',(29.9434031644741,-31.9984978685597,178.795925280538));
#35885=CARTESIAN_POINT('Ctrl Pts',(29.9425886530065,-31.900403685169,178.790592107115));
#35886=CARTESIAN_POINT('Ctrl Pts',(29.9935747042563,-31.1217949684998,178.748215670618));
#35887=CARTESIAN_POINT('Ctrl Pts',(30.988248508056,-29.7919884506806,178.668795971049));
#35888=CARTESIAN_POINT('Ctrl Pts',(33.3060963778469,-29.9525600136615,178.557666181829));
#35889=CARTESIAN_POINT('Ctrl Pts',(34.4285775821774,-31.9866392352977,178.446536392609));
#35890=CARTESIAN_POINT('Ctrl Pts',(33.3284712654795,-34.033087144352,178.33540660339));
#35891=CARTESIAN_POINT('Ctrl Pts',(31.0125524608971,-34.2188064667841,178.22427681417));
#35892=CARTESIAN_POINT('Ctrl Pts',(29.9981273513597,-32.8935904489542,178.144449706553));
#35893=CARTESIAN_POINT('Ctrl Pts',(29.9426985167512,-32.1072447552094,178.101665862009));
#35894=CARTESIAN_POINT('Ctrl Pts',(29.943606531648,-32.0016074863584,178.095925280538));
#35895=CARTESIAN_POINT('Ctrl Pts',(29.9473399238087,-32.0021821257033,178.854074719462));
#35896=CARTESIAN_POINT('Ctrl Pts',(29.950876284898,-31.5321178460643,178.828629953495));
#35897=CARTESIAN_POINT('Ctrl Pts',(30.3432698790764,-30.3707968848796,178.766141924455));
#35898=CARTESIAN_POINT('Ctrl Pts',(32.2716026642884,-29.5870613462295,178.666610632341));
#35899=CARTESIAN_POINT('Ctrl Pts',(34.1744104601116,-30.9184848843002,178.555480843121));
#35900=CARTESIAN_POINT('Ctrl Pts',(34.0880400722661,-33.2405822108959,178.444351053901));
#35901=CARTESIAN_POINT('Ctrl Pts',(32.0903159787745,-34.4268786410256,178.333221264682));
#35902=CARTESIAN_POINT('Ctrl Pts',(30.2791369268827,-33.526119436994,178.236462486535));
#35903=CARTESIAN_POINT('Ctrl Pts',(29.9500603938313,-32.4182642842386,178.176746971462));
#35904=CARTESIAN_POINT('Ctrl Pts',(29.9478812476528,-31.9988328933335,178.154074719462));
#35905=CARTESIAN_POINT('Ctrl Pts',(33.2690708798528,-30.920641346952,179.));
#35906=CARTESIAN_POINT('Ctrl Pts',(33.6279571482409,-31.3426068457268,178.962956736927));
#35907=CARTESIAN_POINT('Ctrl Pts',(33.8850557275035,-32.5658743636166,178.88887021078));
#35908=CARTESIAN_POINT('Ctrl Pts',(32.5454537305004,-33.893241966271,178.777740421561));
#35909=CARTESIAN_POINT('Ctrl Pts',(30.7060861201286,-33.483868903691,178.666610632341));
#35910=CARTESIAN_POINT('Ctrl Pts',(30.0511744258997,-31.7184481767343,178.555480843121));
#35911=CARTESIAN_POINT('Ctrl Pts',(31.1796676064832,-30.2097348868884,178.444351053901));
#35912=CARTESIAN_POINT('Ctrl Pts',(33.0589884732901,-30.339926990028,178.333221264682));
#35913=CARTESIAN_POINT('Ctrl Pts',(33.9691009864497,-31.9891670354087,178.222091475462));
#35914=CARTESIAN_POINT('Ctrl Pts',(33.07713012692,-33.6484356649181,178.110961686242));
#35915=CARTESIAN_POINT('Ctrl Pts',(31.1993733543519,-33.7990176778987,177.999831897022));
#35916=CARTESIAN_POINT('Ctrl Pts',(30.0543453845802,-32.3031858100374,177.888702107803));
#35917=CARTESIAN_POINT('Ctrl Pts',(30.6899574647931,-30.5298680270273,177.777572318583));
#35918=CARTESIAN_POINT('Ctrl Pts',(32.5245072262386,-30.102005737538,177.666442529363));
#35919=CARTESIAN_POINT('Ctrl Pts',(33.8790331908656,-31.4111639457544,177.555312740143));
#35920=CARTESIAN_POINT('Ctrl Pts',(33.5138885880054,-33.2592201303934,177.444182950924));
#35921=CARTESIAN_POINT('Ctrl Pts',(31.7632494531294,-33.9548509189774,177.333053161704));
#35922=CARTESIAN_POINT('Ctrl Pts',(30.2292819071445,-32.8614237331979,177.221923372484));
#35923=CARTESIAN_POINT('Ctrl Pts',(30.3158563296739,-30.9796306983742,177.110793583265));
#35924=CARTESIAN_POINT('Ctrl Pts',(31.9437407889795,-30.0316686763551,176.999663794045));
#35925=CARTESIAN_POINT('Ctrl Pts',(33.6231130614891,-30.8851020901988,176.888534004825));
#35926=CARTESIAN_POINT('Ctrl Pts',(33.8170298653015,-32.758878003058,176.777404215605));
#35927=CARTESIAN_POINT('Ctrl Pts',(32.3480206396625,-33.9381369861425,176.666274426386));
#35928=CARTESIAN_POINT('Ctrl Pts',(30.5605066995148,-33.3436340231644,176.555144637166));
#35929=CARTESIAN_POINT('Ctrl Pts',(30.0904014169314,-31.5194517706213,176.444014847946));
#35930=CARTESIAN_POINT('Ctrl Pts',(31.3679400490272,-30.135062047588,176.332885058727));
#35931=CARTESIAN_POINT('Ctrl Pts',(33.2239330937557,-30.4574433135484,176.221755269507));
#35932=CARTESIAN_POINT('Ctrl Pts',(33.9597958441263,-32.1915557309348,176.110625480287));
#35933=CARTESIAN_POINT('Ctrl Pts',(32.9020746910311,-33.7503584205498,175.999495691067));
#35934=CARTESIAN_POINT('Ctrl Pts',(31.0187845633079,-33.7072520656006,175.888365901848));
#35935=CARTESIAN_POINT('Ctrl Pts',(30.0334921624016,-32.1016871345539,175.777236112628));
#35936=CARTESIAN_POINT('Ctrl Pts',(30.8479264085786,-30.403059240733,175.666106323408));
#35937=CARTESIAN_POINT('Ctrl Pts',(32.7167259119053,-30.1659342116828,175.554976534189));
#35938=CARTESIAN_POINT('Ctrl Pts',(33.9295856332257,-31.6073263024897,175.443846744969));
#35939=CARTESIAN_POINT('Ctrl Pts',(33.3765095085026,-33.4080891028869,175.332716955749));
#35940=CARTESIAN_POINT('Ctrl Pts',(31.563666809222,-33.9201840264136,175.221587166529));
#35941=CARTESIAN_POINT('Ctrl Pts',(30.150151514305,-32.6749473524947,175.11045737731));
#35942=CARTESIAN_POINT('Ctrl Pts',(30.4295974927246,-30.8120061810721,174.99932758809));
#35943=CARTESIAN_POINT('Ctrl Pts',(32.1462588154966,-30.0363040694758,174.88819779887));
#35944=CARTESIAN_POINT('Ctrl Pts',(33.729065656437,-31.0577551780996,174.77706800965));
#35945=CARTESIAN_POINT('Ctrl Pts',(33.7294503595424,-32.9415385295071,174.665938220431));
#35946=CARTESIAN_POINT('Ctrl Pts',(32.1470608487029,-33.9636360292698,174.554808431211));
#35947=CARTESIAN_POINT('Ctrl Pts',(30.4300828439389,-33.1886351297909,174.443678641991));
#35948=CARTESIAN_POINT('Ctrl Pts',(30.1498759953595,-31.3258082497385,174.332548852772));
#35949=CARTESIAN_POINT('Ctrl Pts',(31.5628825720676,-30.0799943482204,174.221419063552));
#35950=CARTESIAN_POINT('Ctrl Pts',(33.3759342784784,-30.5913487976167,174.110289274332));
#35951=CARTESIAN_POINT('Ctrl Pts',(33.9297458546116,-32.391885551248,173.999159485112));
#35952=CARTESIAN_POINT('Ctrl Pts',(32.7174749518267,-33.833772898199,173.888029695892));
#35953=CARTESIAN_POINT('Ctrl Pts',(30.8485787538218,-33.5974111751572,173.776899906673));
#35954=CARTESIAN_POINT('Ctrl Pts',(30.0334507936758,-31.8991160678144,173.665770117453));
#35955=CARTESIAN_POINT('Ctrl Pts',(31.0180873408195,-30.2931488411672,173.554640328233));
#35956=CARTESIAN_POINT('Ctrl Pts',(32.901359705246,-30.2492732850537,173.443510539014));
#35957=CARTESIAN_POINT('Ctrl Pts',(33.9597174422702,-31.8076438326184,173.332380749794));
#35958=CARTESIAN_POINT('Ctrl Pts',(33.2245630283795,-33.542056658555,173.221250960574));
#35959=CARTESIAN_POINT('Ctrl Pts',(31.3687018107489,-33.8651959534902,173.110121171354));
#35960=CARTESIAN_POINT('Ctrl Pts',(30.0905978497772,-32.4813281389989,172.998991382135));
#35961=CARTESIAN_POINT('Ctrl Pts',(30.5599580300852,-30.6569540314822,172.887861592915));
#35962=CARTESIAN_POINT('Ctrl Pts',(32.3472290046545,-30.0617210296259,172.776731803695));
#35963=CARTESIAN_POINT('Ctrl Pts',(33.8167197597056,-31.2403799216958,172.665602014475));
#35964=CARTESIAN_POINT('Ctrl Pts',(33.6235682921796,-33.114234871693,172.554472225256));
#35965=CARTESIAN_POINT('Ctrl Pts',(31.9445447305158,-33.9683541504908,172.443342436036));
#35966=CARTESIAN_POINT('Ctrl Pts',(30.3162732300965,-33.0210570566713,172.332212646816));
#35967=CARTESIAN_POINT('Ctrl Pts',(30.2289302102365,-31.139299617489,172.221082857597));
#35968=CARTESIAN_POINT('Ctrl Pts',(31.7624510555159,-30.0452458344737,172.109953068377));
#35969=CARTESIAN_POINT('Ctrl Pts',(33.5133741186761,-30.740161865322,171.998823279157));
#35970=CARTESIAN_POINT('Ctrl Pts',(33.8792736002829,-32.5880680946519,171.887693489937));
#35971=CARTESIAN_POINT('Ctrl Pts',(32.5252822627843,-33.8977807810893,171.776563700718));
#35972=CARTESIAN_POINT('Ctrl Pts',(30.6905582948345,-33.4706650772494,171.665433911498));
#35973=CARTESIAN_POINT('Ctrl Pts',(30.0542211751481,-31.6976126434095,171.554304122278));
#35974=CARTESIAN_POINT('Ctrl Pts',(31.1986397348735,-30.2013018390669,171.443174333059));
#35975=CARTESIAN_POINT('Ctrl Pts',(33.0764545188525,-30.3511400855409,171.332044543839));
#35976=CARTESIAN_POINT('Ctrl Pts',(33.9691098008408,-32.0099970445868,171.220914754619));
#35977=CARTESIAN_POINT('Ctrl Pts',(33.0596571472062,-33.6597048168402,171.1097849654));
#35978=CARTESIAN_POINT('Ctrl Pts',(31.1804177639518,-33.7904687394708,170.99865517618));
#35979=CARTESIAN_POINT('Ctrl Pts',(30.0512511551294,-32.2826150885626,170.88752538696));
#35980=CARTESIAN_POINT('Ctrl Pts',(30.7055583558314,-30.516115173435,170.77639559774));
#35981=CARTESIAN_POINT('Ctrl Pts',(32.5445245116414,-30.1076505595188,170.665265808521));
#35982=CARTESIAN_POINT('Ctrl Pts',(33.8851477395197,-31.4310436318559,170.554136019301));
#35983=CARTESIAN_POINT('Ctrl Pts',(33.5005041997655,-33.2751394022435,170.443006230081));
#35984=CARTESIAN_POINT('Ctrl Pts',(31.7426154886764,-33.952241420009,170.331876440861));
#35985=CARTESIAN_POINT('Ctrl Pts',(30.2202822911319,-32.8426732613587,170.220746651642));
#35986=CARTESIAN_POINT('Ctrl Pts',(30.3267274405086,-30.9618996723241,170.109616862422));
#35987=CARTESIAN_POINT('Ctrl Pts',(31.9645334904465,-30.0311842454491,169.998487073202));
#35988=CARTESIAN_POINT('Ctrl Pts',(33.6347981053096,-30.9023076462213,169.887357283982));
#35989=CARTESIAN_POINT('Ctrl Pts',(33.8089132228404,-32.7780271851939,169.776227494763));
#35990=CARTESIAN_POINT('Ctrl Pts',(32.3275305756749,-33.9417046816305,169.665097705543));
#35991=CARTESIAN_POINT('Ctrl Pts',(30.5463954975727,-33.3283551103494,169.553967916323));
#35992=CARTESIAN_POINT('Ctrl Pts',(30.095583496408,-31.4993093474876,169.442838127103));
#35993=CARTESIAN_POINT('Ctrl Pts',(31.3876728267927,-30.1284902400415,169.331708337884));
#35994=CARTESIAN_POINT('Ctrl Pts',(33.2401573456871,-30.4704565692305,169.220578548664));
#35995=CARTESIAN_POINT('Ctrl Pts',(33.9576633107509,-32.2122444590535,169.109448759444));
#35996=CARTESIAN_POINT('Ctrl Pts',(32.8835370437985,-33.7597885216428,168.998318970225));
#35997=CARTESIAN_POINT('Ctrl Pts',(31.0008072559047,-33.6967932133432,168.887189181005));
#35998=CARTESIAN_POINT('Ctrl Pts',(30.032527831648,-32.0809111571343,168.776059391785));
#35999=CARTESIAN_POINT('Ctrl Pts',(30.8648575994482,-30.3909800873892,168.664929602566));
#36000=CARTESIAN_POINT('Ctrl Pts',(32.7360573822727,-30.1736065925138,168.553799813346));
#36001=CARTESIAN_POINT('Ctrl Pts',(33.9336254307537,-31.6277285378747,168.442670024126));
#36002=CARTESIAN_POINT('Ctrl Pts',(33.3615604549092,-33.4225492880192,168.331540234906));
#36003=CARTESIAN_POINT('Ctrl Pts',(31.543410115007,-33.9154683571568,168.220410445686));
#36004=CARTESIAN_POINT('Ctrl Pts',(30.1431258888499,-32.6553715572293,168.109280656467));
#36005=CARTESIAN_POINT('Ctrl Pts',(30.4422327071443,-30.7954858173387,167.998150867247));
#36006=CARTESIAN_POINT('Ctrl Pts',(32.1669912689855,-30.0379583909259,167.887021078027));
#36007=CARTESIAN_POINT('Ctrl Pts',(33.7389212112043,-31.0760701759928,167.775891288808));
#36008=CARTESIAN_POINT('Ctrl Pts',(33.7194093618925,-32.9597524994687,167.664761499588));
#36009=CARTESIAN_POINT('Ctrl Pts',(32.1263126229409,-33.9650797779653,167.553631710368));
#36010=CARTESIAN_POINT('Ctrl Pts',(30.4176161201555,-33.1719872839235,167.442501921148));
#36011=CARTESIAN_POINT('Ctrl Pts',(30.1570998197528,-31.306304880134,167.331372131929));
#36012=CARTESIAN_POINT('Ctrl Pts',(31.5831865204611,-30.0754844364286,167.220242342709));
#36013=CARTESIAN_POINT('Ctrl Pts',(33.3907348875884,-30.6059603581105,167.109112553489));
#36014=CARTESIAN_POINT('Ctrl Pts',(33.9255008417806,-32.4122450367323,166.997982764269));
#36015=CARTESIAN_POINT('Ctrl Pts',(32.6980630472242,-33.8412499830313,166.88685297505));
#36016=CARTESIAN_POINT('Ctrl Pts',(30.8317782670075,-33.5851579144293,166.77572318583));
#36017=CARTESIAN_POINT('Ctrl Pts',(30.0346113980645,-31.878356689149,166.664593396611));
#36018=CARTESIAN_POINT('Ctrl Pts',(31.0361997002367,-30.2828613829585,166.55346360739));
#36019=CARTESIAN_POINT('Ctrl Pts',(32.9197400051123,-30.2589149050105,166.442333818171));
#36020=CARTESIAN_POINT('Ctrl Pts',(33.9617632742068,-31.8283047261835,166.331204028951));
#36021=CARTESIAN_POINT('Ctrl Pts',(33.2079560627009,-33.5550031183362,166.220074239732));
#36022=CARTESIAN_POINT('Ctrl Pts',(31.3495488780108,-33.8582231808284,166.108944450512));
#36023=CARTESIAN_POINT('Ctrl Pts',(30.0845739050515,-32.4615493362111,165.997814661292));
#36024=CARTESIAN_POINT('Ctrl Pts',(30.5763937621187,-30.6409583631627,165.886684872072));
#36025=CARTESIAN_POINT('Ctrl Pts',(31.7668777668628,-30.2598665970073,165.812598345926));
#36026=CARTESIAN_POINT('Ctrl Pts',(32.3110796379508,-30.3633004372053,165.775555082853));
#36027=CARTESIAN_POINT('Ctrl Pts',(33.3677806246593,-30.8366876301908,179.074814972382));
#36028=CARTESIAN_POINT('Ctrl Pts',(33.7545814662438,-31.2914740748737,179.037771709309));
#36029=CARTESIAN_POINT('Ctrl Pts',(34.0316774590095,-32.6098887011227,178.963685183163));
#36030=CARTESIAN_POINT('Ctrl Pts',(32.587879728446,-34.0405004325351,178.852555393943));
#36031=CARTESIAN_POINT('Ctrl Pts',(30.6054440591442,-33.5992858777425,178.741425604723));
#36032=CARTESIAN_POINT('Ctrl Pts',(29.899592604785,-31.6965487627099,178.630295815504));
#36033=CARTESIAN_POINT('Ctrl Pts',(31.1158612403408,-30.0704860748191,178.519166026284));
#36034=CARTESIAN_POINT('Ctrl Pts',(33.141357774809,-30.2108046645725,178.408036237064));
#36035=CARTESIAN_POINT('Ctrl Pts',(34.1222598516922,-31.9883244353717,178.296906447844));
#36036=CARTESIAN_POINT('Ctrl Pts',(33.1609105064398,-33.7766528247294,178.185776658625));
#36037=CARTESIAN_POINT('Ctrl Pts',(31.1370997232003,-33.9389472741939,178.074646869405));
#36038=CARTESIAN_POINT('Ctrl Pts',(29.9030102041591,-32.3267679396196,177.963517080185));
#36039=CARTESIAN_POINT('Ctrl Pts',(30.5880608990545,-30.4155195267286,177.852387290966));
#36040=CARTESIAN_POINT('Ctrl Pts',(32.565303981781,-29.9543776323896,177.741257501746));
#36041=CARTESIAN_POINT('Ctrl Pts',(34.0251864827721,-31.3653636224075,177.630127712526));
#36042=CARTESIAN_POINT('Ctrl Pts',(33.6316405264983,-33.3571636729485,177.518997923307));
#36043=CARTESIAN_POINT('Ctrl Pts',(31.7448347322218,-34.1069013981196,177.407868134086));
#36044=CARTESIAN_POINT('Ctrl Pts',(30.0915534840557,-32.9284262294525,177.296738344867));
#36045=CARTESIAN_POINT('Ctrl Pts',(30.1848617614787,-30.900265238989,177.185608555647));
#36046=CARTESIAN_POINT('Ctrl Pts',(31.9393648849611,-29.8785696763417,177.074478766427));
#36047=CARTESIAN_POINT('Ctrl Pts',(33.7493606010357,-30.7983840905119,176.963348977208));
#36048=CARTESIAN_POINT('Ctrl Pts',(33.9583604695705,-32.8179043783459,176.852219187988));
#36049=CARTESIAN_POINT('Ctrl Pts',(32.3750900721692,-34.0888874369954,176.741089398768));
#36050=CARTESIAN_POINT('Ctrl Pts',(30.448541309246,-33.448143372205,176.629959609548));
#36051=CARTESIAN_POINT('Ctrl Pts',(29.941870714817,-31.4820741947568,176.518829820329));
#36052=CARTESIAN_POINT('Ctrl Pts',(31.3187777229086,-29.9900050990085,176.407700031109));
#36053=CARTESIAN_POINT('Ctrl Pts',(33.3191319713462,-30.3374615384667,176.296570241889));
#36054=CARTESIAN_POINT('Ctrl Pts',(34.1122309450475,-32.2064551487821,176.18544045267));
#36055=CARTESIAN_POINT('Ctrl Pts',(32.9722390640079,-33.8865032456776,176.07431066345));
#36056=CARTESIAN_POINT('Ctrl Pts',(30.9424645350938,-33.8400440304869,175.96318087423));
#36057=CARTESIAN_POINT('Ctrl Pts',(29.8805349951614,-32.1095964730009,175.85205108501));
#36058=CARTESIAN_POINT('Ctrl Pts',(30.7583168430193,-30.2788474119684,175.740921295791));
#36059=CARTESIAN_POINT('Ctrl Pts',(32.7724736506514,-30.0232785343702,175.629791506571));
#36060=CARTESIAN_POINT('Ctrl Pts',(34.0796709503359,-31.5767837054694,175.518661717351));
#36061=CARTESIAN_POINT('Ctrl Pts',(33.483575949365,-33.5176118397311,175.407531928131));
#36062=CARTESIAN_POINT('Ctrl Pts',(31.5297283282466,-34.0695380760871,175.296402138912));
#36063=CARTESIAN_POINT('Ctrl Pts',(30.006268241233,-32.7274455084135,175.185272349692));
#36064=CARTESIAN_POINT('Ctrl Pts',(30.3074498387223,-30.7196027002582,175.074142560473));
#36065=CARTESIAN_POINT('Ctrl Pts',(32.1576349888708,-29.8835656154959,174.963012771252));
#36066=CARTESIAN_POINT('Ctrl Pts',(33.863554306685,-30.9844663276567,174.851882982033));
#36067=CARTESIAN_POINT('Ctrl Pts',(33.863968932426,-33.014772443742,174.740753192813));
#36068=CARTESIAN_POINT('Ctrl Pts',(32.1584994051121,-34.1163698240635,174.629623403594));
#36069=CARTESIAN_POINT('Ctrl Pts',(30.307972941094,-33.2810884924772,174.518493614374));
#36070=CARTESIAN_POINT('Ctrl Pts',(30.0059712921174,-31.273368865402,174.407363825154));
#36071=CARTESIAN_POINT('Ctrl Pts',(31.528883092254,-29.9306541727243,174.296234035934));
#36072=CARTESIAN_POINT('Ctrl Pts',(33.4829559773097,-30.4817823400484,174.185104246715));
#36073=CARTESIAN_POINT('Ctrl Pts',(34.0798436339194,-32.4223668453752,174.073974457495));
#36074=CARTESIAN_POINT('Ctrl Pts',(32.7732809517312,-33.9764057941924,173.962844668275));
#36075=CARTESIAN_POINT('Ctrl Pts',(30.7590199284013,-33.721659593393,173.851714879055));
#36076=CARTESIAN_POINT('Ctrl Pts',(29.88049040873,-31.8912692033412,173.740585089836));
#36077=CARTESIAN_POINT('Ctrl Pts',(30.9417130818647,-30.1603880592551,173.629455300616));
#36078=CARTESIAN_POINT('Ctrl Pts',(32.971468465833,-30.113099813578,173.518325511396));
#36079=CARTESIAN_POINT('Ctrl Pts',(34.1121464450078,-31.7926821559338,173.407195722176));
#36080=CARTESIAN_POINT('Ctrl Pts',(33.3198109029858,-33.6619995409107,173.296065932957));
#36081=CARTESIAN_POINT('Ctrl Pts',(31.3195987353044,-34.0102729696805,173.184936143737));
#36082=CARTESIAN_POINT('Ctrl Pts',(29.942082426428,-32.5187663771014,173.073806354517));
#36083=CARTESIAN_POINT('Ctrl Pts',(30.4479499636978,-30.5524904219861,172.962676565298));
#36084=CARTESIAN_POINT('Ctrl Pts',(32.3742368629097,-29.9109595350815,172.851546776078));
#36085=CARTESIAN_POINT('Ctrl Pts',(33.9580262436163,-31.1812958269698,172.740416986858));
#36086=CARTESIAN_POINT('Ctrl Pts',(33.7498512400758,-33.2009012995383,172.629287197638));
#36087=CARTESIAN_POINT('Ctrl Pts',(31.9402313579644,-34.1214549260016,172.518157408419));
#36088=CARTESIAN_POINT('Ctrl Pts',(30.18531108888,-33.100476010409,172.407027619199));
#36089=CARTESIAN_POINT('Ctrl Pts',(30.0911744317709,-31.0723533842554,172.295897829979));
#36090=CARTESIAN_POINT('Ctrl Pts',(31.7439742343537,-29.8932028809226,172.184768040759));
#36091=CARTESIAN_POINT('Ctrl Pts',(33.6310860411722,-30.6421702537061,172.07363825154));
#36092=CARTESIAN_POINT('Ctrl Pts',(34.0254455915014,-32.6338086852473,171.96250846232));
#36093=CARTESIAN_POINT('Ctrl Pts',(32.5661393015313,-34.0453922814192,171.8513786731));
#36094=CARTESIAN_POINT('Ctrl Pts',(30.5887084623249,-33.5850550429918,171.74024888388));
#36095=CARTESIAN_POINT('Ctrl Pts',(29.9028763335792,-31.6740926184246,171.629119094661));
#36096=CARTESIAN_POINT('Ctrl Pts',(31.1363090419827,-30.0613970951568,171.517989305441));
#36097=CARTESIAN_POINT('Ctrl Pts',(33.1601823488252,-30.2228899271284,171.406859516221));
#36098=CARTESIAN_POINT('Ctrl Pts',(34.1222693516765,-32.0107746258359,171.295729727002));
#36099=CARTESIAN_POINT('Ctrl Pts',(33.1420784589262,-33.7887985038243,171.184599937782));
#36100=CARTESIAN_POINT('Ctrl Pts',(31.1166697458918,-33.9297333898248,171.073470148562));
#36101=CARTESIAN_POINT('Ctrl Pts',(29.8996753020995,-32.3045972045447,170.962340359342));
#36102=CARTESIAN_POINT('Ctrl Pts',(30.6048752447529,-30.4006969608846,170.851210570123));
#36103=CARTESIAN_POINT('Ctrl Pts',(32.5868782339104,-29.9604615149035,170.740080780903));
#36104=CARTESIAN_POINT('Ctrl Pts',(34.0317766278226,-31.386789572609,170.628950991683));
#36105=CARTESIAN_POINT('Ctrl Pts',(33.6172150856516,-33.3743211634725,170.517821202464));
#36106=CARTESIAN_POINT('Ctrl Pts',(31.7225958350595,-34.1040889294184,170.406691413244));
#36107=CARTESIAN_POINT('Ctrl Pts',(30.0818538678981,-32.9082173250549,170.295561624024));
#36108=CARTESIAN_POINT('Ctrl Pts',(30.1965784394077,-30.8811550740079,170.184431834804));
#36109=CARTESIAN_POINT('Ctrl Pts',(31.961774865879,-29.8780475658609,170.073302045585));
#36110=CARTESIAN_POINT('Ctrl Pts',(33.7619545205635,-30.8169279138221,169.962172256365));
#36111=CARTESIAN_POINT('Ctrl Pts',(33.9496125056294,-32.8385430051708,169.851042467145));
#36112=CARTESIAN_POINT('Ctrl Pts',(32.3530062682106,-34.0927326318073,169.739912677925));
#36113=CARTESIAN_POINT('Ctrl Pts',(30.4333325223188,-33.4316760485543,169.628782888706));
#36114=CARTESIAN_POINT('Ctrl Pts',(29.9474558622,-31.4603650715444,169.517653099486));
#36115=CARTESIAN_POINT('Ctrl Pts',(31.3400453380804,-29.9829221289604,169.406523310266));
#36116=CARTESIAN_POINT('Ctrl Pts',(33.3366181636415,-30.3514869796523,169.295393521046));
#36117=CARTESIAN_POINT('Ctrl Pts',(34.1099325408538,-32.228753069189,169.184263731827));
#36118=CARTESIAN_POINT('Ctrl Pts',(32.9522595379514,-33.896666830524,169.073133942607));
#36119=CARTESIAN_POINT('Ctrl Pts',(30.923088932722,-33.8287716770662,168.962004153387));
#36120=CARTESIAN_POINT('Ctrl Pts',(29.8794956576891,-32.0872045169454,168.850874364168));
#36121=CARTESIAN_POINT('Ctrl Pts',(30.7765649607498,-30.2658287286403,168.739744574948));
#36122=CARTESIAN_POINT('Ctrl Pts',(32.7933087442892,-30.0315476815174,168.628614785728));
#36123=CARTESIAN_POINT('Ctrl Pts',(34.0840249678096,-31.5987728494191,168.517484996508));
#36124=CARTESIAN_POINT('Ctrl Pts',(33.4674641417531,-33.5331967541492,168.406355207289));
#36125=CARTESIAN_POINT('Ctrl Pts',(31.5078960458211,-34.0644556168296,168.295225418069));
#36126=CARTESIAN_POINT('Ctrl Pts',(29.9986961548143,-32.7063470860153,168.184095628849));
#36127=CARTESIAN_POINT('Ctrl Pts',(30.3210678341756,-30.7017973642556,168.07296583963));
#36128=CARTESIAN_POINT('Ctrl Pts',(32.1799800356558,-29.8853486119087,167.96183605041));
#36129=CARTESIAN_POINT('Ctrl Pts',(33.8741764374659,-31.0042058864605,167.85070626119));
#36130=CARTESIAN_POINT('Ctrl Pts',(33.8531469348088,-33.0344031165493,167.73957647197));
#36131=CARTESIAN_POINT('Ctrl Pts',(32.1361373592691,-34.1179258691386,167.628446682751));
#36132=CARTESIAN_POINT('Ctrl Pts',(30.2945365416662,-33.2631457586385,167.517316893531));
#36133=CARTESIAN_POINT('Ctrl Pts',(30.0137569936081,-31.2523485020131,167.406187104311));
#36134=CARTESIAN_POINT('Ctrl Pts',(31.5507663043405,-29.9257934749763,167.295057315091));
#36135=CARTESIAN_POINT('Ctrl Pts',(33.4989077942611,-30.4975304039719,167.183927525872));
#36136=CARTESIAN_POINT('Ctrl Pts',(34.075268439268,-32.4443099142892,167.072797736652));
#36137=CARTESIAN_POINT('Ctrl Pts',(32.752359167594,-33.9844644550008,166.961667947433));
#36138=CARTESIAN_POINT('Ctrl Pts',(30.740912681033,-33.7084532604145,166.850538158212));
#36139=CARTESIAN_POINT('Ctrl Pts',(29.8817412862193,-31.8688951371095,166.739408368993));
#36140=CARTESIAN_POINT('Ctrl Pts',(30.9612342407464,-30.1493004311028,166.628278579773));
#36141=CARTESIAN_POINT('Ctrl Pts',(32.9912784058701,-30.1234913694608,166.517148790553));
#36142=CARTESIAN_POINT('Ctrl Pts',(34.1143514040283,-31.8149500767845,166.406019001334));
#36143=CARTESIAN_POINT('Ctrl Pts',(33.3019122290424,-33.6759529907359,166.294889212114));
#36144=CARTESIAN_POINT('Ctrl Pts',(31.2989560661514,-34.0027578470042,166.183759422894));
#36145=CARTESIAN_POINT('Ctrl Pts',(29.9355899325803,-32.4974491570299,166.072629633675));
#36146=CARTESIAN_POINT('Ctrl Pts',(30.4656640852527,-30.5352505927904,165.961499844455));
#36147=CARTESIAN_POINT('Ctrl Pts',(31.7487452602337,-30.1245170851199,165.887413318308));
#36148=CARTESIAN_POINT('Ctrl Pts',(32.3352757582496,-30.2359961244729,165.850370055235));
#36149=CARTESIAN_POINT('Ctrl Pts',(33.4664903694657,-30.7527339134296,179.149629944765));
#36150=CARTESIAN_POINT('Ctrl Pts',(33.8812057842467,-31.2403413040207,179.112586681692));
#36151=CARTESIAN_POINT('Ctrl Pts',(34.1782991905155,-32.653903038629,179.038500155545));
#36152=CARTESIAN_POINT('Ctrl Pts',(32.6303057263916,-34.1877588987991,178.927370366325));
#36153=CARTESIAN_POINT('Ctrl Pts',(30.5048019981598,-33.7147028517942,178.816240577106));
#36154=CARTESIAN_POINT('Ctrl Pts',(29.7480107836703,-31.6746493486853,178.705110787886));
#36155=CARTESIAN_POINT('Ctrl Pts',(31.0520548741984,-29.9312372627499,178.593980998666));
#36156=CARTESIAN_POINT('Ctrl Pts',(33.223727076328,-30.081682339117,178.482851209447));
#36157=CARTESIAN_POINT('Ctrl Pts',(34.2754187169348,-31.9874818353347,178.371721420227));
#36158=CARTESIAN_POINT('Ctrl Pts',(33.2446908859597,-33.9048699845407,178.260591631007));
#36159=CARTESIAN_POINT('Ctrl Pts',(31.0748260920487,-34.0788768704889,178.149461841788));
#36160=CARTESIAN_POINT('Ctrl Pts',(29.751675023738,-32.3503500692018,178.038332052568));
#36161=CARTESIAN_POINT('Ctrl Pts',(30.4861643333158,-30.3011710264298,177.927202263348));
#36162=CARTESIAN_POINT('Ctrl Pts',(32.6061007373232,-29.8067495272411,177.816072474128));
#36163=CARTESIAN_POINT('Ctrl Pts',(34.1713397746787,-31.3195632990606,177.704942684908));
#36164=CARTESIAN_POINT('Ctrl Pts',(33.7493924649911,-33.4551072155036,177.593812895689));
#36165=CARTESIAN_POINT('Ctrl Pts',(31.7264200113143,-34.2589518772617,177.482683106469));
#36166=CARTESIAN_POINT('Ctrl Pts',(29.953825060967,-32.9954287257072,177.371553317249));
#36167=CARTESIAN_POINT('Ctrl Pts',(30.0538671932836,-30.8208997796038,177.26042352803));
#36168=CARTESIAN_POINT('Ctrl Pts',(31.9349889809426,-29.7254706763283,177.14929373881));
#36169=CARTESIAN_POINT('Ctrl Pts',(33.8756081405823,-30.7116660908249,177.03816394959));
#36170=CARTESIAN_POINT('Ctrl Pts',(34.0996910738393,-32.8769307536337,176.92703416037));
#36171=CARTESIAN_POINT('Ctrl Pts',(32.402159504676,-34.2396378878484,176.815904371151));
#36172=CARTESIAN_POINT('Ctrl Pts',(30.3365759189771,-33.5526527212457,176.704774581931));
#36173=CARTESIAN_POINT('Ctrl Pts',(29.7933400127026,-31.4446966188922,176.593644792711));
#36174=CARTESIAN_POINT('Ctrl Pts',(31.26961539679,-29.844948150429,176.482515003491));
#36175=CARTESIAN_POINT('Ctrl Pts',(33.4143308489367,-30.2174797633851,176.371385214272));
#36176=CARTESIAN_POINT('Ctrl Pts',(34.2646660459687,-32.2213545666294,176.260255425052));
#36177=CARTESIAN_POINT('Ctrl Pts',(33.0424034369847,-34.0226480708054,176.149125635832));
#36178=CARTESIAN_POINT('Ctrl Pts',(30.8661445068797,-33.9728359953733,176.037995846613));
#36179=CARTESIAN_POINT('Ctrl Pts',(29.7275778279212,-32.1175058114478,175.926866057393));
#36180=CARTESIAN_POINT('Ctrl Pts',(30.6687072774601,-30.1546355832039,175.815736268173));
#36181=CARTESIAN_POINT('Ctrl Pts',(32.8282213893975,-29.8806228570576,175.704606478953));
#36182=CARTESIAN_POINT('Ctrl Pts',(34.229756267446,-31.5462411084492,175.593476689734));
#36183=CARTESIAN_POINT('Ctrl Pts',(33.5906423902274,-33.6271345765753,175.482346900514));
#36184=CARTESIAN_POINT('Ctrl Pts',(31.4957898472712,-34.2188921257606,175.371217111294));
#36185=CARTESIAN_POINT('Ctrl Pts',(29.8623849681609,-32.7799436643323,175.260087322075));
#36186=CARTESIAN_POINT('Ctrl Pts',(30.1853021847201,-30.6271992194443,175.148957532855));
#36187=CARTESIAN_POINT('Ctrl Pts',(32.169011162245,-29.730827161516,175.037827743635));
#36188=CARTESIAN_POINT('Ctrl Pts',(33.9980429569331,-30.9111774772138,174.926697954415));
#36189=CARTESIAN_POINT('Ctrl Pts',(33.9984875053096,-33.0880063579768,174.815568165196));
#36190=CARTESIAN_POINT('Ctrl Pts',(32.1699379615213,-34.2691036188572,174.704438375976));
#36191=CARTESIAN_POINT('Ctrl Pts',(30.1858630382491,-33.3735418551635,174.593308586756));
#36192=CARTESIAN_POINT('Ctrl Pts',(29.8620665888753,-31.2209294810654,174.482178797537));
#36193=CARTESIAN_POINT('Ctrl Pts',(31.4948836124403,-29.7813139972282,174.371049008317));
#36194=CARTESIAN_POINT('Ctrl Pts',(33.5899776761409,-30.3722158824801,174.259919219097));
#36195=CARTESIAN_POINT('Ctrl Pts',(34.2299414132272,-32.4528481395024,174.148789429877));
#36196=CARTESIAN_POINT('Ctrl Pts',(32.8290869516356,-34.1190386901857,174.037659640658));
#36197=CARTESIAN_POINT('Ctrl Pts',(30.6694611029807,-33.8459080116287,173.926529851438));
#36198=CARTESIAN_POINT('Ctrl Pts',(29.7275300237844,-31.883422338868,173.815400062218));
#36199=CARTESIAN_POINT('Ctrl Pts',(30.8653388229099,-30.0276272773431,173.704270272998));
#36200=CARTESIAN_POINT('Ctrl Pts',(33.0415772264202,-29.9769263421023,173.593140483779));
#36201=CARTESIAN_POINT('Ctrl Pts',(34.2645754477454,-31.7777204792493,173.482010694559));
#36202=CARTESIAN_POINT('Ctrl Pts',(33.4150587775922,-33.7819424232662,173.370880905339));
#36203=CARTESIAN_POINT('Ctrl Pts',(31.27049565986,-34.1553499858709,173.259751116119));
#36204=CARTESIAN_POINT('Ctrl Pts',(29.7935670030788,-32.5562046152037,173.1486213269));
#36205=CARTESIAN_POINT('Ctrl Pts',(30.3359418973104,-30.4480268124901,173.03749153768));
#36206=CARTESIAN_POINT('Ctrl Pts',(32.4012447211648,-29.7601980405371,172.92636174846));
#36207=CARTESIAN_POINT('Ctrl Pts',(34.099332727527,-31.1222117322437,172.81523195924));
#36208=CARTESIAN_POINT('Ctrl Pts',(33.8761341879719,-33.2875677273836,172.704102170021));
#36209=CARTESIAN_POINT('Ctrl Pts',(31.935917985413,-34.2745557015125,172.592972380801));
#36210=CARTESIAN_POINT('Ctrl Pts',(30.0543489476635,-33.1798949641467,172.481842591581));
#36211=CARTESIAN_POINT('Ctrl Pts',(29.9534186533055,-31.0054071510219,172.370712802362));
#36212=CARTESIAN_POINT('Ctrl Pts',(31.7254974131916,-29.7411599273715,172.259583013142));
#36213=CARTESIAN_POINT('Ctrl Pts',(33.7487979636683,-30.5441786420902,172.148453223922));
#36214=CARTESIAN_POINT('Ctrl Pts',(34.1716175827199,-32.6795492758427,172.037323434702));
#36215=CARTESIAN_POINT('Ctrl Pts',(32.6069963402783,-34.193003781749,171.926193645483));
#36216=CARTESIAN_POINT('Ctrl Pts',(30.4868586298152,-33.6994450087343,171.815063856263));
#36217=CARTESIAN_POINT('Ctrl Pts',(29.7515314920104,-31.6505725934397,171.703934067043));
#36218=CARTESIAN_POINT('Ctrl Pts',(31.073978349092,-29.9214923512466,171.592804277824));
#36219=CARTESIAN_POINT('Ctrl Pts',(33.243910178798,-30.0946397687158,171.481674488604));
#36220=CARTESIAN_POINT('Ctrl Pts',(34.2754289025122,-32.011552207085,171.370544699384));
#36221=CARTESIAN_POINT('Ctrl Pts',(33.2244997706462,-33.9178921908084,171.259414910164));
#36222=CARTESIAN_POINT('Ctrl Pts',(31.0529217278318,-34.0689980401788,171.148285120945));
#36223=CARTESIAN_POINT('Ctrl Pts',(29.7480994490696,-32.3265793205269,171.037155331725));
#36224=CARTESIAN_POINT('Ctrl Pts',(30.5041921336743,-30.2852787483341,170.926025542505));
#36225=CARTESIAN_POINT('Ctrl Pts',(32.6292319561795,-29.8132724702883,170.814895753285));
#36226=CARTESIAN_POINT('Ctrl Pts',(34.1784055161256,-31.3425355133621,170.703765964066));
#36227=CARTESIAN_POINT('Ctrl Pts',(33.7339259715377,-33.4735029247014,170.592636174846));
#36228=CARTESIAN_POINT('Ctrl Pts',(31.7025761814426,-34.2559364388279,170.481506385626));
#36229=CARTESIAN_POINT('Ctrl Pts',(29.9434254446643,-32.973761388751,170.370376596406));
#36230=CARTESIAN_POINT('Ctrl Pts',(30.0664294383068,-30.8004104756918,170.259246807187));
#36231=CARTESIAN_POINT('Ctrl Pts',(31.9590162413113,-29.7249108862727,170.148117017967));
#36232=CARTESIAN_POINT('Ctrl Pts',(33.8891109358174,-30.7315481814228,170.036987228747));
#36233=CARTESIAN_POINT('Ctrl Pts',(34.0903117884183,-32.8990588251476,169.925857439528));
#36234=CARTESIAN_POINT('Ctrl Pts',(32.3784819607464,-34.2437605819842,169.814727650308));
#36235=CARTESIAN_POINT('Ctrl Pts',(30.320269547065,-33.5349969867593,169.703597861088));
#36236=CARTESIAN_POINT('Ctrl Pts',(29.7993282279921,-31.4214207956012,169.592468071869));
#36237=CARTESIAN_POINT('Ctrl Pts',(31.292417849368,-29.8373540178792,169.481338282649));
#36238=CARTESIAN_POINT('Ctrl Pts',(33.4330789815959,-30.2325173900741,169.370208493429));
#36239=CARTESIAN_POINT('Ctrl Pts',(34.2622017709567,-32.2452616793244,169.259078704209));
#36240=CARTESIAN_POINT('Ctrl Pts',(33.0209820321044,-34.0335451394052,169.14794891499));
#36241=CARTESIAN_POINT('Ctrl Pts',(30.8453706095393,-33.9607501407891,169.03681912577));
#36242=CARTESIAN_POINT('Ctrl Pts',(29.7264634837301,-32.0934978767565,168.92568933655));
#36243=CARTESIAN_POINT('Ctrl Pts',(30.6882723220514,-30.1406773698913,168.814559547331));
#36244=CARTESIAN_POINT('Ctrl Pts',(32.8505601063057,-29.8894887705209,168.703429758111));
#36245=CARTESIAN_POINT('Ctrl Pts',(34.2344245048656,-31.5698171609635,168.592299968891));
#36246=CARTESIAN_POINT('Ctrl Pts',(33.573367828597,-33.6438442202791,168.481170179671));
#36247=CARTESIAN_POINT('Ctrl Pts',(31.4723819766352,-34.2134428765023,168.370040390451));
#36248=CARTESIAN_POINT('Ctrl Pts',(29.8542664207788,-32.7573226148014,168.258910601232));
#36249=CARTESIAN_POINT('Ctrl Pts',(30.1999029612069,-30.6081089111724,168.147780812012));
#36250=CARTESIAN_POINT('Ctrl Pts',(32.1929688023261,-29.7327388328916,168.036651022792));
#36251=CARTESIAN_POINT('Ctrl Pts',(34.0094316637276,-30.932341596928,167.925521233573));
#36252=CARTESIAN_POINT('Ctrl Pts',(33.9868845077251,-33.1090537336298,167.814391444353));
#36253=CARTESIAN_POINT('Ctrl Pts',(32.1459620955973,-34.2707719603118,167.703261655133));
#36254=CARTESIAN_POINT('Ctrl Pts',(30.1714569631769,-33.3543042333534,167.592131865913));
#36255=CARTESIAN_POINT('Ctrl Pts',(29.8704141674635,-31.1983921238923,167.481002076694));
#36256=CARTESIAN_POINT('Ctrl Pts',(31.5183460882199,-29.776102513524,167.369872287474));
#36257=CARTESIAN_POINT('Ctrl Pts',(33.6070807009338,-30.3891004498334,167.258742498254));
#36258=CARTESIAN_POINT('Ctrl Pts',(34.2250360367554,-32.4763747918462,167.147612709035));
#36259=CARTESIAN_POINT('Ctrl Pts',(32.8066552879638,-34.1276789269702,167.036482919815));
#36260=CARTESIAN_POINT('Ctrl Pts',(30.6500470950584,-33.8317486063998,166.925353130595));
#36261=CARTESIAN_POINT('Ctrl Pts',(29.7288711743741,-31.85943358507,166.814223341375));
#36262=CARTESIAN_POINT('Ctrl Pts',(30.8862687812559,-30.0157394792471,166.703093552156));
#36263=CARTESIAN_POINT('Ctrl Pts',(33.0628168066279,-29.9880678339112,166.591963762936));
#36264=CARTESIAN_POINT('Ctrl Pts',(34.2669395338498,-31.8015954273855,166.480833973716));
#36265=CARTESIAN_POINT('Ctrl Pts',(33.395868395384,-33.7969028631354,166.369704184497));
#36266=CARTESIAN_POINT('Ctrl Pts',(31.248363254292,-34.1472925131801,166.258574395277));
#36267=CARTESIAN_POINT('Ctrl Pts',(29.786605960109,-32.5333489778486,166.147444606057));
#36268=CARTESIAN_POINT('Ctrl Pts',(30.3549344083866,-30.4295428224182,166.036314816837));
#36269=CARTESIAN_POINT('Ctrl Pts',(31.7306127536046,-29.9891675732324,165.962228290691));
#36270=CARTESIAN_POINT('Ctrl Pts',(32.3594718785484,-30.1086918117405,165.925185027618));
#36271=CARTESIAN_POINT('Ctrl Pts',(33.5652001142722,-30.6687801966684,179.224444917147));
#36272=CARTESIAN_POINT('Ctrl Pts',(34.0078301022497,-31.1892085331676,179.187401654074));
#36273=CARTESIAN_POINT('Ctrl Pts',(34.3249209220215,-32.6979173761351,179.113315127928));
#36274=CARTESIAN_POINT('Ctrl Pts',(32.6727317243372,-34.3350173650632,179.002185338708));
#36275=CARTESIAN_POINT('Ctrl Pts',(30.4041599371754,-33.8301198258457,178.891055549488));
#36276=CARTESIAN_POINT('Ctrl Pts',(29.5964289625556,-31.6527499346609,178.779925760269));
#36277=CARTESIAN_POINT('Ctrl Pts',(30.988248508056,-29.7919884506806,178.668795971049));
#36278=CARTESIAN_POINT('Ctrl Pts',(33.3060963778469,-29.9525600136615,178.557666181829));
#36279=CARTESIAN_POINT('Ctrl Pts',(34.4285775821774,-31.9866392352977,178.446536392609));
#36280=CARTESIAN_POINT('Ctrl Pts',(33.3284712654795,-34.033087144352,178.33540660339));
#36281=CARTESIAN_POINT('Ctrl Pts',(31.0125524608971,-34.2188064667841,178.22427681417));
#36282=CARTESIAN_POINT('Ctrl Pts',(29.600339843317,-32.3739321987841,178.11314702495));
#36283=CARTESIAN_POINT('Ctrl Pts',(30.3842677675772,-30.186822526131,178.002017235731));
#36284=CARTESIAN_POINT('Ctrl Pts',(32.6468974928654,-29.6591214220926,177.890887446511));
#36285=CARTESIAN_POINT('Ctrl Pts',(34.3174930665853,-31.2737629757136,177.779757657291));
#36286=CARTESIAN_POINT('Ctrl Pts',(33.8671444034839,-33.5530507580587,177.668627868071));
#36287=CARTESIAN_POINT('Ctrl Pts',(31.7080052904067,-34.4110023564038,177.557498078852));
#36288=CARTESIAN_POINT('Ctrl Pts',(29.8160966378782,-33.0624312219618,177.446368289632));
#36289=CARTESIAN_POINT('Ctrl Pts',(29.9228726250884,-30.7415343202187,177.335238500412));
#36290=CARTESIAN_POINT('Ctrl Pts',(31.9306130769242,-29.5723716763149,177.224108711192));
#36291=CARTESIAN_POINT('Ctrl Pts',(34.0018556801289,-30.624948091138,177.112978921973));
#36292=CARTESIAN_POINT('Ctrl Pts',(34.2410216781083,-32.9359571289216,177.001849132753));
#36293=CARTESIAN_POINT('Ctrl Pts',(32.4292289371827,-34.3903883387013,176.890719343533));
#36294=CARTESIAN_POINT('Ctrl Pts',(30.2246105287083,-33.6571620702863,176.779589554314));
#36295=CARTESIAN_POINT('Ctrl Pts',(29.6448093105881,-31.4073190430277,176.668459765094));
#36296=CARTESIAN_POINT('Ctrl Pts',(31.2204530706714,-29.6998912018496,176.557329975874));
#36297=CARTESIAN_POINT('Ctrl Pts',(33.5095297265273,-30.0974979883034,176.446200186654));
#36298=CARTESIAN_POINT('Ctrl Pts',(34.4171011468898,-32.2362539844767,176.335070397435));
#36299=CARTESIAN_POINT('Ctrl Pts',(33.1125678099616,-34.1587928959332,176.223940608215));
#36300=CARTESIAN_POINT('Ctrl Pts',(30.7898244786656,-34.1056279602598,176.112810818995));
#36301=CARTESIAN_POINT('Ctrl Pts',(29.5746206606811,-32.1254151498947,176.001681029775));
#36302=CARTESIAN_POINT('Ctrl Pts',(30.5790977119008,-30.0304237544394,175.890551240556));
#36303=CARTESIAN_POINT('Ctrl Pts',(32.8839691281437,-29.737967179745,175.779421451336));
#36304=CARTESIAN_POINT('Ctrl Pts',(34.3798415845562,-31.515698511429,175.668291662116));
#36305=CARTESIAN_POINT('Ctrl Pts',(33.6977088310898,-33.7366573134195,175.557161872896));
#36306=CARTESIAN_POINT('Ctrl Pts',(31.4618513662959,-34.3682461754341,175.446032083677));
#36307=CARTESIAN_POINT('Ctrl Pts',(29.7185016950889,-32.8324418202512,175.334902294457));
#36308=CARTESIAN_POINT('Ctrl Pts',(30.0631545307178,-30.5347957386302,175.223772505237));
#36309=CARTESIAN_POINT('Ctrl Pts',(32.1803873356192,-29.5780887075362,175.112642716017));
#36310=CARTESIAN_POINT('Ctrl Pts',(34.1325316071812,-30.8378886267708,175.001512926798));
#36311=CARTESIAN_POINT('Ctrl Pts',(34.1330060781932,-33.1612402722117,174.890383137578));
#36312=CARTESIAN_POINT('Ctrl Pts',(32.1813765179305,-34.4218374136508,174.779253348358));
#36313=CARTESIAN_POINT('Ctrl Pts',(30.0637531354043,-33.4659952178498,174.668123559139));
#36314=CARTESIAN_POINT('Ctrl Pts',(29.7181618856332,-31.1684900967289,174.556993769919));
#36315=CARTESIAN_POINT('Ctrl Pts',(31.4608841326267,-29.6319738217322,174.445863980699));
#36316=CARTESIAN_POINT('Ctrl Pts',(33.6969993749721,-30.2626494249117,174.33473419148));
#36317=CARTESIAN_POINT('Ctrl Pts',(34.380039192535,-32.4833294336296,174.22360440226));
#36318=CARTESIAN_POINT('Ctrl Pts',(32.8848929515401,-34.2616715861791,174.11247461304));
#36319=CARTESIAN_POINT('Ctrl Pts',(30.5799022775602,-33.9701564298645,174.00134482382));
#36320=CARTESIAN_POINT('Ctrl Pts',(29.5745696388387,-31.8755754743948,173.890215034601));
#36321=CARTESIAN_POINT('Ctrl Pts',(30.788964563955,-29.8948664954311,173.779085245381));
#36322=CARTESIAN_POINT('Ctrl Pts',(33.1116859870073,-29.8407528706267,173.667955456161));
#36323=CARTESIAN_POINT('Ctrl Pts',(34.417004450483,-31.7627588025647,173.556825666941));
#36324=CARTESIAN_POINT('Ctrl Pts',(33.5103066521985,-33.9018853056218,173.445695877722));
#36325=CARTESIAN_POINT('Ctrl Pts',(31.2213925844155,-34.3004270020612,173.334566088502));
#36326=CARTESIAN_POINT('Ctrl Pts',(29.6450515797297,-32.5936428533062,173.223436299282));
#36327=CARTESIAN_POINT('Ctrl Pts',(30.223933830923,-30.343563202994,173.112306510062));
#36328=CARTESIAN_POINT('Ctrl Pts',(32.4282525794201,-29.6094365459927,173.001176720843));
#36329=CARTESIAN_POINT('Ctrl Pts',(34.2406392114377,-31.0631276375177,172.890046931623));
#36330=CARTESIAN_POINT('Ctrl Pts',(34.002417135868,-33.3742341552288,172.778917142403));
#36331=CARTESIAN_POINT('Ctrl Pts',(31.9316046128615,-34.4276564770234,172.667787353183));
#36332=CARTESIAN_POINT('Ctrl Pts',(29.9233868064471,-33.2593139178844,172.556657563964));
#36333=CARTESIAN_POINT('Ctrl Pts',(29.8156628748399,-30.9384609177883,172.445527774744));
#36334=CARTESIAN_POINT('Ctrl Pts',(31.7070205920295,-29.5891169738205,172.334397985525));
#36335=CARTESIAN_POINT('Ctrl Pts',(33.8665098861644,-30.4461870304743,172.223268196305));
#36336=CARTESIAN_POINT('Ctrl Pts',(34.3177895739383,-32.7252898664381,172.112138407085));
#36337=CARTESIAN_POINT('Ctrl Pts',(32.6478533790253,-34.3406152820788,172.001008617865));
#36338=CARTESIAN_POINT('Ctrl Pts',(30.3850087973056,-33.8138349744767,171.889878828646));
#36339=CARTESIAN_POINT('Ctrl Pts',(29.6001866504415,-31.6270525684548,171.778749039426));
#36340=CARTESIAN_POINT('Ctrl Pts',(31.0116476562013,-29.7815876073365,171.667619250206));
#36341=CARTESIAN_POINT('Ctrl Pts',(33.3276380087708,-29.9663896103033,171.556489460986));
#36342=CARTESIAN_POINT('Ctrl Pts',(34.4285884533479,-32.0123297883341,171.445359671767));
#36343=CARTESIAN_POINT('Ctrl Pts',(33.3069210823662,-34.0469858777925,171.334229882547));
#36344=CARTESIAN_POINT('Ctrl Pts',(30.9891737097718,-34.2082626905328,171.223100093327));
#36345=CARTESIAN_POINT('Ctrl Pts',(29.5965235960397,-32.348561436509,171.111970304107));
#36346=CARTESIAN_POINT('Ctrl Pts',(30.4035090225958,-30.1698605357837,171.000840514888));
#36347=CARTESIAN_POINT('Ctrl Pts',(32.6715856784485,-29.666083425673,170.889710725668));
#36348=CARTESIAN_POINT('Ctrl Pts',(34.3250344044286,-31.2982814541151,170.778580936448));
#36349=CARTESIAN_POINT('Ctrl Pts',(33.8506368574238,-33.5726846859303,170.667451147228));
#36350=CARTESIAN_POINT('Ctrl Pts',(31.6825565278258,-34.4077839482373,170.556321358009));
#36351=CARTESIAN_POINT('Ctrl Pts',(29.8049970214305,-33.0393054524471,170.445191568789));
#36352=CARTESIAN_POINT('Ctrl Pts',(29.9362804372059,-30.7196658773756,170.334061779569));
#36353=CARTESIAN_POINT('Ctrl Pts',(31.9562576167437,-29.5717742066846,170.22293199035));
#36354=CARTESIAN_POINT('Ctrl Pts',(34.0162673510713,-30.6461684490236,170.11180220113));
#36355=CARTESIAN_POINT('Ctrl Pts',(34.2310110712073,-32.9595746451244,170.00067241191));
#36356=CARTESIAN_POINT('Ctrl Pts',(32.4039576532821,-34.394788532161,169.88954262269));
#36357=CARTESIAN_POINT('Ctrl Pts',(30.2072065718112,-33.6383179249642,169.778412833471));
#36358=CARTESIAN_POINT('Ctrl Pts',(29.6512005937841,-31.382476519658,169.667283044251));
#36359=CARTESIAN_POINT('Ctrl Pts',(31.2447903606557,-29.6917859067979,169.556153255031));
#36360=CARTESIAN_POINT('Ctrl Pts',(33.5295397995502,-30.113547800496,169.445023465812));
#36361=CARTESIAN_POINT('Ctrl Pts',(34.4144710010597,-32.2617702894598,169.333893676592));
#36362=CARTESIAN_POINT('Ctrl Pts',(33.0897045262574,-34.1704234482866,169.222763887372));
#36363=CARTESIAN_POINT('Ctrl Pts',(30.7676522863566,-34.092728604512,169.111634098152));
#36364=CARTESIAN_POINT('Ctrl Pts',(29.5734313097712,-32.0997912365677,169.000504308933));
#36365=CARTESIAN_POINT('Ctrl Pts',(30.599979683353,-30.0155260111423,168.889374519713));
#36366=CARTESIAN_POINT('Ctrl Pts',(32.9078114683222,-29.7474298595245,168.778244730493));
#36367=CARTESIAN_POINT('Ctrl Pts',(34.3848240419215,-31.5408614725078,168.667114941273));
#36368=CARTESIAN_POINT('Ctrl Pts',(33.679271515441,-33.7544916864091,168.555985152054));
#36369=CARTESIAN_POINT('Ctrl Pts',(31.4368679074494,-34.3624301361752,168.444855362834));
#36370=CARTESIAN_POINT('Ctrl Pts',(29.7098366867433,-32.8082981435875,168.333725573614));
#36371=CARTESIAN_POINT('Ctrl Pts',(30.0787380882382,-30.5144204580892,168.222595784395));
#36372=CARTESIAN_POINT('Ctrl Pts',(32.2059575689964,-29.5801290538745,168.111465995175));
#36373=CARTESIAN_POINT('Ctrl Pts',(34.1446868899892,-30.8604773073957,168.000336205955));
#36374=CARTESIAN_POINT('Ctrl Pts',(34.1206220806415,-33.1837043507103,167.889206416735));
#36375=CARTESIAN_POINT('Ctrl Pts',(32.1557868319255,-34.4236180514851,167.778076627515));
#36376=CARTESIAN_POINT('Ctrl Pts',(30.0483773846876,-33.4454627080684,167.666946838296));
#36377=CARTESIAN_POINT('Ctrl Pts',(29.7270713413188,-31.1444357457715,167.555817049076));
#36378=CARTESIAN_POINT('Ctrl Pts',(31.4859258720994,-29.6264115520718,167.444687259857));
#36379=CARTESIAN_POINT('Ctrl Pts',(33.7152536076064,-30.2806704956948,167.333557470637));
#36380=CARTESIAN_POINT('Ctrl Pts',(34.3748036342428,-32.5084396694031,167.222427681417));
#36381=CARTESIAN_POINT('Ctrl Pts',(32.8609514083336,-34.2708933989397,167.111297892197));
#36382=CARTESIAN_POINT('Ctrl Pts',(30.5591815090839,-33.9550439523851,167.000168102978));
#36383=CARTESIAN_POINT('Ctrl Pts',(29.5760010625288,-31.8499720330306,166.889038313758));
#36384=CARTESIAN_POINT('Ctrl Pts',(30.8113033217656,-29.8821785273914,166.777908524538));
#36385=CARTESIAN_POINT('Ctrl Pts',(33.1343552073857,-29.8526442983615,166.666778735318));
#36386=CARTESIAN_POINT('Ctrl Pts',(34.4195276636713,-31.7882407779865,166.555648946099));
#36387=CARTESIAN_POINT('Ctrl Pts',(33.4898245617256,-33.917852735535,166.444519156879));
#36388=CARTESIAN_POINT('Ctrl Pts',(31.1977704424326,-34.291827179356,166.333389367659));
#36389=CARTESIAN_POINT('Ctrl Pts',(29.6376219876378,-32.5692487986674,166.222259578439));
#36390=CARTESIAN_POINT('Ctrl Pts',(30.2442047315206,-30.3238350520459,166.11112978922));
#36391=CARTESIAN_POINT('Ctrl Pts',(31.7124802469756,-29.853818061345,166.037043263073));
#36392=CARTESIAN_POINT('Ctrl Pts',(32.3836679988472,-29.9813874990082,166.));
#36393=CARTESIAN_POINT('Ctrl Pts',(33.2690708798528,-30.920641346952,179.));
#36394=CARTESIAN_POINT('Ctrl Pts',(33.3143937870934,-30.9629228091432,179.));
#36395=CARTESIAN_POINT('Ctrl Pts',(33.3569863363192,-31.0077738608052,179.));
#36396=CARTESIAN_POINT('Ctrl Pts',(33.3968502559163,-31.0548493575027,179.));
#36397=CARTESIAN_POINT('Ctrl Pts',(33.4393504278583,-31.1050380174266,179.));
#36398=CARTESIAN_POINT('Ctrl Pts',(33.4787498660929,-31.1577552940212,179.));
#36399=CARTESIAN_POINT('Ctrl Pts',(33.515021814116,-31.2126376739653,179.));
#36400=CARTESIAN_POINT('Ctrl Pts',(33.5467597686362,-31.2606597564164,179.));
#36401=CARTESIAN_POINT('Ctrl Pts',(33.5761029944634,-31.3103407222917,179.));
#36402=CARTESIAN_POINT('Ctrl Pts',(33.6030106666263,-31.361464609715,179.));
#36403=CARTESIAN_POINT('Ctrl Pts',(33.6165048228579,-31.3871031606784,179.));
#36404=CARTESIAN_POINT('Ctrl Pts',(33.6293860750336,-31.4131049631121,179.));
#36405=CARTESIAN_POINT('Ctrl Pts',(33.641646934939,-31.4394446180088,179.));
#36406=CARTESIAN_POINT('Ctrl Pts',(33.6472617614843,-31.4515067893939,179.));
#36407=CARTESIAN_POINT('Ctrl Pts',(33.6527470722687,-31.4636415260275,179.));
#36408=CARTESIAN_POINT('Ctrl Pts',(33.658093608444,-31.4758263637454,179.));
#36409=CARTESIAN_POINT('Ctrl Pts',(33.6850051809481,-31.5371582490902,179.));
#36410=CARTESIAN_POINT('Ctrl Pts',(33.7084559555629,-31.5998656904031,179.));
#36411=CARTESIAN_POINT('Ctrl Pts',(33.7284227072741,-31.663590733636,179.));
#36412=CARTESIAN_POINT('Ctrl Pts',(33.7487447393774,-31.7284496747945,179.));
#36413=CARTESIAN_POINT('Ctrl Pts',(33.765458215908,-31.7943635951405,179.));
#36414=CARTESIAN_POINT('Ctrl Pts',(33.7784993315041,-31.8609916099304,179.));
#36415=CARTESIAN_POINT('Ctrl Pts',(33.7894070090125,-31.9167197332644,179.));
#36416=CARTESIAN_POINT('Ctrl Pts',(33.797745034606,-31.9729483616004,179.));
#36417=CARTESIAN_POINT('Ctrl Pts',(33.8034512516889,-32.029490320182,179.));
#36418=CARTESIAN_POINT('Ctrl Pts',(33.8060783951693,-32.0555222491633,179.));
#36419=CARTESIAN_POINT('Ctrl Pts',(33.8081473437298,-32.0816207072311,179.));
#36420=CARTESIAN_POINT('Ctrl Pts',(33.8096502328989,-32.1077678283934,179.));
#36421=CARTESIAN_POINT('Ctrl Pts',(33.8103081534512,-32.1192142668601,179.));
#36422=CARTESIAN_POINT('Ctrl Pts',(33.810857477492,-32.130669870472,179.));
#36423=CARTESIAN_POINT('Ctrl Pts',(33.8112972071105,-32.1421189247609,179.));
#36424=CARTESIAN_POINT('Ctrl Pts',(33.8139908004847,-32.2122508773816,179.));
#36425=CARTESIAN_POINT('Ctrl Pts',(33.8125842846173,-32.2822684969545,179.));
#36426=CARTESIAN_POINT('Ctrl Pts',(33.8070233187848,-32.3518106703801,179.));
#36427=CARTESIAN_POINT('Ctrl Pts',(33.802053136137,-32.4139648561934,179.));
#36428=CARTESIAN_POINT('Ctrl Pts',(33.7937639803061,-32.4757402141871,179.));
#36429=CARTESIAN_POINT('Ctrl Pts',(33.7820839574515,-32.5368910554573,179.));
#36430=CARTESIAN_POINT('Ctrl Pts',(33.7693542202861,-32.6035376833369,179.));
#36431=CARTESIAN_POINT('Ctrl Pts',(33.7525978242256,-32.6694433303306,179.));
#36432=CARTESIAN_POINT('Ctrl Pts',(33.7320598219069,-32.7343945881359,179.));
#36433=CARTESIAN_POINT('Ctrl Pts',(33.7241290562722,-32.7594755670618,179.));
#36434=CARTESIAN_POINT('Ctrl Pts',(33.7156338517038,-32.7844141873628,179.));
#36435=CARTESIAN_POINT('Ctrl Pts',(33.7065863065718,-32.8091978397264,179.));
#36436=CARTESIAN_POINT('Ctrl Pts',(33.7026186329799,-32.820066361691,179.));
#36437=CARTESIAN_POINT('Ctrl Pts',(33.698544834818,-32.8309045228361,179.));
#36438=CARTESIAN_POINT('Ctrl Pts',(33.6943710227137,-32.841698708458,179.));
#36439=CARTESIAN_POINT('Ctrl Pts',(33.6691495102391,-32.9069258151202,179.));
#36440=CARTESIAN_POINT('Ctrl Pts',(33.6402375808801,-32.9706664152282,179.));
#36441=CARTESIAN_POINT('Ctrl Pts',(33.6079477009133,-33.0327018841654,179.));
#36442=CARTESIAN_POINT('Ctrl Pts',(33.5749109983802,-33.096172152122,179.));
#36443=CARTESIAN_POINT('Ctrl Pts',(33.5383379809688,-33.1578583209809,179.));
#36444=CARTESIAN_POINT('Ctrl Pts',(33.498507171859,-33.2175225123557,179.));
#36445=CARTESIAN_POINT('Ctrl Pts',(33.4680143720159,-33.2631989192893,179.));
#36446=CARTESIAN_POINT('Ctrl Pts',(33.4356110327496,-33.3076903192047,179.));
#36447=CARTESIAN_POINT('Ctrl Pts',(33.4014025677393,-33.3508838705313,179.));
#36448=CARTESIAN_POINT('Ctrl Pts',(33.3801002535635,-33.3777813826077,179.));
#36449=CARTESIAN_POINT('Ctrl Pts',(33.3580976222504,-33.4041754908389,179.));
#36450=CARTESIAN_POINT('Ctrl Pts',(33.3354172175954,-33.4300372539183,179.));
#36451=CARTESIAN_POINT('Ctrl Pts',(33.3227588439286,-33.4444712054162,179.));
#36452=CARTESIAN_POINT('Ctrl Pts',(33.3098849003051,-33.4587438432578,179.));
#36453=CARTESIAN_POINT('Ctrl Pts',(33.2968229201931,-33.4728248058561,179.));
#36454=CARTESIAN_POINT('Ctrl Pts',(33.2459584485793,-33.527657282727,179.));
#36455=CARTESIAN_POINT('Ctrl Pts',(33.1921974637621,-33.5796446805326,179.));
#36456=CARTESIAN_POINT('Ctrl Pts',(33.1358246431769,-33.6285233175597,179.));
#36457=CARTESIAN_POINT('Ctrl Pts',(33.0936773563628,-33.6650675584275,179.));
#36458=CARTESIAN_POINT('Ctrl Pts',(33.0500689377864,-33.6998738513906,179.));
#36459=CARTESIAN_POINT('Ctrl Pts',(33.0051019841789,-33.7328222569625,179.));
#36460=CARTESIAN_POINT('Ctrl Pts',(32.9910181375986,-33.7431418417224,179.));
#36461=CARTESIAN_POINT('Ctrl Pts',(32.976800930029,-33.7532790962547,179.));
#36462=CARTESIAN_POINT('Ctrl Pts',(32.9624532710857,-33.7632301075464,179.));
#36463=CARTESIAN_POINT('Ctrl Pts',(32.9486742705369,-33.7727867181818,179.));
#36464=CARTESIAN_POINT('Ctrl Pts',(32.9347820152157,-33.7821665966601,179.));
#36465=CARTESIAN_POINT('Ctrl Pts',(32.9207844060457,-33.7913635692792,179.));
#36466=CARTESIAN_POINT('Ctrl Pts',(32.8578362168016,-33.8327229732939,179.));
#36467=CARTESIAN_POINT('Ctrl Pts',(32.7927300171995,-33.8704071115942,179.));
#36468=CARTESIAN_POINT('Ctrl Pts',(32.7257268190738,-33.9041370513948,179.));
#36469=CARTESIAN_POINT('Ctrl Pts',(32.6745421251937,-33.9299038310647,179.));
#36470=CARTESIAN_POINT('Ctrl Pts',(32.6222494359116,-33.9533626701466,179.));
#36471=CARTESIAN_POINT('Ctrl Pts',(32.5689512759831,-33.9743740101343,179.));
#36472=CARTESIAN_POINT('Ctrl Pts',(32.5564668663362,-33.9792956467535,179.));
#36473=CARTESIAN_POINT('Ctrl Pts',(32.5439272450406,-33.9840829288593,179.));
#36474=CARTESIAN_POINT('Ctrl Pts',(32.5313343692882,-33.9887364495513,179.));
#36475=CARTESIAN_POINT('Ctrl Pts',(30.3326674689016,-32.0013033567452,177.87148036339));
#36476=CARTESIAN_POINT('Ctrl Pts',(30.3319312465786,-32.0869545016077,177.877220944861));
#36477=CARTESIAN_POINT('Ctrl Pts',(30.3379613926568,-32.1725016619386,177.882961526332));
#36478=CARTESIAN_POINT('Ctrl Pts',(30.3511187262443,-32.2569381575126,177.888702107803));
#36479=CARTESIAN_POINT('Ctrl Pts',(30.4360213745041,-32.8017964326578,177.925745370876));
#36480=CARTESIAN_POINT('Ctrl Pts',(30.817697364428,-33.3004070552782,177.962788633949));
#36481=CARTESIAN_POINT('Ctrl Pts',(31.3214948214846,-33.524615364425,177.999831897022));
#36482=CARTESIAN_POINT('Ctrl Pts',(31.8252922785413,-33.7488236735718,178.036875160096));
#36483=CARTESIAN_POINT('Ctrl Pts',(32.4512112027306,-33.698629669245,178.073918423169));
#36484=CARTESIAN_POINT('Ctrl Pts',(32.9128324747469,-33.3969878954966,178.110961686242));
#36485=CARTESIAN_POINT('Ctrl Pts',(33.3744537467632,-33.0953461217483,178.148004949315));
#36486=CARTESIAN_POINT('Ctrl Pts',(33.6717773666064,-32.5422565785785,178.185048212389));
#36487=CARTESIAN_POINT('Ctrl Pts',(33.6687537576681,-31.9908384660968,178.222091475462));
#36488=CARTESIAN_POINT('Ctrl Pts',(33.6657301487298,-31.4394203536152,178.259134738535));
#36489=CARTESIAN_POINT('Ctrl Pts',(33.36235931101,-30.8896736718216,178.296178001608));
#36490=CARTESIAN_POINT('Ctrl Pts',(32.8974537476822,-30.5931016470682,178.333221264682));
#36491=CARTESIAN_POINT('Ctrl Pts',(32.4325481843545,-30.2965296223148,178.370264527755));
#36492=CARTESIAN_POINT('Ctrl Pts',(31.8061078954188,-30.2531322546016,178.407307790828));
#36493=CARTESIAN_POINT('Ctrl Pts',(31.3048055541871,-30.4828857857193,178.444351053901));
#36494=CARTESIAN_POINT('Ctrl Pts',(30.8035032129554,-30.7126393168371,178.481394316974));
#36495=CARTESIAN_POINT('Ctrl Pts',(30.4273388194276,-31.2155437467857,178.518437580048));
#36496=CARTESIAN_POINT('Ctrl Pts',(30.3484085717018,-31.7612327495861,178.555480843121));
#36497=CARTESIAN_POINT('Ctrl Pts',(30.3370448670893,-31.8397964031507,178.560814016544));
#36498=CARTESIAN_POINT('Ctrl Pts',(30.3318421685893,-31.9192468862352,178.566147189967));
#36499=CARTESIAN_POINT('Ctrl Pts',(30.3325025779359,-31.9987820654682,178.57148036339));
#36500=CARTESIAN_POINT('Ctrl Pts',(31.4698297828105,-33.9851743256715,179.));
#36501=CARTESIAN_POINT('Ctrl Pts',(30.8097602092464,-33.8088929660693,178.962956736927));
#36502=CARTESIAN_POINT('Ctrl Pts',(29.6908221036295,-32.748363474976,178.88887021078));
#36503=CARTESIAN_POINT('Ctrl Pts',(30.1185590192689,-30.4621264977465,178.777740421561));
#36504=CARTESIAN_POINT('Ctrl Pts',(32.2716026642884,-29.5870613462295,178.666610632341));
#36505=CARTESIAN_POINT('Ctrl Pts',(34.1744104601116,-30.9184848843002,178.555480843121));
#36506=CARTESIAN_POINT('Ctrl Pts',(34.0880400722661,-33.2405822108959,178.444351053901));
#36507=CARTESIAN_POINT('Ctrl Pts',(32.0903159787745,-34.4268786410256,178.333221264682));
#36508=CARTESIAN_POINT('Ctrl Pts',(30.0101331764293,-33.3923349810139,178.222091475462));
#36509=CARTESIAN_POINT('Ctrl Pts',(29.750957902677,-31.0834368587032,178.110961686242));
#36510=CARTESIAN_POINT('Ctrl Pts',(31.5501292172184,-29.6134187564108,177.999831897022));
#36511=CARTESIAN_POINT('Ctrl Pts',(33.7609939876075,-30.3275486926383,177.888702107803));
#36512=CARTESIAN_POINT('Ctrl Pts',(34.3602276546561,-32.5723003233786,177.777572318583));
#36513=CARTESIAN_POINT('Ctrl Pts',(32.7994009204969,-34.2932828161059,177.666442529363));
#36514=CARTESIAN_POINT('Ctrl Pts',(30.506973906968,-33.9154807357568,177.555312740144));
#36515=CARTESIAN_POINT('Ctrl Pts',(29.580946820041,-31.7846499895867,177.444182950924));
#36516=CARTESIAN_POINT('Ctrl Pts',(30.8688116391535,-29.8509059591332,177.333053161704));
#36517=CARTESIAN_POINT('Ctrl Pts',(33.1919274501366,-29.8839891344978,177.221923372484));
#36518=CARTESIAN_POINT('Ctrl Pts',(34.4242043461506,-31.8536226808824,177.110793583265));
#36519=CARTESIAN_POINT('Ctrl Pts',(33.4378756346499,-33.9572190768126,176.999663794045));
#36520=CARTESIAN_POINT('Ctrl Pts',(31.1356187743909,-34.2695898408057,176.888534004825));
#36521=CARTESIAN_POINT('Ctrl Pts',(29.6244342188476,-32.5048565745377,176.777404215605));
#36522=CARTESIAN_POINT('Ctrl Pts',(30.2873417136773,-30.2780840563291,176.666274426386));
#36523=CARTESIAN_POINT('Ctrl Pts',(32.5176554945262,-29.6271903313891,176.555144637166));
#36524=CARTESIAN_POINT('Ctrl Pts',(34.2742165827931,-31.1478662855577,176.444014847946));
#36525=CARTESIAN_POINT('Ctrl Pts',(33.9494393162254,-33.4484057729775,176.332885058727));
#36526=CARTESIAN_POINT('Ctrl Pts',(31.8405563287846,-34.4233800048647,176.221755269507));
#36527=CARTESIAN_POINT('Ctrl Pts',(29.8775944598767,-33.1805031364718,176.110625480287));
#36528=CARTESIAN_POINT('Ctrl Pts',(29.857035124892,-30.8572425997456,175.999495691067));
#36529=CARTESIAN_POINT('Ctrl Pts',(31.797694004055,-29.5798212429744,175.888365901848));
#36530=CARTESIAN_POINT('Ctrl Pts',(33.9235011368215,-30.5173212389216,175.777236112628));
#36531=CARTESIAN_POINT('Ctrl Pts',(34.2889408886545,-32.8117527580092,175.666106323408));
#36532=CARTESIAN_POINT('Ctrl Pts',(32.5595667617289,-34.3632769560673,175.554976534188));
#36533=CARTESIAN_POINT('Ctrl Pts',(30.3180832027141,-33.7519557125998,175.443846744969));
#36534=CARTESIAN_POINT('Ctrl Pts',(29.615871656949,-31.5372636001316,175.332716955749));
#36535=CARTESIAN_POINT('Ctrl Pts',(31.095588515948,-29.7460628226547,175.221587166529));
#36536=CARTESIAN_POINT('Ctrl Pts',(33.4030129572177,-30.0176409069538,175.110457377309));
#36537=CARTESIAN_POINT('Ctrl Pts',(34.4264151550835,-32.1034525354194,174.99932758809));
#36538=CARTESIAN_POINT('Ctrl Pts',(33.2291885163936,-34.0945855253653,174.88819779887));
#36539=CARTESIAN_POINT('Ctrl Pts',(30.9070218774947,-34.168776557331,174.777068009651));
#36540=CARTESIAN_POINT('Ctrl Pts',(29.5851369634584,-32.2581268034298,174.665938220431));
#36541=CARTESIAN_POINT('Ctrl Pts',(30.4733085123659,-30.1112421982983,174.554808431211));
#36542=CARTESIAN_POINT('Ctrl Pts',(32.7586915544763,-29.6929282505587,174.443678641991));
#36543=CARTESIAN_POINT('Ctrl Pts',(34.3497283135974,-31.3860213487566,174.332548852772));
#36544=CARTESIAN_POINT('Ctrl Pts',(33.7903192018566,-33.6410210502512,174.221419063552));
#36545=CARTESIAN_POINT('Ctrl Pts',(31.5924293717799,-34.3941760826881,174.110289274332));
#36546=CARTESIAN_POINT('Ctrl Pts',(29.7675437607309,-32.9562071280074,173.999159485112));
#36547=CARTESIAN_POINT('Ctrl Pts',(29.9857778898812,-30.6431277794088,173.888029695893));
#36548=CARTESIAN_POINT('Ctrl Pts',(32.0474062508829,-29.5718431724288,173.776899906673));
#36549=CARTESIAN_POINT('Ctrl Pts',(34.0656489251761,-30.7227813617776,173.665770117453));
#36550=CARTESIAN_POINT('Ctrl Pts',(34.1934321041778,-33.0426161979683,173.554640328233));
#36551=CARTESIAN_POINT('Ctrl Pts',(32.3138100082167,-34.4082599964802,173.443510539014));
#36552=CARTESIAN_POINT('Ctrl Pts',(30.1469923958635,-33.5698903627056,173.332380749794));
#36553=CARTESIAN_POINT('Ctrl Pts',(29.6760272477853,-31.2947740937349,173.221250960574));
#36554=CARTESIAN_POINT('Ctrl Pts',(31.331936760099,-29.6650729263216,173.110121171355));
#36555=CARTESIAN_POINT('Ctrl Pts',(33.5992505047259,-30.1722716955089,172.998991382135));
#36556=CARTESIAN_POINT('Ctrl Pts',(34.4029475305773,-32.3521875880785,172.887861592915));
#36557=CARTESIAN_POINT('Ctrl Pts',(33.0074930353251,-34.2097852193539,172.776731803695));
#36558=CARTESIAN_POINT('Ctrl Pts',(30.6899918399505,-34.0450113819995,172.665602014476));
#36559=CARTESIAN_POINT('Ctrl Pts',(29.5713959062062,-32.0086653050641,172.554472225256));
#36560=CARTESIAN_POINT('Ctrl Pts',(30.6754321019873,-29.9643888349053,172.443342436036));
#36561=CARTESIAN_POINT('Ctrl Pts',(32.9916984736889,-29.7830816277574,172.332212646816));
#36562=CARTESIAN_POINT('Ctrl Pts',(34.4003731567925,-31.6306740734072,172.221082857597));
#36563=CARTESIAN_POINT('Ctrl Pts',(33.6122523577626,-33.8162696019019,172.109953068377));
#36564=CARTESIAN_POINT('Ctrl Pts',(31.3486156850571,-34.3396348873596,171.998823279157));
#36565=CARTESIAN_POINT('Ctrl Pts',(29.6811188734186,-32.7217916961897,171.887693489937));
#36566=CARTESIAN_POINT('Ctrl Pts',(30.1358369216088,-30.4433725721719,171.776563700718));
#36567=CARTESIAN_POINT('Ctrl Pts',(32.2966168031358,-29.589561989181,171.665433911498));
#36568=CARTESIAN_POINT('Ctrl Pts',(34.1859362031082,-30.9417581335798,171.554304122278));
#36569=CARTESIAN_POINT('Ctrl Pts',(34.0747104954871,-33.2624457579713,171.443174333059));
#36570=CARTESIAN_POINT('Ctrl Pts',(32.0647322416946,-34.4277567153216,171.332044543839));
#36571=CARTESIAN_POINT('Ctrl Pts',(29.9955117422951,-33.3712110547348,171.220914754619));
#36572=CARTESIAN_POINT('Ctrl Pts',(29.7607771585773,-31.0597479070194,171.1097849654));
#36573=CARTESIAN_POINT('Ctrl Pts',(31.5753550359689,-29.6087932781905,170.99865517618));
#36574=CARTESIAN_POINT('Ctrl Pts',(33.778563379359,-30.3462451096045,170.88752538696));
#36575=CARTESIAN_POINT('Ctrl Pts',(34.3540498056764,-32.5971954824835,170.77639559774));
#36576=CARTESIAN_POINT('Ctrl Pts',(32.7751353784459,-34.3015990261089,170.665265808521));
#36577=CARTESIAN_POINT('Ctrl Pts',(30.4868254588548,-33.8996041008415,170.554136019301));
#36578=CARTESIAN_POINT('Ctrl Pts',(29.5833564696252,-31.7591121028326,170.443006230081));
#36579=CARTESIAN_POINT('Ctrl Pts',(30.8915734319869,-29.8390780959909,170.331876440861));
#36580=CARTESIAN_POINT('Ctrl Pts',(33.2142103690085,-29.896696381476,170.220746651642));
#36581=CARTESIAN_POINT('Ctrl Pts',(34.4256151438767,-31.8792353292564,170.109616862422));
#36582=CARTESIAN_POINT('Ctrl Pts',(33.4171232437699,-33.9722967940629,169.998487073202));
#36583=CARTESIAN_POINT('Ctrl Pts',(31.1116955190265,-34.2603336216113,169.887357283983));
#36584=CARTESIAN_POINT('Ctrl Pts',(29.6192344220091,-32.4797376309583,169.776227494763));
#36585=CARTESIAN_POINT('Ctrl Pts',(30.3056241636414,-30.2600909629904,169.665097705543));
#36586=CARTESIAN_POINT('Ctrl Pts',(32.5426882959684,-29.6327901771656,169.553967916323));
#36587=CARTESIAN_POINT('Ctrl Pts',(34.2830899850343,-31.1719341498779,169.442838127104));
#36588=CARTESIAN_POINT('Ctrl Pts',(33.9340324788774,-33.4689150086206,169.331708337884));
#36589=CARTESIAN_POINT('Ctrl Pts',(31.8149694217593,-34.4215607811959,169.220578548664));
#36590=CARTESIAN_POINT('Ctrl Pts',(29.8652443432771,-33.1580203875493,169.109448759444));
#36591=CARTESIAN_POINT('Ctrl Pts',(29.8692244913603,-30.8346722934351,168.998318970224));
#36592=CARTESIAN_POINT('Ctrl Pts',(31.8232672776651,-29.5778194788973,168.887189181005));
#36593=CARTESIAN_POINT('Ctrl Pts',(33.9390539348382,-30.5377200098576,168.776059391785));
#36594=CARTESIAN_POINT('Ctrl Pts',(34.2802394590648,-32.8358833299508,168.664929602565));
#36595=CARTESIAN_POINT('Ctrl Pts',(32.5345745584143,-34.3690552914116,168.553799813346));
#36596=CARTESIAN_POINT('Ctrl Pts',(30.299672819343,-33.7340935411791,168.442670024126));
#36597=CARTESIAN_POINT('Ctrl Pts',(29.62089207628,-31.5121081881889,168.331540234906));
#36598=CARTESIAN_POINT('Ctrl Pts',(31.1194451055679,-29.7366361290419,168.220410445686));
#36599=CARTESIAN_POINT('Ctrl Pts',(33.42387242316,-30.0325701422052,168.109280656467));
#36600=CARTESIAN_POINT('Ctrl Pts',(34.4251871441161,-32.1290746196978,167.998150867247));
#36601=CARTESIAN_POINT('Ctrl Pts',(33.2069968831276,-34.107451416473,167.887021078027));
#36602=CARTESIAN_POINT('Ctrl Pts',(30.8841761797311,-34.1571115078919,167.775891288808));
#36603=CARTESIAN_POINT('Ctrl Pts',(29.5825453040883,-32.2326065877438,167.664761499588));
#36604=CARTESIAN_POINT('Ctrl Pts',(30.4933428149864,-30.0952225441907,167.553631710368));
#36605=CARTESIAN_POINT('Ctrl Pts',(32.7830165101667,-29.7010703688433,167.442501921148));
#36606=CARTESIAN_POINT('Ctrl Pts',(34.3560822562997,-31.4108732598121,167.331372131929));
#36607=CARTESIAN_POINT('Ctrl Pts',(33.7728865232597,-33.6598393714977,167.220242342709));
#36608=CARTESIAN_POINT('Ctrl Pts',(31.567165387668,-34.3897368274991,167.10911255349));
#36609=CARTESIAN_POINT('Ctrl Pts',(29.7575675205768,-32.9325764403901,166.997982764269));
#36610=CARTESIAN_POINT('Ctrl Pts',(30.0002241716332,-30.6219253154616,166.88685297505));
#36611=CARTESIAN_POINT('Ctrl Pts',(32.0730445458741,-29.572487230153,166.77572318583));
#36612=CARTESIAN_POINT('Ctrl Pts',(34.0790345383106,-30.7446539377421,166.66459339661));
#36613=CARTESIAN_POINT('Ctrl Pts',(34.1822755906712,-33.0657579093129,166.55346360739));
#36614=CARTESIAN_POINT('Ctrl Pts',(32.2884012423449,-34.4113733924264,166.442333818171));
#36615=CARTESIAN_POINT('Ctrl Pts',(30.1304232450055,-33.550367157342,166.331204028951));
#36616=CARTESIAN_POINT('Ctrl Pts',(29.6837913440556,-31.2699909201536,166.220074239732));
#36617=CARTESIAN_POINT('Ctrl Pts',(31.3562571438711,-29.6587105925812,166.108944450511));
#36618=CARTESIAN_POINT('Ctrl Pts',(33.6192360418519,-30.188108801921,165.997814661292));
#36619=CARTESIAN_POINT('Ctrl Pts',(34.3974969940138,-32.3799455374906,165.886684872072));
#36620=CARTESIAN_POINT('Ctrl Pts',(33.4572031808892,-33.601662702255,165.812598345926));
#36621=CARTESIAN_POINT('Ctrl Pts',(32.8326019491383,-33.8785024771853,165.775555082853));
#36622=CARTESIAN_POINT('Ctrl Pts',(31.5032651029115,-33.8599788000025,179.074814972382));
#36623=CARTESIAN_POINT('Ctrl Pts',(30.8848229855218,-33.6948146693488,179.037771709309));
#36624=CARTESIAN_POINT('Ctrl Pts',(29.8364509972035,-32.7011677413673,178.963685183163));
#36625=CARTESIAN_POINT('Ctrl Pts',(30.2372125750557,-30.5591128827894,178.852555393943));
#36626=CARTESIAN_POINT('Ctrl Pts',(32.2544739729241,-29.7392339384594,178.741425604723));
#36627=CARTESIAN_POINT('Ctrl Pts',(34.0372807093117,-30.9866909111856,178.630295815504));
#36628=CARTESIAN_POINT('Ctrl Pts',(33.9563572920262,-33.1623445770418,178.519166026284));
#36629=CARTESIAN_POINT('Ctrl Pts',(32.0846201785151,-34.2738269199405,178.408036237064));
#36630=CARTESIAN_POINT('Ctrl Pts',(30.1356246356763,-33.3045270199694,178.296906447844));
#36631=CARTESIAN_POINT('Ctrl Pts',(29.8927943167313,-31.1412401472102,178.185776658625));
#36632=CARTESIAN_POINT('Ctrl Pts',(31.5785004329878,-29.7639291118385,178.074646869405));
#36633=CARTESIAN_POINT('Ctrl Pts',(33.6499364521924,-30.4330222613185,177.963517080185));
#36634=CARTESIAN_POINT('Ctrl Pts',(34.2113792950426,-32.5362080573748,177.852387290966));
#36635=CARTESIAN_POINT('Ctrl Pts',(32.7489864973565,-34.1486563498267,177.741257501746));
#36636=CARTESIAN_POINT('Ctrl Pts',(30.6011319786987,-33.7946804541288,177.630127712526));
#36637=CARTESIAN_POINT('Ctrl Pts',(29.733505026426,-31.7982310929729,177.518997923306));
#36638=CARTESIAN_POINT('Ctrl Pts',(30.9401503219258,-29.98643912349,177.407868134087));
#36639=CARTESIAN_POINT('Ctrl Pts',(33.1167582411914,-30.0174358999541,177.296738344867));
#36640=CARTESIAN_POINT('Ctrl Pts',(34.2713212801546,-31.8628540038831,177.185608555647));
#36641=CARTESIAN_POINT('Ctrl Pts',(33.347195640657,-33.83378655605,177.074478766427));
#36642=CARTESIAN_POINT('Ctrl Pts',(31.1901311970629,-34.1264575780627,176.963348977208));
#36643=CARTESIAN_POINT('Ctrl Pts',(29.7742498813245,-32.4730176657732,176.852219187988));
#36644=CARTESIAN_POINT('Ctrl Pts',(30.3953509457505,-30.3866771249266,176.741089398768));
#36645=CARTESIAN_POINT('Ctrl Pts',(32.4850094186051,-29.7768321789249,176.629959609548));
#36646=CARTESIAN_POINT('Ctrl Pts',(34.1307925333854,-31.2016063158112,176.518829820329));
#36647=CARTESIAN_POINT('Ctrl Pts',(33.8264974280504,-33.3570616931227,176.407700031109));
#36648=CARTESIAN_POINT('Ctrl Pts',(31.8506116846162,-34.2705489261624,176.296570241889));
#36649=CARTESIAN_POINT('Ctrl Pts',(30.0114445071206,-33.1060544047845,176.18544045267));
#36650=CARTESIAN_POINT('Ctrl Pts',(29.9921817518455,-30.9293108869418,176.07431066345));
#36651=CARTESIAN_POINT('Ctrl Pts',(31.8104524833385,-29.7324504341645,175.96318087423));
#36652=CARTESIAN_POINT('Ctrl Pts',(33.8021950465527,-30.610826753521,175.85205108501));
#36653=CARTESIAN_POINT('Ctrl Pts',(34.1445882471386,-32.7605593630827,175.740921295791));
#36654=CARTESIAN_POINT('Ctrl Pts',(32.5242775410416,-34.2142362914817,175.629791506571));
#36655=CARTESIAN_POINT('Ctrl Pts',(30.4241537149329,-33.6414681783056,175.518661717351));
#36656=CARTESIAN_POINT('Ctrl Pts',(29.766227319578,-31.5664461893272,175.407531928131));
#36657=CARTESIAN_POINT('Ctrl Pts',(31.1526254570884,-29.8882079461803,175.296402138912));
#36658=CARTESIAN_POINT('Ctrl Pts',(33.3145315868777,-30.1426588892585,175.185272349692));
#36659=CARTESIAN_POINT('Ctrl Pts',(34.2733926638577,-32.0969282748614,175.074142560472));
#36660=CARTESIAN_POINT('Ctrl Pts',(33.1516694287921,-33.9624899544547,174.963012771252));
#36661=CARTESIAN_POINT('Ctrl Pts',(30.9759508218308,-34.0320021100483,174.851882982033));
#36662=CARTESIAN_POINT('Ctrl Pts',(29.7374309173791,-32.241847970671,174.740753192813));
#36663=CARTESIAN_POINT('Ctrl Pts',(30.5695897008021,-30.2303571912677,174.629623403593));
#36664=CARTESIAN_POINT('Ctrl Pts',(32.7108444778972,-29.838424319439,174.518493614374));
#36665=CARTESIAN_POINT('Ctrl Pts',(34.2015420976082,-31.4247420691477,174.407363825154));
#36666=CARTESIAN_POINT('Ctrl Pts',(33.6774122643181,-33.5375296387599,174.296234035934));
#36667=CARTESIAN_POINT('Ctrl Pts',(31.6181329175025,-34.2431867567937,174.185104246714));
#36668=CARTESIAN_POINT('Ctrl Pts',(29.9083341834127,-32.8959036813573,174.073974457495));
#36669=CARTESIAN_POINT('Ctrl Pts',(30.1128053214922,-30.7286992724136,173.962844668275));
#36670=CARTESIAN_POINT('Ctrl Pts',(32.0444165635681,-29.7249755026746,173.851714879055));
#36671=CARTESIAN_POINT('Ctrl Pts',(33.935378248344,-30.8033294812745,173.740585089836));
#36672=CARTESIAN_POINT('Ctrl Pts',(34.0551027485386,-32.9768633412606,173.629455300616));
#36673=CARTESIAN_POINT('Ctrl Pts',(32.2940194999319,-34.2563824649668,173.518325511396));
#36674=CARTESIAN_POINT('Ctrl Pts',(30.2638527934963,-33.4708848261843,173.407195722177));
#36675=CARTESIAN_POINT('Ctrl Pts',(29.8225891827203,-31.3392493455597,173.296065932956));
#36676=CARTESIAN_POINT('Ctrl Pts',(31.3740683388817,-29.8123256983364,173.184936143737));
#36677=CARTESIAN_POINT('Ctrl Pts',(33.4983933633523,-30.2875378476557,173.073806354517));
#36678=CARTESIAN_POINT('Ctrl Pts',(34.2514050310823,-32.3299767879219,172.962676565298));
#36679=CARTESIAN_POINT('Ctrl Pts',(32.9439552298366,-34.0704245503311,172.851546776078));
#36680=CARTESIAN_POINT('Ctrl Pts',(30.7726078390127,-33.9160422170966,172.740416986858));
#36681=CARTESIAN_POINT('Ctrl Pts',(29.7245564434107,-32.0081188253879,172.629287197638));
#36682=CARTESIAN_POINT('Ctrl Pts',(30.7589663146413,-30.0927651727292,172.518157408419));
#36683=CARTESIAN_POINT('Ctrl Pts',(32.9291567562624,-29.9228921508882,172.407027619199));
#36684=CARTESIAN_POINT('Ctrl Pts',(34.2489930108375,-31.6539657072577,172.295897829979));
#36685=CARTESIAN_POINT('Ctrl Pts',(33.5105752512078,-33.7017260957593,172.184768040759));
#36686=CARTESIAN_POINT('Ctrl Pts',(31.3896954031792,-34.192085215873,172.07363825154));
#36687=CARTESIAN_POINT('Ctrl Pts',(29.8273597036832,-32.676271718594,171.96250846232));
#36688=CARTESIAN_POINT('Ctrl Pts',(30.2534008420735,-30.5415416783192,171.8513786731));
#36689=CARTESIAN_POINT('Ctrl Pts',(32.2779105887189,-29.7415768777247,171.74024888388));
#36690=CARTESIAN_POINT('Ctrl Pts',(34.0480795783837,-31.0084964270577,171.629119094661));
#36691=CARTESIAN_POINT('Ctrl Pts',(33.9438683484098,-33.1828292939389,171.517989305441));
#36692=CARTESIAN_POINT('Ctrl Pts',(32.0606498863458,-34.2746496182569,171.406859516222));
#36693=CARTESIAN_POINT('Ctrl Pts',(30.1219253060186,-33.284735279494,171.295729727001));
#36694=CARTESIAN_POINT('Ctrl Pts',(29.9019943187514,-31.1190451453122,171.184599937782));
#36695=CARTESIAN_POINT('Ctrl Pts',(31.6021353790386,-29.7595953405831,171.073470148562));
#36696=CARTESIAN_POINT('Ctrl Pts',(33.6663978257676,-30.4505395839755,170.962340359342));
#36697=CARTESIAN_POINT('Ctrl Pts',(34.205591053686,-32.559533196915,170.851210570123));
#36698=CARTESIAN_POINT('Ctrl Pts',(32.72625126791,-34.1564480959227,170.740080780903));
#36699=CARTESIAN_POINT('Ctrl Pts',(30.5822541976098,-33.7798050832478,170.628950991683));
#36700=CARTESIAN_POINT('Ctrl Pts',(29.7357627108441,-31.7743037595668,170.517821202464));
#36701=CARTESIAN_POINT('Ctrl Pts',(30.9614766364829,-29.9753571875565,170.406691413244));
#36702=CARTESIAN_POINT('Ctrl Pts',(33.1376358820957,-30.0293417611574,170.295561624024));
#36703=CARTESIAN_POINT('Ctrl Pts',(34.2726431055619,-31.8868513840484,170.184431834804));
#36704=CARTESIAN_POINT('Ctrl Pts',(33.327752004606,-33.8479133932125,170.073302045585));
#36705=CARTESIAN_POINT('Ctrl Pts',(31.1677166679057,-34.117785104695,169.962172256365));
#36706=CARTESIAN_POINT('Ctrl Pts',(29.7693780110011,-32.4494828547835,169.851042467145));
#36707=CARTESIAN_POINT('Ctrl Pts',(30.4124804083402,-30.369818770613,169.739912677925));
#36708=CARTESIAN_POINT('Ctrl Pts',(32.5084635200333,-29.7820788689979,169.628782888706));
#36709=CARTESIAN_POINT('Ctrl Pts',(34.139106332249,-31.2241563341233,169.517653099486));
#36710=CARTESIAN_POINT('Ctrl Pts',(33.8120622268332,-33.3762775085839,169.406523310266));
#36711=CARTESIAN_POINT('Ctrl Pts',(31.8266384224149,-34.2688444322986,169.295393521047));
#36712=CARTESIAN_POINT('Ctrl Pts',(29.9998732537773,-33.0849895361627,169.184263731827));
#36713=CARTESIAN_POINT('Ctrl Pts',(30.0036023928055,-30.908163982761,169.073133942607));
#36714=CARTESIAN_POINT('Ctrl Pts',(31.8344129719196,-29.73057491185,168.962004153387));
#36715=CARTESIAN_POINT('Ctrl Pts',(33.8167670033918,-30.62993907076,168.850874364168));
#36716=CARTESIAN_POINT('Ctrl Pts',(34.1364355754274,-32.7831681343442,168.739744574948));
#36717=CARTESIAN_POINT('Ctrl Pts',(32.5008614774095,-34.2196502146324,168.628614785728));
#36718=CARTESIAN_POINT('Ctrl Pts',(30.4069043870894,-33.6247324892858,168.517484996508));
#36719=CARTESIAN_POINT('Ctrl Pts',(29.7709311248822,-31.5428772098609,168.406355207289));
#36720=CARTESIAN_POINT('Ctrl Pts',(31.1749775247933,-29.8793757494069,168.295225418069));
#36721=CARTESIAN_POINT('Ctrl Pts',(33.3340755452748,-30.1566466084773,168.184095628849));
#36722=CARTESIAN_POINT('Ctrl Pts',(34.2722420977155,-32.1209344958534,168.072965839629));
#36723=CARTESIAN_POINT('Ctrl Pts',(33.1308773165435,-33.974544454855,167.96183605041));
#36724=CARTESIAN_POINT('Ctrl Pts',(30.9545458938293,-34.0210727199301,167.85070626119));
#36725=CARTESIAN_POINT('Ctrl Pts',(29.7350027016688,-32.2179371939027,167.73957647197));
#36726=CARTESIAN_POINT('Ctrl Pts',(30.588360535013,-30.2153478207362,167.628446682751));
#36727=CARTESIAN_POINT('Ctrl Pts',(32.7336353740468,-29.8460529529552,167.517316893531));
#36728=CARTESIAN_POINT('Ctrl Pts',(34.2074953272919,-31.4480266880878,167.406187104311));
#36729=CARTESIAN_POINT('Ctrl Pts',(33.6610789820475,-33.5551611777726,167.295057315091));
#36730=CARTESIAN_POINT('Ctrl Pts',(31.5944622129986,-34.2390274643665,167.183927525872));
#36731=CARTESIAN_POINT('Ctrl Pts',(29.8989870973908,-32.8737632690876,167.072797736652));
#36732=CARTESIAN_POINT('Ctrl Pts',(30.1263405447975,-30.7088339472683,166.961667947432));
#36733=CARTESIAN_POINT('Ctrl Pts',(32.06843797294,-29.7255789427341,166.850538158213));
#36734=CARTESIAN_POINT('Ctrl Pts',(33.9479196943688,-30.8238226576517,166.739408368993));
#36735=CARTESIAN_POINT('Ctrl Pts',(34.0446498234045,-32.9985456146712,166.628278579773));
#36736=CARTESIAN_POINT('Ctrl Pts',(32.2702131443668,-34.2592995138028,166.517148790553));
#36737=CARTESIAN_POINT('Ctrl Pts',(30.2483285803673,-33.4525928567512,166.406019001334));
#36738=CARTESIAN_POINT('Ctrl Pts',(29.8298636342772,-31.3160291291474,166.294889212114));
#36739=CARTESIAN_POINT('Ctrl Pts',(31.3968549514422,-29.8063646067977,166.183759422894));
#36740=CARTESIAN_POINT('Ctrl Pts',(33.517118507477,-30.3023761829087,166.072629633675));
#36741=CARTESIAN_POINT('Ctrl Pts',(34.2462982339988,-32.3559841751676,165.961499844455));
#36742=CARTESIAN_POINT('Ctrl Pts',(33.3653042902584,-33.5006534350284,165.887413318308));
#36743=CARTESIAN_POINT('Ctrl Pts',(32.7800936946503,-33.7600342388747,165.850370055235));
#36744=CARTESIAN_POINT('Ctrl Pts',(31.5367004230124,-33.7347832743336,179.149629944765));
#36745=CARTESIAN_POINT('Ctrl Pts',(30.9598857617972,-33.5807363726283,179.112586681692));
#36746=CARTESIAN_POINT('Ctrl Pts',(29.9820798907776,-32.6539720077587,179.038500155545));
#36747=CARTESIAN_POINT('Ctrl Pts',(30.3558661308426,-30.6560992678324,178.927370366326));
#36748=CARTESIAN_POINT('Ctrl Pts',(32.2373452815599,-29.8914065306893,178.816240577106));
#36749=CARTESIAN_POINT('Ctrl Pts',(33.9001509585118,-31.054896938071,178.705110787886));
#36750=CARTESIAN_POINT('Ctrl Pts',(33.8246745117864,-33.0841069431875,178.593980998666));
#36751=CARTESIAN_POINT('Ctrl Pts',(32.0789243782558,-34.1207751988554,178.482851209447));
#36752=CARTESIAN_POINT('Ctrl Pts',(30.2611160949232,-33.2167190589247,178.371721420227));
#36753=CARTESIAN_POINT('Ctrl Pts',(30.0346307307857,-31.1990434357172,178.260591631007));
#36754=CARTESIAN_POINT('Ctrl Pts',(31.6068716487571,-29.9144394672662,178.149461841787));
#36755=CARTESIAN_POINT('Ctrl Pts',(33.5388789167773,-30.5384958299987,178.038332052568));
#36756=CARTESIAN_POINT('Ctrl Pts',(34.0625309354291,-32.5001157913711,177.927202263348));
#36757=CARTESIAN_POINT('Ctrl Pts',(32.6985720742161,-34.0040298835476,177.816072474128));
#36758=CARTESIAN_POINT('Ctrl Pts',(30.6952900504295,-33.6738801725007,177.704942684908));
#36759=CARTESIAN_POINT('Ctrl Pts',(29.8860632328111,-31.811812196359,177.593812895689));
#36760=CARTESIAN_POINT('Ctrl Pts',(31.011489004698,-30.1219722878469,177.482683106469));
#36761=CARTESIAN_POINT('Ctrl Pts',(33.0415890322462,-30.1508826654104,177.371553317249));
#36762=CARTESIAN_POINT('Ctrl Pts',(34.1184382141585,-31.8720853268838,177.26042352803));
#36763=CARTESIAN_POINT('Ctrl Pts',(33.2565156466643,-33.7103540352874,177.14929373881));
#36764=CARTESIAN_POINT('Ctrl Pts',(31.2446436197348,-33.9833253153198,177.03816394959));
#36765=CARTESIAN_POINT('Ctrl Pts',(29.9240655438013,-32.4411787570087,176.92703416037));
#36766=CARTESIAN_POINT('Ctrl Pts',(30.5033601778239,-30.4952701935241,176.815904371151));
#36767=CARTESIAN_POINT('Ctrl Pts',(32.4523633426839,-29.9264740264607,176.704774581931));
#36768=CARTESIAN_POINT('Ctrl Pts',(33.9873684839778,-31.2553463460645,176.593644792711));
#36769=CARTESIAN_POINT('Ctrl Pts',(33.7035555398755,-33.2657176132679,176.482515003491));
#36770=CARTESIAN_POINT('Ctrl Pts',(31.8606670404478,-34.11771784746,176.371385214272));
#36771=CARTESIAN_POINT('Ctrl Pts',(30.1452945543645,-33.0316056730973,176.260255425052));
#36772=CARTESIAN_POINT('Ctrl Pts',(30.127328378799,-31.0013791741379,176.149125635832));
#36773=CARTESIAN_POINT('Ctrl Pts',(31.8232109626221,-29.8850796253547,176.037995846613));
#36774=CARTESIAN_POINT('Ctrl Pts',(33.6808889562839,-30.7043322681203,175.926866057393));
#36775=CARTESIAN_POINT('Ctrl Pts',(34.0002356056227,-32.7093659681561,175.815736268173));
#36776=CARTESIAN_POINT('Ctrl Pts',(32.4889883203542,-34.0651956268962,175.704606478953));
#36777=CARTESIAN_POINT('Ctrl Pts',(30.5302242271517,-33.5309806440114,175.593476689734));
#36778=CARTESIAN_POINT('Ctrl Pts',(29.9165829822071,-31.5956287785228,175.482346900514));
#36779=CARTESIAN_POINT('Ctrl Pts',(31.2096623982289,-30.030353069706,175.371217111294));
#36780=CARTESIAN_POINT('Ctrl Pts',(33.2260502165377,-30.2676768715632,175.260087322075));
#36781=CARTESIAN_POINT('Ctrl Pts',(34.1203701726319,-32.0904040143035,175.148957532855));
#36782=CARTESIAN_POINT('Ctrl Pts',(33.0741503411905,-33.8303943835441,175.037827743635));
#36783=CARTESIAN_POINT('Ctrl Pts',(31.0448797661669,-33.8952276627656,174.926697954415));
#36784=CARTESIAN_POINT('Ctrl Pts',(29.8897248712998,-32.2255691379122,174.815568165196));
#36785=CARTESIAN_POINT('Ctrl Pts',(30.6658708892383,-30.349472184237,174.704438375976));
#36786=CARTESIAN_POINT('Ctrl Pts',(32.6629974013181,-29.9839203883193,174.593308586756));
#36787=CARTESIAN_POINT('Ctrl Pts',(34.0533558816191,-31.4634627895388,174.482178797536));
#36788=CARTESIAN_POINT('Ctrl Pts',(33.5645053267795,-33.4340382272686,174.371049008317));
#36789=CARTESIAN_POINT('Ctrl Pts',(31.6438364632251,-34.0921974308992,174.259919219097));
#36790=CARTESIAN_POINT('Ctrl Pts',(30.0491246060944,-32.8356002347072,174.148789429877));
#36791=CARTESIAN_POINT('Ctrl Pts',(30.2398327531034,-30.8142707654184,174.037659640658));
#36792=CARTESIAN_POINT('Ctrl Pts',(32.0414268762532,-29.8781078329205,173.926529851438));
#36793=CARTESIAN_POINT('Ctrl Pts',(33.8051075715119,-30.8838776007715,173.815400062218));
#36794=CARTESIAN_POINT('Ctrl Pts',(33.9167733928993,-32.9111104845529,173.704270272998));
#36795=CARTESIAN_POINT('Ctrl Pts',(32.2742289916473,-34.1045049334533,173.593140483779));
#36796=CARTESIAN_POINT('Ctrl Pts',(30.3807131911291,-33.3718792896629,173.482010694559));
#36797=CARTESIAN_POINT('Ctrl Pts',(29.9691511176554,-31.3837245973844,173.370880905339));
#36798=CARTESIAN_POINT('Ctrl Pts',(31.4161999176645,-29.9595784703513,173.25975111612));
#36799=CARTESIAN_POINT('Ctrl Pts',(33.3975362219787,-30.4028039998025,173.1486213269));
#36800=CARTESIAN_POINT('Ctrl Pts',(34.0998625315873,-32.3077659877652,173.03749153768));
#36801=CARTESIAN_POINT('Ctrl Pts',(32.8804174243481,-33.9310638813083,172.92636174846));
#36802=CARTESIAN_POINT('Ctrl Pts',(30.8552238380749,-33.7870730521938,172.81523195924));
#36803=CARTESIAN_POINT('Ctrl Pts',(29.877716980615,-32.0075723457118,172.704102170021));
#36804=CARTESIAN_POINT('Ctrl Pts',(30.8425005272953,-30.221141510553,172.592972380801));
#36805=CARTESIAN_POINT('Ctrl Pts',(32.8666150388358,-30.0627026740191,172.481842591581));
#36806=CARTESIAN_POINT('Ctrl Pts',(34.0976128648825,-31.6772573411082,172.370712802362));
#36807=CARTESIAN_POINT('Ctrl Pts',(33.4088981446531,-33.5871825896167,172.259583013142));
#36808=CARTESIAN_POINT('Ctrl Pts',(31.4307751213012,-34.0445355443865,172.148453223922));
#36809=CARTESIAN_POINT('Ctrl Pts',(29.9736005339478,-32.6307517409984,172.037323434702));
#36810=CARTESIAN_POINT('Ctrl Pts',(30.3709647625382,-30.6397107844664,171.926193645483));
#36811=CARTESIAN_POINT('Ctrl Pts',(32.2592043743021,-29.8935917662685,171.815063856263));
#36812=CARTESIAN_POINT('Ctrl Pts',(33.9102229536591,-31.0752347205356,171.703934067043));
#36813=CARTESIAN_POINT('Ctrl Pts',(33.8130262013327,-33.1032128299065,171.592804277823));
#36814=CARTESIAN_POINT('Ctrl Pts',(32.056567530997,-34.1215425211921,171.481674488604));
#36815=CARTESIAN_POINT('Ctrl Pts',(30.2483388697421,-33.1982595042532,171.370544699384));
#36816=CARTESIAN_POINT('Ctrl Pts',(30.0432114789254,-31.178342383605,171.259414910164));
#36817=CARTESIAN_POINT('Ctrl Pts',(31.6289157221082,-29.9103974029757,171.148285120945));
#36818=CARTESIAN_POINT('Ctrl Pts',(33.5542322721762,-30.5548340583465,171.037155331725));
#36819=CARTESIAN_POINT('Ctrl Pts',(34.0571323016956,-32.5218709113466,170.926025542505));
#36820=CARTESIAN_POINT('Ctrl Pts',(32.6773671573741,-34.0112971657366,170.814895753285));
#36821=CARTESIAN_POINT('Ctrl Pts',(30.6776829363647,-33.6600060656541,170.703765964066));
#36822=CARTESIAN_POINT('Ctrl Pts',(29.8881689520629,-31.789495416301,170.592636174846));
#36823=CARTESIAN_POINT('Ctrl Pts',(31.0313798409791,-30.1116362791222,170.481506385626));
#36824=CARTESIAN_POINT('Ctrl Pts',(33.0610613951829,-30.1619871408389,170.370376596406));
#36825=CARTESIAN_POINT('Ctrl Pts',(34.1196710672471,-31.8944674388404,170.259246807187));
#36826=CARTESIAN_POINT('Ctrl Pts',(33.2383807654422,-33.7235299923622,170.148117017967));
#36827=CARTESIAN_POINT('Ctrl Pts',(31.2237378167849,-33.9752365877787,170.036987228748));
#36828=CARTESIAN_POINT('Ctrl Pts',(29.9195215999931,-32.4192280786088,169.925857439527));
#36829=CARTESIAN_POINT('Ctrl Pts',(30.519336653039,-30.4795465782356,169.814727650308));
#36830=CARTESIAN_POINT('Ctrl Pts',(32.4742387440983,-29.9313675608301,169.703597861088));
#36831=CARTESIAN_POINT('Ctrl Pts',(33.9951226794636,-31.2763785183688,169.592468071869));
#36832=CARTESIAN_POINT('Ctrl Pts',(33.690091974789,-33.2836400085472,169.481338282649));
#36833=CARTESIAN_POINT('Ctrl Pts',(31.8383074230704,-34.1161280834014,169.370208493429));
#36834=CARTESIAN_POINT('Ctrl Pts',(30.1345021642776,-33.0119586847762,169.259078704209));
#36835=CARTESIAN_POINT('Ctrl Pts',(30.1379802942507,-30.9816556720869,169.14794891499));
#36836=CARTESIAN_POINT('Ctrl Pts',(31.845558666174,-29.8833303448027,169.03681912577));
#36837=CARTESIAN_POINT('Ctrl Pts',(33.6944800719454,-30.7221581316624,168.92568933655));
#36838=CARTESIAN_POINT('Ctrl Pts',(33.9926316917901,-32.7304529387375,168.81455954733));
#36839=CARTESIAN_POINT('Ctrl Pts',(32.4671483964048,-34.0702451378531,168.703429758111));
#36840=CARTESIAN_POINT('Ctrl Pts',(30.5141359548357,-33.5153714373925,168.592299968891));
#36841=CARTESIAN_POINT('Ctrl Pts',(29.9209701734844,-31.5736462315329,168.481170179671));
#36842=CARTESIAN_POINT('Ctrl Pts',(31.2305099440188,-30.0221153697719,168.370040390451));
#36843=CARTESIAN_POINT('Ctrl Pts',(33.2442786673897,-30.2807230747493,168.258910601232));
#36844=CARTESIAN_POINT('Ctrl Pts',(34.1192970513148,-32.1127943720091,168.147780812012));
#36845=CARTESIAN_POINT('Ctrl Pts',(33.0547577499595,-33.841637493237,168.036651022792));
#36846=CARTESIAN_POINT('Ctrl Pts',(31.0249156079274,-33.8850339319685,167.925521233573));
#36847=CARTESIAN_POINT('Ctrl Pts',(29.8874600992493,-32.2032678000614,167.814391444353));
#36848=CARTESIAN_POINT('Ctrl Pts',(30.6833782550396,-30.3354730972818,167.703261655133));
#36849=CARTESIAN_POINT('Ctrl Pts',(32.6842542379269,-29.9910355370672,167.592131865913));
#36850=CARTESIAN_POINT('Ctrl Pts',(34.0589083982841,-31.4851801163634,167.481002076694));
#36851=CARTESIAN_POINT('Ctrl Pts',(33.5492714408353,-33.4504829840476,167.369872287474));
#36852=CARTESIAN_POINT('Ctrl Pts',(31.6217590383292,-34.0883181012338,167.258742498254));
#36853=CARTESIAN_POINT('Ctrl Pts',(30.0404066742048,-32.8149500977851,167.147612709034));
#36854=CARTESIAN_POINT('Ctrl Pts',(30.2524569179617,-30.7957425790749,167.036482919815));
#36855=CARTESIAN_POINT('Ctrl Pts',(32.063831400006,-29.8786706553152,166.925353130595));
#36856=CARTESIAN_POINT('Ctrl Pts',(33.816804850427,-30.9029913775613,166.814223341375));
#36857=CARTESIAN_POINT('Ctrl Pts',(33.9070240561379,-32.9313333200294,166.703093552155));
#36858=CARTESIAN_POINT('Ctrl Pts',(32.2520250463887,-34.1072256351791,166.591963762936));
#36859=CARTESIAN_POINT('Ctrl Pts',(30.3662339157292,-33.3548185561604,166.480833973716));
#36860=CARTESIAN_POINT('Ctrl Pts',(29.9759359244988,-31.3620673381413,166.369704184496));
#36861=CARTESIAN_POINT('Ctrl Pts',(31.4374527590133,-29.9540186210142,166.258574395277));
#36862=CARTESIAN_POINT('Ctrl Pts',(33.4150009731022,-30.4166435638964,166.147444606057));
#36863=CARTESIAN_POINT('Ctrl Pts',(34.0950994739837,-32.3320228128446,166.036314816837));
#36864=CARTESIAN_POINT('Ctrl Pts',(33.2734053996277,-33.3996441678017,165.962228290691));
#36865=CARTESIAN_POINT('Ctrl Pts',(32.7275854401623,-33.6415660005642,165.925185027618));
#36866=CARTESIAN_POINT('Ctrl Pts',(31.5701357431134,-33.6095877486647,179.224444917147));
#36867=CARTESIAN_POINT('Ctrl Pts',(31.0349485380725,-33.4666580759078,179.187401654074));
#36868=CARTESIAN_POINT('Ctrl Pts',(30.1277087843517,-32.6067762741501,179.113315127928));
#36869=CARTESIAN_POINT('Ctrl Pts',(30.4745196866295,-30.7530856528753,179.002185338708));
#36870=CARTESIAN_POINT('Ctrl Pts',(32.2202165901956,-30.0435791229192,178.891055549488));
#36871=CARTESIAN_POINT('Ctrl Pts',(33.7630212077119,-31.1231029649564,178.779925760268));
#36872=CARTESIAN_POINT('Ctrl Pts',(33.6929917315466,-33.0058693093333,178.668795971049));
#36873=CARTESIAN_POINT('Ctrl Pts',(32.0732285779965,-33.9677234777703,178.557666181829));
#36874=CARTESIAN_POINT('Ctrl Pts',(30.3866075541702,-33.1289110978801,178.446536392609));
#36875=CARTESIAN_POINT('Ctrl Pts',(30.17646714484,-31.2568467242241,178.33540660339));
#36876=CARTESIAN_POINT('Ctrl Pts',(31.6352428645265,-30.064949822694,178.22427681417));
#36877=CARTESIAN_POINT('Ctrl Pts',(33.4278213813623,-30.6439693986789,178.11314702495));
#36878=CARTESIAN_POINT('Ctrl Pts',(33.9136825758156,-32.4640235253674,178.002017235731));
#36879=CARTESIAN_POINT('Ctrl Pts',(32.6481576510757,-33.8594034172685,177.890887446511));
#36880=CARTESIAN_POINT('Ctrl Pts',(30.7894481221602,-33.5530798908727,177.779757657291));
#36881=CARTESIAN_POINT('Ctrl Pts',(30.0386214391961,-31.8253932997452,177.668627868071));
#36882=CARTESIAN_POINT('Ctrl Pts',(31.0828276874703,-30.2575054522038,177.557498078852));
#36883=CARTESIAN_POINT('Ctrl Pts',(32.9664198233009,-30.2843294308667,177.446368289632));
#36884=CARTESIAN_POINT('Ctrl Pts',(33.9655551481625,-31.8813166498845,177.335238500412));
#36885=CARTESIAN_POINT('Ctrl Pts',(33.1658356526715,-33.5869215145248,177.224108711192));
#36886=CARTESIAN_POINT('Ctrl Pts',(31.2991560424068,-33.8401930525768,177.112978921973));
#36887=CARTESIAN_POINT('Ctrl Pts',(30.0738812062782,-32.4093398482442,177.001849132753));
#36888=CARTESIAN_POINT('Ctrl Pts',(30.6113694098972,-30.6038632621215,176.890719343533));
#36889=CARTESIAN_POINT('Ctrl Pts',(32.4197172667628,-30.0761158739965,176.779589554313));
#36890=CARTESIAN_POINT('Ctrl Pts',(33.8439444345702,-31.3090863763179,176.668459765094));
#36891=CARTESIAN_POINT('Ctrl Pts',(33.5806136517005,-33.1743735334131,176.557329975874));
#36892=CARTESIAN_POINT('Ctrl Pts',(31.8707223962794,-33.9648867687576,176.446200186654));
#36893=CARTESIAN_POINT('Ctrl Pts',(30.2791446016083,-32.9571569414099,176.335070397435));
#36894=CARTESIAN_POINT('Ctrl Pts',(30.2624750057525,-31.0734474613341,176.223940608215));
#36895=CARTESIAN_POINT('Ctrl Pts',(31.8359694419057,-30.0377088165447,176.112810818995));
#36896=CARTESIAN_POINT('Ctrl Pts',(33.5595828660151,-30.7978377827197,176.001681029775));
#36897=CARTESIAN_POINT('Ctrl Pts',(33.8558829641068,-32.6581725732295,175.890551240556));
#36898=CARTESIAN_POINT('Ctrl Pts',(32.4536990996669,-33.9161549623108,175.779421451336));
#36899=CARTESIAN_POINT('Ctrl Pts',(30.6362947393706,-33.4204931097171,175.668291662116));
#36900=CARTESIAN_POINT('Ctrl Pts',(30.0669386448361,-31.6248113677183,175.557161872896));
#36901=CARTESIAN_POINT('Ctrl Pts',(31.2666993393694,-30.1724981932316,175.446032083677));
#36902=CARTESIAN_POINT('Ctrl Pts',(33.1375688461977,-30.3926948538679,175.334902294457));
#36903=CARTESIAN_POINT('Ctrl Pts',(33.9673476814061,-32.0838797537456,175.223772505237));
#36904=CARTESIAN_POINT('Ctrl Pts',(32.9966312535889,-33.6982988126334,175.112642716018));
#36905=CARTESIAN_POINT('Ctrl Pts',(31.113808710503,-33.7584532154829,175.001512926798));
#36906=CARTESIAN_POINT('Ctrl Pts',(30.0420188252204,-32.2092903051534,174.890383137578));
#36907=CARTESIAN_POINT('Ctrl Pts',(30.7621520776745,-30.4685871772064,174.779253348358));
#36908=CARTESIAN_POINT('Ctrl Pts',(32.615150324739,-30.1294164571996,174.668123559139));
#36909=CARTESIAN_POINT('Ctrl Pts',(33.90516966563,-31.5021835099298,174.556993769919));
#36910=CARTESIAN_POINT('Ctrl Pts',(33.451598389241,-33.3305468157773,174.445863980699));
#36911=CARTESIAN_POINT('Ctrl Pts',(31.6695400089477,-33.9412081050047,174.334734191479));
#36912=CARTESIAN_POINT('Ctrl Pts',(30.1899150287761,-32.7752967880571,174.22360440226));
#36913=CARTESIAN_POINT('Ctrl Pts',(30.3668601847145,-30.8998422584232,174.11247461304));
#36914=CARTESIAN_POINT('Ctrl Pts',(32.0384371889383,-30.0312401631664,174.00134482382));
#36915=CARTESIAN_POINT('Ctrl Pts',(33.6748368946798,-30.9644257202684,173.890215034601));
#36916=CARTESIAN_POINT('Ctrl Pts',(33.7784440372601,-32.8453576278453,173.779085245381));
#36917=CARTESIAN_POINT('Ctrl Pts',(32.2544384833625,-33.9526274019399,173.667955456161));
#36918=CARTESIAN_POINT('Ctrl Pts',(30.4975735887619,-33.2728737531416,173.556825666941));
#36919=CARTESIAN_POINT('Ctrl Pts',(30.1157130525905,-31.4281998492091,173.445695877722));
#36920=CARTESIAN_POINT('Ctrl Pts',(31.4583314964472,-30.1068312423661,173.334566088502));
#36921=CARTESIAN_POINT('Ctrl Pts',(33.2966790806051,-30.5180701519493,173.223436299282));
#36922=CARTESIAN_POINT('Ctrl Pts',(33.9483200320923,-32.2855551876086,173.112306510063));
#36923=CARTESIAN_POINT('Ctrl Pts',(32.8168796188595,-33.7917032122855,173.001176720843));
#36924=CARTESIAN_POINT('Ctrl Pts',(30.9378398371371,-33.658103887291,172.890046931623));
#36925=CARTESIAN_POINT('Ctrl Pts',(30.0308775178194,-32.0070258660356,172.778917142403));
#36926=CARTESIAN_POINT('Ctrl Pts',(30.9260347399493,-30.3495178483768,172.667787353183));
#36927=CARTESIAN_POINT('Ctrl Pts',(32.8040733214092,-30.2025131971499,172.556657563964));
#36928=CARTESIAN_POINT('Ctrl Pts',(33.9462327189276,-31.7005489749587,172.445527774744));
#36929=CARTESIAN_POINT('Ctrl Pts',(33.3072210380983,-33.4726390834741,172.334397985525));
#36930=CARTESIAN_POINT('Ctrl Pts',(31.4718548394233,-33.8969858728999,172.223268196305));
#36931=CARTESIAN_POINT('Ctrl Pts',(30.1198413642124,-32.5852317634028,172.112138407085));
#36932=CARTESIAN_POINT('Ctrl Pts',(30.4885286830029,-30.7378798906137,172.001008617865));
#36933=CARTESIAN_POINT('Ctrl Pts',(32.2404981598852,-30.0456066548122,171.889878828646));
#36934=CARTESIAN_POINT('Ctrl Pts',(33.7723663289346,-31.1419730140134,171.778749039426));
#36935=CARTESIAN_POINT('Ctrl Pts',(33.6821840542554,-33.0235963658742,171.667619250206));
#36936=CARTESIAN_POINT('Ctrl Pts',(32.0524851756482,-33.9684354241274,171.556489460986));
#36937=CARTESIAN_POINT('Ctrl Pts',(30.3747524334657,-33.1117837290124,171.445359671766));
#36938=CARTESIAN_POINT('Ctrl Pts',(30.1844286390995,-31.2376396218978,171.334229882547));
#36939=CARTESIAN_POINT('Ctrl Pts',(31.6556960651779,-30.0611994653682,171.223100093327));
#36940=CARTESIAN_POINT('Ctrl Pts',(33.4420667185848,-30.6591285327175,171.111970304107));
#36941=CARTESIAN_POINT('Ctrl Pts',(33.9086735497053,-32.4842086257781,171.000840514888));
#36942=CARTESIAN_POINT('Ctrl Pts',(32.6284830468382,-33.8661462355505,170.889710725668));
#36943=CARTESIAN_POINT('Ctrl Pts',(30.7731116751197,-33.5402070480603,170.778580936448));
#36944=CARTESIAN_POINT('Ctrl Pts',(30.0405751932818,-31.8046870730353,170.667451147228));
#36945=CARTESIAN_POINT('Ctrl Pts',(31.1012830454752,-30.2479153706878,170.556321358009));
#36946=CARTESIAN_POINT('Ctrl Pts',(32.9844869082701,-30.2946325205203,170.445191568789));
#36947=CARTESIAN_POINT('Ctrl Pts',(33.9666990289323,-31.9020834936324,170.334061779569));
#36948=CARTESIAN_POINT('Ctrl Pts',(33.1490095262784,-33.5991465915118,170.222931990349));
#36949=CARTESIAN_POINT('Ctrl Pts',(31.279758965664,-33.8326880708624,170.11180220113));
#36950=CARTESIAN_POINT('Ctrl Pts',(30.0696651889851,-32.3889733024341,170.00067241191));
#36951=CARTESIAN_POINT('Ctrl Pts',(30.6261928977377,-30.5892743858582,169.889542622691));
#36952=CARTESIAN_POINT('Ctrl Pts',(32.4400139681632,-30.0806562526623,169.77841283347));
#36953=CARTESIAN_POINT('Ctrl Pts',(33.8511390266782,-31.3286007026142,169.667283044251));
#36954=CARTESIAN_POINT('Ctrl Pts',(33.5681217227447,-33.1910025085104,169.556153255031));
#36955=CARTESIAN_POINT('Ctrl Pts',(31.849976423726,-33.9634117345042,169.445023465811));
#36956=CARTESIAN_POINT('Ctrl Pts',(30.2691310747778,-32.9389278333895,169.333893676592));
#36957=CARTESIAN_POINT('Ctrl Pts',(30.2723581956959,-31.0551473614128,169.222763887372));
#36958=CARTESIAN_POINT('Ctrl Pts',(31.8567043604284,-30.0360857777554,169.111634098152));
#36959=CARTESIAN_POINT('Ctrl Pts',(33.572193140499,-30.8143771925649,169.000504308933));
#36960=CARTESIAN_POINT('Ctrl Pts',(33.8488278081528,-32.6777377431309,168.889374519713));
#36961=CARTESIAN_POINT('Ctrl Pts',(32.4334353154,-33.920840061074,168.778244730493));
#36962=CARTESIAN_POINT('Ctrl Pts',(30.6213675225821,-33.4060103854991,168.667114941273));
#36963=CARTESIAN_POINT('Ctrl Pts',(30.0710092220866,-31.6044152532049,168.555985152054));
#36964=CARTESIAN_POINT('Ctrl Pts',(31.2860423632443,-30.1648549901369,168.444855362834));
#36965=CARTESIAN_POINT('Ctrl Pts',(33.1544817895046,-30.4047995410214,168.333725573614));
#36966=CARTESIAN_POINT('Ctrl Pts',(33.9663520049142,-32.1046542481647,168.222595784395));
#36967=CARTESIAN_POINT('Ctrl Pts',(32.9786381833754,-33.7087305316189,168.111465995175));
#36968=CARTESIAN_POINT('Ctrl Pts',(31.0952853220256,-33.7489951440067,168.000336205955));
#36969=CARTESIAN_POINT('Ctrl Pts',(30.0399174968298,-32.1885984062203,167.889206416735));
#36970=CARTESIAN_POINT('Ctrl Pts',(30.7783959750662,-30.4555983738273,167.778076627515));
#36971=CARTESIAN_POINT('Ctrl Pts',(32.634873101807,-30.1360181211792,167.666946838296));
#36972=CARTESIAN_POINT('Ctrl Pts',(33.9103214692762,-31.522333544639,167.555817049076));
#36973=CARTESIAN_POINT('Ctrl Pts',(33.4374638996232,-33.3458047903225,167.444687259856));
#36974=CARTESIAN_POINT('Ctrl Pts',(31.6490558636597,-33.9376087381012,167.333557470637));
#36975=CARTESIAN_POINT('Ctrl Pts',(30.1818262510189,-32.7561369264825,167.222427681417));
#36976=CARTESIAN_POINT('Ctrl Pts',(30.3785732911259,-30.8826512108817,167.111297892197));
#36977=CARTESIAN_POINT('Ctrl Pts',(32.059224827072,-30.0317623678963,167.000168102977));
#36978=CARTESIAN_POINT('Ctrl Pts',(33.6856900064852,-30.9821600974709,166.889038313758));
#36979=CARTESIAN_POINT('Ctrl Pts',(33.7693982888712,-32.8641210253877,166.777908524538));
#36980=CARTESIAN_POINT('Ctrl Pts',(32.2338369484106,-33.9551517565555,166.666778735318));
#36981=CARTESIAN_POINT('Ctrl Pts',(30.484139251091,-33.2570442555697,166.555648946099));
#36982=CARTESIAN_POINT('Ctrl Pts',(30.1220082147204,-31.4081055471351,166.444519156879));
#36983=CARTESIAN_POINT('Ctrl Pts',(31.4780505665844,-30.1016726352307,166.333389367659));
#36984=CARTESIAN_POINT('Ctrl Pts',(33.3128834387275,-30.530910944884,166.222259578439));
#36985=CARTESIAN_POINT('Ctrl Pts',(33.9439007139686,-32.3080614505216,166.11112978922));
#36986=CARTESIAN_POINT('Ctrl Pts',(33.1815065089969,-33.2986349005751,166.037043263073));
#36987=CARTESIAN_POINT('Ctrl Pts',(32.6750771856743,-33.5230977622536,166.));
#36988=CARTESIAN_POINT('Ctrl Pts',(30.3361334267378,-31.9990537049732,178.37851963661));
#36989=CARTESIAN_POINT('Ctrl Pts',(30.3350134860168,-31.7834929963847,178.364148625536));
#36990=CARTESIAN_POINT('Ctrl Pts',(30.3738847213991,-31.5683196627767,178.349777614463));
#36991=CARTESIAN_POINT('Ctrl Pts',(30.4546198330094,-31.3702079695784,178.33540660339));
#36992=CARTESIAN_POINT('Ctrl Pts',(30.6627257180688,-30.8595477570474,178.298363340316));
#36993=CARTESIAN_POINT('Ctrl Pts',(31.1489842912976,-30.4622487898707,178.261320077243));
#36994=CARTESIAN_POINT('Ctrl Pts',(31.6908766640514,-30.3601025689465,178.22427681417));
#36995=CARTESIAN_POINT('Ctrl Pts',(32.2327690368051,-30.2579563480223,178.187233551097));
#36996=CARTESIAN_POINT('Ctrl Pts',(32.8302952090837,-30.4509628733506,178.150190288023));
#36997=CARTESIAN_POINT('Ctrl Pts',(33.2100351609652,-30.8508084904628,178.11314702495));
#36998=CARTESIAN_POINT('Ctrl Pts',(33.5897751128467,-31.2506541075751,178.076103761877));
#36999=CARTESIAN_POINT('Ctrl Pts',(33.7517288443312,-31.8573388164712,178.039060498804));
#37000=CARTESIAN_POINT('Ctrl Pts',(33.6217848892834,-32.3932444862362,178.002017235731));
#37001=CARTESIAN_POINT('Ctrl Pts',(33.4918409342357,-32.9291501560011,177.964973972657));
#37002=CARTESIAN_POINT('Ctrl Pts',(33.0699992926557,-33.3942767866348,177.927930709584));
#37003=CARTESIAN_POINT('Ctrl Pts',(32.5492935503798,-33.5757861808857,177.890887446511));
#37004=CARTESIAN_POINT('Ctrl Pts',(32.0285878081039,-33.7572955751366,177.853844183437));
#37005=CARTESIAN_POINT('Ctrl Pts',(31.4090179651321,-33.6551877330046,177.816800920364));
#37006=CARTESIAN_POINT('Ctrl Pts',(30.9740952631521,-33.3161860467508,177.779757657291));
#37007=CARTESIAN_POINT('Ctrl Pts',(30.5778854457224,-33.0073592239439,177.746011650397));
#37008=CARTESIAN_POINT('Ctrl Pts',(30.3349144830452,-32.5019339530042,177.712265643504));
#37009=CARTESIAN_POINT('Ctrl Pts',(30.3317668085256,-31.999144727569,177.67851963661));
#37010=CARTESIAN_POINT('Ctrl Pts',(31.4698297828105,-33.9851743256715,179.));
#37011=CARTESIAN_POINT('Ctrl Pts',(31.4011717473165,-33.959752800589,179.));
#37012=CARTESIAN_POINT('Ctrl Pts',(31.3342169943201,-33.9304405272318,179.));
#37013=CARTESIAN_POINT('Ctrl Pts',(31.2691543409406,-33.8975318476629,179.));
#37014=CARTESIAN_POINT('Ctrl Pts',(31.2022750469363,-33.8637043115593,179.));
#37015=CARTESIAN_POINT('Ctrl Pts',(31.1373942160753,-33.8260760433842,179.));
#37016=CARTESIAN_POINT('Ctrl Pts',(31.0747481415806,-33.7849220758473,179.));
#37017=CARTESIAN_POINT('Ctrl Pts',(31.0218168792491,-33.7501500415378,179.));
#37018=CARTESIAN_POINT('Ctrl Pts',(30.9704813415884,-33.7128599624529,179.));
#37019=CARTESIAN_POINT('Ctrl Pts',(30.9209067960986,-33.6731997220801,179.));
#37020=CARTESIAN_POINT('Ctrl Pts',(30.8988714343571,-33.6555711642237,179.));
#37021=CARTESIAN_POINT('Ctrl Pts',(30.8771842966684,-33.6374741525735,179.));
#37022=CARTESIAN_POINT('Ctrl Pts',(30.8558614512686,-33.6189209496161,179.));
#37023=CARTESIAN_POINT('Ctrl Pts',(30.8441499403614,-33.6087306567763,179.));
#37024=CARTESIAN_POINT('Ctrl Pts',(30.8325483440617,-33.5984027370162,179.));
#37025=CARTESIAN_POINT('Ctrl Pts',(30.8210594589826,-33.5879391805166,179.));
#37026=CARTESIAN_POINT('Ctrl Pts',(30.8104646008526,-33.5782898632951,179.));
#37027=CARTESIAN_POINT('Ctrl Pts',(30.79996415815,-33.5685236791905,179.));
#37028=CARTESIAN_POINT('Ctrl Pts',(30.7895762178146,-33.558657652978,179.));
#37029=CARTESIAN_POINT('Ctrl Pts',(30.7364925058988,-33.5082409893936,179.));
#37030=CARTESIAN_POINT('Ctrl Pts',(30.6862488283153,-33.4551355694144,179.));
#37031=CARTESIAN_POINT('Ctrl Pts',(30.6390637895127,-33.3996012573837,179.));
#37032=CARTESIAN_POINT('Ctrl Pts',(30.5922435997919,-33.3444963535567,179.));
#37033=CARTESIAN_POINT('Ctrl Pts',(30.5484344225798,-33.2869990900772,179.));
#37034=CARTESIAN_POINT('Ctrl Pts',(30.5078946257251,-33.2273391119527,179.));
#37035=CARTESIAN_POINT('Ctrl Pts',(30.4742099597326,-33.1777674171696,179.));
#37036=CARTESIAN_POINT('Ctrl Pts',(30.4427831212109,-33.1267019303825,179.));
#37037=CARTESIAN_POINT('Ctrl Pts',(30.4137899183792,-33.0742679245007,179.));
#37038=CARTESIAN_POINT('Ctrl Pts',(30.4016832373463,-33.0523730759677,179.));
#37039=CARTESIAN_POINT('Ctrl Pts',(30.3900012174127,-33.0302395674683,179.));
#37040=CARTESIAN_POINT('Ctrl Pts',(30.3787581006213,-33.0078764377137,179.));
#37041=CARTESIAN_POINT('Ctrl Pts',(30.3735598553067,-32.9975368640329,179.));
#37042=CARTESIAN_POINT('Ctrl Pts',(30.368455445269,-32.9871482050211,179.));
#37043=CARTESIAN_POINT('Ctrl Pts',(30.3634463432331,-32.9767113560277,179.));
#37044=CARTESIAN_POINT('Ctrl Pts',(30.3582116535791,-32.9658044778979,179.));
#37045=CARTESIAN_POINT('Ctrl Pts',(30.3530846523394,-32.9548524099599,179.));
#37046=CARTESIAN_POINT('Ctrl Pts',(30.3480684170179,-32.9438605003377,179.));
#37047=CARTESIAN_POINT('Ctrl Pts',(30.3195275433178,-32.8813198330565,179.));
#37048=CARTESIAN_POINT('Ctrl Pts',(30.2945476959897,-32.8174470078339,179.));
#37049=CARTESIAN_POINT('Ctrl Pts',(30.2733523004482,-32.752446851706,179.));
#37050=CARTESIAN_POINT('Ctrl Pts',(30.2541560082979,-32.6935773682653,179.));
#37051=CARTESIAN_POINT('Ctrl Pts',(30.2380642754967,-32.6337825821927,179.));
#37052=CARTESIAN_POINT('Ctrl Pts',(30.2252797403903,-32.5732098531994,179.));
#37053=CARTESIAN_POINT('Ctrl Pts',(30.2101450163511,-32.5015020022702,179.));
#37054=CARTESIAN_POINT('Ctrl Pts',(30.1996445746367,-32.4287023826296,179.));
#37055=CARTESIAN_POINT('Ctrl Pts',(30.1937033647945,-32.3552336691758,179.));
#37056=CARTESIAN_POINT('Ctrl Pts',(30.1923960684006,-32.3390677052201,179.));
#37057=CARTESIAN_POINT('Ctrl Pts',(30.1913097402832,-32.3228694274561,179.));
#37058=CARTESIAN_POINT('Ctrl Pts',(30.1904439498812,-32.3066435031514,179.));
#37059=CARTESIAN_POINT('Ctrl Pts',(30.1895460181996,-32.2898152136935,179.));
#37060=CARTESIAN_POINT('Ctrl Pts',(30.188885292102,-32.2729509603928,179.));
#37061=CARTESIAN_POINT('Ctrl Pts',(30.1884618549855,-32.2560903450774,179.));
#37062=CARTESIAN_POINT('Ctrl Pts',(30.1867401326158,-32.1875340059679,179.));
#37063=CARTESIAN_POINT('Ctrl Pts',(30.1889297256531,-32.1189513246165,179.));
#37064=CARTESIAN_POINT('Ctrl Pts',(30.1949101410477,-32.050680284215,179.));
#37065=CARTESIAN_POINT('Ctrl Pts',(30.2008893408697,-31.9824231205106,179.));
#37066=CARTESIAN_POINT('Ctrl Pts',(30.2106582755871,-31.9144764003355,179.));
#37067=CARTESIAN_POINT('Ctrl Pts',(30.224146128777,-31.8471929428052,179.));
#37068=CARTESIAN_POINT('Ctrl Pts',(30.2339040657141,-31.7985159794482,179.));
#37069=CARTESIAN_POINT('Ctrl Pts',(30.2456095194275,-31.7501864309561,179.));
#37070=CARTESIAN_POINT('Ctrl Pts',(30.2592498723843,-31.7023475393497,179.));
#37071=CARTESIAN_POINT('Ctrl Pts',(30.2694853564288,-31.6664500656337,179.));
#37072=CARTESIAN_POINT('Ctrl Pts',(30.2808105812034,-31.6308290228568,179.));
#37073=CARTESIAN_POINT('Ctrl Pts',(30.2932241308889,-31.595549108902,179.));
#37074=CARTESIAN_POINT('Ctrl Pts',(30.2973532985701,-31.5838138128595,179.));
#37075=CARTESIAN_POINT('Ctrl Pts',(30.3015996892027,-31.572125456135,179.));
#37076=CARTESIAN_POINT('Ctrl Pts',(30.3059626598347,-31.5604865933038,179.));
#37077=CARTESIAN_POINT('Ctrl Pts',(30.3290856768936,-31.4988025604527,179.));
#37078=CARTESIAN_POINT('Ctrl Pts',(30.3554815657399,-31.4385021658608,179.));
#37079=CARTESIAN_POINT('Ctrl Pts',(30.385100405382,-31.3799192305409,179.));
#37080=CARTESIAN_POINT('Ctrl Pts',(30.4059269993117,-31.3387264282618,179.));
#37081=CARTESIAN_POINT('Ctrl Pts',(30.4283479556147,-31.2983833101766,179.));
#37082=CARTESIAN_POINT('Ctrl Pts',(30.4523563132414,-31.2590172662485,179.));
#37083=CARTESIAN_POINT('Ctrl Pts',(30.4600693856112,-31.2463702892894,179.));
#37084=CARTESIAN_POINT('Ctrl Pts',(30.4679474502836,-31.233822557199,179.));
#37085=CARTESIAN_POINT('Ctrl Pts',(30.4759869645798,-31.2213839090576,179.));
#37086=CARTESIAN_POINT('Ctrl Pts',(30.5102319017654,-31.168400518695,179.));
#37087=CARTESIAN_POINT('Ctrl Pts',(30.5473331851848,-31.1175005866592,179.));
#37088=CARTESIAN_POINT('Ctrl Pts',(30.5872566410985,-31.0689991104218,179.));
#37089=CARTESIAN_POINT('Ctrl Pts',(30.6240225828063,-31.0243335771588,179.));
#37090=CARTESIAN_POINT('Ctrl Pts',(30.6631825310147,-30.9817020284588,179.));
#37091=CARTESIAN_POINT('Ctrl Pts',(30.7047312003651,-30.9413832981698,179.));
#37092=CARTESIAN_POINT('Ctrl Pts',(30.7125728983667,-30.9337737330097,179.));
#37093=CARTESIAN_POINT('Ctrl Pts',(30.7204997382999,-30.9262466564544,179.));
#37094=CARTESIAN_POINT('Ctrl Pts',(30.7285101132666,-30.9188027417083,179.));
#37095=CARTESIAN_POINT('Origin',(32.,-32.,172.));
#37096=CARTESIAN_POINT('Origin',(32.,-32.,165.));
#37097=CARTESIAN_POINT('Origin',(-32.,-32.,165.));
#37098=CARTESIAN_POINT('Origin',(-32.,32.,165.));
#37099=CARTESIAN_POINT('Origin',(32.,32.,165.));
#37100=CARTESIAN_POINT('Origin',(-32.,-32.,54.));
#37101=CARTESIAN_POINT('Ctrl Pts',(-32.6750771856749,-33.5230977622534,
54.));
#37102=CARTESIAN_POINT('Ctrl Pts',(-32.7347606773045,-33.5045114867892,
54.));
#37103=CARTESIAN_POINT('Ctrl Pts',(-32.7931316179784,-33.4823506253332,
54.));
#37104=CARTESIAN_POINT('Ctrl Pts',(-32.8500334557689,-33.4569140519098,
54.));
#37105=CARTESIAN_POINT('Ctrl Pts',(-32.88611617735,-33.4407841546612,54.));
#37106=CARTESIAN_POINT('Ctrl Pts',(-32.9216082071983,-33.4233359556206,
54.));
#37107=CARTESIAN_POINT('Ctrl Pts',(-32.9564687278967,-33.404635225715,54.));
#37108=CARTESIAN_POINT('Ctrl Pts',(-32.9802307380722,-33.3918882292444,
54.));
#37109=CARTESIAN_POINT('Ctrl Pts',(-33.0036993179247,-33.3785591155432,
54.));
#37110=CARTESIAN_POINT('Ctrl Pts',(-33.026861076465,-33.3646667567952,54.));
#37111=CARTESIAN_POINT('Ctrl Pts',(-33.0392102711152,-33.35725974398,54.));
#37112=CARTESIAN_POINT('Ctrl Pts',(-33.0514720828672,-33.3496925419692,
54.));
#37113=CARTESIAN_POINT('Ctrl Pts',(-33.0636323953525,-33.3419759097187,
54.));
#37114=CARTESIAN_POINT('Ctrl Pts',(-33.1193342204595,-33.3066289150955,
54.));
#37115=CARTESIAN_POINT('Ctrl Pts',(-33.1729722743323,-33.2681125032569,
54.));
#37116=CARTESIAN_POINT('Ctrl Pts',(-33.2243647334445,-33.2267291539377,
54.));
#37117=CARTESIAN_POINT('Ctrl Pts',(-33.2614335678882,-33.1968797839885,
54.));
#37118=CARTESIAN_POINT('Ctrl Pts',(-33.297334027751,-33.1655376472296,54.));
#37119=CARTESIAN_POINT('Ctrl Pts',(-33.3319925959414,-33.1328003832817,
54.));
#37120=CARTESIAN_POINT('Ctrl Pts',(-33.3414614125186,-33.1238564723314,
54.));
#37121=CARTESIAN_POINT('Ctrl Pts',(-33.3508375003105,-33.1148083596757,
54.));
#37122=CARTESIAN_POINT('Ctrl Pts',(-33.360119276131,-33.1056578841604,54.));
#37123=CARTESIAN_POINT('Ctrl Pts',(-33.3696833014298,-33.0962291518769,
54.));
#37124=CARTESIAN_POINT('Ctrl Pts',(-33.3791414850281,-33.0866973059031,
54.));
#37125=CARTESIAN_POINT('Ctrl Pts',(-33.3884886005182,-33.0770687715598,
54.));
#37126=CARTESIAN_POINT('Ctrl Pts',(-33.4357509408447,-33.0283834774211,
54.));
#37127=CARTESIAN_POINT('Ctrl Pts',(-33.4802063982923,-32.9771992571969,
54.));
#37128=CARTESIAN_POINT('Ctrl Pts',(-33.5216712678792,-32.9238232033015,
54.));
#37129=CARTESIAN_POINT('Ctrl Pts',(-33.5637353819771,-32.869675766121,54.));
#37130=CARTESIAN_POINT('Ctrl Pts',(-33.6027227351054,-32.8132721038918,
54.));
#37131=CARTESIAN_POINT('Ctrl Pts',(-33.6384171844749,-32.7548859058909,
54.));
#37132=CARTESIAN_POINT('Ctrl Pts',(-33.6605278962276,-32.7187189270709,
54.));
#37133=CARTESIAN_POINT('Ctrl Pts',(-33.6813745553917,-32.6817903356339,
54.));
#37134=CARTESIAN_POINT('Ctrl Pts',(-33.7008988738744,-32.6441579100733,
54.));
#37135=CARTESIAN_POINT('Ctrl Pts',(-33.716883135418,-32.6133488176477,54.));
#37136=CARTESIAN_POINT('Ctrl Pts',(-33.7319810240453,-32.5820678683706,
54.));
#37137=CARTESIAN_POINT('Ctrl Pts',(-33.7461572317173,-32.5503445540004,
54.));
#37138=CARTESIAN_POINT('Ctrl Pts',(-33.7519692674621,-32.5373384637026,
54.));
#37139=CARTESIAN_POINT('Ctrl Pts',(-33.7576272327853,-32.5242555213422,
54.));
#37140=CARTESIAN_POINT('Ctrl Pts',(-33.7631195251678,-32.5111202466595,
54.));
#37141=CARTESIAN_POINT('Ctrl Pts',(-33.7903101131696,-32.4460916907641,
54.));
#37142=CARTESIAN_POINT('Ctrl Pts',(-33.8134949920671,-32.3796713042743,
54.));
#37143=CARTESIAN_POINT('Ctrl Pts',(-33.8324625892457,-32.3121542210127,
54.));
#37144=CARTESIAN_POINT('Ctrl Pts',(-33.8345626238842,-32.304678935018,54.));
#37145=CARTESIAN_POINT('Ctrl Pts',(-33.836610926341,-32.2971901668236,54.));
#37146=CARTESIAN_POINT('Ctrl Pts',(-33.8386071814357,-32.2896882893515,
54.));
#37147=CARTESIAN_POINT('Ctrl Pts',(-33.8559453184839,-32.2245319974152,
54.));
#37148=CARTESIAN_POINT('Ctrl Pts',(-33.8693611558278,-32.1583888617247,
54.));
#37149=CARTESIAN_POINT('Ctrl Pts',(-33.8790087385963,-32.091563338769,54.));
#37150=CARTESIAN_POINT('Ctrl Pts',(-33.8893872049359,-32.0196752340216,
54.));
#37151=CARTESIAN_POINT('Ctrl Pts',(-33.8954054565889,-31.9469966406791,
54.));
#37152=CARTESIAN_POINT('Ctrl Pts',(-33.8971951234157,-31.873884038871,54.));
#37153=CARTESIAN_POINT('Ctrl Pts',(-33.8975151977,-31.8608081616469,54.));
#37154=CARTESIAN_POINT('Ctrl Pts',(-33.8976998585592,-31.8477183678653,
54.));
#37155=CARTESIAN_POINT('Ctrl Pts',(-33.8977496523165,-31.8346166621305,
54.));
#37156=CARTESIAN_POINT('Ctrl Pts',(-33.8977946179896,-31.822785319217,54.));
#37157=CARTESIAN_POINT('Ctrl Pts',(-33.8977295479978,-31.8109528682838,
54.));
#37158=CARTESIAN_POINT('Ctrl Pts',(-33.8975553940223,-31.7991242809208,
54.));
#37159=CARTESIAN_POINT('Ctrl Pts',(-33.8965091698478,-31.7280644385481,
54.));
#37160=CARTESIAN_POINT('Ctrl Pts',(-33.8915303674477,-31.6571067098811,
54.));
#37161=CARTESIAN_POINT('Ctrl Pts',(-33.8827991172353,-31.58658669665,54.));
#37162=CARTESIAN_POINT('Ctrl Pts',(-33.8738836330992,-31.5145786744368,
54.));
#37163=CARTESIAN_POINT('Ctrl Pts',(-33.8610557270815,-31.4430260992478,
54.));
#37164=CARTESIAN_POINT('Ctrl Pts',(-33.8444544762436,-31.3722700783463,
54.));
#37165=CARTESIAN_POINT('Ctrl Pts',(-33.8277523080762,-31.30108393873,54.));
#37166=CARTESIAN_POINT('Ctrl Pts',(-33.8072307013535,-31.230702996705,54.));
#37167=CARTESIAN_POINT('Ctrl Pts',(-33.7829788829121,-31.1614736899745,
54.));
#37168=CARTESIAN_POINT('Ctrl Pts',(-33.7769978633042,-31.1444002551724,
54.));
#37169=CARTESIAN_POINT('Ctrl Pts',(-33.7707897192942,-31.1273969048688,
54.));
#37170=CARTESIAN_POINT('Ctrl Pts',(-33.7643553120831,-31.110468945581,54.));
#37171=CARTESIAN_POINT('Ctrl Pts',(-33.759286336738,-31.0971332325215,54.));
#37172=CARTESIAN_POINT('Ctrl Pts',(-33.7540761635107,-31.0838427060458,
54.));
#37173=CARTESIAN_POINT('Ctrl Pts',(-33.7487336536153,-31.0706201630216,
54.));
#37174=CARTESIAN_POINT('Ctrl Pts',(-33.7205084795823,-31.000763749964,54.));
#37175=CARTESIAN_POINT('Ctrl Pts',(-33.6885470726678,-30.9326782822882,
54.));
#37176=CARTESIAN_POINT('Ctrl Pts',(-33.6530075396668,-30.8667211000107,
54.));
#37177=CARTESIAN_POINT('Ctrl Pts',(-33.6174289999564,-30.8006915258803,
54.));
#37178=CARTESIAN_POINT('Ctrl Pts',(-33.5782643040916,-30.7367937961817,
54.));
#37179=CARTESIAN_POINT('Ctrl Pts',(-33.5356203132441,-30.6753908521558,
54.));
#37180=CARTESIAN_POINT('Ctrl Pts',(-33.4939464409215,-30.6153847786457,
54.));
#37181=CARTESIAN_POINT('Ctrl Pts',(-33.4489494371178,-30.5577602901018,
54.));
#37182=CARTESIAN_POINT('Ctrl Pts',(-33.4006836999752,-30.5028757358465,
54.));
#37183=CARTESIAN_POINT('Ctrl Pts',(-33.3903485119752,-30.4911232542703,
54.));
#37184=CARTESIAN_POINT('Ctrl Pts',(-33.3798632874165,-30.4794965079344,
54.));
#37185=CARTESIAN_POINT('Ctrl Pts',(-33.3692283040305,-30.4679992023154,
54.));
#37186=CARTESIAN_POINT('Ctrl Pts',(-33.3601172578224,-30.4581494001143,
54.));
#37187=CARTESIAN_POINT('Ctrl Pts',(-33.3508962951961,-30.4483946015766,
54.));
#37188=CARTESIAN_POINT('Ctrl Pts',(-33.3415672767799,-30.4387352221184,
54.));
#37189=CARTESIAN_POINT('Ctrl Pts',(-32.3836679988468,-29.9813874990081,
54.));
#37190=CARTESIAN_POINT('Ctrl Pts',(-32.3093502868603,-29.9743669052867,
54.));
#37191=CARTESIAN_POINT('Ctrl Pts',(-32.2347844751733,-29.9717482530017,
54.));
#37192=CARTESIAN_POINT('Ctrl Pts',(-32.1602926808089,-29.9733679476272,
54.));
#37193=CARTESIAN_POINT('Ctrl Pts',(-32.0877589921938,-29.9749450666458,
54.));
#37194=CARTESIAN_POINT('Ctrl Pts',(-32.0152946982106,-29.9805412908907,
54.));
#37195=CARTESIAN_POINT('Ctrl Pts',(-31.9432103771728,-29.9900494467721,
54.));
#37196=CARTESIAN_POINT('Ctrl Pts',(-31.9271201986695,-29.9921717935344,
54.));
#37197=CARTESIAN_POINT('Ctrl Pts',(-31.9110468988445,-29.9944895420622,
54.));
#37198=CARTESIAN_POINT('Ctrl Pts',(-31.895000900343,-29.9970006837775,54.));
#37199=CARTESIAN_POINT('Ctrl Pts',(-31.8213673331251,-30.0085240752489,
54.));
#37200=CARTESIAN_POINT('Ctrl Pts',(-31.7484534163863,-30.0240919768973,
54.));
#37201=CARTESIAN_POINT('Ctrl Pts',(-31.6765910828333,-30.0435648983486,
54.));
#37202=CARTESIAN_POINT('Ctrl Pts',(-31.6261438372765,-30.0572348586962,
54.));
#37203=CARTESIAN_POINT('Ctrl Pts',(-31.5762150877003,-30.072830311071,54.));
#37204=CARTESIAN_POINT('Ctrl Pts',(-31.5269276035993,-30.0903161409675,
54.));
#37205=CARTESIAN_POINT('Ctrl Pts',(-31.5082001964427,-30.0969601046819,
54.));
#37206=CARTESIAN_POINT('Ctrl Pts',(-31.4895654530443,-30.1038770881373,
54.));
#37207=CARTESIAN_POINT('Ctrl Pts',(-31.4710304416861,-30.1110655275264,
54.));
#37208=CARTESIAN_POINT('Ctrl Pts',(-31.4533429018407,-30.1179252917674,
54.));
#37209=CARTESIAN_POINT('Ctrl Pts',(-31.4357407210111,-30.1250347094918,
54.));
#37210=CARTESIAN_POINT('Ctrl Pts',(-31.4182609553468,-30.1323791943156,
54.));
#37211=CARTESIAN_POINT('Ctrl Pts',(-31.3513338021807,-30.160500021,54.));
#37212=CARTESIAN_POINT('Ctrl Pts',(-31.2861267740855,-30.1920888911457,
54.));
#37213=CARTESIAN_POINT('Ctrl Pts',(-31.2229480770285,-30.2270186551939,
54.));
#37214=CARTESIAN_POINT('Ctrl Pts',(-31.1611263845489,-30.2611981687319,
54.));
#37215=CARTESIAN_POINT('Ctrl Pts',(-31.1012461299126,-30.2985772270485,
54.));
#37216=CARTESIAN_POINT('Ctrl Pts',(-31.0436284472419,-30.3390735157394,
54.));
#37217=CARTESIAN_POINT('Ctrl Pts',(-30.9872742147514,-30.3786817950404,
54.));
#37218=CARTESIAN_POINT('Ctrl Pts',(-30.9330838522464,-30.4212726194304,
54.));
#37219=CARTESIAN_POINT('Ctrl Pts',(-30.8813982632594,-30.46679619445,54.));
#37220=CARTESIAN_POINT('Ctrl Pts',(-30.8645714248051,-30.4816169183254,
54.));
#37221=CARTESIAN_POINT('Ctrl Pts',(-30.848010428094,-30.4967486715566,54.));
#37222=CARTESIAN_POINT('Ctrl Pts',(-30.831728140297,-30.512190239164,54.));
#37223=CARTESIAN_POINT('Ctrl Pts',(-30.8225975381376,-30.5208493915078,
54.));
#37224=CARTESIAN_POINT('Ctrl Pts',(-30.8135537587495,-30.5296069313898,
54.));
#37225=CARTESIAN_POINT('Ctrl Pts',(-30.8046115260975,-30.5384500275864,
54.));
#37226=CARTESIAN_POINT('Ctrl Pts',(-30.7560460841086,-30.5864770575297,
54.));
#37227=CARTESIAN_POINT('Ctrl Pts',(-30.7103849485071,-30.6371066388124,
54.));
#37228=CARTESIAN_POINT('Ctrl Pts',(-30.6679204829488,-30.6902577823286,
54.));
#37229=CARTESIAN_POINT('Ctrl Pts',(-30.6618145456302,-30.697900349978,54.));
#37230=CARTESIAN_POINT('Ctrl Pts',(-30.6557747732231,-30.7055951018378,
54.));
#37231=CARTESIAN_POINT('Ctrl Pts',(-30.6498021107534,-30.7133418456573,
54.));
#37232=CARTESIAN_POINT('Ctrl Pts',(-30.6074436402858,-30.7682822044938,
54.));
#37233=CARTESIAN_POINT('Ctrl Pts',(-30.568456554529,-30.8258362406613,54.));
#37234=CARTESIAN_POINT('Ctrl Pts',(-30.5329080920352,-30.8856417419126,
54.));
#37235=CARTESIAN_POINT('Ctrl Pts',(-30.4997462572144,-30.9414320634833,
54.));
#37236=CARTESIAN_POINT('Ctrl Pts',(-30.4695772268648,-30.9991826610177,
54.));
#37237=CARTESIAN_POINT('Ctrl Pts',(-30.4424952980961,-31.058604931198,54.));
#37238=CARTESIAN_POINT('Ctrl Pts',(-30.4366014843027,-31.0715369420091,
54.));
#37239=CARTESIAN_POINT('Ctrl Pts',(-30.4308540294333,-31.0845481194749,
54.));
#37240=CARTESIAN_POINT('Ctrl Pts',(-30.4252541510133,-31.0976354614338,
54.));
#37241=CARTESIAN_POINT('Ctrl Pts',(-30.4207268514394,-31.1082161050176,
54.));
#37242=CARTESIAN_POINT('Ctrl Pts',(-30.4162962339789,-31.1188462321919,
54.));
#37243=CARTESIAN_POINT('Ctrl Pts',(-30.4119679662711,-31.1295112213537,
54.));
#37244=CARTESIAN_POINT('Ctrl Pts',(-30.3862551907436,-31.1928683172718,
54.));
#37245=CARTESIAN_POINT('Ctrl Pts',(-30.3640997107775,-31.2575711336523,
54.));
#37246=CARTESIAN_POINT('Ctrl Pts',(-30.3455477942828,-31.3232696018123,
54.));
#37247=CARTESIAN_POINT('Ctrl Pts',(-30.3270815170559,-31.3886647930192,
54.));
#37248=CARTESIAN_POINT('Ctrl Pts',(-30.3121856030553,-31.4550476008397,
54.));
#37249=CARTESIAN_POINT('Ctrl Pts',(-30.3009567442566,-31.5220754131288,
54.));
#37250=CARTESIAN_POINT('Ctrl Pts',(-30.289968467501,-31.5876671321944,54.));
#37251=CARTESIAN_POINT('Ctrl Pts',(-30.2824919234282,-31.6538774769525,
54.));
#37252=CARTESIAN_POINT('Ctrl Pts',(-30.27866560992,-31.7203725063053,54.));
#37253=CARTESIAN_POINT('Ctrl Pts',(-30.2775523112949,-31.7397198035387,
54.));
#37254=CARTESIAN_POINT('Ctrl Pts',(-30.2767483380266,-31.7590910662344,
54.));
#37255=CARTESIAN_POINT('Ctrl Pts',(-30.2762578628063,-31.7784776822845,
54.));
#37256=CARTESIAN_POINT('Ctrl Pts',(-30.2759857202441,-31.7892344405202,
54.));
#37257=CARTESIAN_POINT('Ctrl Pts',(-30.2758103453474,-31.7999861747191,
54.));
#37258=CARTESIAN_POINT('Ctrl Pts',(-30.2757319690388,-31.8107314277276,
54.));
#37259=CARTESIAN_POINT('Ctrl Pts',(-30.2752558284876,-31.8760094534826,
54.));
#37260=CARTESIAN_POINT('Ctrl Pts',(-30.2783554819153,-31.9410502912499,
54.));
#37261=CARTESIAN_POINT('Ctrl Pts',(-30.2851111645757,-32.005544110067,54.));
#37262=CARTESIAN_POINT('Ctrl Pts',(-30.2920241952358,-32.0715400677344,
54.));
#37263=CARTESIAN_POINT('Ctrl Pts',(-30.3027653449035,-32.1369643722245,
54.));
#37264=CARTESIAN_POINT('Ctrl Pts',(-30.3174745232328,-32.2014643058222,
54.));
#37265=CARTESIAN_POINT('Ctrl Pts',(-30.3311068192429,-32.261242096787,54.));
#37266=CARTESIAN_POINT('Ctrl Pts',(-30.3481479568216,-32.3202263605165,
54.));
#37267=CARTESIAN_POINT('Ctrl Pts',(-30.3687510889275,-32.3781081209656,
54.));
#37268=CARTESIAN_POINT('Ctrl Pts',(-30.3703786319819,-32.3826804867937,
54.));
#37269=CARTESIAN_POINT('Ctrl Pts',(-30.3720284233314,-32.3872459552685,
54.));
#37270=CARTESIAN_POINT('Ctrl Pts',(-30.3737005491397,-32.3918043647069,
54.));
#37271=CARTESIAN_POINT('Ctrl Pts',(-30.377463203204,-32.4020617973208,54.));
#37272=CARTESIAN_POINT('Ctrl Pts',(-30.3813389467107,-32.4122834887951,
54.));
#37273=CARTESIAN_POINT('Ctrl Pts',(-30.3853267233299,-32.4224680762713,
54.));
#37274=CARTESIAN_POINT('Origin',(-32.,-32.,39.4540747194623));
#37275=CARTESIAN_POINT('Ctrl Pts',(-29.9434322372613,-31.9985074052702,
41.2040747194623));
#37276=CARTESIAN_POINT('Ctrl Pts',(-29.9426158455512,-31.9004173014865,
41.2094078928854));
#37277=CARTESIAN_POINT('Ctrl Pts',(-29.9935881722041,-31.121837189222,41.2517843293816));
#37278=CARTESIAN_POINT('Ctrl Pts',(-30.9882785852064,-29.7919911926234,
41.3312040289512));
#37279=CARTESIAN_POINT('Ctrl Pts',(-33.3060692951901,-29.9526095058617,
41.4423338181709));
#37280=CARTESIAN_POINT('Ctrl Pts',(-34.4285436397314,-31.9866292178594,
41.5534636073906));
#37281=CARTESIAN_POINT('Ctrl Pts',(-33.3284492207144,-34.0330616120671,
41.6645933966103));
#37282=CARTESIAN_POINT('Ctrl Pts',(-31.0125684200493,-34.218769212662,41.7757231858301));
#37283=CARTESIAN_POINT('Ctrl Pts',(-29.9981580665322,-32.8935770673079,
41.8555502934473));
#37284=CARTESIAN_POINT('Ctrl Pts',(-29.9427300189926,-32.1072436601885,
41.8983341379914));
#37285=CARTESIAN_POINT('Ctrl Pts',(-29.9436380165453,-32.001608018912,41.9040747194623));
#37286=CARTESIAN_POINT('Ctrl Pts',(-29.9473238289665,-32.0023603893952,
41.1459252805377));
#37287=CARTESIAN_POINT('Ctrl Pts',(-29.950874167023,-31.5322379170384,41.171370046505));
#37288=CARTESIAN_POINT('Ctrl Pts',(-30.3433200420557,-30.3706660396747,
41.2338580755455));
#37289=CARTESIAN_POINT('Ctrl Pts',(-32.2715961806528,-29.5872035622868,
41.3333893676592));
#37290=CARTESIAN_POINT('Ctrl Pts',(-34.1743722595742,-30.9184415569553,
41.444519156879));
#37291=CARTESIAN_POINT('Ctrl Pts',(-34.0880140492357,-33.2405968969734,
41.5556489460986));
#37292=CARTESIAN_POINT('Ctrl Pts',(-32.090310165188,-34.4268231234318,41.6667787353184));
#37293=CARTESIAN_POINT('Ctrl Pts',(-30.279165136739,-33.5261027188181,41.7635375134647));
#37294=CARTESIAN_POINT('Ctrl Pts',(-29.95009226531,-32.4182605833851,41.8232530285378));
#37295=CARTESIAN_POINT('Ctrl Pts',(-29.9479126462767,-31.9988339667449,
41.8459252805377));
#37296=CARTESIAN_POINT('Ctrl Pts',(-33.2690708798524,-30.9206413469515,
41.));
#37297=CARTESIAN_POINT('Ctrl Pts',(-33.6279571482407,-31.3426068457263,
41.0370432630732));
#37298=CARTESIAN_POINT('Ctrl Pts',(-33.8852968192855,-32.5656196832009,
41.1111297892197));
#37299=CARTESIAN_POINT('Ctrl Pts',(-32.5453396492552,-33.8933251529091,
41.2222595784395));
#37300=CARTESIAN_POINT('Ctrl Pts',(-30.7061567832839,-33.4837760673271,
41.3333893676592));
#37301=CARTESIAN_POINT('Ctrl Pts',(-30.0511799688433,-31.7184951900074,
41.4445191568789));
#37302=CARTESIAN_POINT('Ctrl Pts',(-31.1796919931641,-30.2097371100672,
41.5556489460986));
#37303=CARTESIAN_POINT('Ctrl Pts',(-33.0589665145573,-30.3399671185134,
41.6667787353183));
#37304=CARTESIAN_POINT('Ctrl Pts',(-33.9690734657708,-31.9891589132273,
41.7779085245381));
#37305=CARTESIAN_POINT('Ctrl Pts',(-33.0771122529311,-33.6484149632334,
41.8890383137578));
#37306=CARTESIAN_POINT('Ctrl Pts',(-31.1993862941002,-33.7989874720987,
42.0001681029776));
#37307=CARTESIAN_POINT('Ctrl Pts',(-30.0543749801228,-32.3031825501919,
42.1112978921972));
#37308=CARTESIAN_POINT('Ctrl Pts',(-30.6899777445458,-30.5298898605771,
42.222427681417));
#37309=CARTESIAN_POINT('Ctrl Pts',(-32.5244990950944,-30.1020353158865,
42.3335574706367));
#37310=CARTESIAN_POINT('Ctrl Pts',(-33.8790043473039,-31.4111727754414,
42.4446872598565));
#37311=CARTESIAN_POINT('Ctrl Pts',(-33.513865306157,-33.25920089568,42.5558170490762));
#37312=CARTESIAN_POINT('Ctrl Pts',(-31.7632530992687,-33.9548208142199,
42.6669468382959));
#37313=CARTESIAN_POINT('Ctrl Pts',(-30.2293091161659,-32.8614105276525,
42.7780766275156));
#37314=CARTESIAN_POINT('Ctrl Pts',(-30.3158822136371,-30.9796463621952,
42.8892064167354));
#37315=CARTESIAN_POINT('Ctrl Pts',(-31.9437416527471,-30.0316989351598,
43.0003362059551));
#37316=CARTESIAN_POINT('Ctrl Pts',(-33.6230881176018,-30.885119219342,43.1114659951748));
#37317=CARTESIAN_POINT('Ctrl Pts',(-33.8170019406859,-32.7588663430016,
43.2225957843946));
#37318=CARTESIAN_POINT('Ctrl Pts',(-32.34801529131,-33.938107199206,43.3337255736143));
#37319=CARTESIAN_POINT('Ctrl Pts',(-30.5605288218555,-33.343613374649,43.444855362834));
#37320=CARTESIAN_POINT('Ctrl Pts',(-30.0904307639918,-31.5194591554142,
43.5559851520537));
#37321=CARTESIAN_POINT('Ctrl Pts',(-31.367949762624,-30.1350907084618,43.6671149412734));
#37322=CARTESIAN_POINT('Ctrl Pts',(-33.2239142841442,-30.4574670197298,
43.7782447304932));
#37323=CARTESIAN_POINT('Ctrl Pts',(-33.9597657256432,-32.1915527871223,
43.8893745197128));
#37324=CARTESIAN_POINT('Ctrl Pts',(-32.9020608277928,-33.7503315207131,
44.0005043089327));
#37325=CARTESIAN_POINT('Ctrl Pts',(-31.0187996427964,-33.7072258282694,
44.1116340981523));
#37326=CARTESIAN_POINT('Ctrl Pts',(-30.0335223840341,-32.1016855718022,
44.2227638873721));
#37327=CARTESIAN_POINT('Ctrl Pts',(-30.847944113844,-30.4030837827984,44.3338936765918));
#37328=CARTESIAN_POINT('Ctrl Pts',(-32.7167148971371,-30.1659623979207,
44.4450234658116));
#37329=CARTESIAN_POINT('Ctrl Pts',(-33.9295559790202,-31.6073323371673,
44.5561532550312));
#37330=CARTESIAN_POINT('Ctrl Pts',(-33.376488354067,-33.4080674631294,44.667283044251));
#37331=CARTESIAN_POINT('Ctrl Pts',(-31.5636735148665,-33.920154516694,44.7784128334707));
#37332=CARTESIAN_POINT('Ctrl Pts',(-30.1501799430964,-32.6749369797875,
44.8895426226904));
#37333=CARTESIAN_POINT('Ctrl Pts',(-30.4296216269414,-30.812024438367,45.0006724119102));
#37334=CARTESIAN_POINT('Ctrl Pts',(-32.1462565677652,-30.0363342478941,
45.1118022011299));
#37335=CARTESIAN_POINT('Ctrl Pts',(-33.7290390838569,-31.0577696586804,
45.2229319903496));
#37336=CARTESIAN_POINT('Ctrl Pts',(-33.7294237810507,-32.9415240597797,
45.3340617795693));
#37337=CARTESIAN_POINT('Ctrl Pts',(-32.1470585886469,-33.963605851772,45.4451915687891));
#37338=CARTESIAN_POINT('Ctrl Pts',(-30.4301069706974,-33.1886168626412,
45.5563213580088));
#37339=CARTESIAN_POINT('Ctrl Pts',(-30.1499044283847,-31.3258186108344,
45.6674511472285));
#37340=CARTESIAN_POINT('Ctrl Pts',(-31.5628892897633,-30.0800238551992,
45.7785809364483));
#37341=CARTESIAN_POINT('Ctrl Pts',(-33.3759131328822,-30.5913704460114,
45.889710725668));
#37342=CARTESIAN_POINT('Ctrl Pts',(-33.929716197944,-32.3918795286826,46.0008405148877));
#37343=CARTESIAN_POINT('Ctrl Pts',(-32.7174639255481,-33.83374471646,46.1119703041074));
#37344=CARTESIAN_POINT('Ctrl Pts',(-30.8485964490629,-33.5973866258666,
46.2231000933272));
#37345=CARTESIAN_POINT('Ctrl Pts',(-30.0334810159438,-31.8991176182166,
46.3342298825469));
#37346=CARTESIAN_POINT('Ctrl Pts',(-31.0181024310225,-30.293175072351,46.4453596717666));
#37347=CARTESIAN_POINT('Ctrl Pts',(-32.9013458529938,-30.2493001905241,
46.5564894609864));
#37348=CARTESIAN_POINT('Ctrl Pts',(-33.9596873249938,-31.8076467887807,
46.6676192502061));
#37349=CARTESIAN_POINT('Ctrl Pts',(-33.2245442090837,-33.5420329599615,
46.7787490394258));
#37350=CARTESIAN_POINT('Ctrl Pts',(-31.3687115126491,-33.8651672888366,
46.8898788286455));
#37351=CARTESIAN_POINT('Ctrl Pts',(-30.0906271937995,-32.4813207418654,
47.0010086178652));
#37352=CARTESIAN_POINT('Ctrl Pts',(-30.5599801608987,-30.6569746716451,
47.112138407085));
#37353=CARTESIAN_POINT('Ctrl Pts',(-32.3472236683786,-30.061750817432,47.2232681963047));
#37354=CARTESIAN_POINT('Ctrl Pts',(-33.8166918400422,-31.2403915956679,
47.3343979855244));
#37355=CARTESIAN_POINT('Ctrl Pts',(-33.6235433409019,-33.1142177479385,
47.4455277747442));
#37356=CARTESIAN_POINT('Ctrl Pts',(-31.9445455827624,-33.9683239004841,
47.5566575639638));
#37357=CARTESIAN_POINT('Ctrl Pts',(-30.3162991059008,-33.0210413648905,
47.6677873531837));
#37358=CARTESIAN_POINT('Ctrl Pts',(-30.2289574283427,-31.1393128448816,
47.7789171424033));
#37359=CARTESIAN_POINT('Ctrl Pts',(-31.7624547062086,-30.0452758754736,
47.8900469316231));
#37360=CARTESIAN_POINT('Ctrl Pts',(-33.5133508608809,-30.7401812267317,
48.0011767208428));
#37361=CARTESIAN_POINT('Ctrl Pts',(-33.8792447192816,-32.5880590571192,
48.1123065100625));
#37362=CARTESIAN_POINT('Ctrl Pts',(-32.5252741901563,-33.8977516156662,
48.2234362992822));
#37363=CARTESIAN_POINT('Ctrl Pts',(-30.6905784185613,-33.4706424758147,
48.334566088502));
#37364=CARTESIAN_POINT('Ctrl Pts',(-30.0542510782132,-31.6976172905512,
48.4456958777217));
#37365=CARTESIAN_POINT('Ctrl Pts',(-31.1986520503161,-30.2013294817713,
48.5568256669414));
#37366=CARTESIAN_POINT('Ctrl Pts',(-33.076437975713,-30.3511654255047,48.6679554561611));
#37367=CARTESIAN_POINT('Ctrl Pts',(-33.9690795392212,-32.0099968909499,
48.7790852453809));
#37368=CARTESIAN_POINT('Ctrl Pts',(-33.0596408622125,-33.6596793102095,
48.8902150346006));
#37369=CARTESIAN_POINT('Ctrl Pts',(-31.1804303594337,-33.790441223238,49.0013448238204));
#37370=CARTESIAN_POINT('Ctrl Pts',(-30.0512811038385,-32.2826107452856,
49.11247461304));
#37371=CARTESIAN_POINT('Ctrl Pts',(-30.7055782490339,-30.5161379780338,
49.2236044022598));
#37372=CARTESIAN_POINT('Ctrl Pts',(-32.5445161432941,-30.1076796414719,
49.3347341914795));
#37373=CARTESIAN_POINT('Ctrl Pts',(-33.8851187682433,-31.4310523756752,
49.4458639806993));
#37374=CARTESIAN_POINT('Ctrl Pts',(-33.5004811397579,-33.2751198056805,
49.5569937699189));
#37375=CARTESIAN_POINT('Ctrl Pts',(-31.7426194442066,-33.9522114176255,
49.6681235591387));
#37376=CARTESIAN_POINT('Ctrl Pts',(-30.2203096421414,-32.8426603110109,
49.7792533483584));
#37377=CARTESIAN_POINT('Ctrl Pts',(-30.3267531556502,-30.9619156260297,
49.8903831375781));
#37378=CARTESIAN_POINT('Ctrl Pts',(-31.9645340355014,-30.0312145025498,
50.0015129267979));
#37379=CARTESIAN_POINT('Ctrl Pts',(-33.6347729814496,-30.9023245157467,
50.1126427160176));
#37380=CARTESIAN_POINT('Ctrl Pts',(-33.8088854231495,-32.7780152283373,
50.2237725052373));
#37381=CARTESIAN_POINT('Ctrl Pts',(-32.327525542129,-33.9416748411773,50.3349022944571));
#37382=CARTESIAN_POINT('Ctrl Pts',(-30.546417836818,-33.328334695959,50.4460320836767));
#37383=CARTESIAN_POINT('Ctrl Pts',(-30.0956127638102,-31.4993170421883,
50.5571618728965));
#37384=CARTESIAN_POINT('Ctrl Pts',(-31.3876822371413,-30.1285190017276,
50.6682916621162));
#37385=CARTESIAN_POINT('Ctrl Pts',(-33.2401382867359,-30.470480075517,50.779421451336));
#37386=CARTESIAN_POINT('Ctrl Pts',(-33.9576332250398,-32.2122411972453,
50.8905512405557));
#37387=CARTESIAN_POINT('Ctrl Pts',(-32.8835234654548,-33.7597614769049,
51.0016810297755));
#37388=CARTESIAN_POINT('Ctrl Pts',(-31.0008226116605,-33.6967671367391,
51.1128108189951));
#37389=CARTESIAN_POINT('Ctrl Pts',(-30.0325580681222,-32.0809099136646,
51.2239406082149));
#37390=CARTESIAN_POINT('Ctrl Pts',(-30.8648750444701,-30.3910048151118,
51.3350703974346));
#37391=CARTESIAN_POINT('Ctrl Pts',(-32.7360460704965,-30.1736346607921,
51.4462001866543));
#37392=CARTESIAN_POINT('Ctrl Pts',(-33.9335957143077,-31.6277342591057,
51.557329975874));
#37393=CARTESIAN_POINT('Ctrl Pts',(-33.3615395305129,-33.4225274258428,
51.6684597650937));
#37394=CARTESIAN_POINT('Ctrl Pts',(-31.5434171313856,-33.9154389202823,
51.7795895543135));
#37395=CARTESIAN_POINT('Ctrl Pts',(-30.1431544267094,-32.655361484641,51.8907193435332));
#37396=CARTESIAN_POINT('Ctrl Pts',(-30.4422566450893,-30.7955043299255,
52.001849132753));
#37397=CARTESIAN_POINT('Ctrl Pts',(-32.1669887066119,-30.0379885412045,
52.1129789219726));
#37398=CARTESIAN_POINT('Ctrl Pts',(-33.738894479621,-31.0760843803515,52.2241087111924));
#37399=CARTESIAN_POINT('Ctrl Pts',(-33.7193829519648,-32.9597377397069,
52.3352385004121));
#37400=CARTESIAN_POINT('Ctrl Pts',(-32.126310654911,-33.9650495977709,52.4463682896319));
#37401=CARTESIAN_POINT('Ctrl Pts',(-30.4176404888248,-33.1719692351367,
52.5574980788516));
#37402=CARTESIAN_POINT('Ctrl Pts',(-30.1571280478576,-31.3063156129234,
52.6686278680713));
#37403=CARTESIAN_POINT('Ctrl Pts',(-31.5831931003876,-30.0755138748217,
52.779757657291));
#37404=CARTESIAN_POINT('Ctrl Pts',(-33.3907131932281,-30.6059820456399,
52.8908874465108));
#37405=CARTESIAN_POINT('Ctrl Pts',(-33.9254718382176,-32.4122381981941,
53.0020172357305));
#37406=CARTESIAN_POINT('Ctrl Pts',(-32.6980512536445,-33.8412226437882,
53.1131470249502));
#37407=CARTESIAN_POINT('Ctrl Pts',(-30.8317981301991,-33.5851317365559,
53.2242768141699));
#37408=CARTESIAN_POINT('Ctrl Pts',(-30.0346382286355,-31.87836199572,53.3354066033897));
#37409=CARTESIAN_POINT('Ctrl Pts',(-31.0362203629822,-30.2828812929693,
53.4465363926094));
#37410=CARTESIAN_POINT('Ctrl Pts',(-32.9197159734883,-30.2589538275277,
53.5576661818291));
#37411=CARTESIAN_POINT('Ctrl Pts',(-33.9617492885598,-31.8282846250777,
53.6687959710488));
#37412=CARTESIAN_POINT('Ctrl Pts',(-33.207912453419,-33.5550215357871,53.7799257602685));
#37413=CARTESIAN_POINT('Ctrl Pts',(-31.3495946578974,-33.8581158678563,
53.8910555494883));
#37414=CARTESIAN_POINT('Ctrl Pts',(-30.0845579730524,-32.461689624197,54.002185338708));
#37415=CARTESIAN_POINT('Ctrl Pts',(-30.5764960032975,-30.6406229021335,
54.1133151279277));
#37416=CARTESIAN_POINT('Ctrl Pts',(-31.7668777668624,-30.2598665970073,
54.1874016540742));
#37417=CARTESIAN_POINT('Ctrl Pts',(-32.3110796379505,-30.3633004372052,
54.2244449171475));
#37418=CARTESIAN_POINT('Ctrl Pts',(-33.3677806246589,-30.8366876301903,
40.9251850276175));
#37419=CARTESIAN_POINT('Ctrl Pts',(-33.7545814662436,-31.2914740748731,
40.9622282906908));
#37420=CARTESIAN_POINT('Ctrl Pts',(-34.0319373031784,-32.609614211381,41.0363148168372));
#37421=CARTESIAN_POINT('Ctrl Pts',(-32.5877567738346,-34.0405900895225,
41.147444606057));
#37422=CARTESIAN_POINT('Ctrl Pts',(-30.6055202185583,-33.599185820463,41.2585743952767));
#37423=CARTESIAN_POINT('Ctrl Pts',(-29.8995985788648,-31.6965994327276,
41.3697041844964));
#37424=CARTESIAN_POINT('Ctrl Pts',(-31.1158875238449,-30.0704884709193,
41.4808339737161));
#37425=CARTESIAN_POINT('Ctrl Pts',(-33.1413341081016,-30.2108479142962,
41.5919637629359));
#37426=CARTESIAN_POINT('Ctrl Pts',(-34.1222301904244,-31.988315681438,41.7030935521556));
#37427=CARTESIAN_POINT('Ctrl Pts',(-33.1608912421922,-33.7766305128446,
41.8142233413753));
#37428=CARTESIAN_POINT('Ctrl Pts',(-31.1371136694165,-33.9389147189532,
41.925353130595));
#37429=CARTESIAN_POINT('Ctrl Pts',(-29.903042101676,-32.3267644262197,42.0364829198148));
#37430=CARTESIAN_POINT('Ctrl Pts',(-30.5880827561889,-30.4155430585161,
42.1476127090345));
#37431=CARTESIAN_POINT('Ctrl Pts',(-32.5652952181873,-29.9544095113748,
42.2587424982543));
#37432=CARTESIAN_POINT('Ctrl Pts',(-34.0251553957261,-31.3653731388774,
42.3698722874739));
#37433=CARTESIAN_POINT('Ctrl Pts',(-33.6316154337617,-33.3571429421376,
42.4810020766937));
#37434=CARTESIAN_POINT('Ctrl Pts',(-31.7448386619619,-34.1068689517806,
42.5921318659134));
#37435=CARTESIAN_POINT('Ctrl Pts',(-30.0915828094251,-32.928411996765,42.7032616551332));
#37436=CARTESIAN_POINT('Ctrl Pts',(-30.1848896587255,-30.9002821211595,
42.8143914443528));
#37437=CARTESIAN_POINT('Ctrl Pts',(-31.9393658159135,-29.8786022887098,
42.9255212335726));
#37438=CARTESIAN_POINT('Ctrl Pts',(-33.7493337169851,-30.7984025519789,
43.0366510227924));
#37439=CARTESIAN_POINT('Ctrl Pts',(-33.9583303729471,-32.8178918113572,
43.147780812012));
#37440=CARTESIAN_POINT('Ctrl Pts',(-32.3750843078159,-34.088855333198,43.2589106012318));
#37441=CARTESIAN_POINT('Ctrl Pts',(-30.4485651522869,-33.4481211176251,
43.3700403904515));
#37442=CARTESIAN_POINT('Ctrl Pts',(-29.9419023445243,-31.4820821539471,
43.4811701796712));
#37443=CARTESIAN_POINT('Ctrl Pts',(-31.3187881920398,-29.990035989157,43.5922999688909));
#37444=CARTESIAN_POINT('Ctrl Pts',(-33.3191116987022,-30.3374870885413,
43.7034297581107));
#37445=CARTESIAN_POINT('Ctrl Pts',(-34.1121984839153,-32.2064519759966,
43.8145595473304));
#37446=CARTESIAN_POINT('Ctrl Pts',(-32.9722241224715,-33.8864742535418,
43.9256893365502));
#37447=CARTESIAN_POINT('Ctrl Pts',(-30.9424807874817,-33.840015752387,44.0368191257698));
#37448=CARTESIAN_POINT('Ctrl Pts',(-29.8805675674661,-32.1095947886966,
44.1479489149896));
#37449=CARTESIAN_POINT('Ctrl Pts',(-30.75833592542,-30.278873862943,44.2590787042093));
#37450=CARTESIAN_POINT('Ctrl Pts',(-32.7724617791423,-30.0233089129651,
44.370208493429));
#37451=CARTESIAN_POINT('Ctrl Pts',(-34.0796389895932,-31.576790209531,44.4813382826488));
#37452=CARTESIAN_POINT('Ctrl Pts',(-33.4835531495139,-33.5175885168092,
44.5924680718685));
#37453=CARTESIAN_POINT('Ctrl Pts',(-31.5297355554636,-34.0695062710687,
44.7035978610883));
#37454=CARTESIAN_POINT('Ctrl Pts',(-30.0062988812474,-32.7274343289057,
44.8147276503079));
#37455=CARTESIAN_POINT('Ctrl Pts',(-30.3074758501253,-30.7196223776258,
44.9258574395277));
#37456=CARTESIAN_POINT('Ctrl Pts',(-32.1576325663084,-29.8835981412252,
45.0369872287474));
#37457=CARTESIAN_POINT('Ctrl Pts',(-33.8635256672601,-30.9844819345531,
45.1481170179671));
#37458=CARTESIAN_POINT('Ctrl Pts',(-33.8639402866296,-33.0147568485431,
45.2592468071869));
#37459=CARTESIAN_POINT('Ctrl Pts',(-32.1584969692665,-34.1163372993263,
45.3703765964066));
#37460=CARTESIAN_POINT('Ctrl Pts',(-30.3079989444586,-33.2810688044883,
45.4815063856263));
#37461=CARTESIAN_POINT('Ctrl Pts',(-30.0060019366949,-31.2733800323954,
45.592636174846));
#37462=CARTESIAN_POINT('Ctrl Pts',(-31.5288903324594,-29.9306859747887,
45.7037659640658));
#37463=CARTESIAN_POINT('Ctrl Pts',(-33.4829331869855,-30.4818056722793,
45.8148957532855));
#37464=CARTESIAN_POINT('Ctrl Pts',(-34.0798116705231,-32.4223603543679,
45.9260255425052));
#37465=CARTESIAN_POINT('Ctrl Pts',(-32.7732690678164,-33.9763754204464,
46.0371553317249));
#37466=CARTESIAN_POINT('Ctrl Pts',(-30.7590389999979,-33.7216331346312,
46.1482851209446));
#37467=CARTESIAN_POINT('Ctrl Pts',(-29.8805229817197,-31.8912708743355,
46.2594149101644));
#37468=CARTESIAN_POINT('Ctrl Pts',(-30.9417293458004,-30.1604163307297,
46.3705446993841));
#37469=CARTESIAN_POINT('Ctrl Pts',(-32.9714535361373,-30.1131288117858,
46.4816744886039));
#37470=CARTESIAN_POINT('Ctrl Pts',(-34.1121139851762,-31.7926853420297,
46.5928042778235));
#37471=CARTESIAN_POINT('Ctrl Pts',(-33.3197906199043,-33.6619739990141,
46.7039340670433));
#37472=CARTESIAN_POINT('Ctrl Pts',(-31.3196091918293,-34.0102420754583,
46.815063856263));
#37473=CARTESIAN_POINT('Ctrl Pts',(-29.942114052861,-32.5187584046106,46.9261936454828));
#37474=CARTESIAN_POINT('Ctrl Pts',(-30.4479738158706,-30.5525126675639,
47.0373234347025));
#37475=CARTESIAN_POINT('Ctrl Pts',(-32.3742311115723,-29.9109916398163,
47.1484532239222));
#37476=CARTESIAN_POINT('Ctrl Pts',(-33.9579961523304,-31.1813084089564,
47.2595830131419));
#37477=CARTESIAN_POINT('Ctrl Pts',(-33.7498243480599,-33.2008828438791,
47.3707128023617));
#37478=CARTESIAN_POINT('Ctrl Pts',(-31.9402322764998,-34.1214223231157,
47.4818425915813));
#37479=CARTESIAN_POINT('Ctrl Pts',(-30.1853389773331,-33.100459098104,47.5929723808012));
#37480=CARTESIAN_POINT('Ctrl Pts',(-30.0912037669319,-31.0723676404894,
47.7041021700208));
#37481=CARTESIAN_POINT('Ctrl Pts',(-31.7439781690014,-29.8932352585449,
47.8152319592406));
#37482=CARTESIAN_POINT('Ctrl Pts',(-33.6310609743597,-30.6421911210678,
47.9263617484603));
#37483=CARTESIAN_POINT('Ctrl Pts',(-34.0254144641037,-32.6337989447653,
48.03749153768));
#37484=CARTESIAN_POINT('Ctrl Pts',(-32.5661306010053,-34.0453608474769,
48.1486213268997));
#37485=CARTESIAN_POINT('Ctrl Pts',(-30.5887301512975,-33.5850306835924,
48.2597511161195));
#37486=CARTESIAN_POINT('Ctrl Pts',(-29.9029085625381,-31.6740976270261,
48.3708809053392));
#37487=CARTESIAN_POINT('Ctrl Pts',(-31.1363223153341,-30.0614268879414,
48.4820106945589));
#37488=CARTESIAN_POINT('Ctrl Pts',(-33.160164518942,-30.2229172380628,48.5931404837787));
#37489=CARTESIAN_POINT('Ctrl Pts',(-34.1222367362744,-32.010774460249,48.7042702729984));
#37490=CARTESIAN_POINT('Ctrl Pts',(-33.1420609072676,-33.7887710132595,
48.8154000622181));
#37491=CARTESIAN_POINT('Ctrl Pts',(-31.1166833210643,-33.9297037333487,
48.9265298514378));
#37492=CARTESIAN_POINT('Ctrl Pts',(-29.8997075802525,-32.3045925234428,
49.0376596406576));
#37493=CARTESIAN_POINT('Ctrl Pts',(-30.6048966852708,-30.4007215392504,
49.1487894298773));
#37494=CARTESIAN_POINT('Ctrl Pts',(-32.5868692146638,-29.9604928588832,
49.259919219097));
#37495=CARTESIAN_POINT('Ctrl Pts',(-34.0317454031282,-31.3867989965323,
49.3710490083168));
#37496=CARTESIAN_POINT('Ctrl Pts',(-33.617190232011,-33.3743000426669,49.4821787975364));
#37497=CARTESIAN_POINT('Ctrl Pts',(-31.7226000982552,-34.1040565934162,
49.5933085867562));
#37498=CARTESIAN_POINT('Ctrl Pts',(-30.0818833462996,-32.9082033674146,
49.7044383759759));
#37499=CARTESIAN_POINT('Ctrl Pts',(-30.1966061547016,-30.8811722686105,
49.8155681651957));
#37500=CARTESIAN_POINT('Ctrl Pts',(-31.9617754533289,-29.8780801763926,
49.9266979544154));
#37501=CARTESIAN_POINT('Ctrl Pts',(-33.7619274425416,-30.8169460954779,
50.0378277436351));
#37502=CARTESIAN_POINT('Ctrl Pts',(-33.9495825436476,-32.8385301182965,
50.1489575328548));
#37503=CARTESIAN_POINT('Ctrl Pts',(-32.3530008431499,-34.0927004703305,
50.2600873220746));
#37504=CARTESIAN_POINT('Ctrl Pts',(-30.4333565991355,-33.4316540463099,
50.3712171112942));
#37505=CARTESIAN_POINT('Ctrl Pts',(-29.9474874060534,-31.4603733647475,
50.4823469005141));
#37506=CARTESIAN_POINT('Ctrl Pts',(-31.3400554803763,-29.9829531277623,
50.5934766897337));
#37507=CARTESIAN_POINT('Ctrl Pts',(-33.3365976222639,-30.351512314284,50.7046064789536));
#37508=CARTESIAN_POINT('Ctrl Pts',(-34.1099001150427,-32.2287495536736,
50.8157362681731));
#37509=CARTESIAN_POINT('Ctrl Pts',(-32.9522449034691,-33.8966376822164,
50.926866057393));
#37510=CARTESIAN_POINT('Ctrl Pts',(-30.9231054828656,-33.8287435721946,
51.0379958466126));
#37511=CARTESIAN_POINT('Ctrl Pts',(-29.8795282459899,-32.0872031767573,
51.1491256358324));
#37512=CARTESIAN_POINT('Ctrl Pts',(-30.776583762665,-30.2658553797126,51.2602554250521));
#37513=CARTESIAN_POINT('Ctrl Pts',(-32.7932965526705,-30.0315779329776,
51.3713852142718));
#37514=CARTESIAN_POINT('Ctrl Pts',(-34.0839929399853,-31.5987790156538,
51.4825150034916));
#37515=CARTESIAN_POINT('Ctrl Pts',(-33.4674415898341,-33.5331731915083,
51.5936447927112));
#37516=CARTESIAN_POINT('Ctrl Pts',(-31.5079036079414,-34.0644238903223,
51.7047745819311));
#37517=CARTESIAN_POINT('Ctrl Pts',(-29.9987269123803,-32.70633622997,51.8159043711507));
#37518=CARTESIAN_POINT('Ctrl Pts',(-30.3210936340406,-30.7018173167719,
51.9270341603705));
#37519=CARTESIAN_POINT('Ctrl Pts',(-32.1799772739779,-29.8853811073095,
52.0381639495902));
#37520=CARTESIAN_POINT('Ctrl Pts',(-33.8741476266704,-31.0042211956499,
52.1492937388099));
#37521=CARTESIAN_POINT('Ctrl Pts',(-33.8531184706876,-33.0343872087567,
52.2604235280296));
#37522=CARTESIAN_POINT('Ctrl Pts',(-32.1361352381636,-34.1178933414951,
52.3715533172494));
#37523=CARTESIAN_POINT('Ctrl Pts',(-30.2945628057577,-33.2631263059969,
52.4826831064691));
#37524=CARTESIAN_POINT('Ctrl Pts',(-30.0137874173263,-31.2523600696109,
52.5938128956888));
#37525=CARTESIAN_POINT('Ctrl Pts',(-31.5507733960611,-29.9258252031204,
52.7049426849085));
#37526=CARTESIAN_POINT('Ctrl Pts',(-33.4988844124893,-30.4975537783814,
52.8160724741283));
#37527=CARTESIAN_POINT('Ctrl Pts',(-34.0752371797756,-32.444302543842,52.927202263348));
#37528=CARTESIAN_POINT('Ctrl Pts',(-32.7523464566965,-33.9844349892809,
53.0383320525677));
#37529=CARTESIAN_POINT('Ctrl Pts',(-30.7409340892057,-33.708425046397,53.1494618417874));
#37530=CARTESIAN_POINT('Ctrl Pts',(-29.881770203702,-31.8689008564315,53.2605916310072));
#37531=CARTESIAN_POINT('Ctrl Pts',(-30.9612565106631,-30.1493218897363,
53.3717214202269));
#37532=CARTESIAN_POINT('Ctrl Pts',(-32.9912525050397,-30.1235333194147,
53.4828512094466));
#37533=CARTESIAN_POINT('Ctrl Pts',(-34.1143363305622,-31.8149284121924,
53.5939809986663));
#37534=CARTESIAN_POINT('Ctrl Pts',(-33.301865227782,-33.6759728407165,53.7051107878861));
#37535=CARTESIAN_POINT('Ctrl Pts',(-31.2990054068485,-34.0026421871099,
53.8162405771058));
#37536=CARTESIAN_POINT('Ctrl Pts',(-29.9355727613726,-32.4976003567713,
53.9273703663255));
#37537=CARTESIAN_POINT('Ctrl Pts',(-30.4657742788641,-30.5348890392292,
54.0385001555452));
#37538=CARTESIAN_POINT('Ctrl Pts',(-31.7487452602333,-30.1245170851199,
54.1125866816917));
#37539=CARTESIAN_POINT('Ctrl Pts',(-32.3352757582493,-30.2359961244728,
54.149629944765));
#37540=CARTESIAN_POINT('Ctrl Pts',(-33.4664903694653,-30.7527339134291,
40.850370055235));
#37541=CARTESIAN_POINT('Ctrl Pts',(-33.8812057842465,-31.24034130402,40.8874133183083));
#37542=CARTESIAN_POINT('Ctrl Pts',(-34.1785777870715,-32.6536087395612,
40.9614998444547));
#37543=CARTESIAN_POINT('Ctrl Pts',(-32.630173898414,-34.1878550261358,41.0726296336745));
#37544=CARTESIAN_POINT('Ctrl Pts',(-30.5048836538327,-33.7145955735989,
41.1837594228942));
#37545=CARTESIAN_POINT('Ctrl Pts',(-29.7480171888864,-31.6747036754478,
41.2948892121139));
#37546=CARTESIAN_POINT('Ctrl Pts',(-31.0520830545257,-29.9312398317713,
41.4060190013337));
#37547=CARTESIAN_POINT('Ctrl Pts',(-33.2237017016458,-30.0817287100789,
41.5171487905533));
#37548=CARTESIAN_POINT('Ctrl Pts',(-34.2753869150779,-31.9874724496487,
41.6282785797731));
#37549=CARTESIAN_POINT('Ctrl Pts',(-33.2446702314533,-33.9048460624559,
41.7394083689928));
#37550=CARTESIAN_POINT('Ctrl Pts',(-31.0748410447329,-34.0788419658076,
41.8505381582126));
#37551=CARTESIAN_POINT('Ctrl Pts',(-29.7517092232292,-32.3503463022476,
41.9616679474323));
#37552=CARTESIAN_POINT('Ctrl Pts',(-30.486187767832,-30.3011962564552,42.072797736652));
#37553=CARTESIAN_POINT('Ctrl Pts',(-32.6060913412801,-29.8067837068632,
42.1839275258717));
#37554=CARTESIAN_POINT('Ctrl Pts',(-34.1713064441483,-31.3195735023133,
42.2950573150915));
#37555=CARTESIAN_POINT('Ctrl Pts',(-33.7493655613665,-33.4550849885953,
42.4061871043112));
#37556=CARTESIAN_POINT('Ctrl Pts',(-31.7264242246551,-34.2589170893411,
42.5173168935309));
#37557=CARTESIAN_POINT('Ctrl Pts',(-29.9538565026843,-32.9954134658777,
42.6284466827507));
#37558=CARTESIAN_POINT('Ctrl Pts',(-30.0538971038138,-30.8209178801238,
42.7395764719703));
#37559=CARTESIAN_POINT('Ctrl Pts',(-31.9349899790798,-29.7255056422599,
42.8507062611902));
#37560=CARTESIAN_POINT('Ctrl Pts',(-33.8755793163684,-30.7116858846159,
42.9618360504098));
#37561=CARTESIAN_POINT('Ctrl Pts',(-34.0996588052083,-32.8769172797129,
43.0729658396296));
#37562=CARTESIAN_POINT('Ctrl Pts',(-32.4021533243219,-34.2396034671898,
43.1840956288493));
#37563=CARTESIAN_POINT('Ctrl Pts',(-30.3366014827183,-33.5526288606013,
43.295225418069));
#37564=CARTESIAN_POINT('Ctrl Pts',(-29.7933739250569,-31.44470515248,43.4063552072888));
#37565=CARTESIAN_POINT('Ctrl Pts',(-31.2696266214556,-29.8449812698521,
43.5174849965084));
#37566=CARTESIAN_POINT('Ctrl Pts',(-33.4143091132602,-30.2175071573529,
43.6286147857283));
#37567=CARTESIAN_POINT('Ctrl Pts',(-34.2646312421873,-32.2213511648709,
43.7397445749479));
#37568=CARTESIAN_POINT('Ctrl Pts',(-33.0423874171503,-34.0226169863703,
43.8508743641677));
#37569=CARTESIAN_POINT('Ctrl Pts',(-30.866161932167,-33.9728056765046,43.9620041533873));
#37570=CARTESIAN_POINT('Ctrl Pts',(-29.7276127508981,-32.117504005591,44.0731339426071));
#37571=CARTESIAN_POINT('Ctrl Pts',(-30.668727736996,-30.1546639430877,44.1842637318268));
#37572=CARTESIAN_POINT('Ctrl Pts',(-32.8282086611475,-29.8806554280094,
44.2953935210466));
#37573=CARTESIAN_POINT('Ctrl Pts',(-34.2297220001662,-31.5462480818947,
44.4065233102663));
#37574=CARTESIAN_POINT('Ctrl Pts',(-33.5906179449608,-33.6271095704889,
44.517653099486));
#37575=CARTESIAN_POINT('Ctrl Pts',(-31.4957975960606,-34.2188580254434,
44.6287828887057));
#37576=CARTESIAN_POINT('Ctrl Pts',(-29.8624178193984,-32.7799316780238,
44.7399126779255));
#37577=CARTESIAN_POINT('Ctrl Pts',(-30.1853300733093,-30.6272203168844,
44.8510424671452));
#37578=CARTESIAN_POINT('Ctrl Pts',(-32.1690085648516,-29.7308620345563,
44.9621722563649));
#37579=CARTESIAN_POINT('Ctrl Pts',(-33.9980122506633,-30.9111942104258,
45.0733020455847));
#37580=CARTESIAN_POINT('Ctrl Pts',(-33.9984567922086,-33.0879896373065,
45.1844318348043));
#37581=CARTESIAN_POINT('Ctrl Pts',(-32.169935349886,-34.2690687468806,45.2955616240241));
#37582=CARTESIAN_POINT('Ctrl Pts',(-30.1858909182199,-33.3735207463354,
45.4066914132438));
#37583=CARTESIAN_POINT('Ctrl Pts',(-29.8620994450051,-31.2209414539564,
45.5178212024635));
#37584=CARTESIAN_POINT('Ctrl Pts',(-31.4948913751556,-29.7813480943783,
45.6289509916833));
#37585=CARTESIAN_POINT('Ctrl Pts',(-33.5899532410887,-30.3722408985472,
45.740080780903));
#37586=CARTESIAN_POINT('Ctrl Pts',(-34.2299071431023,-32.4528411800533,
45.8512105701227));
#37587=CARTESIAN_POINT('Ctrl Pts',(-32.8290742100847,-34.1190061244327,
45.9623403593424));
#37588=CARTESIAN_POINT('Ctrl Pts',(-30.669481550933,-33.8458796433958,46.0734701485622));
#37589=CARTESIAN_POINT('Ctrl Pts',(-29.7275649474956,-31.8834241304543,
46.1845999377818));
#37590=CARTESIAN_POINT('Ctrl Pts',(-30.8653562605783,-30.0276575891083,
46.2957297270017));
#37591=CARTESIAN_POINT('Ctrl Pts',(-33.0415612192808,-29.9769574330476,
46.4068595162213));
#37592=CARTESIAN_POINT('Ctrl Pts',(-34.2645406453585,-31.7777238952787,
46.5179893054411));
#37593=CARTESIAN_POINT('Ctrl Pts',(-33.4150370307248,-33.7819150380667,
46.6291190946608));
#37594=CARTESIAN_POINT('Ctrl Pts',(-31.2705068710094,-34.15531686208,46.7402488838806));
#37595=CARTESIAN_POINT('Ctrl Pts',(-29.7936009119226,-32.5561960673557,
46.8513786731002));
#37596=CARTESIAN_POINT('Ctrl Pts',(-30.3359674708425,-30.4480506634827,
46.96250846232));
#37597=CARTESIAN_POINT('Ctrl Pts',(-32.401238554766,-29.7602324622005,47.0736382515397));
#37598=CARTESIAN_POINT('Ctrl Pts',(-34.0993004646186,-31.1222252222449,
47.1847680407595));
#37599=CARTESIAN_POINT('Ctrl Pts',(-33.8761053552179,-33.2875479398197,
47.2958978299791));
#37600=CARTESIAN_POINT('Ctrl Pts',(-31.935918970237,-34.2745207457474,47.4070276191989));
#37601=CARTESIAN_POINT('Ctrl Pts',(-30.0543788487655,-33.1798768313175,
47.5181574084186));
#37602=CARTESIAN_POINT('Ctrl Pts',(-29.9534501055209,-31.0054224360972,
47.6292871976384));
#37603=CARTESIAN_POINT('Ctrl Pts',(-31.7255016317942,-29.7411946416163,
47.740416986858));
#37604=CARTESIAN_POINT('Ctrl Pts',(-33.7487710878386,-30.5442010154039,
47.8515467760779));
#37605=CARTESIAN_POINT('Ctrl Pts',(-34.1715842089258,-32.6795388324115,
47.9626765652975));
#37606=CARTESIAN_POINT('Ctrl Pts',(-32.6069870118542,-34.1929700792877,
48.0738063545173));
#37607=CARTESIAN_POINT('Ctrl Pts',(-30.4868818840338,-33.6994188913702,
48.184936143737));
#37608=CARTESIAN_POINT('Ctrl Pts',(-29.7515660468629,-31.6505779635011,
48.2960659329567));
#37609=CARTESIAN_POINT('Ctrl Pts',(-31.0739925803522,-29.9215242941116,
48.4071957221765));
#37610=CARTESIAN_POINT('Ctrl Pts',(-33.2438910621709,-30.0946690506208,
48.5183255113961));
#37611=CARTESIAN_POINT('Ctrl Pts',(-34.2753939333276,-32.0115520295481,
48.6294553006159));
#37612=CARTESIAN_POINT('Ctrl Pts',(-33.2244809523226,-33.9178627163095,
48.7405850898355));
#37613=CARTESIAN_POINT('Ctrl Pts',(-31.0529362826949,-34.0689662434596,
48.8517148790554));
#37614=CARTESIAN_POINT('Ctrl Pts',(-29.7481340566664,-32.3265743016,48.962844668275));
#37615=CARTESIAN_POINT('Ctrl Pts',(-30.5042151215077,-30.285305100467,49.0739744574949));
#37616=CARTESIAN_POINT('Ctrl Pts',(-32.6292222860334,-29.8133060762947,
49.1851042467144));
#37617=CARTESIAN_POINT('Ctrl Pts',(-34.1783720380131,-31.3425456173894,
49.2962340359344));
#37618=CARTESIAN_POINT('Ctrl Pts',(-33.7338993242641,-33.4734802796533,
49.4073638251538));
#37619=CARTESIAN_POINT('Ctrl Pts',(-31.7025807523039,-34.2559017692069,
49.5184936143738));
#37620=CARTESIAN_POINT('Ctrl Pts',(-29.9434570504577,-32.9737464238182,
49.6296234035934));
#37621=CARTESIAN_POINT('Ctrl Pts',(-30.066459153753,-30.8004289111914,49.7407531928132));
#37622=CARTESIAN_POINT('Ctrl Pts',(-31.9590168711562,-29.7249458502354,
49.8518829820329));
#37623=CARTESIAN_POINT('Ctrl Pts',(-33.8890819036338,-30.7315676752091,
49.9630127712526));
#37624=CARTESIAN_POINT('Ctrl Pts',(-34.0902796641457,-32.8990450082557,
50.0741425604723));
#37625=CARTESIAN_POINT('Ctrl Pts',(-32.3784761441709,-34.2437260994837,
50.1852723496921));
#37626=CARTESIAN_POINT('Ctrl Pts',(-30.320295361453,-33.5349733966608,50.2964021389118));
#37627=CARTESIAN_POINT('Ctrl Pts',(-29.7993620482965,-31.4214296873067,
50.4075319281315));
#37628=CARTESIAN_POINT('Ctrl Pts',(-31.2924287236113,-29.837387253797,50.5186617173512));
#37629=CARTESIAN_POINT('Ctrl Pts',(-33.4330569577918,-30.2325445530509,
50.629791506571));
#37630=CARTESIAN_POINT('Ctrl Pts',(-34.2621670050455,-32.2452579101021,
50.7409212957906));
#37631=CARTESIAN_POINT('Ctrl Pts',(-33.0209663414834,-34.0335138875278,
50.8520510850105));
#37632=CARTESIAN_POINT('Ctrl Pts',(-30.8453883540707,-33.9607200076503,
50.9631808742301));
#37633=CARTESIAN_POINT('Ctrl Pts',(-29.7264984238575,-32.09349643985,51.0743106634499));
#37634=CARTESIAN_POINT('Ctrl Pts',(-30.6882924808598,-30.1407059443134,
51.1854404526696));
#37635=CARTESIAN_POINT('Ctrl Pts',(-32.8505470348444,-29.889521205163,51.2965702418894));
#37636=CARTESIAN_POINT('Ctrl Pts',(-34.234390165663,-31.5698237722019,51.407700031109));
#37637=CARTESIAN_POINT('Ctrl Pts',(-33.5733436491552,-33.6438189571738,
51.5188298203288));
#37638=CARTESIAN_POINT('Ctrl Pts',(-31.4723900844973,-34.2134088603623,
51.6299596095485));
#37639=CARTESIAN_POINT('Ctrl Pts',(-29.8542993980512,-32.757310975299,51.7410893987683));
#37640=CARTESIAN_POINT('Ctrl Pts',(-30.1999306229919,-30.6081303036183,
51.8522191879879));
#37641=CARTESIAN_POINT('Ctrl Pts',(-32.1929658413439,-29.7327736734147,
51.9633489772077));
#37642=CARTESIAN_POINT('Ctrl Pts',(-34.0094007737198,-30.9323580109484,
52.0744787664274));
#37643=CARTESIAN_POINT('Ctrl Pts',(-33.9868539894103,-33.1090366778066,
52.1856085556471));
#37644=CARTESIAN_POINT('Ctrl Pts',(-32.1459598214163,-34.2707370852193,
52.2967383448669));
#37645=CARTESIAN_POINT('Ctrl Pts',(-30.1714851226906,-33.3542833768571,
52.4078681340866));
#37646=CARTESIAN_POINT('Ctrl Pts',(-29.8704467867951,-31.1984045262985,
52.5189979233063));
#37647=CARTESIAN_POINT('Ctrl Pts',(-31.5183536917345,-29.7761365314191,
52.6301277125261));
#37648=CARTESIAN_POINT('Ctrl Pts',(-33.6070556317504,-30.389125511123,52.7412575017458));
#37649=CARTESIAN_POINT('Ctrl Pts',(-34.2250025213337,-32.4763668894899,
52.8523872909655));
#37650=CARTESIAN_POINT('Ctrl Pts',(-32.8066416597486,-34.1276473347736,
52.9635170801852));
#37651=CARTESIAN_POINT('Ctrl Pts',(-30.6500700482123,-33.8317183562382,
53.074646869405));
#37652=CARTESIAN_POINT('Ctrl Pts',(-29.7289021787684,-31.859439717143,53.1857766586246));
#37653=CARTESIAN_POINT('Ctrl Pts',(-30.8862926583441,-30.0157624865034,
53.2969064478444));
#37654=CARTESIAN_POINT('Ctrl Pts',(-33.062789036591,-29.9881128113017,53.4080362370641));
#37655=CARTESIAN_POINT('Ctrl Pts',(-34.2669233725645,-31.801572199307,53.5191660262839));
#37656=CARTESIAN_POINT('Ctrl Pts',(-33.3958180021451,-33.796924145646,53.6302958155035));
#37657=CARTESIAN_POINT('Ctrl Pts',(-31.2484161557996,-34.1471685063634,
53.7414256047234));
#37658=CARTESIAN_POINT('Ctrl Pts',(-29.7865875496927,-32.5335110893457,
53.852555393943));
#37659=CARTESIAN_POINT('Ctrl Pts',(-30.3550525544307,-30.4291551763249,
53.9636851831628));
#37660=CARTESIAN_POINT('Ctrl Pts',(-31.7306127536042,-29.9891675732325,
54.0377717093093));
#37661=CARTESIAN_POINT('Ctrl Pts',(-32.359471878548,-30.1086918117405,54.0748149723825));
#37662=CARTESIAN_POINT('Ctrl Pts',(-33.5652001142718,-30.6687801966679,
40.7755550828525));
#37663=CARTESIAN_POINT('Ctrl Pts',(-34.0078301022494,-31.1892085331669,
40.8125983459258));
#37664=CARTESIAN_POINT('Ctrl Pts',(-34.3252182709644,-32.6976032677414,
40.8866848720723));
#37665=CARTESIAN_POINT('Ctrl Pts',(-32.6725910229935,-34.3351199627491,
40.997814661292));
#37666=CARTESIAN_POINT('Ctrl Pts',(-30.4042470891071,-33.8300053267349,
41.1089444505117));
#37667=CARTESIAN_POINT('Ctrl Pts',(-29.596435798908,-31.652807918168,41.2200742397314));
#37668=CARTESIAN_POINT('Ctrl Pts',(-30.9882785852064,-29.7919911926234,
41.3312040289512));
#37669=CARTESIAN_POINT('Ctrl Pts',(-33.3060692951901,-29.9526095058617,
41.4423338181709));
#37670=CARTESIAN_POINT('Ctrl Pts',(-34.4285436397314,-31.9866292178594,
41.5534636073906));
#37671=CARTESIAN_POINT('Ctrl Pts',(-33.3284492207144,-34.0330616120671,
41.6645933966103));
#37672=CARTESIAN_POINT('Ctrl Pts',(-31.0125684200493,-34.218769212662,41.7757231858301));
#37673=CARTESIAN_POINT('Ctrl Pts',(-29.6003763447824,-32.3739281782754,
41.8868529750497));
#37674=CARTESIAN_POINT('Ctrl Pts',(-30.384292779475,-30.1868494543942,41.9979827642696));
#37675=CARTESIAN_POINT('Ctrl Pts',(-32.646887464373,-29.6591579023516,42.1091125534892));
#37676=CARTESIAN_POINT('Ctrl Pts',(-34.3174574925706,-31.2737738657493,
42.220242342709));
#37677=CARTESIAN_POINT('Ctrl Pts',(-33.8671156889712,-33.553027035053,42.3313721319286));
#37678=CARTESIAN_POINT('Ctrl Pts',(-31.7080097873483,-34.4109652269018,
42.4425019211485));
#37679=CARTESIAN_POINT('Ctrl Pts',(-29.8161301959435,-33.0624149349904,
42.5536317103682));
#37680=CARTESIAN_POINT('Ctrl Pts',(-29.9229045489022,-30.741553639088,42.6647614995879));
#37681=CARTESIAN_POINT('Ctrl Pts',(-31.9306141422462,-29.57240899581,42.7758912888076));
#37682=CARTESIAN_POINT('Ctrl Pts',(-34.0018249157517,-30.6249692172527,
42.8870210780274));
#37683=CARTESIAN_POINT('Ctrl Pts',(-34.2409872374696,-32.9359427480687,
42.9981508672471));
#37684=CARTESIAN_POINT('Ctrl Pts',(-32.4292223408278,-34.3903516011817,
43.1092806564668));
#37685=CARTESIAN_POINT('Ctrl Pts',(-30.2246378131498,-33.6571366035775,
43.2204104456865));
#37686=CARTESIAN_POINT('Ctrl Pts',(-29.6448455055895,-31.4073281510128,
43.3315402349062));
#37687=CARTESIAN_POINT('Ctrl Pts',(-31.2204650508714,-29.6999265505474,
43.442670024126));
#37688=CARTESIAN_POINT('Ctrl Pts',(-33.5095065278182,-30.0975272261643,
43.5537998133457));
#37689=CARTESIAN_POINT('Ctrl Pts',(-34.4170640004594,-32.2362503537452,
43.6649296025654));
#37690=CARTESIAN_POINT('Ctrl Pts',(-33.1125507118291,-34.1587597191989,
43.7760593917852));
#37691=CARTESIAN_POINT('Ctrl Pts',(-30.7898430768523,-34.1055956006222,
43.8871891810049));
#37692=CARTESIAN_POINT('Ctrl Pts',(-29.5746579343302,-32.1254132224854,
43.9983189702246));
#37693=CARTESIAN_POINT('Ctrl Pts',(-30.579119548572,-30.0304540232323,44.1094487594443));
#37694=CARTESIAN_POINT('Ctrl Pts',(-32.8839555431527,-29.7380019430538,
44.2205785486641));
#37695=CARTESIAN_POINT('Ctrl Pts',(-34.3798050107393,-31.5157059542584,
44.3317083378838));
#37696=CARTESIAN_POINT('Ctrl Pts',(-33.6976827404077,-33.7366306241687,
44.4428381271036));
#37697=CARTESIAN_POINT('Ctrl Pts',(-31.4618596366578,-34.3682097798181,
44.5539679163232));
#37698=CARTESIAN_POINT('Ctrl Pts',(-29.7185367575494,-32.832429027142,44.665097705543));
#37699=CARTESIAN_POINT('Ctrl Pts',(-30.0631842964932,-30.5348182561432,
44.7762274947627));
#37700=CARTESIAN_POINT('Ctrl Pts',(-32.1803845633948,-29.5781259278874,
44.8873572839824));
#37701=CARTESIAN_POINT('Ctrl Pts',(-34.1324988340666,-30.8379064862986,
44.9984870732022));
#37702=CARTESIAN_POINT('Ctrl Pts',(-34.1329732977875,-33.1612224260699,
45.1096168624218));
#37703=CARTESIAN_POINT('Ctrl Pts',(-32.1813737305056,-34.4218001944348,
45.2207466516416));
#37704=CARTESIAN_POINT('Ctrl Pts',(-30.0637828919811,-33.4659726881825,
45.3318764408613));
#37705=CARTESIAN_POINT('Ctrl Pts',(-29.7181969533154,-31.1685028755174,
45.4430062300811));
#37706=CARTESIAN_POINT('Ctrl Pts',(-31.4608924178518,-29.6320102139679,
45.5541360193008));
#37707=CARTESIAN_POINT('Ctrl Pts',(-33.6969732951919,-30.2626761248151,
45.6652658085205));
#37708=CARTESIAN_POINT('Ctrl Pts',(-34.3800026156816,-32.4833220057386,
45.7763955977402));
#37709=CARTESIAN_POINT('Ctrl Pts',(-32.8848793523529,-34.2616368284191,
45.88752538696));
#37710=CARTESIAN_POINT('Ctrl Pts',(-30.579924101868,-33.9701261521605,45.9986551761797));
#37711=CARTESIAN_POINT('Ctrl Pts',(-29.5746069132715,-31.8755773865731,
46.1097849653994));
#37712=CARTESIAN_POINT('Ctrl Pts',(-30.7889831753562,-29.8948988474869,
46.2209147546191));
#37713=CARTESIAN_POINT('Ctrl Pts',(-33.1116689024243,-29.8407860543094,
46.3320445438389));
#37714=CARTESIAN_POINT('Ctrl Pts',(-34.4169673055408,-31.7627624485277,
46.4431743330586));
#37715=CARTESIAN_POINT('Ctrl Pts',(-33.5102834415455,-33.9018560771194,
46.5543041222783));
#37716=CARTESIAN_POINT('Ctrl Pts',(-31.2214045501895,-34.3003916487017,
46.665433911498));
#37717=CARTESIAN_POINT('Ctrl Pts',(-29.6450877709841,-32.5936337301009,
46.7765637007178));
#37718=CARTESIAN_POINT('Ctrl Pts',(-30.2239611258143,-30.3435886594015,
46.8876934899375));
#37719=CARTESIAN_POINT('Ctrl Pts',(-32.4282459979597,-29.6094732845848,
46.9988232791572));
#37720=CARTESIAN_POINT('Ctrl Pts',(-34.2406047769068,-31.0631420355334,
47.109953068377));
#37721=CARTESIAN_POINT('Ctrl Pts',(-34.0023863623759,-33.3742130357603,
47.2210828575967));
#37722=CARTESIAN_POINT('Ctrl Pts',(-31.9316056639743,-34.4276191683791,
47.3322126468164));
#37723=CARTESIAN_POINT('Ctrl Pts',(-29.9234187201979,-33.2592945645311,
47.4433424360361));
#37724=CARTESIAN_POINT('Ctrl Pts',(-29.8156964441101,-30.938477231705,47.5544722252559));
#37725=CARTESIAN_POINT('Ctrl Pts',(-31.707025094587,-29.5891540246876,47.6656020144756));
#37726=CARTESIAN_POINT('Ctrl Pts',(-33.8664812013175,-30.44621090974,47.7767318036953));
#37727=CARTESIAN_POINT('Ctrl Pts',(-34.3177539537478,-32.7252787200575,
47.887861592915));
#37728=CARTESIAN_POINT('Ctrl Pts',(-32.6478434227033,-34.3405793110984,
47.9989913821348));
#37729=CARTESIAN_POINT('Ctrl Pts',(-30.38503361677,-33.8138070991479,48.1101211713545));
#37730=CARTESIAN_POINT('Ctrl Pts',(-29.6002235311877,-31.627058299976,48.2212509605742));
#37731=CARTESIAN_POINT('Ctrl Pts',(-31.0116628453703,-29.7816217002818,
48.3323807497939));
#37732=CARTESIAN_POINT('Ctrl Pts',(-33.3276176053999,-29.9664208631788,
48.4435105390137));
#37733=CARTESIAN_POINT('Ctrl Pts',(-34.4285511303809,-32.0123295988471,
48.5546403282334));
#37734=CARTESIAN_POINT('Ctrl Pts',(-33.3069009973776,-34.0469544193595,
48.6657701174531));
#37735=CARTESIAN_POINT('Ctrl Pts',(-30.9891892443255,-34.2082287535704,
48.7768999066729));
#37736=CARTESIAN_POINT('Ctrl Pts',(-29.5965605330805,-32.3485560797573,
48.8880296958926));
#37737=CARTESIAN_POINT('Ctrl Pts',(-30.4035335577445,-30.1698886616836,
48.9991594851123));
#37738=CARTESIAN_POINT('Ctrl Pts',(-32.6715753574031,-29.6661192937061,
49.110289274332));
#37739=CARTESIAN_POINT('Ctrl Pts',(-34.3249986728979,-31.2982922382464,
49.2214190635518));
#37740=CARTESIAN_POINT('Ctrl Pts',(-33.8506084165172,-33.5726605166398,
49.3325488527714));
#37741=CARTESIAN_POINT('Ctrl Pts',(-31.6825614063526,-34.4077469449976,
49.4436786419912));
#37742=CARTESIAN_POINT('Ctrl Pts',(-29.8050307546158,-33.0392894802219,
49.5548084312109));
#37743=CARTESIAN_POINT('Ctrl Pts',(-29.9363121528045,-30.7196855537722,
49.6659382204306));
#37744=CARTESIAN_POINT('Ctrl Pts',(-31.9562582889836,-29.5718115240782,
49.7770680096504));
#37745=CARTESIAN_POINT('Ctrl Pts',(-34.0162363647259,-30.6461892549403,
49.8881977988701));
#37746=CARTESIAN_POINT('Ctrl Pts',(-34.2309767846438,-32.9595598982149,
49.9993275880899));
#37747=CARTESIAN_POINT('Ctrl Pts',(-32.4039514451918,-34.3947517286369,
50.1104573773095));
#37748=CARTESIAN_POINT('Ctrl Pts',(-30.2072341237705,-33.6382927470118,
50.2215871665293));
#37749=CARTESIAN_POINT('Ctrl Pts',(-29.6512366905396,-31.3824860098658,
50.332716955749));
#37750=CARTESIAN_POINT('Ctrl Pts',(-31.2448019668464,-29.6918213798318,
50.4438467449688));
#37751=CARTESIAN_POINT('Ctrl Pts',(-33.5295162933197,-30.1135767918179,
50.5549765341885));
#37752=CARTESIAN_POINT('Ctrl Pts',(-34.4144338950484,-32.2617662665304,
50.6661063234082));
#37753=CARTESIAN_POINT('Ctrl Pts',(-33.0896877794978,-34.1703900928393,
50.7772361126279));
#37754=CARTESIAN_POINT('Ctrl Pts',(-30.7676712252758,-34.0926964431059,
50.8883659018477));
#37755=CARTESIAN_POINT('Ctrl Pts',(-29.5734686017252,-32.0997897029427,
50.9994956910673));
#37756=CARTESIAN_POINT('Ctrl Pts',(-30.6000011990546,-30.0155565089142,
51.1106254802872));
#37757=CARTESIAN_POINT('Ctrl Pts',(-32.9077975170184,-29.7474644773485,
51.2217552695068));
#37758=CARTESIAN_POINT('Ctrl Pts',(-34.3847873913407,-31.54086852875,51.3328850587266));
#37759=CARTESIAN_POINT('Ctrl Pts',(-33.6792457084763,-33.7544647228394,
51.4440148479463));
#37760=CARTESIAN_POINT('Ctrl Pts',(-31.4368765610531,-34.3623938304022,
51.5551446371661));
#37761=CARTESIAN_POINT('Ctrl Pts',(-29.7098718837221,-32.808285720628,51.6662744263857));
#37762=CARTESIAN_POINT('Ctrl Pts',(-30.0787676119431,-30.5144432904648,
51.7774042156055));
#37763=CARTESIAN_POINT('Ctrl Pts',(-32.2059544087099,-29.5801662395198,
51.8885340048252));
#37764=CARTESIAN_POINT('Ctrl Pts',(-34.1446539207691,-30.8604948262468,
51.9996637940449));
#37765=CARTESIAN_POINT('Ctrl Pts',(-34.1205895081331,-33.1836861468564,
52.1107935832646));
#37766=CARTESIAN_POINT('Ctrl Pts',(-32.1557844046688,-34.4235808289435,
52.2219233724844));
#37767=CARTESIAN_POINT('Ctrl Pts',(-30.0484074396236,-33.4454404477173,
52.333053161704));
#37768=CARTESIAN_POINT('Ctrl Pts',(-29.7271061562637,-31.1444489829859,
52.4441829509239));
#37769=CARTESIAN_POINT('Ctrl Pts',(-31.4859339874079,-29.6264478597178,
52.5553127401435));
#37770=CARTESIAN_POINT('Ctrl Pts',(-33.7152268510116,-30.2806972438647,
52.6664425293633));
#37771=CARTESIAN_POINT('Ctrl Pts',(-34.3747678628917,-32.5084312351377,
52.777572318583));
#37772=CARTESIAN_POINT('Ctrl Pts',(-32.8609368628007,-34.2708596802663,
52.8887021078028));
#37773=CARTESIAN_POINT('Ctrl Pts',(-30.5592060072189,-33.9550116660794,
52.9998318970225));
#37774=CARTESIAN_POINT('Ctrl Pts',(-29.5760341538348,-31.8499785778545,
53.1109616862422));
#37775=CARTESIAN_POINT('Ctrl Pts',(-30.811328806025,-29.8822030832705,53.2220914754619));
#37776=CARTESIAN_POINT('Ctrl Pts',(-33.1343255681424,-29.8526923031888,
53.3332212646816));
#37777=CARTESIAN_POINT('Ctrl Pts',(-34.4195104145668,-31.7882159864216,
53.4443510539014));
#37778=CARTESIAN_POINT('Ctrl Pts',(-33.4897707765082,-33.9178754505755,
53.555480843121));
#37779=CARTESIAN_POINT('Ctrl Pts',(-31.1978269047507,-34.2916948256168,
53.6666106323409));
#37780=CARTESIAN_POINT('Ctrl Pts',(-29.6376023380129,-32.5694218219201,
53.7777404215605));
#37781=CARTESIAN_POINT('Ctrl Pts',(-30.2443308299973,-30.3234213134206,
53.8888702107803));
#37782=CARTESIAN_POINT('Ctrl Pts',(-31.7124802469751,-29.853818061345,53.9629567369268));
#37783=CARTESIAN_POINT('Ctrl Pts',(-32.3836679988468,-29.9813874990081,
54.));
#37784=CARTESIAN_POINT('Ctrl Pts',(-33.2690708798524,-30.9206413469515,
41.));
#37785=CARTESIAN_POINT('Ctrl Pts',(-33.3144021339049,-30.9629305958324,
41.));
#37786=CARTESIAN_POINT('Ctrl Pts',(-33.3570035121663,-31.0077888080552,
41.));
#37787=CARTESIAN_POINT('Ctrl Pts',(-33.3968764064509,-31.0548709990206,
41.));
#37788=CARTESIAN_POINT('Ctrl Pts',(-33.4393774015784,-31.1050564697451,
41.));
#37789=CARTESIAN_POINT('Ctrl Pts',(-33.4787791039696,-31.1577689887107,
41.));
#37790=CARTESIAN_POINT('Ctrl Pts',(-33.5150543778823,-31.2126454611912,
41.));
#37791=CARTESIAN_POINT('Ctrl Pts',(-33.5467952425558,-31.2606623746115,
41.));
#37792=CARTESIAN_POINT('Ctrl Pts',(-33.5761421922477,-31.3103372901136,
41.));
#37793=CARTESIAN_POINT('Ctrl Pts',(-33.6030541620467,-31.3614545089767,
41.));
#37794=CARTESIAN_POINT('Ctrl Pts',(-33.6165537378605,-31.3870959160009,
41.));
#37795=CARTESIAN_POINT('Ctrl Pts',(-33.6294402577063,-31.4131005944397,
41.));
#37796=CARTESIAN_POINT('Ctrl Pts',(-33.6417061981854,-31.4394431592821,
41.));
#37797=CARTESIAN_POINT('Ctrl Pts',(-33.6473173626409,-31.4514938017715,
41.));
#37798=CARTESIAN_POINT('Ctrl Pts',(-33.6527992406224,-31.4636168448061,
41.));
#37799=CARTESIAN_POINT('Ctrl Pts',(-33.6581425910225,-31.4757898827236,
41.));
#37800=CARTESIAN_POINT('Ctrl Pts',(-33.6850641954014,-31.5371217599846,
41.));
#37801=CARTESIAN_POINT('Ctrl Pts',(-33.7085245215074,-31.5998290858622,
41.));
#37802=CARTESIAN_POINT('Ctrl Pts',(-33.7284999672539,-31.6635541553473,
41.));
#37803=CARTESIAN_POINT('Ctrl Pts',(-33.7488294277261,-31.7284085920203,
41.));
#37804=CARTESIAN_POINT('Ctrl Pts',(-33.7655499493255,-31.7943180072714,
41.));
#37805=CARTESIAN_POINT('Ctrl Pts',(-33.778597337887,-31.8609418493504,41.));
#37806=CARTESIAN_POINT('Ctrl Pts',(-33.7895089410008,-31.9166597364401,
41.));
#37807=CARTESIAN_POINT('Ctrl Pts',(-33.79785097422,-31.9728782395951,41.));
#37808=CARTESIAN_POINT('Ctrl Pts',(-33.8035610724783,-32.0294104457794,
41.));
#37809=CARTESIAN_POINT('Ctrl Pts',(-33.8061908595079,-32.0554463659775,
41.));
#37810=CARTESIAN_POINT('Ctrl Pts',(-33.8082620610742,-32.0815489376605,
41.));
#37811=CARTESIAN_POINT('Ctrl Pts',(-33.8097667846064,-32.1077003030272,
41.));
#37812=CARTESIAN_POINT('Ctrl Pts',(-33.810424820059,-32.1191366401208,41.));
#37813=CARTESIAN_POINT('Ctrl Pts',(-33.8109744041467,-32.1305821183287,
41.));
#37814=CARTESIAN_POINT('Ctrl Pts',(-33.8114145404549,-32.1420210826457,
41.));
#37815=CARTESIAN_POINT('Ctrl Pts',(-33.8141127124152,-32.2121454786513,
41.));
#37816=CARTESIAN_POINT('Ctrl Pts',(-33.8127099139614,-32.2821564492406,
41.));
#37817=CARTESIAN_POINT('Ctrl Pts',(-33.8071514190027,-32.3516932928698,
41.));
#37818=CARTESIAN_POINT('Ctrl Pts',(-33.8021840417643,-32.4138352461935,
41.));
#37819=CARTESIAN_POINT('Ctrl Pts',(-33.7938974934504,-32.4755995156626,
41.));
#37820=CARTESIAN_POINT('Ctrl Pts',(-33.7822196326176,-32.5367407937649,
41.));
#37821=CARTESIAN_POINT('Ctrl Pts',(-33.7694915938875,-32.6033804435122,
41.));
#37822=CARTESIAN_POINT('Ctrl Pts',(-33.7527359516846,-32.6692808462158,
41.));
#37823=CARTESIAN_POINT('Ctrl Pts',(-33.7321979940556,-32.7342283571542,
41.));
#37824=CARTESIAN_POINT('Ctrl Pts',(-33.724265767216,-32.759312564588,41.));
#37825=CARTESIAN_POINT('Ctrl Pts',(-33.7157687851902,-32.7842545839253,
41.));
#37826=CARTESIAN_POINT('Ctrl Pts',(-33.7067191665299,-32.8090417859885,
41.));
#37827=CARTESIAN_POINT('Ctrl Pts',(-33.70275069803,-32.8199115512552,41.));
#37828=CARTESIAN_POINT('Ctrl Pts',(-33.6986760523364,-32.8307509911782,
41.));
#37829=CARTESIAN_POINT('Ctrl Pts',(-33.6945013450319,-32.8415464817173,
41.));
#37830=CARTESIAN_POINT('Ctrl Pts',(-33.6692787045914,-32.9067704019559,
41.));
#37831=CARTESIAN_POINT('Ctrl Pts',(-33.6403651464208,-32.9705093076493,
41.));
#37832=CARTESIAN_POINT('Ctrl Pts',(-33.6080733761304,-33.032544316927,41.));
#37833=CARTESIAN_POINT('Ctrl Pts',(-33.5750332258155,-33.0960170226008,
41.));
#37834=CARTESIAN_POINT('Ctrl Pts',(-33.5384561627934,-33.1577067585806,
41.));
#37835=CARTESIAN_POINT('Ctrl Pts',(-33.498621001724,-33.217375363133,41.));
#37836=CARTESIAN_POINT('Ctrl Pts',(-33.4681150091642,-33.2630699193408,
41.));
#37837=CARTESIAN_POINT('Ctrl Pts',(-33.4356970622739,-33.3075791992015,
41.));
#37838=CARTESIAN_POINT('Ctrl Pts',(-33.4014728035091,-33.3507901304747,
41.));
#37839=CARTESIAN_POINT('Ctrl Pts',(-33.3801641715878,-33.3776940244585,
41.));
#37840=CARTESIAN_POINT('Ctrl Pts',(-33.3581549933686,-33.4040944868308,
41.));
#37841=CARTESIAN_POINT('Ctrl Pts',(-33.3354678533328,-33.429962533573,41.));
#37842=CARTESIAN_POINT('Ctrl Pts',(-33.3228125188513,-33.444392240596,41.));
#37843=CARTESIAN_POINT('Ctrl Pts',(-33.3099417870806,-33.4586607850949,
41.));
#37844=CARTESIAN_POINT('Ctrl Pts',(-33.296883176771,-33.4727378235807,41.));
#37845=CARTESIAN_POINT('Ctrl Pts',(-33.2460103594919,-33.5275781618508,
41.));
#37846=CARTESIAN_POINT('Ctrl Pts',(-33.1922409760063,-33.5795735763044,
41.));
#37847=CARTESIAN_POINT('Ctrl Pts',(-33.1358600432967,-33.6284600523803,
41.));
#37848=CARTESIAN_POINT('Ctrl Pts',(-33.0937060761678,-33.665010687613,41.));
#37849=CARTESIAN_POINT('Ctrl Pts',(-33.0500910944577,-33.6998232253623,
41.));
#37850=CARTESIAN_POINT('Ctrl Pts',(-33.0051178395859,-33.7327775840894,
41.));
#37851=CARTESIAN_POINT('Ctrl Pts',(-32.9910336310623,-33.7430978524666,
41.));
#37852=CARTESIAN_POINT('Ctrl Pts',(-32.9768161177428,-33.753235803731,41.));
#37853=CARTESIAN_POINT('Ctrl Pts',(-32.9624682127011,-33.7631875218369,
41.));
#37854=CARTESIAN_POINT('Ctrl Pts',(-32.9486861828198,-33.772746748491,41.));
#37855=CARTESIAN_POINT('Ctrl Pts',(-32.9347908997058,-33.7821291855208,
41.));
#37856=CARTESIAN_POINT('Ctrl Pts',(-32.9207902802946,-33.7913286466319,
41.));
#37857=CARTESIAN_POINT('Ctrl Pts',(-32.8578346063116,-33.8326952646019,
41.));
#37858=CARTESIAN_POINT('Ctrl Pts',(-32.7927216231867,-33.8703859566203,
41.));
#37859=CARTESIAN_POINT('Ctrl Pts',(-32.7257126837587,-33.904121456021,41.));
#37860=CARTESIAN_POINT('Ctrl Pts',(-32.6745222121957,-33.9298931834572,
41.));
#37861=CARTESIAN_POINT('Ctrl Pts',(-32.6222242930451,-33.9533562649217,
41.));
#37862=CARTESIAN_POINT('Ctrl Pts',(-32.5689216133098,-33.9743709796003,
41.));
#37863=CARTESIAN_POINT('Ctrl Pts',(-32.5564364973219,-33.9792932677764,
41.));
#37864=CARTESIAN_POINT('Ctrl Pts',(-32.5438962117701,-33.9840811613941,
41.));
#37865=CARTESIAN_POINT('Ctrl Pts',(-32.5313027126548,-33.9887352548077,
41.));
#37866=CARTESIAN_POINT('Ctrl Pts',(-30.3326929969897,-32.0013037885424,
42.1285196366098));
#37867=CARTESIAN_POINT('Ctrl Pts',(-30.3319567887293,-32.0869536137603,
42.1227790551389));
#37868=CARTESIAN_POINT('Ctrl Pts',(-30.3379868491816,-32.1724994374198,
42.1170384736681));
#37869=CARTESIAN_POINT('Ctrl Pts',(-30.3511439931895,-32.2569345889072,
42.1112978921972));
#37870=CARTESIAN_POINT('Ctrl Pts',(-30.4360454181153,-32.8017841908275,
42.074254629124));
#37871=CARTESIAN_POINT('Ctrl Pts',(-30.8177158561077,-33.3003858314631,
42.0372113660508));
#37872=CARTESIAN_POINT('Ctrl Pts',(-31.3215054015757,-33.5245912336367,
42.0001681029776));
#37873=CARTESIAN_POINT('Ctrl Pts',(-31.8252949470438,-33.7487966358103,
41.9631248399043));
#37874=CARTESIAN_POINT('Ctrl Pts',(-32.4512035999874,-33.6986057995218,
41.9260815768311));
#37875=CARTESIAN_POINT('Ctrl Pts',(-32.9128181285992,-33.3969677063766,
41.8890383137578));
#37876=CARTESIAN_POINT('Ctrl Pts',(-33.374432657211,-33.0953296132314,41.8519950506846));
#37877=CARTESIAN_POINT('Ctrl Pts',(-33.6717530614909,-32.5422442632293,
41.8149517876114));
#37878=CARTESIAN_POINT('Ctrl Pts',(-33.6687287717619,-31.9908362891094,
41.7779085245381));
#37879=CARTESIAN_POINT('Ctrl Pts',(-33.665704482033,-31.4394283149894,41.7408652614649));
#37880=CARTESIAN_POINT('Ctrl Pts',(-33.3623354982951,-30.8896977167514,
41.7038219983916));
#37881=CARTESIAN_POINT('Ctrl Pts',(-32.897438586194,-30.5931274162247,41.6667787353184));
#37882=CARTESIAN_POINT('Ctrl Pts',(-32.4325416740929,-30.296557115698,41.6297354722451));
#37883=CARTESIAN_POINT('Ctrl Pts',(-31.8061168336285,-30.2531471128826,
41.5926922091719));
#37884=CARTESIAN_POINT('Ctrl Pts',(-31.3048190760095,-30.482901791465,41.5556489460986));
#37885=CARTESIAN_POINT('Ctrl Pts',(-30.8035213183905,-30.7126564700473,
41.5186056830254));
#37886=CARTESIAN_POINT('Ctrl Pts',(-30.4273506436169,-31.2155758300274,
41.4815624199522));
#37887=CARTESIAN_POINT('Ctrl Pts',(-30.3484281086368,-31.7612489895707,
41.4445191568789));
#37888=CARTESIAN_POINT('Ctrl Pts',(-30.3370655144398,-31.8398103621579,
41.4391859834559));
#37889=CARTESIAN_POINT('Ctrl Pts',(-30.3318642164196,-31.9192579264029,
41.4338528100328));
#37890=CARTESIAN_POINT('Ctrl Pts',(-30.3325261502749,-31.9987897978733,
41.4285196366098));
#37891=CARTESIAN_POINT('Ctrl Pts',(-31.4698297828114,-33.9851743256717,
41.));
#37892=CARTESIAN_POINT('Ctrl Pts',(-30.8097602092473,-33.8088929660699,
41.0370432630732));
#37893=CARTESIAN_POINT('Ctrl Pts',(-29.6907568933951,-32.7487864588875,
41.1111297892197));
#37894=CARTESIAN_POINT('Ctrl Pts',(-30.1186157833437,-30.4619638323954,
41.2222595784395));
#37895=CARTESIAN_POINT('Ctrl Pts',(-32.2715961806528,-29.5872035622868,
41.3333893676592));
#37896=CARTESIAN_POINT('Ctrl Pts',(-34.1743722595742,-30.9184415569553,
41.444519156879));
#37897=CARTESIAN_POINT('Ctrl Pts',(-34.0880140492357,-33.2405968969734,
41.5556489460986));
#37898=CARTESIAN_POINT('Ctrl Pts',(-32.090310165188,-34.4268231234318,41.6667787353184));
#37899=CARTESIAN_POINT('Ctrl Pts',(-30.0101664395875,-33.3923240254871,
41.7779085245381));
#37900=CARTESIAN_POINT('Ctrl Pts',(-29.7509902158367,-31.0834452339837,
41.8890383137579));
#37901=CARTESIAN_POINT('Ctrl Pts',(-31.5501371962138,-29.6134580581644,
42.0001681029775));
#37902=CARTESIAN_POINT('Ctrl Pts',(-33.7609665425501,-30.3275725104634,
42.1112978921973));
#37903=CARTESIAN_POINT('Ctrl Pts',(-34.3601921411462,-32.5722924840244,
42.2224276814169));
#37904=CARTESIAN_POINT('Ctrl Pts',(-32.7993885499411,-34.2932474809962,
42.3335574706367));
#37905=CARTESIAN_POINT('Ctrl Pts',(-30.5069967308568,-33.9154518496341,
42.4446872598564));
#37906=CARTESIAN_POINT('Ctrl Pts',(-29.580983542908,-31.7846531357871,42.5558170490762));
#37907=CARTESIAN_POINT('Ctrl Pts',(-30.8688288772728,-29.8509387094972,
42.6669468382958));
#37908=CARTESIAN_POINT('Ctrl Pts',(-33.1919093046072,-29.8840212783247,
42.7780766275157));
#37909=CARTESIAN_POINT('Ctrl Pts',(-34.4241674901357,-31.8536249255854,
42.8892064167353));
#37910=CARTESIAN_POINT('Ctrl Pts',(-33.4378537625072,-33.9571893024616,
43.0003362059551));
#37911=CARTESIAN_POINT('Ctrl Pts',(-31.1356319224862,-34.2695553308866,
43.1114659951748));
#37912=CARTESIAN_POINT('Ctrl Pts',(-29.6244703439387,-32.5048488942348,
43.2225957843946));
#37913=CARTESIAN_POINT('Ctrl Pts',(-30.2873677599144,-30.2781102439097,
43.3337255736142));
#37914=CARTESIAN_POINT('Ctrl Pts',(-32.5176476217965,-29.6272264154066,
43.444855362834));
#37915=CARTESIAN_POINT('Ctrl Pts',(-34.2741819976516,-31.1478792448328,
43.5559851520537));
#37916=CARTESIAN_POINT('Ctrl Pts',(-33.9494096698203,-33.4483837460143,
43.6671149412734));
#37917=CARTESIAN_POINT('Ctrl Pts',(-31.8405587536029,-34.4233431511784,
43.7782447304932));
#37918=CARTESIAN_POINT('Ctrl Pts',(-29.877626736532,-33.1804851838061,43.8893745197129));
#37919=CARTESIAN_POINT('Ctrl Pts',(-29.8570677142538,-30.8572599783665,
44.0005043089327));
#37920=CARTESIAN_POINT('Ctrl Pts',(-31.7976970806331,-29.5798580480631,
44.1116340981523));
#37921=CARTESIAN_POINT('Ctrl Pts',(-33.923471884996,-30.5173437869082,44.2227638873721));
#37922=CARTESIAN_POINT('Ctrl Pts',(-34.2889060793629,-32.8117404131962,
44.3338936765918));
#37923=CARTESIAN_POINT('Ctrl Pts',(-32.5595582520656,-34.3632410163062,
44.4450234658115));
#37924=CARTESIAN_POINT('Ctrl Pts',(-30.3181087806264,-33.7519290695639,
44.5561532550312));
#37925=CARTESIAN_POINT('Ctrl Pts',(-29.6159079138112,-31.5372706372416,
44.667283044251));
#37926=CARTESIAN_POINT('Ctrl Pts',(-31.0956022698719,-29.7460970996221,
44.7784128334707));
#37927=CARTESIAN_POINT('Ctrl Pts',(-33.4029916207618,-30.0176710538707,
44.8895426226904));
#37928=CARTESIAN_POINT('Ctrl Pts',(-34.4263782551407,-32.1034509621539,
45.0006724119102));
#37929=CARTESIAN_POINT('Ctrl Pts',(-33.2291698233915,-34.0945536717531,
45.1118022011298));
#37930=CARTESIAN_POINT('Ctrl Pts',(-30.907038499066,-34.1687435754524,45.2229319903497));
#37931=CARTESIAN_POINT('Ctrl Pts',(-29.5851736877214,-32.2581228779425,
45.3340617795693));
#37932=CARTESIAN_POINT('Ctrl Pts',(-30.4733317296733,-30.1112709217656,
45.4451915687891));
#37933=CARTESIAN_POINT('Ctrl Pts',(-32.7586800166002,-29.6929633355749,
45.5563213580088));
#37934=CARTESIAN_POINT('Ctrl Pts',(-34.3496925798768,-31.3860306858952,
45.6674511472285));
#37935=CARTESIAN_POINT('Ctrl Pts',(-33.7902919754051,-33.6409960942643,
45.7785809364483));
#37936=CARTESIAN_POINT('Ctrl Pts',(-31.5924355699507,-34.3941396730243,
45.889710725668));
#37937=CARTESIAN_POINT('Ctrl Pts',(-29.7675777110252,-32.9561925863961,
46.0008405148877));
#37938=CARTESIAN_POINT('Ctrl Pts',(-29.9858085213579,-30.643148414175,46.1119703041075));
#37939=CARTESIAN_POINT('Ctrl Pts',(-32.0474055299468,-29.5718800988582,
46.2231000933271));
#37940=CARTESIAN_POINT('Ctrl Pts',(-34.06561751162,-30.7228007852025,46.3342298825469));
#37941=CARTESIAN_POINT('Ctrl Pts',(-34.1933987473477,-33.0426003422808,
46.4453596717667));
#37942=CARTESIAN_POINT('Ctrl Pts',(-32.3138052359217,-34.4082233726336,
46.5564894609863));
#37943=CARTESIAN_POINT('Ctrl Pts',(-30.1470205756562,-33.5698664884471,
46.6676192502061));
#37944=CARTESIAN_POINT('Ctrl Pts',(-29.6760625898251,-31.294784818527,46.7787490394258));
#37945=CARTESIAN_POINT('Ctrl Pts',(-31.3319469197342,-29.6651084349508,
46.8898788286455));
#37946=CARTESIAN_POINT('Ctrl Pts',(-33.5992261839687,-30.172299490863,47.0010086178653));
#37947=CARTESIAN_POINT('Ctrl Pts',(-34.4029109875207,-32.3521822321507,
47.1121384070849));
#37948=CARTESIAN_POINT('Ctrl Pts',(-33.0074777137784,-34.2097516138314,
47.2232681963047));
#37949=CARTESIAN_POINT('Ctrl Pts',(-30.6900117620269,-34.0449802822919,
47.3343979855244));
#37950=CARTESIAN_POINT('Ctrl Pts',(-29.5714328394375,-32.0086651732867,
47.4455277747442));
#37951=CARTESIAN_POINT('Ctrl Pts',(-30.6754522454808,-29.9644197916593,
47.5566575639639));
#37952=CARTESIAN_POINT('Ctrl Pts',(-32.9916833923377,-29.7831153417573,
47.6677873531836));
#37953=CARTESIAN_POINT('Ctrl Pts',(-34.4003366528858,-31.6306796899659,
47.7789171424033));
#37954=CARTESIAN_POINT('Ctrl Pts',(-33.6122278392798,-33.8162419808058,
47.890046931623));
#37955=CARTESIAN_POINT('Ctrl Pts',(-31.3486255910479,-34.3395993071363,
48.0011767208428));
#37956=CARTESIAN_POINT('Ctrl Pts',(-29.6811541380276,-32.7217807194736,
48.1123065100625));
#37957=CARTESIAN_POINT('Ctrl Pts',(-30.1358652710482,-30.4433962447347,
48.2234362992822));
#37958=CARTESIAN_POINT('Ctrl Pts',(-32.2966122923061,-29.5895986461497,
48.334566088502));
#37959=CARTESIAN_POINT('Ctrl Pts',(-34.1859029602719,-30.9417742268944,
48.4456958777216));
#37960=CARTESIAN_POINT('Ctrl Pts',(-34.0746789441273,-33.2624265592047,
48.5568256669415));
#37961=CARTESIAN_POINT('Ctrl Pts',(-32.0647312572736,-34.4277197949768,
48.6679554561611));
#37962=CARTESIAN_POINT('Ctrl Pts',(-29.9955422257445,-33.3711902019111,
48.7790852453809));
#37963=CARTESIAN_POINT('Ctrl Pts',(-29.7608112117745,-31.0597622059948,
48.8902150346006));
#37964=CARTESIAN_POINT('Ctrl Pts',(-31.5753614937973,-29.6088296426979,
49.0013448238204));
#37965=CARTESIAN_POINT('Ctrl Pts',(-33.7785363316839,-30.346270259241,49.11247461304));
#37966=CARTESIAN_POINT('Ctrl Pts',(-34.3540140062368,-32.5971864005746,
49.2236044022598));
#37967=CARTESIAN_POINT('Ctrl Pts',(-32.7751235905007,-34.3015640243191,
49.3347341914795));
#37968=CARTESIAN_POINT('Ctrl Pts',(-30.4868484706035,-33.8995752124292,
49.4458639806993));
#37969=CARTESIAN_POINT('Ctrl Pts',(-29.5833932209651,-31.7591157661596,
49.5569937699189));
#37970=CARTESIAN_POINT('Ctrl Pts',(-30.8915902884901,-29.8391109584199,
49.6681235591387));
#37971=CARTESIAN_POINT('Ctrl Pts',(-33.2141919037862,-29.8967283676685,
49.7792533483584));
#37972=CARTESIAN_POINT('Ctrl Pts',(-34.4255782561001,-31.8792371657958,
49.8903831375781));
#37973=CARTESIAN_POINT('Ctrl Pts',(-33.417101692732,-33.9722668001683,50.0015129267978));
#37974=CARTESIAN_POINT('Ctrl Pts',(-31.1117090280035,-34.2602992473698,
50.1126427160177));
#37975=CARTESIAN_POINT('Ctrl Pts',(-29.6192706277318,-32.4797303353027,
50.2237725052373));
#37976=CARTESIAN_POINT('Ctrl Pts',(-30.3056499310248,-30.2601174228259,
50.3349022944571));
#37977=CARTESIAN_POINT('Ctrl Pts',(-32.5426800429829,-29.6328261767372,
50.4460320836768));
#37978=CARTESIAN_POINT('Ctrl Pts',(-34.2830552647223,-31.1719467427689,
50.5571618728965));
#37979=CARTESIAN_POINT('Ctrl Pts',(-33.9340030668927,-33.4688926699519,
50.6682916621162));
#37980=CARTESIAN_POINT('Ctrl Pts',(-31.8149722356298,-34.4215239550785,
50.7794214513359));
#37981=CARTESIAN_POINT('Ctrl Pts',(-29.8652768077821,-33.1580027768393,
50.8905512405557));
#37982=CARTESIAN_POINT('Ctrl Pts',(-29.8692568953308,-30.8346900152772,
51.0016810297753));
#37983=CARTESIAN_POINT('Ctrl Pts',(-31.8232699653508,-29.5778563144268,
51.1128108189952));
#37984=CARTESIAN_POINT('Ctrl Pts',(-33.9390244464751,-30.5377422476497,
51.2239406082148));
#37985=CARTESIAN_POINT('Ctrl Pts',(-34.2802047821274,-32.8358706181179,
51.3350703974346));
#37986=CARTESIAN_POINT('Ctrl Pts',(-32.5345664287748,-34.3690192638818,
51.4462001866543));
#37987=CARTESIAN_POINT('Ctrl Pts',(-30.2996986773214,-33.7340671695768,
51.557329975874));
#37988=CARTESIAN_POINT('Ctrl Pts',(-29.6209282566264,-31.5121156082528,
51.6684597650938));
#37989=CARTESIAN_POINT('Ctrl Pts',(-31.119458497007,-29.7366705485938,51.7795895543135));
#37990=CARTESIAN_POINT('Ctrl Pts',(-33.4238507688844,-30.0326000635722,
51.8907193435332));
#37991=CARTESIAN_POINT('Ctrl Pts',(-34.4251502639725,-32.1290726539236,
52.001849132753));
#37992=CARTESIAN_POINT('Ctrl Pts',(-33.2069785255006,-34.1074193726832,
52.1129789219726));
#37993=CARTESIAN_POINT('Ctrl Pts',(-30.8841931526569,-34.1570786929198,
52.2241087111924));
#37994=CARTESIAN_POINT('Ctrl Pts',(-29.5825820604857,-32.2326030703908,
52.3352385004121));
#37995=CARTESIAN_POINT('Ctrl Pts',(-30.4933657410223,-30.0952514731161,
52.4463682896319));
#37996=CARTESIAN_POINT('Ctrl Pts',(-32.7830045778855,-29.7011054025381,
52.5574980788515));
#37997=CARTESIAN_POINT('Ctrl Pts',(-34.3560464702414,-31.4108820816923,
52.6686278680714));
#37998=CARTESIAN_POINT('Ctrl Pts',(-33.7728594827364,-33.6598143885419,
52.779757657291));
#37999=CARTESIAN_POINT('Ctrl Pts',(-31.5671721094895,-34.389699997922,52.8908874465108));
#38000=CARTESIAN_POINT('Ctrl Pts',(-29.7576013817629,-32.9325631706899,
53.0020172357305));
#38001=CARTESIAN_POINT('Ctrl Pts',(-30.0002549884253,-30.6219445728053,
53.1131470249502));
#38002=CARTESIAN_POINT('Ctrl Pts',(-32.0730427793273,-29.5725272947448,
53.2242768141699));
#38003=CARTESIAN_POINT('Ctrl Pts',(-34.0790039218848,-30.7446672388737,
53.3354066033898));
#38004=CARTESIAN_POINT('Ctrl Pts',(-34.1822410279863,-33.0657522628949,
53.4465363926093));
#38005=CARTESIAN_POINT('Ctrl Pts',(-32.2883983467057,-34.4113176464284,
53.5576661818292));
#38006=CARTESIAN_POINT('Ctrl Pts',(-30.1304512362118,-33.5503776154227,
53.6687959710488));
#38007=CARTESIAN_POINT('Ctrl Pts',(-29.6838223376843,-31.2699421765937,
53.7799257602686));
#38008=CARTESIAN_POINT('Ctrl Pts',(-31.3562856770569,-29.6588500676751,
53.8910555494883));
#38009=CARTESIAN_POINT('Ctrl Pts',(-33.6191546587482,-30.1879569501259,
54.002185338708));
#38010=CARTESIAN_POINT('Ctrl Pts',(-34.3976272254265,-32.3803532230823,
54.1133151279277));
#38011=CARTESIAN_POINT('Ctrl Pts',(-33.4572031808897,-33.6016627022545,
54.1874016540742));
#38012=CARTESIAN_POINT('Ctrl Pts',(-32.8326019491389,-33.878502477185,54.2244449171475));
#38013=CARTESIAN_POINT('Ctrl Pts',(-31.5032651029123,-33.8599788000028,
40.9251850276175));
#38014=CARTESIAN_POINT('Ctrl Pts',(-30.8848229855226,-33.6948146693493,
40.9622282906908));
#38015=CARTESIAN_POINT('Ctrl Pts',(-29.8363898994693,-32.7015640496904,
41.0363148168372));
#38016=CARTESIAN_POINT('Ctrl Pts',(-30.2372657592897,-30.5589604759703,
41.147444606057));
#38017=CARTESIAN_POINT('Ctrl Pts',(-32.2544678981807,-29.7393671856248,
41.2585743952767));
#38018=CARTESIAN_POINT('Ctrl Pts',(-34.0372449179009,-30.9866503162908,
41.3697041844964));
#38019=CARTESIAN_POINT('Ctrl Pts',(-33.9563329101449,-33.162358336938,41.4808339737161));
#38020=CARTESIAN_POINT('Ctrl Pts',(-32.084614731564,-34.2737749035779,41.5919637629359));
#38021=CARTESIAN_POINT('Ctrl Pts',(-30.1356558010849,-33.3045167553556,
41.7030935521555));
#38022=CARTESIAN_POINT('Ctrl Pts',(-29.8928245920533,-31.1412479943015,
41.8142233413754));
#38023=CARTESIAN_POINT('Ctrl Pts',(-31.5785079087858,-29.763965935017,41.925353130595));
#38024=CARTESIAN_POINT('Ctrl Pts',(-33.6499107379646,-30.4330445770664,
42.0364829198149));
#38025=CARTESIAN_POINT('Ctrl Pts',(-34.2113460212012,-32.5362007124115,
42.1476127090345));
#38026=CARTESIAN_POINT('Ctrl Pts',(-32.7489749069529,-34.1486232431348,
42.2587424982543));
#38027=CARTESIAN_POINT('Ctrl Pts',(-30.6011533631931,-33.7946533897167,
42.3698722874739));
#38028=CARTESIAN_POINT('Ctrl Pts',(-29.7335394333561,-31.7982340407573,
42.4810020766937));
#38029=CARTESIAN_POINT('Ctrl Pts',(-30.9401664729187,-29.9864698084441,
42.5921318659134));
#38030=CARTESIAN_POINT('Ctrl Pts',(-33.1167412400144,-30.0174660166224,
42.7032616551331));
#38031=CARTESIAN_POINT('Ctrl Pts',(-34.2712867484736,-31.8628561070233,
42.8143914443529));
#38032=CARTESIAN_POINT('Ctrl Pts',(-33.3471751478867,-33.8337586594261,
42.9255212335726));
#38033=CARTESIAN_POINT('Ctrl Pts',(-31.1901435159702,-34.1264252445205,
43.0366510227923));
#38034=CARTESIAN_POINT('Ctrl Pts',(-29.7742837281775,-32.4730104698306,
43.147780812012));
#38035=CARTESIAN_POINT('Ctrl Pts',(-30.3953753493751,-30.3867016609807,
43.2589106012318));
#38036=CARTESIAN_POINT('Ctrl Pts',(-32.4850020423711,-29.7768659872946,
43.3700403904515));
#38037=CARTESIAN_POINT('Ctrl Pts',(-34.1307601293648,-31.2016184578062,
43.4811701796712));
#38038=CARTESIAN_POINT('Ctrl Pts',(-33.8264696513034,-33.3570410552955,
43.592299968891));
#38039=CARTESIAN_POINT('Ctrl Pts',(-31.8506139565128,-34.2705143966632,
43.7034297581107));
#38040=CARTESIAN_POINT('Ctrl Pts',(-30.0114747482403,-33.1060375843082,
43.8145595473304));
#38041=CARTESIAN_POINT('Ctrl Pts',(-29.9922122859509,-30.9293271695755,
43.9256893365501));
#38042=CARTESIAN_POINT('Ctrl Pts',(-31.8104553658915,-29.7324849181309,
44.0368191257699));
#38043=CARTESIAN_POINT('Ctrl Pts',(-33.8021676395011,-30.610847879513,44.1479489149896));
#38044=CARTESIAN_POINT('Ctrl Pts',(-34.1445556331039,-32.7605477967984,
44.2590787042093));
#38045=CARTESIAN_POINT('Ctrl Pts',(-32.5242695680424,-34.2142026182709,
44.370208493429));
#38046=CARTESIAN_POINT('Ctrl Pts',(-30.4241776797676,-33.6414432155195,
44.4813382826488));
#38047=CARTESIAN_POINT('Ctrl Pts',(-29.766261289892,-31.56645278264,44.5924680718685));
#38048=CARTESIAN_POINT('Ctrl Pts',(-31.1526383436176,-29.8882400614621,
44.7035978610882));
#38049=CARTESIAN_POINT('Ctrl Pts',(-33.3145115960109,-30.1426871349524,
44.8147276503079));
#38050=CARTESIAN_POINT('Ctrl Pts',(-34.2733580910192,-32.0969268008144,
44.9258574395277));
#38051=CARTESIAN_POINT('Ctrl Pts',(-33.1516519146688,-33.9624601096987,
45.0369872287474));
#38052=CARTESIAN_POINT('Ctrl Pts',(-30.9759663951584,-34.0319712081804,
45.1481170179671));
#38053=CARTESIAN_POINT('Ctrl Pts',(-29.7374653256171,-32.2418442927456,
45.2592468071868));
#38054=CARTESIAN_POINT('Ctrl Pts',(-30.5696114539041,-30.2303841032822,
45.3703765964066));
#38055=CARTESIAN_POINT('Ctrl Pts',(-32.7108336676603,-29.8384571918097,
45.4815063856263));
#38056=CARTESIAN_POINT('Ctrl Pts',(-34.2015086174439,-31.4247508174373,
45.5926361748461));
#38057=CARTESIAN_POINT('Ctrl Pts',(-33.6773867549097,-33.5375062566287,
45.7037659640658));
#38058=CARTESIAN_POINT('Ctrl Pts',(-31.618138724784,-34.2431526433146,45.8148957532855));
#38059=CARTESIAN_POINT('Ctrl Pts',(-29.908365992623,-32.8958900568164,45.9260255425052));
#38060=CARTESIAN_POINT('Ctrl Pts',(-30.1128340211871,-30.728718605843,46.037155331725));
#38061=CARTESIAN_POINT('Ctrl Pts',(-32.044415888098,-29.7250101003294,46.1482851209446));
#38062=CARTESIAN_POINT('Ctrl Pts',(-33.9353488158918,-30.8033476797562,
46.2594149101645));
#38063=CARTESIAN_POINT('Ctrl Pts',(-34.0550714953655,-32.9768484855161,
46.3705446993841));
#38064=CARTESIAN_POINT('Ctrl Pts',(-32.294015028603,-34.2563481508123,46.4816744886038));
#38065=CARTESIAN_POINT('Ctrl Pts',(-30.2638791961233,-33.4708624575619,
46.5928042778236));
#38066=CARTESIAN_POINT('Ctrl Pts',(-29.8226222959054,-31.3392593939899,
46.7039340670433));
#38067=CARTESIAN_POINT('Ctrl Pts',(-31.374077857797,-29.8123589676049,46.815063856263));
#38068=CARTESIAN_POINT('Ctrl Pts',(-33.4983705763898,-30.2875638900887,
46.9261936454827));
#38069=CARTESIAN_POINT('Ctrl Pts',(-34.2513707926229,-32.329971769767,47.0373234347024));
#38070=CARTESIAN_POINT('Ctrl Pts',(-32.9439408745472,-34.0703930641495,
47.1484532239223));
#38071=CARTESIAN_POINT('Ctrl Pts',(-30.7726265046983,-33.9160130787,47.2595830131419));
#38072=CARTESIAN_POINT('Ctrl Pts',(-29.7245910474383,-32.0081187019211,
47.3707128023617));
#38073=CARTESIAN_POINT('Ctrl Pts',(-30.7589851877802,-30.0927941771875,
47.4818425915813));
#38074=CARTESIAN_POINT('Ctrl Pts',(-32.9291426260204,-29.9229237387061,
47.5929723808012));
#38075=CARTESIAN_POINT('Ctrl Pts',(-34.248958809059,-31.6539709696068,47.7041021700208));
#38076=CARTESIAN_POINT('Ctrl Pts',(-33.5105522789894,-33.7017002165947,
47.8152319592406));
#38077=CARTESIAN_POINT('Ctrl Pts',(-31.3897046844462,-34.1920518795256,
47.9263617484603));
#38078=CARTESIAN_POINT('Ctrl Pts',(-29.8273927443206,-32.6762614341274,
48.03749153768));
#38079=CARTESIAN_POINT('Ctrl Pts',(-30.2534274036483,-30.5415638579657,
48.1486213268997));
#38080=CARTESIAN_POINT('Ctrl Pts',(-32.2779063623659,-29.7416112229124,
48.2597511161195));
#38081=CARTESIAN_POINT('Ctrl Pts',(-34.0480484320153,-31.0085115054432,
48.3708809053392));
#38082=CARTESIAN_POINT('Ctrl Pts',(-33.9438387868447,-33.1828113059475,
48.482010694559));
#38083=CARTESIAN_POINT('Ctrl Pts',(-32.0606489640076,-34.274615026303,48.5931404837787));
#38084=CARTESIAN_POINT('Ctrl Pts',(-30.1219538670215,-33.2847157417589,
48.7042702729984));
#38085=CARTESIAN_POINT('Ctrl Pts',(-29.902026224375,-31.1190585425191,48.8154000622181));
#38086=CARTESIAN_POINT('Ctrl Pts',(-31.6021414296023,-29.7596294117535,
48.9265298514378));
#38087=CARTESIAN_POINT('Ctrl Pts',(-33.6663724838611,-30.4505631475438,
49.0376596406575));
#38088=CARTESIAN_POINT('Ctrl Pts',(-34.2055575119472,-32.559524687759,49.1487894298773));
#38089=CARTESIAN_POINT('Ctrl Pts',(-32.7262402233745,-34.1564153015298,
49.259919219097));
#38090=CARTESIAN_POINT('Ctrl Pts',(-30.5822757581167,-33.7797780166906,
49.3710490083167));
#38091=CARTESIAN_POINT('Ctrl Pts',(-29.7357971444513,-31.7743071918651,
49.4821787975364));
#38092=CARTESIAN_POINT('Ctrl Pts',(-30.9614924299265,-29.9753879775081,
49.5933085867562));
#38093=CARTESIAN_POINT('Ctrl Pts',(-33.1376185813874,-30.0293717301325,
49.7044383759759));
#38094=CARTESIAN_POINT('Ctrl Pts',(-34.2726085441223,-31.886853104766,49.8155681651957));
#38095=CARTESIAN_POINT('Ctrl Pts',(-33.3277318126898,-33.8478852908906,
49.9266979544153));
#38096=CARTESIAN_POINT('Ctrl Pts',(-31.1677293249357,-34.1177528982737,
50.0378277436351));
#38097=CARTESIAN_POINT('Ctrl Pts',(-29.7694119334007,-32.4494760192304,
50.1489575328548));
#38098=CARTESIAN_POINT('Ctrl Pts',(-30.412504550697,-30.3698435617522,50.2600873220745));
#38099=CARTESIAN_POINT('Ctrl Pts',(-32.5084557875245,-29.7821125982472,
50.3712171112943));
#38100=CARTESIAN_POINT('Ctrl Pts',(-34.1390738015822,-31.2241681328405,
50.482346900514));
#38101=CARTESIAN_POINT('Ctrl Pts',(-33.8120346697228,-33.3762565787091,
50.5934766897338));
#38102=CARTESIAN_POINT('Ctrl Pts',(-31.8266410588278,-34.2688099286297,
50.7046064789534));
#38103=CARTESIAN_POINT('Ctrl Pts',(-29.9999036709001,-33.0849730360767,
50.8157362681733));
#38104=CARTESIAN_POINT('Ctrl Pts',(-30.0036327532113,-30.9081805869706,
50.9268660573928));
#38105=CARTESIAN_POINT('Ctrl Pts',(-31.8344154901056,-29.7306094243374,
51.0379958466127));
#38106=CARTESIAN_POINT('Ctrl Pts',(-33.8167393747198,-30.6299599061201,
51.1491256358324));
#38107=CARTESIAN_POINT('Ctrl Pts',(-34.1364030854,-32.7831562241863,51.2602554250521));
#38108=CARTESIAN_POINT('Ctrl Pts',(-32.5008538604679,-34.2196164591879,
51.3713852142718));
#38109=CARTESIAN_POINT('Ctrl Pts',(-30.4069286143277,-33.6247077808154,
51.4825150034915));
#38110=CARTESIAN_POINT('Ctrl Pts',(-29.7709650235058,-31.5428841619766,
51.5936447927113));
#38111=CARTESIAN_POINT('Ctrl Pts',(-31.1749900716979,-29.8794079982809,
51.704774581931));
#38112=CARTESIAN_POINT('Ctrl Pts',(-33.3340552566317,-30.1566746428456,
51.8159043711507));
#38113=CARTESIAN_POINT('Ctrl Pts',(-34.2722075434275,-32.1209326540513,
51.9270341603704));
#38114=CARTESIAN_POINT('Ctrl Pts',(-33.130860116645,-33.974514431915,52.0381639495902));
#38115=CARTESIAN_POINT('Ctrl Pts',(-30.9545617963531,-34.0210419744427,
52.1492937388099));
#38116=CARTESIAN_POINT('Ctrl Pts',(-29.7350371400147,-32.2179338983725,
52.2604235280296));
#38117=CARTESIAN_POINT('Ctrl Pts',(-30.5883820152126,-30.2153749252516,
52.3715533172494));
#38118=CARTESIAN_POINT('Ctrl Pts',(-32.7336241942779,-29.8460857772412,
52.482683106469));
#38119=CARTESIAN_POINT('Ctrl Pts',(-34.2074617980904,-31.4480349536138,
52.5938128956888));
#38120=CARTESIAN_POINT('Ctrl Pts',(-33.6610536468417,-33.5551377703734,
52.7049426849085));
#38121=CARTESIAN_POINT('Ctrl Pts',(-31.5944685109066,-34.238992957456,52.8160724741283));
#38122=CARTESIAN_POINT('Ctrl Pts',(-29.8990188231126,-32.8737508362444,
52.9272022633479));
#38123=CARTESIAN_POINT('Ctrl Pts',(-30.1263694181206,-30.7088519901427,
53.0383320525678));
#38124=CARTESIAN_POINT('Ctrl Pts',(-32.068436317801,-29.7256164806422,53.1494618417873));
#38125=CARTESIAN_POINT('Ctrl Pts',(-33.9478910087757,-30.823835119944,53.2605916310073));
#38126=CARTESIAN_POINT('Ctrl Pts',(-34.0446174404242,-32.9985403243459,
53.3717214202267));
#38127=CARTESIAN_POINT('Ctrl Pts',(-32.2702104313418,-34.2592472834404,
53.4828512094467));
#38128=CARTESIAN_POINT('Ctrl Pts',(-30.2483548063011,-33.4526026552904,
53.5939809986663));
#38129=CARTESIAN_POINT('Ctrl Pts',(-29.8298926732848,-31.3159834596125,
53.7051107878861));
#38130=CARTESIAN_POINT('Ctrl Pts',(-31.3968816851753,-29.8064952858593,
53.8162405771058));
#38131=CARTESIAN_POINT('Ctrl Pts',(-33.5170422568196,-30.3022339076858,
53.9273703663255));
#38132=CARTESIAN_POINT('Ctrl Pts',(-34.2464202523342,-32.3563661499634,
54.0385001555453));
#38133=CARTESIAN_POINT('Ctrl Pts',(-33.3653042902589,-33.5006534350279,
54.1125866816917));
#38134=CARTESIAN_POINT('Ctrl Pts',(-32.7800936946509,-33.7600342388745,
54.149629944765));
#38135=CARTESIAN_POINT('Ctrl Pts',(-31.5367004230132,-33.7347832743338,
40.850370055235));
#38136=CARTESIAN_POINT('Ctrl Pts',(-30.9598857617979,-33.5807363726288,
40.8874133183083));
#38137=CARTESIAN_POINT('Ctrl Pts',(-29.9820229055434,-32.6543416404935,
40.9614998444548));
#38138=CARTESIAN_POINT('Ctrl Pts',(-30.3559157352357,-30.6559571195451,
41.0726296336744));
#38139=CARTESIAN_POINT('Ctrl Pts',(-32.2373396157086,-29.8915308089627,
41.1837594228943));
#38140=CARTESIAN_POINT('Ctrl Pts',(-33.9001175762276,-31.0548590756262,
41.2948892121139));
#38141=CARTESIAN_POINT('Ctrl Pts',(-33.8246517710542,-33.0841197769025,
41.4060190013337));
#38142=CARTESIAN_POINT('Ctrl Pts',(-32.0789192979399,-34.1207266837241,
41.5171487905534));
#38143=CARTESIAN_POINT('Ctrl Pts',(-30.2611451625824,-33.2167094852241,
41.6282785797731));
#38144=CARTESIAN_POINT('Ctrl Pts',(-30.03465896827,-31.1990507546193,41.7394083689928));
#38145=CARTESIAN_POINT('Ctrl Pts',(-31.6068786213577,-29.9144738118696,
41.8505381582125));
#38146=CARTESIAN_POINT('Ctrl Pts',(-33.5388549333791,-30.5385166436693,
41.9616679474323));
#38147=CARTESIAN_POINT('Ctrl Pts',(-34.0624999012563,-32.5001089407987,
42.072797736652));
#38148=CARTESIAN_POINT('Ctrl Pts',(-32.6985612639648,-34.0039990052734,
42.1839275258718));
#38149=CARTESIAN_POINT('Ctrl Pts',(-30.6953099955295,-33.6738549297995,
42.2950573150914));
#38150=CARTESIAN_POINT('Ctrl Pts',(-29.8860953238041,-31.8118149457275,
42.4061871043112));
#38151=CARTESIAN_POINT('Ctrl Pts',(-31.0115040685646,-30.1220009073909,
42.5173168935309));
#38152=CARTESIAN_POINT('Ctrl Pts',(-33.0415731754216,-30.15091075492,42.6284466827507));
#38153=CARTESIAN_POINT('Ctrl Pts',(-34.1184060068116,-31.8720872884612,
42.7395764719704));
#38154=CARTESIAN_POINT('Ctrl Pts',(-33.2564965332661,-33.7103280163905,
42.8507062611901));
#38155=CARTESIAN_POINT('Ctrl Pts',(-31.2446551094542,-33.9832951581544,
42.9618360504098));
#38156=CARTESIAN_POINT('Ctrl Pts',(-29.9240971124162,-32.4411720454263,
43.0729658396296));
#38157=CARTESIAN_POINT('Ctrl Pts',(-30.5033829388359,-30.4952930780518,
43.1840956288492));
#38158=CARTESIAN_POINT('Ctrl Pts',(-32.4523564629456,-29.9265055591826,
43.2952254180691));
#38159=CARTESIAN_POINT('Ctrl Pts',(-33.987338261078,-31.2553576707796,43.4063552072887));
#38160=CARTESIAN_POINT('Ctrl Pts',(-33.7035296327865,-33.2656983645767,
43.5174849965085));
#38161=CARTESIAN_POINT('Ctrl Pts',(-31.8606691594226,-34.1176856421479,
43.6286147857282));
#38162=CARTESIAN_POINT('Ctrl Pts',(-30.1453227599487,-33.0315899848104,
43.7397445749479));
#38163=CARTESIAN_POINT('Ctrl Pts',(-30.127356857648,-31.0013943607845,43.8508743641676));
#38164=CARTESIAN_POINT('Ctrl Pts',(-31.8232136511498,-29.8851117881987,
43.9620041533874));
#38165=CARTESIAN_POINT('Ctrl Pts',(-33.6808633940062,-30.7043519721179,
44.0731339426071));
#38166=CARTESIAN_POINT('Ctrl Pts',(-34.0002051868448,-32.7093551804006,
44.1842637318269));
#38167=CARTESIAN_POINT('Ctrl Pts',(-32.4889808840191,-34.0651642202357,
44.2953935210465));
#38168=CARTESIAN_POINT('Ctrl Pts',(-30.5302465789089,-33.5309573614752,
44.4065233102663));
#38169=CARTESIAN_POINT('Ctrl Pts',(-29.9166146659727,-31.5956349280385,
44.517653099486));
#38170=CARTESIAN_POINT('Ctrl Pts',(-31.2096744173634,-30.030383023302,44.6287828887057));
#38171=CARTESIAN_POINT('Ctrl Pts',(-33.2260315712599,-30.2677032160341,
44.7399126779254));
#38172=CARTESIAN_POINT('Ctrl Pts',(-34.1203379268977,-32.0904026394748,
44.8510424671452));
#38173=CARTESIAN_POINT('Ctrl Pts',(-33.0741340059462,-33.8303665476442,
44.9621722563649));
#38174=CARTESIAN_POINT('Ctrl Pts',(-31.044894291251,-33.8951988409082,45.0733020455846));
#38175=CARTESIAN_POINT('Ctrl Pts',(-29.8897569635127,-32.2255657075486,
45.1844318348043));
#38176=CARTESIAN_POINT('Ctrl Pts',(-30.6658911781349,-30.3494972847988,
45.2955616240241));
#38177=CARTESIAN_POINT('Ctrl Pts',(-32.6629873187203,-29.9839510480444,
45.4066914132438));
#38178=CARTESIAN_POINT('Ctrl Pts',(-34.053324655011,-31.4634709489793,45.5178212024635));
#38179=CARTESIAN_POINT('Ctrl Pts',(-33.5644815344143,-33.4340164189931,
45.6289509916833));
#38180=CARTESIAN_POINT('Ctrl Pts',(-31.6438418796174,-34.0921656136048,
45.740080780903));
#38181=CARTESIAN_POINT('Ctrl Pts',(-30.0491542742207,-32.8355875272368,
45.8512105701227));
#38182=CARTESIAN_POINT('Ctrl Pts',(-30.2398595210163,-30.814288797511,45.9623403593425));
#38183=CARTESIAN_POINT('Ctrl Pts',(-32.0414262462491,-29.8781401018006,
46.0734701485621));
#38184=CARTESIAN_POINT('Ctrl Pts',(-33.8050801201637,-30.8838945743099,
46.1845999377819));
#38185=CARTESIAN_POINT('Ctrl Pts',(-33.9167442433832,-32.9110966287515,
46.2957297270016));
#38186=CARTESIAN_POINT('Ctrl Pts',(-32.2742248212842,-34.1044729289912,
46.4068595162214));
#38187=CARTESIAN_POINT('Ctrl Pts',(-30.3807378165902,-33.3718584266768,
46.517989305441));
#38188=CARTESIAN_POINT('Ctrl Pts',(-29.9691820019857,-31.3837339694529,
46.6291190946608));
#38189=CARTESIAN_POINT('Ctrl Pts',(-31.4162087958597,-29.959609500259,46.7402488838805));
#38190=CARTESIAN_POINT('Ctrl Pts',(-33.397514968811,-30.4028282893144,46.8513786731003));
#38191=CARTESIAN_POINT('Ctrl Pts',(-34.0998305977251,-32.3077613073833,
46.96250846232));
#38192=CARTESIAN_POINT('Ctrl Pts',(-32.8804040353159,-33.9310345144675,
47.0736382515397));
#38193=CARTESIAN_POINT('Ctrl Pts',(-30.8552412473697,-33.7870458751082,
47.1847680407594));
#38194=CARTESIAN_POINT('Ctrl Pts',(-29.8777492554391,-32.0075722305555,
47.2958978299792));
#38195=CARTESIAN_POINT('Ctrl Pts',(-30.8425181300796,-30.2211685627158,
47.4070276191989));
#38196=CARTESIAN_POINT('Ctrl Pts',(-32.8666018597031,-30.062732135655,47.5181574084186));
#38197=CARTESIAN_POINT('Ctrl Pts',(-34.0975809652322,-31.6772622492475,
47.6292871976383));
#38198=CARTESIAN_POINT('Ctrl Pts',(-33.408876718699,-33.5871584523836,47.7404169868581));
#38199=CARTESIAN_POINT('Ctrl Pts',(-31.4307837778444,-34.0445044519149,
47.8515467760778));
#38200=CARTESIAN_POINT('Ctrl Pts',(-29.9736313506136,-32.6307421487812,
47.9626765652975));
#38201=CARTESIAN_POINT('Ctrl Pts',(-30.3709895362484,-30.6397314711967,
48.0738063545172));
#38202=CARTESIAN_POINT('Ctrl Pts',(-32.2592004324257,-29.8936237996751,
48.184936143737));
#38203=CARTESIAN_POINT('Ctrl Pts',(-33.9101939037587,-31.075248783992,48.2960659329567));
#38204=CARTESIAN_POINT('Ctrl Pts',(-33.8129986295621,-33.1031960526903,
48.4071957221765));
#38205=CARTESIAN_POINT('Ctrl Pts',(-32.0565666707416,-34.1215102576292,
48.5183255113961));
#38206=CARTESIAN_POINT('Ctrl Pts',(-30.2483655082985,-33.1982412816068,
48.6294553006159));
#38207=CARTESIAN_POINT('Ctrl Pts',(-30.0432412369755,-31.1783548790433,
48.7405850898356));
#38208=CARTESIAN_POINT('Ctrl Pts',(-31.6289213654074,-29.9104291808092,
48.8517148790554));
#38209=CARTESIAN_POINT('Ctrl Pts',(-33.5542086360382,-30.5548560358465,
48.962844668275));
#38210=CARTESIAN_POINT('Ctrl Pts',(-34.0571010176577,-32.5218629749434,
49.0739744574949));
#38211=CARTESIAN_POINT('Ctrl Pts',(-32.6773568562484,-34.0112665787405,
49.1851042467145));
#38212=CARTESIAN_POINT('Ctrl Pts',(-30.6777030456298,-33.659980820952,49.2962340359343));
#38213=CARTESIAN_POINT('Ctrl Pts',(-29.8882010679375,-31.7894986175706,
49.407363825154));
#38214=CARTESIAN_POINT('Ctrl Pts',(-31.0313945713629,-30.1116649965963,
49.5184936143737));
#38215=CARTESIAN_POINT('Ctrl Pts',(-33.0610452589886,-30.1620150925965,
49.6296234035934));
#38216=CARTESIAN_POINT('Ctrl Pts',(-34.1196388321445,-31.8944690437362,
49.7407531928132));
#38217=CARTESIAN_POINT('Ctrl Pts',(-33.2383619326478,-33.7235037816128,
49.8518829820328));
#38218=CARTESIAN_POINT('Ctrl Pts',(-31.2237496218677,-33.9752065491778,
49.9630127712527));
#38219=CARTESIAN_POINT('Ctrl Pts',(-29.9195532390696,-32.4192217031581,
50.0741425604723));
#38220=CARTESIAN_POINT('Ctrl Pts',(-30.5193591703691,-30.4795697006785,
50.1852723496921));
#38221=CARTESIAN_POINT('Ctrl Pts',(-32.4742315320661,-29.9313990197574,
50.2964021389118));
#38222=CARTESIAN_POINT('Ctrl Pts',(-33.9950923384422,-31.276389522912,50.4075319281315));
#38223=CARTESIAN_POINT('Ctrl Pts',(-33.6900662725529,-33.2836204874662,
50.5186617173512));
#38224=CARTESIAN_POINT('Ctrl Pts',(-31.8383098820259,-34.116095902181,50.629791506571));
#38225=CARTESIAN_POINT('Ctrl Pts',(-30.134530534018,-33.011943295314,50.7409212957907));
#38226=CARTESIAN_POINT('Ctrl Pts',(-30.1380086110919,-30.981671158664,50.8520510850104));
#38227=CARTESIAN_POINT('Ctrl Pts',(-31.8455610148604,-29.883362534248,50.9631808742302));
#38228=CARTESIAN_POINT('Ctrl Pts',(-33.6944543029646,-30.7221775645905,
51.0743106634498));
#38229=CARTESIAN_POINT('Ctrl Pts',(-33.9926013886726,-32.7304418302546,
51.1854404526696));
#38230=CARTESIAN_POINT('Ctrl Pts',(-32.4671412921609,-34.0702136544941,
51.2965702418893));
#38231=CARTESIAN_POINT('Ctrl Pts',(-30.5141585513341,-33.5153483920539,
51.407700031109));
#38232=CARTESIAN_POINT('Ctrl Pts',(-29.9210017903852,-31.5736527157003,
51.5188298203288));
#38233=CARTESIAN_POINT('Ctrl Pts',(-31.2305216463888,-30.0221454479681,
51.6299596095485));
#38234=CARTESIAN_POINT('Ctrl Pts',(-33.244259744379,-30.280749222119,51.7410893987682));
#38235=CARTESIAN_POINT('Ctrl Pts',(-34.1192648228826,-32.112792654179,51.852219187988));
#38236=CARTESIAN_POINT('Ctrl Pts',(-33.0547417077894,-33.8416094911468,
51.9633489772076));
#38237=CARTESIAN_POINT('Ctrl Pts',(-31.0249304400494,-33.8850052559656,
52.0744787664275));
#38238=CARTESIAN_POINT('Ctrl Pts',(-29.8874922195436,-32.203264726354,52.1856085556471));
#38239=CARTESIAN_POINT('Ctrl Pts',(-30.683398289403,-30.335498377387,52.2967383448669));
#38240=CARTESIAN_POINT('Ctrl Pts',(-32.6842438106703,-29.9910661519442,
52.4078681340866));
#38241=CARTESIAN_POINT('Ctrl Pts',(-34.0588771259395,-31.4851878255353,
52.5189979233063));
#38242=CARTESIAN_POINT('Ctrl Pts',(-33.549247810947,-33.4504611522048,52.630127712526));
#38243=CARTESIAN_POINT('Ctrl Pts',(-31.6217649123239,-34.0882859169901,
52.7412575017457));
#38244=CARTESIAN_POINT('Ctrl Pts',(-30.0404362644622,-32.8149385017989,
52.8523872909655));
#38245=CARTESIAN_POINT('Ctrl Pts',(-30.2524838478161,-30.79575940748,52.9635170801852));
#38246=CARTESIAN_POINT('Ctrl Pts',(-32.0638298562746,-29.8787056665396,
53.0746468694049));
#38247=CARTESIAN_POINT('Ctrl Pts',(-33.8167780956667,-30.9030030010144,
53.1857766586247));
#38248=CARTESIAN_POINT('Ctrl Pts',(-33.9069938528621,-32.931328385797,53.2969064478444));
#38249=CARTESIAN_POINT('Ctrl Pts',(-32.252022515978,-34.1071769204523,53.4080362370642));
#38250=CARTESIAN_POINT('Ctrl Pts',(-30.3662583763903,-33.3548276951581,
53.5191660262838));
#38251=CARTESIAN_POINT('Ctrl Pts',(-29.9759630088853,-31.3620247426314,
53.6302958155036));
#38252=CARTESIAN_POINT('Ctrl Pts',(-31.4374776932937,-29.9541405040433,
53.7414256047233));
#38253=CARTESIAN_POINT('Ctrl Pts',(-33.414929854891,-30.4165108652457,53.852555393943));
#38254=CARTESIAN_POINT('Ctrl Pts',(-34.0952132792418,-32.3323790768444,
53.9636851831628));
#38255=CARTESIAN_POINT('Ctrl Pts',(-33.2734053996281,-33.3996441678013,
54.0377717093093));
#38256=CARTESIAN_POINT('Ctrl Pts',(-32.7275854401629,-33.6415660005639,
54.0748149723825));
#38257=CARTESIAN_POINT('Ctrl Pts',(-31.5701357431141,-33.6095877486649,
40.7755550828525));
#38258=CARTESIAN_POINT('Ctrl Pts',(-31.0349485380732,-33.4666580759082,
40.8125983459258));
#38259=CARTESIAN_POINT('Ctrl Pts',(-30.1276559116176,-32.6071192312965,
40.8866848720723));
#38260=CARTESIAN_POINT('Ctrl Pts',(-30.4745657111817,-30.75295376312,40.997814661292));
#38261=CARTESIAN_POINT('Ctrl Pts',(-32.2202113332364,-30.0436944323007,
41.1089444505117));
#38262=CARTESIAN_POINT('Ctrl Pts',(-33.7629902345544,-31.1230678349617,
41.2200742397315));
#38263=CARTESIAN_POINT('Ctrl Pts',(-33.6929706319633,-33.0058812168671,
41.3312040289511));
#38264=CARTESIAN_POINT('Ctrl Pts',(-32.073223864316,-33.9676784638702,41.4423338181709));
#38265=CARTESIAN_POINT('Ctrl Pts',(-30.3866345240797,-33.1289022150926,
41.5534636073906));
#38266=CARTESIAN_POINT('Ctrl Pts',(-30.1764933444867,-31.256853514937,41.6645933966103));
#38267=CARTESIAN_POINT('Ctrl Pts',(-31.6352493339297,-30.0649816887222,
41.7757231858301));
#38268=CARTESIAN_POINT('Ctrl Pts',(-33.4277991287936,-30.6439887102723,
41.8868529750498));
#38269=CARTESIAN_POINT('Ctrl Pts',(-33.9136537813114,-32.4640171691859,
41.9979827642695));
#38270=CARTESIAN_POINT('Ctrl Pts',(-32.6481476209767,-33.8593747674119,
42.1091125534893));
#38271=CARTESIAN_POINT('Ctrl Pts',(-30.7894666278659,-33.5530564698822,
42.220242342709));
#38272=CARTESIAN_POINT('Ctrl Pts',(-30.0386512142522,-31.8253958506977,
42.3313721319287));
#38273=CARTESIAN_POINT('Ctrl Pts',(-31.0828416642105,-30.2575320063377,
42.4425019211484));
#38274=CARTESIAN_POINT('Ctrl Pts',(-32.9664051108288,-30.2843554932176,
42.5536317103682));
#38275=CARTESIAN_POINT('Ctrl Pts',(-33.9655252651496,-31.8813184698992,
42.6647614995879));
#38276=CARTESIAN_POINT('Ctrl Pts',(-33.1658179186456,-33.5868973733549,
42.7758912888076));
#38277=CARTESIAN_POINT('Ctrl Pts',(-31.2991667029381,-33.8401650717883,
42.8870210780273));
#38278=CARTESIAN_POINT('Ctrl Pts',(-30.073910496655,-32.4093336210221,42.9981508672471));
#38279=CARTESIAN_POINT('Ctrl Pts',(-30.6113905282966,-30.6038844951228,
43.1092806564668));
#38280=CARTESIAN_POINT('Ctrl Pts',(-32.4197108835201,-30.0761451310706,
43.2204104456865));
#38281=CARTESIAN_POINT('Ctrl Pts',(-33.8439163927912,-31.309096883753,43.3315402349062));
#38282=CARTESIAN_POINT('Ctrl Pts',(-33.5805896142696,-33.174355673858,43.442670024126));
#38283=CARTESIAN_POINT('Ctrl Pts',(-31.8707243623324,-33.9648568876327,
43.5537998133457));
#38284=CARTESIAN_POINT('Ctrl Pts',(-30.279170771657,-32.9571423853126,43.6649296025654));
#38285=CARTESIAN_POINT('Ctrl Pts',(-30.2625014293451,-31.0734615519935,
43.7760593917852));
#38286=CARTESIAN_POINT('Ctrl Pts',(-31.8359719364082,-30.0377386582665,
43.8871891810048));
#38287=CARTESIAN_POINT('Ctrl Pts',(-33.5595591485112,-30.7978560647227,
43.9983189702246));
#38288=CARTESIAN_POINT('Ctrl Pts',(-33.8558547405858,-32.6581625640029,
44.1094487594443));
#38289=CARTESIAN_POINT('Ctrl Pts',(-32.4536921999958,-33.9161258222004,
44.2205785486641));
#38290=CARTESIAN_POINT('Ctrl Pts',(-30.6363154780501,-33.4204715074308,
44.3317083378838));
#38291=CARTESIAN_POINT('Ctrl Pts',(-30.0669680420535,-31.6248170734369,
44.4428381271035));
#38292=CARTESIAN_POINT('Ctrl Pts',(-31.2667104911091,-30.172525985142,44.5539679163232));
#38293=CARTESIAN_POINT('Ctrl Pts',(-33.1375515465089,-30.3927192971158,
44.665097705543));
#38294=CARTESIAN_POINT('Ctrl Pts',(-33.9673177627762,-32.0838784781352,
44.7762274947627));
#38295=CARTESIAN_POINT('Ctrl Pts',(-32.9966160972236,-33.6982729855898,
44.8873572839825));
#38296=CARTESIAN_POINT('Ctrl Pts',(-31.1138221873434,-33.7584264736361,
44.9984870732021));
#38297=CARTESIAN_POINT('Ctrl Pts',(-30.0420486014084,-32.2092871223517,
45.1096168624219));
#38298=CARTESIAN_POINT('Ctrl Pts',(-30.7621709023656,-30.4686104663154,
45.2207466516416));
#38299=CARTESIAN_POINT('Ctrl Pts',(-32.6151409697803,-30.1294449042792,
45.3318764408613));
#38300=CARTESIAN_POINT('Ctrl Pts',(-33.905140692578,-31.5021910805214,45.443006230081));
#38301=CARTESIAN_POINT('Ctrl Pts',(-33.4515763139189,-33.3305265813575,
45.5541360193008));
#38302=CARTESIAN_POINT('Ctrl Pts',(-31.6695450344508,-33.9411785838951,
45.6652658085205));
#38303=CARTESIAN_POINT('Ctrl Pts',(-30.1899425558184,-32.7752849976571,
45.7763955977402));
#38304=CARTESIAN_POINT('Ctrl Pts',(-30.3668850208455,-30.899858989179,45.88752538696));
#38305=CARTESIAN_POINT('Ctrl Pts',(-32.0384366044002,-30.0312701032718,
45.9986551761797));
#38306=CARTESIAN_POINT('Ctrl Pts',(-33.6748114244356,-30.9644414688636,
46.1097849653994));
#38307=CARTESIAN_POINT('Ctrl Pts',(-33.778416991401,-32.8453447719867,46.2209147546191));
#38308=CARTESIAN_POINT('Ctrl Pts',(-32.2544346139655,-33.95259770717,46.3320445438389));
#38309=CARTESIAN_POINT('Ctrl Pts',(-30.4975964370572,-33.2728543957916,
46.4431743330586));
#38310=CARTESIAN_POINT('Ctrl Pts',(-30.115741708066,-31.4282085449159,46.5543041222783));
#38311=CARTESIAN_POINT('Ctrl Pts',(-31.4583397339225,-30.106860032913,46.6654339114981));
#38312=CARTESIAN_POINT('Ctrl Pts',(-33.2966593612321,-30.5180926885401,
46.7765637007177));
#38313=CARTESIAN_POINT('Ctrl Pts',(-33.9482904028273,-32.2855508449996,
46.8876934899375));
#38314=CARTESIAN_POINT('Ctrl Pts',(-32.8168671960847,-33.7916759647855,
46.9988232791572));
#38315=CARTESIAN_POINT('Ctrl Pts',(-30.937855990041,-33.6580786715164,47.1099530683769));
#38316=CARTESIAN_POINT('Ctrl Pts',(-30.0309074634399,-32.0070257591899,
47.2210828575967));
#38317=CARTESIAN_POINT('Ctrl Pts',(-30.926051072379,-30.349542948244,47.3322126468164));
#38318=CARTESIAN_POINT('Ctrl Pts',(-32.8040610933859,-30.2025405326038,
47.4433424360361));
#38319=CARTESIAN_POINT('Ctrl Pts',(-33.9462031214054,-31.7005535288883,
47.5544722252559));
#38320=CARTESIAN_POINT('Ctrl Pts',(-33.3072011584087,-33.4726166881725,
47.6656020144756));
#38321=CARTESIAN_POINT('Ctrl Pts',(-31.4718628712426,-33.8969570243042,
47.7767318036953));
#38322=CARTESIAN_POINT('Ctrl Pts',(-30.1198699569067,-32.585222863435,47.8878615929151));
#38323=CARTESIAN_POINT('Ctrl Pts',(-30.4885516688484,-30.7378990844278,
47.9989913821347));
#38324=CARTESIAN_POINT('Ctrl Pts',(-32.2404945024855,-30.0456363764377,
48.1101211713545));
#38325=CARTESIAN_POINT('Ctrl Pts',(-33.7723393755021,-31.1419860625409,
48.2212509605742));
#38326=CARTESIAN_POINT('Ctrl Pts',(-33.6821584722794,-33.023580799433,48.3323807497939));
#38327=CARTESIAN_POINT('Ctrl Pts',(-32.0524843774755,-33.9684054889555,
48.4435105390136));
#38328=CARTESIAN_POINT('Ctrl Pts',(-30.3747771495755,-33.1117668214546,
48.5546403282334));
#38329=CARTESIAN_POINT('Ctrl Pts',(-30.184456249576,-31.2376512155675,48.6657701174531));
#38330=CARTESIAN_POINT('Ctrl Pts',(-31.6557013012125,-30.0612289498648,
48.7768999066729));
#38331=CARTESIAN_POINT('Ctrl Pts',(-33.4420447882153,-30.6591489241492,
48.8880296958926));
#38332=CARTESIAN_POINT('Ctrl Pts',(-33.9086445233681,-32.4842012621279,
48.9991594851123));
#38333=CARTESIAN_POINT('Ctrl Pts',(-32.6284734891223,-33.8661178559511,
49.1102892743321));
#38334=CARTESIAN_POINT('Ctrl Pts',(-30.773130333143,-33.5401836252133,49.2214190635517));
#38335=CARTESIAN_POINT('Ctrl Pts',(-30.0406049914237,-31.8046900432762,
49.3325488527715));
#38336=CARTESIAN_POINT('Ctrl Pts',(-31.1012967127994,-30.2479420156844,
49.4436786419912));
#38337=CARTESIAN_POINT('Ctrl Pts',(-32.9844719365898,-30.2946584550606,
49.554808431211));
#38338=CARTESIAN_POINT('Ctrl Pts',(-33.9666691201668,-31.9020849827063,
49.6659382204307));
#38339=CARTESIAN_POINT('Ctrl Pts',(-33.1489920526057,-33.5991222723351,
49.7770680096504));
#38340=CARTESIAN_POINT('Ctrl Pts',(-31.2797699187998,-33.8326602000818,
49.8881977988701));
#38341=CARTESIAN_POINT('Ctrl Pts',(-30.0696945447384,-32.3889673870857,
49.9993275880899));
#38342=CARTESIAN_POINT('Ctrl Pts',(-30.6262137900413,-30.5892958396048,
50.1104573773095));
#38343=CARTESIAN_POINT('Ctrl Pts',(-32.4400072766077,-30.0806854412674,
50.2215871665294));
#38344=CARTESIAN_POINT('Ctrl Pts',(-33.8511108753022,-31.3286109129836,
50.3327169557489));
#38345=CARTESIAN_POINT('Ctrl Pts',(-33.5680978753831,-33.1909843962233,
50.4438467449688));
#38346=CARTESIAN_POINT('Ctrl Pts',(-31.849978705224,-33.9633818757322,50.5549765341884));
#38347=CARTESIAN_POINT('Ctrl Pts',(-30.2691573971359,-32.9389135545513,
50.6661063234082));
#38348=CARTESIAN_POINT('Ctrl Pts',(-30.2723844689724,-31.0551617303574,
50.7772361126279));
#38349=CARTESIAN_POINT('Ctrl Pts',(-31.8567065396152,-30.0361156441587,
50.8883659018477));
#38350=CARTESIAN_POINT('Ctrl Pts',(-33.5721692312094,-30.8143952230609,
50.9994956910673));
#38351=CARTESIAN_POINT('Ctrl Pts',(-33.8487996919451,-32.6777274363229,
51.1106254802872));
#38352=CARTESIAN_POINT('Ctrl Pts',(-32.4334287238539,-33.9208108498002,
51.2217552695068));
#38353=CARTESIAN_POINT('Ctrl Pts',(-30.6213884883404,-33.4059890032924,
51.3328850587266));
#38354=CARTESIAN_POINT('Ctrl Pts',(-30.0710385572647,-31.6044212694241,
51.4440148479462));
#38355=CARTESIAN_POINT('Ctrl Pts',(-31.2860532210798,-30.1648828976553,
51.5551446371661));
#38356=CARTESIAN_POINT('Ctrl Pts',(-33.1544642321263,-30.4048238013925,
51.6662744263857));
#38357=CARTESIAN_POINT('Ctrl Pts',(-33.9663221023376,-32.1046526543067,
51.7774042156056));
#38358=CARTESIAN_POINT('Ctrl Pts',(-32.9786232989337,-33.7087045503785,
51.8885340048251));
#38359=CARTESIAN_POINT('Ctrl Pts',(-31.0952990837456,-33.7489685374884,
51.9996637940449));
#38360=CARTESIAN_POINT('Ctrl Pts',(-30.0399472990725,-32.1885955543356,
52.1107935832646));
#38361=CARTESIAN_POINT('Ctrl Pts',(-30.7784145635932,-30.4556218295225,
52.2219233724844));
#38362=CARTESIAN_POINT('Ctrl Pts',(-32.6348634270627,-30.1360465266472,
52.3330531617041));
#38363=CARTESIAN_POINT('Ctrl Pts',(-33.9102924537887,-31.5223406974568,
52.4441829509238));
#38364=CARTESIAN_POINT('Ctrl Pts',(-33.4374419750523,-33.3457845340362,
52.5553127401435));
#38365=CARTESIAN_POINT('Ctrl Pts',(-31.6490613137411,-33.9375788765242,
52.6664425293633));
#38366=CARTESIAN_POINT('Ctrl Pts',(-30.1818537058118,-32.7561261673534,
52.777572318583));
#38367=CARTESIAN_POINT('Ctrl Pts',(-30.3785982775114,-30.8826668248174,
52.8887021078027));
#38368=CARTESIAN_POINT('Ctrl Pts',(-32.0592233947483,-30.0317948524369,
52.9998318970224));
#38369=CARTESIAN_POINT('Ctrl Pts',(-33.6856651825576,-30.9821708820847,
53.1109616862422));
#38370=CARTESIAN_POINT('Ctrl Pts',(-33.7693702652999,-32.864116447248,53.2220914754619));
#38371=CARTESIAN_POINT('Ctrl Pts',(-32.2338346006141,-33.9551065574643,
53.3332212646817));
#38372=CARTESIAN_POINT('Ctrl Pts',(-30.4841619464795,-33.2570527350258,
53.4443510539013));
#38373=CARTESIAN_POINT('Ctrl Pts',(-30.1220333444858,-31.4080660256503,
53.5554808431211));
#38374=CARTESIAN_POINT('Ctrl Pts',(-31.4780737014122,-30.1017857222274,
53.6666106323408));
#38375=CARTESIAN_POINT('Ctrl Pts',(-33.3128174529624,-30.5307878228056,
53.7777404215605));
#38376=CARTESIAN_POINT('Ctrl Pts',(-33.9440063061494,-32.3083920037255,
53.8888702107803));
#38377=CARTESIAN_POINT('Ctrl Pts',(-33.1815065089974,-33.2986349005747,
53.9629567369268));
#38378=CARTESIAN_POINT('Ctrl Pts',(-32.6750771856749,-33.5230977622534,
54.));
#38379=CARTESIAN_POINT('Ctrl Pts',(-30.336158884875,-31.9990545752999,41.6214803633902));
#38380=CARTESIAN_POINT('Ctrl Pts',(-30.3350387011371,-31.7834963203764,
41.6358513744636));
#38381=CARTESIAN_POINT('Ctrl Pts',(-30.3739090865848,-31.5683253856938,
41.650222385537));
#38382=CARTESIAN_POINT('Ctrl Pts',(-30.4546428726593,-31.3702163272604,
41.6645933966103));
#38383=CARTESIAN_POINT('Ctrl Pts',(-30.6627453409677,-30.8595629061987,
41.7016366596836));
#38384=CARTESIAN_POINT('Ctrl Pts',(-31.1489973374487,-30.4622722974605,
41.7386799227568));
#38385=CARTESIAN_POINT('Ctrl Pts',(-31.6908816348332,-30.3601281633497,
41.7757231858301));
#38386=CARTESIAN_POINT('Ctrl Pts',(-32.2327659322177,-30.2579840292389,
41.8127664489033));
#38387=CARTESIAN_POINT('Ctrl Pts',(-32.8302825305056,-30.4509863697556,
41.8498097119765));
#38388=CARTESIAN_POINT('Ctrl Pts',(-33.2100166050692,-30.8508256164995,
41.8868529750498));
#38389=CARTESIAN_POINT('Ctrl Pts',(-33.5897506796328,-31.2506648632435,
41.923896238123));
#38390=CARTESIAN_POINT('Ctrl Pts',(-33.7517022304721,-31.8573410162147,
41.9609395011963));
#38391=CARTESIAN_POINT('Ctrl Pts',(-33.6217603125026,-32.3932386924046,
41.9979827642695));
#38392=CARTESIAN_POINT('Ctrl Pts',(-33.4918183945331,-32.9291363685945,
42.0350260273428));
#38393=CARTESIAN_POINT('Ctrl Pts',(-33.0699830077549,-33.3942555680032,
42.072069290416));
#38394=CARTESIAN_POINT('Ctrl Pts',(-32.5492851488473,-33.5757621181193,
42.1091125534892));
#38395=CARTESIAN_POINT('Ctrl Pts',(-32.0285872899397,-33.7572686682353,
42.1461558165625));
#38396=CARTESIAN_POINT('Ctrl Pts',(-31.4090269589028,-33.6551625690588,
42.1831990796357));
#38397=CARTESIAN_POINT('Ctrl Pts',(-30.9741108911154,-33.3161660829397,
42.220242342709));
#38398=CARTESIAN_POINT('Ctrl Pts',(-30.5779071173622,-33.0073439973986,
42.2539883496027));
#38399=CARTESIAN_POINT('Ctrl Pts',(-30.3349398101202,-32.5019263328413,
42.2877343564965));
#38400=CARTESIAN_POINT('Ctrl Pts',(-30.3317921677919,-31.9991447210974,
42.3214803633902));
#38401=CARTESIAN_POINT('Ctrl Pts',(-31.4698297828114,-33.9851743256717,
41.));
#38402=CARTESIAN_POINT('Ctrl Pts',(-31.4011629206477,-33.9597495324007,
41.));
#38403=CARTESIAN_POINT('Ctrl Pts',(-31.3341994075765,-33.9304353968824,
41.));
#38404=CARTESIAN_POINT('Ctrl Pts',(-31.2691282231929,-33.8975258421853,
41.));
#38405=CARTESIAN_POINT('Ctrl Pts',(-31.2022479171691,-33.8637013296902,
41.));
#38406=CARTESIAN_POINT('Ctrl Pts',(-31.1373658528129,-33.8260780092996,
41.));
#38407=CARTESIAN_POINT('Ctrl Pts',(-31.0747184293343,-33.7849303663298,
41.));
#38408=CARTESIAN_POINT('Ctrl Pts',(-31.0217877705273,-33.7501648208402,
41.));
#38409=CARTESIAN_POINT('Ctrl Pts',(-30.970452648882,-33.7128823799464,41.));
#38410=CARTESIAN_POINT('Ctrl Pts',(-30.9208783808178,-33.6732305849818,
41.));
#38411=CARTESIAN_POINT('Ctrl Pts',(-30.8988476542381,-33.6556093898059,
41.));
#38412=CARTESIAN_POINT('Ctrl Pts',(-30.8771649817797,-33.6375200920571,
41.));
#38413=CARTESIAN_POINT('Ctrl Pts',(-30.8558464259774,-33.6189749164796,
41.));
#38414=CARTESIAN_POINT('Ctrl Pts',(-30.8441323514957,-33.6087847530367,
41.));
#38415=CARTESIAN_POINT('Ctrl Pts',(-30.8325282309531,-33.598456941651,41.));
#38416=CARTESIAN_POINT('Ctrl Pts',(-30.821036863453,-33.5879934687363,41.));
#38417=CARTESIAN_POINT('Ctrl Pts',(-30.8104448788549,-33.5783489295678,
41.));
#38418=CARTESIAN_POINT('Ctrl Pts',(-30.7999472574529,-33.5685876204844,
41.));
#38419=CARTESIAN_POINT('Ctrl Pts',(-30.7895620725801,-33.5587265457271,
41.));
#38420=CARTESIAN_POINT('Ctrl Pts',(-30.7364770283431,-33.508320549481,41.));
#38421=CARTESIAN_POINT('Ctrl Pts',(-30.68623196656,-33.4552262597685,41.));
#38422=CARTESIAN_POINT('Ctrl Pts',(-30.6390455793197,-33.3997030109773,
41.));
#38423=CARTESIAN_POINT('Ctrl Pts',(-30.5922257616164,-33.344611097001,41.));
#38424=CARTESIAN_POINT('Ctrl Pts',(-30.5484167718099,-33.2871269332147,
41.));
#38425=CARTESIAN_POINT('Ctrl Pts',(-30.5078770353379,-33.2274796163432,
41.));
#38426=CARTESIAN_POINT('Ctrl Pts',(-30.4741909267921,-33.1779162455506,
41.));
#38427=CARTESIAN_POINT('Ctrl Pts',(-30.4427627578091,-33.1268586479626,
41.));
#38428=CARTESIAN_POINT('Ctrl Pts',(-30.4137683914513,-33.0744317875342,
41.));
#38429=CARTESIAN_POINT('Ctrl Pts',(-30.4016605159042,-33.0525386413428,
41.));
#38430=CARTESIAN_POINT('Ctrl Pts',(-30.3899773803102,-33.0304066773724,
41.));
#38431=CARTESIAN_POINT('Ctrl Pts',(-30.3787332334151,-33.0080449125542,
41.));
#38432=CARTESIAN_POINT('Ctrl Pts',(-30.3735336402044,-32.9977042365018,
41.));
#38433=CARTESIAN_POINT('Ctrl Pts',(-30.3684279320372,-32.9873144202456,
41.));
#38434=CARTESIAN_POINT('Ctrl Pts',(-30.36341758307,-32.9768763573879,41.));
#38435=CARTESIAN_POINT('Ctrl Pts',(-30.3581837835811,-32.9659727799311,
41.));
#38436=CARTESIAN_POINT('Ctrl Pts',(-30.3530576442939,-32.9550240006742,
41.));
#38437=CARTESIAN_POINT('Ctrl Pts',(-30.3480422353361,-32.9440353490892,
41.));
#38438=CARTESIAN_POINT('Ctrl Pts',(-30.319501876602,-32.8815040458843,41.));
#38439=CARTESIAN_POINT('Ctrl Pts',(-30.2945225097578,-32.8176393566208,
41.));
#38440=CARTESIAN_POINT('Ctrl Pts',(-30.273327611576,-32.7526456143523,41.));
#38441=CARTESIAN_POINT('Ctrl Pts',(-30.2541304481184,-32.6937778866872,
41.));
#38442=CARTESIAN_POINT('Ctrl Pts',(-30.238038284882,-32.6339833166677,41.));
#38443=CARTESIAN_POINT('Ctrl Pts',(-30.2252538389208,-32.5734089087092,
41.));
#38444=CARTESIAN_POINT('Ctrl Pts',(-30.2101196528407,-32.5017011190627,
41.));
#38445=CARTESIAN_POINT('Ctrl Pts',(-30.1996202129508,-32.4288989655352,
41.));
#38446=CARTESIAN_POINT('Ctrl Pts',(-30.1936803700894,-32.3554256399494,
41.));
#38447=CARTESIAN_POINT('Ctrl Pts',(-30.1923734295127,-32.3392593418243,
41.));
#38448=CARTESIAN_POINT('Ctrl Pts',(-30.1912874562889,-32.3230606319689,
41.));
#38449=CARTESIAN_POINT('Ctrl Pts',(-30.1904220188582,-32.3068341825425,
41.));
#38450=CARTESIAN_POINT('Ctrl Pts',(-30.1895243797817,-32.2900039709495,
41.));
#38451=CARTESIAN_POINT('Ctrl Pts',(-30.1888639831893,-32.2731376890812,
41.));
#38452=CARTESIAN_POINT('Ctrl Pts',(-30.1884409105021,-32.2562749512595,
41.));
#38453=CARTESIAN_POINT('Ctrl Pts',(-30.1867207285335,-32.1877123178837,
41.));
#38454=CARTESIAN_POINT('Ctrl Pts',(-30.1889121731841,-32.119121789089,41.));
#38455=CARTESIAN_POINT('Ctrl Pts',(-30.1948946640324,-32.0508418040844,
41.));
#38456=CARTESIAN_POINT('Ctrl Pts',(-30.2008758819965,-31.9825763468949,
41.));
#38457=CARTESIAN_POINT('Ctrl Pts',(-30.2106469868098,-31.9146202295201,
41.));
#38458=CARTESIAN_POINT('Ctrl Pts',(-30.2241370789842,-31.8473267076867,
41.));
#38459=CARTESIAN_POINT('Ctrl Pts',(-30.2338950669342,-31.7986502889733,
41.));
#38460=CARTESIAN_POINT('Ctrl Pts',(-30.2455999819607,-31.7503208244277,
41.));
#38461=CARTESIAN_POINT('Ctrl Pts',(-30.2592391795709,-31.7024816531862,
41.));
#38462=CARTESIAN_POINT('Ctrl Pts',(-30.2694738036972,-31.6665839449658,
41.));
#38463=CARTESIAN_POINT('Ctrl Pts',(-30.2807978226536,-31.6309624632629,
41.));
#38464=CARTESIAN_POINT('Ctrl Pts',(-30.2932098063328,-31.5956819460291,
41.));
#38465=CARTESIAN_POINT('Ctrl Pts',(-30.2973425061779,-31.5839349286404,
41.));
#38466=CARTESIAN_POINT('Ctrl Pts',(-30.3015926355275,-31.572234881057,41.));
#38467=CARTESIAN_POINT('Ctrl Pts',(-30.305959527106,-31.5605844299902,41.));
#38468=CARTESIAN_POINT('Ctrl Pts',(-30.3290832944906,-31.498892419655,41.));
#38469=CARTESIAN_POINT('Ctrl Pts',(-30.3554795854277,-31.4385839314187,
41.));
#38470=CARTESIAN_POINT('Ctrl Pts',(-30.3850984048383,-31.3799931438224,
41.));
#38471=CARTESIAN_POINT('Ctrl Pts',(-30.4059238341125,-31.3387970959215,
41.));
#38472=CARTESIAN_POINT('Ctrl Pts',(-30.4283432407334,-31.2984507577224,
41.));
#38473=CARTESIAN_POINT('Ctrl Pts',(-30.4523496359434,-31.2590816244303,
41.));
#38474=CARTESIAN_POINT('Ctrl Pts',(-30.460063473454,-31.2464313662597,41.));
#38475=CARTESIAN_POINT('Ctrl Pts',(-30.4679423137434,-31.2338804122318,
41.));
#38476=CARTESIAN_POINT('Ctrl Pts',(-30.4759826345042,-31.2214385753381,
41.));
#38477=CARTESIAN_POINT('Ctrl Pts',(-30.5102255955582,-31.1684499758944,
41.));
#38478=CARTESIAN_POINT('Ctrl Pts',(-30.5473242690744,-31.1175452556629,
41.));
#38479=CARTESIAN_POINT('Ctrl Pts',(-30.5872444101701,-31.0690397081128,
41.));
#38480=CARTESIAN_POINT('Ctrl Pts',(-30.6240203632449,-31.0243545519083,
41.));
#38481=CARTESIAN_POINT('Ctrl Pts',(-30.6631914251233,-30.9817054320841,
41.));
#38482=CARTESIAN_POINT('Ctrl Pts',(-30.7047522428173,-30.9413717231824,
41.));
#38483=CARTESIAN_POINT('Ctrl Pts',(-30.7125940811408,-30.9337614199751,
41.));
#38484=CARTESIAN_POINT('Ctrl Pts',(-30.7205210515567,-30.926233652583,41.));
#38485=CARTESIAN_POINT('Ctrl Pts',(-30.7285315473809,-30.9187890928311,
41.));
#38486=CARTESIAN_POINT('Origin',(-32.,-32.,48.));
#38487=CARTESIAN_POINT('Origin',(-32.,32.,54.));
#38488=CARTESIAN_POINT('Ctrl Pts',(-32.6750771856749,30.4769022377466,54.));
#38489=CARTESIAN_POINT('Ctrl Pts',(-32.7347606915771,30.4954885176555,54.));
#38490=CARTESIAN_POINT('Ctrl Pts',(-32.7931316468243,30.5176493824028,54.));
#38491=CARTESIAN_POINT('Ctrl Pts',(-32.8500334991629,30.5430859583899,54.));
#38492=CARTESIAN_POINT('Ctrl Pts',(-32.8861162422491,30.5592158627536,54.));
#38493=CARTESIAN_POINT('Ctrl Pts',(-32.9216082931908,30.5766640695137,54.));
#38494=CARTESIAN_POINT('Ctrl Pts',(-32.9564688344476,30.5953648077861,54.));
#38495=CARTESIAN_POINT('Ctrl Pts',(-32.9802311105381,30.6081119450911,54.));
#38496=CARTESIAN_POINT('Ctrl Pts',(-33.0036999498365,30.6214412122672,54.));
#38497=CARTESIAN_POINT('Ctrl Pts',(-33.0268619608851,30.6353337365551,54.));
#38498=CARTESIAN_POINT('Ctrl Pts',(-33.0392110030252,30.6427406654053,54.));
#38499=CARTESIAN_POINT('Ctrl Pts',(-33.0514726639847,30.650307779206,54.));
#38500=CARTESIAN_POINT('Ctrl Pts',(-33.0636328281387,30.6580243195221,54.));
#38501=CARTESIAN_POINT('Ctrl Pts',(-33.1193346579069,30.6933713271479,54.));
#38502=CARTESIAN_POINT('Ctrl Pts',(-33.1729727156271,30.7318877508992,54.));
#38503=CARTESIAN_POINT('Ctrl Pts',(-33.2243651773974,30.7732711116722,54.));
#38504=CARTESIAN_POINT('Ctrl Pts',(-33.2614339884367,30.8031204694929,54.));
#38505=CARTESIAN_POINT('Ctrl Pts',(-33.2973344258717,30.8344625918461,54.));
#38506=CARTESIAN_POINT('Ctrl Pts',(-33.3319929726109,30.8671998395399,54.));
#38507=CARTESIAN_POINT('Ctrl Pts',(-33.3414619332501,30.8761438876612,54.));
#38508=CARTESIAN_POINT('Ctrl Pts',(-33.3508381622407,30.8851921406493,54.));
#38509=CARTESIAN_POINT('Ctrl Pts',(-33.360120076321,30.89434275958,54.));
#38510=CARTESIAN_POINT('Ctrl Pts',(-33.3696838750555,30.9037712758313,54.));
#38511=CARTESIAN_POINT('Ctrl Pts',(-33.3791418362518,30.9133029001982,54.));
#38512=CARTESIAN_POINT('Ctrl Pts',(-33.3884887348017,30.9229312087312,54.));
#38513=CARTESIAN_POINT('Ctrl Pts',(-33.435751083172,30.9716164993304,54.));
#38514=CARTESIAN_POINT('Ctrl Pts',(-33.4802065476745,31.0228007164435,54.));
#38515=CARTESIAN_POINT('Ctrl Pts',(-33.5216714229955,31.0761767682427,54.));
#38516=CARTESIAN_POINT('Ctrl Pts',(-33.5637355354488,31.1303241936916,54.));
#38517=CARTESIAN_POINT('Ctrl Pts',(-33.6027228866653,31.1867278444332,54.));
#38518=CARTESIAN_POINT('Ctrl Pts',(-33.6384173336076,31.2451140319467,54.));
#38519=CARTESIAN_POINT('Ctrl Pts',(-33.6605280372079,31.2812809933946,54.));
#38520=CARTESIAN_POINT('Ctrl Pts',(-33.6813746887815,31.3182095673848,54.));
#38521=CARTESIAN_POINT('Ctrl Pts',(-33.7008990002285,31.3558419756537,54.));
#38522=CARTESIAN_POINT('Ctrl Pts',(-33.7168832701209,31.3866510811169,54.));
#38523=CARTESIAN_POINT('Ctrl Pts',(-33.7319811659046,31.4179320443681,54.));
#38524=CARTESIAN_POINT('Ctrl Pts',(-33.7461573794449,31.4496553736956,54.));
#38525=CARTESIAN_POINT('Ctrl Pts',(-33.7519693974655,31.462661425079,54.));
#38526=CARTESIAN_POINT('Ctrl Pts',(-33.7576273458872,31.4757443280942,54.));
#38527=CARTESIAN_POINT('Ctrl Pts',(-33.7631196222834,31.4888795631979,54.));
#38528=CARTESIAN_POINT('Ctrl Pts',(-33.7903102098283,31.5539081113344,54.));
#38529=CARTESIAN_POINT('Ctrl Pts',(-33.8134950874387,31.6203284923708,54.));
#38530=CARTESIAN_POINT('Ctrl Pts',(-33.8324626822549,31.6878455732216,54.));
#38531=CARTESIAN_POINT('Ctrl Pts',(-33.8345627116769,31.6953208413115,54.));
#38532=CARTESIAN_POINT('Ctrl Pts',(-33.836611009148,31.7028095915747,54.));
#38533=CARTESIAN_POINT('Ctrl Pts',(-33.8386072594899,31.710311451093,54.));
#38534=CARTESIAN_POINT('Ctrl Pts',(-33.855945393719,31.7754677316278,54.));
#38535=CARTESIAN_POINT('Ctrl Pts',(-33.8693612283885,31.8416108585899,54.));
#38536=CARTESIAN_POINT('Ctrl Pts',(-33.8790088087618,31.9084363750645,54.));
#38537=CARTESIAN_POINT('Ctrl Pts',(-33.8893872742774,31.9803244849798,54.));
#38538=CARTESIAN_POINT('Ctrl Pts',(-33.8954055239578,32.0530030863577,54.));
#38539=CARTESIAN_POINT('Ctrl Pts',(-33.8971951879124,32.1261156983931,54.));
#38540=CARTESIAN_POINT('Ctrl Pts',(-33.8975152604702,32.1391915278981,54.));
#38541=CARTESIAN_POINT('Ctrl Pts',(-33.8976999206002,32.1522812739254,54.));
#38542=CARTESIAN_POINT('Ctrl Pts',(-33.897749714621,32.1653829318895,54.));
#38543=CARTESIAN_POINT('Ctrl Pts',(-33.8977946808874,32.177214325139,54.));
#38544=CARTESIAN_POINT('Ctrl Pts',(-33.8977296105587,32.1890468266652,54.));
#38545=CARTESIAN_POINT('Ctrl Pts',(-33.8975554553278,32.2008754645531,54.));
#38546=CARTESIAN_POINT('Ctrl Pts',(-33.8965092280538,32.2719353087169,54.));
#38547=CARTESIAN_POINT('Ctrl Pts',(-33.8915304228521,32.3428930409877,54.));
#38548=CARTESIAN_POINT('Ctrl Pts',(-33.8827991703013,32.4134130591355,54.));
#38549=CARTESIAN_POINT('Ctrl Pts',(-33.8738836831824,32.4854210911754,54.));
#38550=CARTESIAN_POINT('Ctrl Pts',(-33.8610557741427,32.5569736774994,54.));
#38551=CARTESIAN_POINT('Ctrl Pts',(-33.8444545204575,32.6277297102758,54.));
#38552=CARTESIAN_POINT('Ctrl Pts',(-33.8277523485976,32.6989158653678,54.));
#38553=CARTESIAN_POINT('Ctrl Pts',(-33.8072307379804,32.7692968235389,54.));
#38554=CARTESIAN_POINT('Ctrl Pts',(-33.7829789156768,32.8385261464761,54.));
#38555=CARTESIAN_POINT('Ctrl Pts',(-33.7769979005134,32.8555995698689,54.));
#38556=CARTESIAN_POINT('Ctrl Pts',(-33.7707897613597,32.8726029088931,54.));
#38557=CARTESIAN_POINT('Ctrl Pts',(-33.7643553594181,32.8895308570373,54.));
#38558=CARTESIAN_POINT('Ctrl Pts',(-33.7592863747482,32.9028665967708,54.));
#38559=CARTESIAN_POINT('Ctrl Pts',(-33.7540761916856,32.9161571498072,54.));
#38560=CARTESIAN_POINT('Ctrl Pts',(-33.7487336714912,32.9293797191499,54.));
#38561=CARTESIAN_POINT('Ctrl Pts',(-33.7205084932337,32.9992361470419,54.));
#38562=CARTESIAN_POINT('Ctrl Pts',(-33.6885470824167,33.0673216292728,54.));
#38563=CARTESIAN_POINT('Ctrl Pts',(-33.6530075460646,33.1332788252052,54.));
#38564=CARTESIAN_POINT('Ctrl Pts',(-33.6174290020438,33.1993084147791,54.));
#38565=CARTESIAN_POINT('Ctrl Pts',(-33.5782643022281,33.2632061589058,54.));
#38566=CARTESIAN_POINT('Ctrl Pts',(-33.5356203080281,33.3246091157058,54.));
#38567=CARTESIAN_POINT('Ctrl Pts',(-33.4939464336363,33.3846151999615,54.));
#38568=CARTESIAN_POINT('Ctrl Pts',(-33.4489494285267,33.4422396978105,54.));
#38569=CARTESIAN_POINT('Ctrl Pts',(-33.4006836910636,33.497124259357,54.));
#38570=CARTESIAN_POINT('Ctrl Pts',(-33.3903484920103,33.5088767549854,54.));
#38571=CARTESIAN_POINT('Ctrl Pts',(-33.3798632561248,33.5205035150137,54.));
#38572=CARTESIAN_POINT('Ctrl Pts',(-33.3692282611413,33.532000833948,54.));
#38573=CARTESIAN_POINT('Ctrl Pts',(-33.360117214453,33.5418506373343,54.));
#38574=CARTESIAN_POINT('Ctrl Pts',(-33.3508962513759,33.5516054369775,54.));
#38575=CARTESIAN_POINT('Ctrl Pts',(-33.3415672325379,33.5612648174638,54.));
#38576=CARTESIAN_POINT('Ctrl Pts',(-32.3836679988468,34.0186125009919,54.));
#38577=CARTESIAN_POINT('Ctrl Pts',(-32.3093502844899,34.0256330949372,54.));
#38578=CARTESIAN_POINT('Ctrl Pts',(-32.2347844706668,34.0282517480001,54.));
#38579=CARTESIAN_POINT('Ctrl Pts',(-32.1602926743779,34.0266320545354,54.));
#38580=CARTESIAN_POINT('Ctrl Pts',(-32.0877589864994,34.025054936704,54.));
#38581=CARTESIAN_POINT('Ctrl Pts',(-32.0152946934488,34.0194587142989,54.));
#38582=CARTESIAN_POINT('Ctrl Pts',(-31.9432103734882,34.0099505607399,54.));
#38583=CARTESIAN_POINT('Ctrl Pts',(-31.9271201946013,34.0078282144137,54.));
#38584=CARTESIAN_POINT('Ctrl Pts',(-31.9110468943986,34.0055104663305,54.));
#38585=CARTESIAN_POINT('Ctrl Pts',(-31.8950008955345,34.0029993250679,54.));
#38586=CARTESIAN_POINT('Ctrl Pts',(-31.821367329252,33.9914759360805,54.));
#38587=CARTESIAN_POINT('Ctrl Pts',(-31.7484534135904,33.9759080373483,54.));
#38588=CARTESIAN_POINT('Ctrl Pts',(-31.6765910812025,33.9564351190568,54.));
#38589=CARTESIAN_POINT('Ctrl Pts',(-31.6261438367467,33.942765161004,54.));
#38590=CARTESIAN_POINT('Ctrl Pts',(-31.5762150883091,33.9271697110659,54.));
#38591=CARTESIAN_POINT('Ctrl Pts',(-31.526927605364,33.9096838836821,54.));
#38592=CARTESIAN_POINT('Ctrl Pts',(-31.5082001959596,33.9030399199691,54.));
#38593=CARTESIAN_POINT('Ctrl Pts',(-31.4895654503424,33.8961229364477,54.));
#38594=CARTESIAN_POINT('Ctrl Pts',(-31.4710304367965,33.8889344969223,54.));
#38595=CARTESIAN_POINT('Ctrl Pts',(-31.4533429023197,33.882074735443,54.));
#38596=CARTESIAN_POINT('Ctrl Pts',(-31.4357407268156,33.8749653206272,54.));
#38597=CARTESIAN_POINT('Ctrl Pts',(-31.4182609664101,33.8676208388457,54.));
#38598=CARTESIAN_POINT('Ctrl Pts',(-31.3513338147382,33.8395000159774,54.));
#38599=CARTESIAN_POINT('Ctrl Pts',(-31.2861267881216,33.8079111496751,54.));
#38600=CARTESIAN_POINT('Ctrl Pts',(-31.2229480924711,33.7729813893192,54.));
#38601=CARTESIAN_POINT('Ctrl Pts',(-31.1611264019049,33.7388018796912,54.));
#38602=CARTESIAN_POINT('Ctrl Pts',(-31.1012461490794,33.7014228251959,54.));
#38603=CARTESIAN_POINT('Ctrl Pts',(-31.043628468054,33.6609265400657,54.));
#38604=CARTESIAN_POINT('Ctrl Pts',(-30.987274236897,33.6213182640535,54.));
#38605=CARTESIAN_POINT('Ctrl Pts',(-30.9330838755882,33.5787274426741,54.));
#38606=CARTESIAN_POINT('Ctrl Pts',(-30.8813982876013,33.5332038702195,54.));
#38607=CARTESIAN_POINT('Ctrl Pts',(-30.8645714462744,33.5183831443622,54.));
#38608=CARTESIAN_POINT('Ctrl Pts',(-30.8480104467711,33.5032513889838,54.));
#38609=CARTESIAN_POINT('Ctrl Pts',(-30.8317281562672,33.4878098190582,54.));
#38610=CARTESIAN_POINT('Ctrl Pts',(-30.8225975555259,33.4791506681987,54.));
#38611=CARTESIAN_POINT('Ctrl Pts',(-30.8135537775277,33.4703931298114,54.));
#38612=CARTESIAN_POINT('Ctrl Pts',(-30.8046115462315,33.4615500351139,54.));
#38613=CARTESIAN_POINT('Ctrl Pts',(-30.7560461054599,33.4135230072332,54.));
#38614=CARTESIAN_POINT('Ctrl Pts',(-30.7103849708301,33.3628934275024,54.));
#38615=CARTESIAN_POINT('Ctrl Pts',(-30.667920505939,33.3097422848648,54.));
#38616=CARTESIAN_POINT('Ctrl Pts',(-30.6618145678856,33.3020997163021,54.));
#38617=CARTESIAN_POINT('Ctrl Pts',(-30.6557747947556,33.2944049635008,54.));
#38618=CARTESIAN_POINT('Ctrl Pts',(-30.6498021315748,33.2866582187114,54.));
#38619=CARTESIAN_POINT('Ctrl Pts',(-30.6074436612194,33.2317178596821,54.));
#38620=CARTESIAN_POINT('Ctrl Pts',(-30.5684565753518,33.1741638225229,54.));
#38621=CARTESIAN_POINT('Ctrl Pts',(-30.5329081125672,33.1143583196404,54.));
#38622=CARTESIAN_POINT('Ctrl Pts',(-30.4997462774684,33.0585679965369,54.));
#38623=CARTESIAN_POINT('Ctrl Pts',(-30.4695772466851,33.0008173969119,54.));
#38624=CARTESIAN_POINT('Ctrl Pts',(-30.4424953173611,32.9413951242111,54.));
#38625=CARTESIAN_POINT('Ctrl Pts',(-30.4366015041344,32.92846311436,54.));
#38626=CARTESIAN_POINT('Ctrl Pts',(-30.4308540497917,32.9154519378522,54.));
#38627=CARTESIAN_POINT('Ctrl Pts',(-30.4252541718586,32.9023645968498,54.));
#38628=CARTESIAN_POINT('Ctrl Pts',(-30.4207268719756,32.8917839523971,54.));
#38629=CARTESIAN_POINT('Ctrl Pts',(-30.4162962542086,32.8811538243346,54.));
#38630=CARTESIAN_POINT('Ctrl Pts',(-30.4119679861992,32.8704888342707,54.));
#38631=CARTESIAN_POINT('Ctrl Pts',(-30.3862552098172,32.8071317353044,54.));
#38632=CARTESIAN_POINT('Ctrl Pts',(-30.3640997288972,32.7424289154671,54.));
#38633=CARTESIAN_POINT('Ctrl Pts',(-30.3455478113908,32.6767304436005,54.));
#38634=CARTESIAN_POINT('Ctrl Pts',(-30.3270815332802,32.6113352491414,54.));
#38635=CARTESIAN_POINT('Ctrl Pts',(-30.3121856182907,32.5449524378339,54.));
#38636=CARTESIAN_POINT('Ctrl Pts',(-30.3009567584366,32.4779246219716,54.));
#38637=CARTESIAN_POINT('Ctrl Pts',(-30.2899684808235,32.412332900455,54.));
#38638=CARTESIAN_POINT('Ctrl Pts',(-30.2824919357175,32.3461225531827,54.));
#38639=CARTESIAN_POINT('Ctrl Pts',(-30.2786656210298,32.279627521379,54.));
#38640=CARTESIAN_POINT('Ctrl Pts',(-30.2775523223255,32.2602802280194,54.));
#38641=CARTESIAN_POINT('Ctrl Pts',(-30.276748348819,32.2409089692141,54.));
#38642=CARTESIAN_POINT('Ctrl Pts',(-30.2762578731991,32.2215223570683,54.));
#38643=CARTESIAN_POINT('Ctrl Pts',(-30.2759857301979,32.2107655924154,54.));
#38644=CARTESIAN_POINT('Ctrl Pts',(-30.2758103549668,32.2000138517791,54.));
#38645=CARTESIAN_POINT('Ctrl Pts',(-30.2757319784298,32.189268592358,54.));
#38646=CARTESIAN_POINT('Ctrl Pts',(-30.2752558367538,32.1239905637135,54.));
#38647=CARTESIAN_POINT('Ctrl Pts',(-30.2783554890008,32.058949723192,54.));
#38648=CARTESIAN_POINT('Ctrl Pts',(-30.2851111704578,31.9944559018851,54.));
#38649=CARTESIAN_POINT('Ctrl Pts',(-30.292024200112,31.9284599395171,54.));
#38650=CARTESIAN_POINT('Ctrl Pts',(-30.3027653489992,31.8630356306402,54.));
#38651=CARTESIAN_POINT('Ctrl Pts',(-30.3174745268228,31.7985356931485,54.));
#38652=CARTESIAN_POINT('Ctrl Pts',(-30.3311068214881,31.7387579024165,54.));
#38653=CARTESIAN_POINT('Ctrl Pts',(-30.3481479575203,31.679773639241,54.));
#38654=CARTESIAN_POINT('Ctrl Pts',(-30.3687510878919,31.6218918797604,54.));
#38655=CARTESIAN_POINT('Ctrl Pts',(-30.3703786322379,31.6173195099952,54.));
#38656=CARTESIAN_POINT('Ctrl Pts',(-30.372028424917,31.612754037598,54.));
#38657=CARTESIAN_POINT('Ctrl Pts',(-30.373700552093,31.6081956242523,54.));
#38658=CARTESIAN_POINT('Ctrl Pts',(-30.3774632060968,31.597938191401,54.));
#38659=CARTESIAN_POINT('Ctrl Pts',(-30.3813389495473,31.5877164997064,54.));
#38660=CARTESIAN_POINT('Ctrl Pts',(-30.3853267261146,31.5775319120267,54.));
#38661=CARTESIAN_POINT('Origin',(-32.,32.,39.4540747194623));
#38662=CARTESIAN_POINT('Ctrl Pts',(-29.9434322456991,32.0014925908821,41.2040747194623));
#38663=CARTESIAN_POINT('Ctrl Pts',(-29.9426158532448,32.09958269322,41.2094078928853));
#38664=CARTESIAN_POINT('Ctrl Pts',(-29.9935881745736,32.8781627954851,41.2517843293816));
#38665=CARTESIAN_POINT('Ctrl Pts',(-30.9882785960482,34.2080088094421,41.3312040289512));
#38666=CARTESIAN_POINT('Ctrl Pts',(-33.3060692860357,34.0473904772534,41.4423338181709));
#38667=CARTESIAN_POINT('Ctrl Pts',(-34.4285436298619,32.0133707862788,41.5534636073906));
#38668=CARTESIAN_POINT('Ctrl Pts',(-33.3284492137394,29.9669383950752,41.6645933966104));
#38669=CARTESIAN_POINT('Ctrl Pts',(-31.0125684250491,29.7812307990702,41.7757231858301));
#38670=CARTESIAN_POINT('Ctrl Pts',(-29.9981580758837,31.1064229367225,41.8555502934474));
#38671=CARTESIAN_POINT('Ctrl Pts',(-29.9427300285746,31.8927563400753,41.8983341379915));
#38672=CARTESIAN_POINT('Ctrl Pts',(-29.9436380261218,31.9983919808556,41.9040747194623));
#38673=CARTESIAN_POINT('Ctrl Pts',(-29.9473238061977,31.9976393779993,41.1459252805377));
#38674=CARTESIAN_POINT('Ctrl Pts',(-29.9508741641786,32.4677619363521,41.1713700465049));
#38675=CARTESIAN_POINT('Ctrl Pts',(-30.3433201135815,33.6293341735692,41.2338580755455));
#38676=CARTESIAN_POINT('Ctrl Pts',(-32.2715961695763,34.4127962262488,41.3333893676592));
#38677=CARTESIAN_POINT('Ctrl Pts',(-34.1743722121293,33.0815585185448,41.4445191568789));
#38678=CARTESIAN_POINT('Ctrl Pts',(-34.088014018114,30.7594030715832,41.5556489460986));
#38679=CARTESIAN_POINT('Ctrl Pts',(-32.0903101568642,29.5731769531958,41.6667787353184));
#38680=CARTESIAN_POINT('Ctrl Pts',(-30.2791651722886,30.473897298874,41.7635375134647));
#38681=CARTESIAN_POINT('Ctrl Pts',(-29.9500923049499,31.5817394200461,41.8232530285378));
#38682=CARTESIAN_POINT('Ctrl Pts',(-29.9479126851747,32.0011660315207,41.8459252805377));
#38683=CARTESIAN_POINT('Ctrl Pts',(-33.2690708798524,33.0793586530485,41.));
#38684=CARTESIAN_POINT('Ctrl Pts',(-33.6279571482407,32.6573931542737,41.0370432630732));
#38685=CARTESIAN_POINT('Ctrl Pts',(-33.8852969018116,31.4343804031744,41.1111297892197));
#38686=CARTESIAN_POINT('Ctrl Pts',(-32.545339605534,30.1066748127004,41.2222595784395));
#38687=CARTESIAN_POINT('Ctrl Pts',(-30.7061568094468,30.5162239665622,41.3333893676592));
#38688=CARTESIAN_POINT('Ctrl Pts',(-30.0511799680217,32.2815047919735,41.4445191568789));
#38689=CARTESIAN_POINT('Ctrl Pts',(-31.1796920019547,33.7902628916075,41.5556489460986));
#38690=CARTESIAN_POINT('Ctrl Pts',(-33.0589665071349,33.6600328677963,41.6667787353184));
#38691=CARTESIAN_POINT('Ctrl Pts',(-33.9690734577686,32.010841090128,41.7779085245381));
#38692=CARTESIAN_POINT('Ctrl Pts',(-33.0771122472757,30.3515850425576,41.8890383137579));
#38693=CARTESIAN_POINT('Ctrl Pts',(-31.199386298154,30.2010125374138,42.0001681029776));
#38694=CARTESIAN_POINT('Ctrl Pts',(-30.0543749890887,31.6968174506273,42.1112978921972));
#38695=CARTESIAN_POINT('Ctrl Pts',(-30.6899777507586,33.4701101328659,42.222427681417));
#38696=CARTESIAN_POINT('Ctrl Pts',(-32.5244990925998,33.8979646750396,42.3335574706367));
#38697=CARTESIAN_POINT('Ctrl Pts',(-33.8790043385183,32.5888272218981,42.4446872598564));
#38698=CARTESIAN_POINT('Ctrl Pts',(-33.5138652990546,30.7407991101668,42.5558170490762));
#38699=CARTESIAN_POINT('Ctrl Pts',(-31.7632531003825,30.0451791949681,42.6669468382959));
#38700=CARTESIAN_POINT('Ctrl Pts',(-30.2293091244602,31.1385894763683,42.7780766275156));
#38701=CARTESIAN_POINT('Ctrl Pts',(-30.3158822215292,33.0203536330321,42.8892064167354));
#38702=CARTESIAN_POINT('Ctrl Pts',(-31.9437416530102,33.9683010556135,43.000336205955));
#38703=CARTESIAN_POINT('Ctrl Pts',(-33.6230881099971,33.1148807754365,43.1114659951748));
#38704=CARTESIAN_POINT('Ctrl Pts',(-33.8170019321722,31.2411336605529,43.2225957843945));
#38705=CARTESIAN_POINT('Ctrl Pts',(-32.3480152896794,30.0618928098755,43.3337255736143));
#38706=CARTESIAN_POINT('Ctrl Pts',(-30.5605288286001,30.6563866316462,43.444855362834));
#38707=CARTESIAN_POINT('Ctrl Pts',(-30.090430772939,32.4805408423343,43.5559851520537));
#38708=CARTESIAN_POINT('Ctrl Pts',(-31.3679497655855,33.8649092828001,43.6671149412734));
#38709=CARTESIAN_POINT('Ctrl Pts',(-33.2239142784095,33.5425329730427,43.7782447304932));
#38710=CARTESIAN_POINT('Ctrl Pts',(-33.9597657164607,31.8084472137752,43.8893745197128));
#38711=CARTESIAN_POINT('Ctrl Pts',(-32.9020608235662,30.2496684874881,44.0005043089327));
#38712=CARTESIAN_POINT('Ctrl Pts',(-31.0187996473937,30.2927741797298,44.1116340981524));
#38713=CARTESIAN_POINT('Ctrl Pts',(-30.0335223932481,31.8983144286743,44.2227638873721));
#38714=CARTESIAN_POINT('Ctrl Pts',(-30.8479441192419,33.5969162097192,44.3338936765918));
#38715=CARTESIAN_POINT('Ctrl Pts',(-32.7167148937789,33.834037593486,44.4450234658115));
#38716=CARTESIAN_POINT('Ctrl Pts',(-33.9295559699792,32.3926676609928,44.5561532550313));
#38717=CARTESIAN_POINT('Ctrl Pts',(-33.3764883476175,30.5919325434682,44.667283044251));
#38718=CARTESIAN_POINT('Ctrl Pts',(-31.5636735169108,30.0798454923028,44.7784128334707));
#38719=CARTESIAN_POINT('Ctrl Pts',(-30.1501799517637,31.3250630233749,44.8895426226905));
#38720=CARTESIAN_POINT('Ctrl Pts',(-30.4296216342993,33.1879755560667,45.0006724119101));
#38721=CARTESIAN_POINT('Ctrl Pts',(-32.14625656708,33.9636657429052,45.11180220113));
#38722=CARTESIAN_POINT('Ctrl Pts',(-33.7290390757554,32.9422303369048,45.2229319903495));
#38723=CARTESIAN_POINT('Ctrl Pts',(-33.7294237729475,31.0584759446318,45.3340617795694));
#38724=CARTESIAN_POINT('Ctrl Pts',(-32.1470585879579,30.0363941574285,45.4451915687891));
#38725=CARTESIAN_POINT('Ctrl Pts',(-30.4301069780531,30.811383142928,45.5563213580087));
#38726=CARTESIAN_POINT('Ctrl Pts',(-30.1499044370533,32.6741813860068,45.6674511472285));
#38727=CARTESIAN_POINT('Ctrl Pts',(-31.5628892918113,33.9199761358048,45.7785809364482));
#38728=CARTESIAN_POINT('Ctrl Pts',(-33.3759131264354,33.4086295473885,45.889710725668));
#38729=CARTESIAN_POINT('Ctrl Pts',(-33.9297161889023,31.6081204731536,46.0008405148877));
#38730=CARTESIAN_POINT('Ctrl Pts',(-32.7174639221865,30.166255292132,46.1119703041075));
#38731=CARTESIAN_POINT('Ctrl Pts',(-30.8485964544578,30.402613381618,46.2231000933272));
#38732=CARTESIAN_POINT('Ctrl Pts',(-30.0334810251578,32.1008823813106,46.3342298825468));
#38733=CARTESIAN_POINT('Ctrl Pts',(-31.0181024356232,33.7068249196517,46.4453596717667));
#38734=CARTESIAN_POINT('Ctrl Pts',(-32.9013458487704,33.750699801273,46.5564894609863));
#38735=CARTESIAN_POINT('Ctrl Pts',(-33.9596873158118,32.192353210318,46.6676192502061));
#38736=CARTESIAN_POINT('Ctrl Pts',(-33.2245442033461,30.4579670472637,46.7787490394257));
#38737=CARTESIAN_POINT('Ctrl Pts',(-31.3687115156069,30.1348327199026,46.8898788286456));
#38738=CARTESIAN_POINT('Ctrl Pts',(-30.0906272027459,31.5186792603898,47.0010086178652));
#38739=CARTESIAN_POINT('Ctrl Pts',(-30.5599801676459,33.3430253220621,47.112138407085));
#38740=CARTESIAN_POINT('Ctrl Pts',(-32.3472236667517,33.9382491734864,47.2232681963047));
#38741=CARTESIAN_POINT('Ctrl Pts',(-33.8166918315301,32.7596084007729,47.3343979855245));
#38742=CARTESIAN_POINT('Ctrl Pts',(-33.6235433332948,30.8857822572822,47.4455277747441));
#38743=CARTESIAN_POINT('Ctrl Pts',(-31.9445455830223,30.0316761087385,47.5566575639639));
#38744=CARTESIAN_POINT('Ctrl Pts',(-30.3162991137898,30.9789586398936,47.6677873531836));
#38745=CARTESIAN_POINT('Ctrl Pts',(-30.228957436641,32.8606871510856,47.7789171424033));
#38746=CARTESIAN_POINT('Ctrl Pts',(-31.7624547073216,33.9547241153676,47.890046931623));
#38747=CARTESIAN_POINT('Ctrl Pts',(-33.51335085379,33.2598187673654,48.0011767208428));
#38748=CARTESIAN_POINT('Ctrl Pts',(-33.8792447104765,31.4119409456361,48.1123065100625));
#38749=CARTESIAN_POINT('Ctrl Pts',(-32.5252741876951,30.1022483932257,48.2234362992823));
#38750=CARTESIAN_POINT('Ctrl Pts',(-30.6905784246966,30.529357531076,48.3345660885019));
#38751=CARTESIAN_POINT('Ctrl Pts',(-30.05425108733,32.302382708032,48.4456958777217));
#38752=CARTESIAN_POINT('Ctrl Pts',(-31.1986520540708,33.7986705098011,48.5568256669414));
#38753=CARTESIAN_POINT('Ctrl Pts',(-33.0764379706693,33.6488345667696,48.6679554561611));
#38754=CARTESIAN_POINT('Ctrl Pts',(-33.969079529995,31.9900031090969,48.7790852453809));
#38755=CARTESIAN_POINT('Ctrl Pts',(-33.0596408572476,30.3403206975669,48.8902150346006));
#38756=CARTESIAN_POINT('Ctrl Pts',(-31.1804303632738,30.2095587851511,49.0013448238203));
#38757=CARTESIAN_POINT('Ctrl Pts',(-30.0512811129692,31.7173892560386,49.1124746130401));
#38758=CARTESIAN_POINT('Ctrl Pts',(-30.7055782550989,33.4838620150136,49.2236044022597));
#38759=CARTESIAN_POINT('Ctrl Pts',(-32.5445161407428,33.8923203496617,49.3347341914795));
#38760=CARTESIAN_POINT('Ctrl Pts',(-33.8851187594106,32.568947621659,49.4458639806992));
#38761=CARTESIAN_POINT('Ctrl Pts',(-33.5004811327274,30.7248802002941,49.556993769919));
#38762=CARTESIAN_POINT('Ctrl Pts',(-31.7426194454125,30.0477885915216,49.6681235591387));
#38763=CARTESIAN_POINT('Ctrl Pts',(-30.2203096504801,31.1573396929374,49.7792533483584));
#38764=CARTESIAN_POINT('Ctrl Pts',(-30.3267531634902,33.0380843691064,49.8903831375782));
#38765=CARTESIAN_POINT('Ctrl Pts',(-31.9645340356676,33.9687854882254,50.0015129267979));
#38766=CARTESIAN_POINT('Ctrl Pts',(-33.6347729737898,33.0976754791102,50.1126427160176));
#38767=CARTESIAN_POINT('Ctrl Pts',(-33.808885414674,31.2219847753081,50.2237725052373));
#38768=CARTESIAN_POINT('Ctrl Pts',(-32.3275255405944,30.0583251679204,50.334902294457));
#38769=CARTESIAN_POINT('Ctrl Pts',(-30.5464178436287,30.6716653102649,50.4460320836768));
#38770=CARTESIAN_POINT('Ctrl Pts',(-30.0956127727332,32.5006829554657,50.5571618728965));
#38771=CARTESIAN_POINT('Ctrl Pts',(-31.3876822400103,33.8714809895036,50.6682916621163));
#38772=CARTESIAN_POINT('Ctrl Pts',(-33.2401382809253,33.5295199173165,50.7794214513359));
#38773=CARTESIAN_POINT('Ctrl Pts',(-33.9576332158673,31.7877588037492,50.8905512405557));
#38774=CARTESIAN_POINT('Ctrl Pts',(-32.8835234613151,30.2402385313405,51.0016810297754));
#38775=CARTESIAN_POINT('Ctrl Pts',(-31.0008226163421,30.3032328712111,51.1128108189951));
#38776=CARTESIAN_POINT('Ctrl Pts',(-30.0325580773407,31.9190900867144,51.2239406082148));
#38777=CARTESIAN_POINT('Ctrl Pts',(-30.8648750497888,33.6089951773492,51.3350703974346));
#38778=CARTESIAN_POINT('Ctrl Pts',(-32.7360460670478,33.8263653306506,51.4462001866543));
#38779=CARTESIAN_POINT('Ctrl Pts',(-33.9335957052477,32.37226573915,51.557329975874));
#38780=CARTESIAN_POINT('Ctrl Pts',(-33.3615395241336,30.5774725808226,51.6684597650938));
#38781=CARTESIAN_POINT('Ctrl Pts',(-31.5434171335246,30.0845610886922,51.7795895543134));
#38782=CARTESIAN_POINT('Ctrl Pts',(-30.1431544354102,31.3446385184301,51.8907193435332));
#38783=CARTESIAN_POINT('Ctrl Pts',(-30.4422566523871,33.2044956644301,52.0018491327529));
#38784=CARTESIAN_POINT('Ctrl Pts',(-32.1669887058313,33.9620114496039,52.1129789219727));
#38785=CARTESIAN_POINT('Ctrl Pts',(-33.7388944714699,32.9239156153169,52.2241087111924));
#38786=CARTESIAN_POINT('Ctrl Pts',(-33.7193829439153,31.040262264795,52.3352385004122));
#38787=CARTESIAN_POINT('Ctrl Pts',(-32.1263106543069,30.0349504114267,52.4463682896318));
#38788=CARTESIAN_POINT('Ctrl Pts',(-30.4176404962616,30.8280307703727,52.5574980788516));
#38789=CARTESIAN_POINT('Ctrl Pts',(-30.1571280564506,32.693684383792,52.6686278680713));
#38790=CARTESIAN_POINT('Ctrl Pts',(-31.5831931024171,33.9244861162258,52.7797576572911));
#38791=CARTESIAN_POINT('Ctrl Pts',(-33.3907131865728,33.3940179477067,52.8908874465107));
#38792=CARTESIAN_POINT('Ctrl Pts',(-33.9254718294467,31.587761803966,53.0020172357305));
#38793=CARTESIAN_POINT('Ctrl Pts',(-32.6980512499253,30.1587773644109,53.1131470249502));
#38794=CARTESIAN_POINT('Ctrl Pts',(-30.8317981364649,30.4148682716697,53.2242768141699));
#38795=CARTESIAN_POINT('Ctrl Pts',(-30.034638236465,32.1216380022259,53.3354066033897));
#38796=CARTESIAN_POINT('Ctrl Pts',(-31.036220369854,33.7171187017325,53.4465363926093));
#38797=CARTESIAN_POINT('Ctrl Pts',(-32.9197159652556,33.7410461592535,53.5576661818291));
#38798=CARTESIAN_POINT('Ctrl Pts',(-33.961749285671,32.1717153833919,53.6687959710488));
#38799=CARTESIAN_POINT('Ctrl Pts',(-33.2079124381607,30.4449784545928,53.7799257602686));
#38800=CARTESIAN_POINT('Ctrl Pts',(-31.3495946744271,30.1418841716374,53.8910555494884));
#38801=CARTESIAN_POINT('Ctrl Pts',(-30.0845579647649,31.5383103207979,54.0021853387079));
#38802=CARTESIAN_POINT('Ctrl Pts',(-30.5764960375974,33.359377212299,54.1133151279278));
#38803=CARTESIAN_POINT('Ctrl Pts',(-31.7668777668624,33.7401334029927,54.1874016540742));
#38804=CARTESIAN_POINT('Ctrl Pts',(-32.3110796379505,33.6366995627948,54.2244449171475));
#38805=CARTESIAN_POINT('Ctrl Pts',(-33.3677806246589,33.1633123698097,40.9251850276175));
#38806=CARTESIAN_POINT('Ctrl Pts',(-33.7545814662436,32.7085259251269,40.9622282906908));
#38807=CARTESIAN_POINT('Ctrl Pts',(-34.0319373921236,31.3903858817126,41.0363148168372));
#38808=CARTESIAN_POINT('Ctrl Pts',(-32.5877567267128,29.9594098734121,41.147444606057));
#38809=CARTESIAN_POINT('Ctrl Pts',(-30.6055202467562,30.4008142160622,41.2585743952767));
#38810=CARTESIAN_POINT('Ctrl Pts',(-29.8995985779794,32.3034005478518,41.3697041844964));
#38811=CARTESIAN_POINT('Ctrl Pts',(-31.1158875333191,33.9295115308857,41.4808339737162));
#38812=CARTESIAN_POINT('Ctrl Pts',(-33.1413341001019,33.7891520709486,41.5919637629358));
#38813=CARTESIAN_POINT('Ctrl Pts',(-34.1222301817997,32.0116843221782,41.7030935521556));
#38814=CARTESIAN_POINT('Ctrl Pts',(-33.160891236097,30.2233694933969,41.8142233413753));
#38815=CARTESIAN_POINT('Ctrl Pts',(-31.1371136737856,30.0610852912993,41.9253531305951));
#38816=CARTESIAN_POINT('Ctrl Pts',(-29.9030421113392,31.6732355746631,42.0364829198147));
#38817=CARTESIAN_POINT('Ctrl Pts',(-30.5880827628849,33.5844569344168,42.1476127090346));
#38818=CARTESIAN_POINT('Ctrl Pts',(-32.5652952154986,34.0455904788454,42.2587424982542));
#38819=CARTESIAN_POINT('Ctrl Pts',(-34.0251553862571,32.6346268582552,42.369872287474));
#38820=CARTESIAN_POINT('Ctrl Pts',(-33.6316154261069,30.6428570641638,42.4810020766937));
#38821=CARTESIAN_POINT('Ctrl Pts',(-31.7448386631624,29.8931310581221,42.5921318659134));
#38822=CARTESIAN_POINT('Ctrl Pts',(-30.0915828183645,31.0715880075684,42.7032616551331));
#38823=CARTESIAN_POINT('Ctrl Pts',(-30.1848896672314,33.0997178736966,42.8143914443529));
#38824=CARTESIAN_POINT('Ctrl Pts',(-31.9393658161969,34.1213977013457,42.9255212335726));
#38825=CARTESIAN_POINT('Ctrl Pts',(-33.749333708789,33.2015974423935,43.0366510227923));
#38826=CARTESIAN_POINT('Ctrl Pts',(-33.9583303637712,31.1821081924737,43.147780812012));
#38827=CARTESIAN_POINT('Ctrl Pts',(-32.3750843060586,29.9111446765901,43.2589106012318));
#38828=CARTESIAN_POINT('Ctrl Pts',(-30.4485651595561,30.5518788891597,43.3700403904515));
#38829=CARTESIAN_POINT('Ctrl Pts',(-29.9419023541675,32.5179178436264,43.4811701796712));
#38830=CARTESIAN_POINT('Ctrl Pts',(-31.3187881952316,34.0099640014252,43.592299968891));
#38831=CARTESIAN_POINT('Ctrl Pts',(-33.3191116925215,33.6625129036691,43.7034297581106));
#38832=CARTESIAN_POINT('Ctrl Pts',(-34.1121984740185,31.7935480249707,43.8145595473304));
#38833=CARTESIAN_POINT('Ctrl Pts',(-32.9722241179162,30.1135257552974,43.9256893365501));
#38834=CARTESIAN_POINT('Ctrl Pts',(-30.9424807924367,30.1599842562344,44.0368191257698));
#38835=CARTESIAN_POINT('Ctrl Pts',(-29.8805675773967,31.8904052118169,44.1479489149896));
#38836=CARTESIAN_POINT('Ctrl Pts',(-30.7583359312378,33.7211261289926,44.2590787042093));
#38837=CARTESIAN_POINT('Ctrl Pts',(-32.7724617755229,33.9766910777731,44.3702084934291));
#38838=CARTESIAN_POINT('Ctrl Pts',(-34.0796389798491,32.4232097884861,44.4813382826487));
#38839=CARTESIAN_POINT('Ctrl Pts',(-33.4835531425627,30.4824114903015,44.5924680718685));
#38840=CARTESIAN_POINT('Ctrl Pts',(-31.529735557667,29.9304937386279,44.7035978610882));
#38841=CARTESIAN_POINT('Ctrl Pts',(-30.0062988905888,31.2725656745027,44.814727650308));
#38842=CARTESIAN_POINT('Ctrl Pts',(-30.3074758580556,33.2803776163751,44.9258574395276));
#38843=CARTESIAN_POINT('Ctrl Pts',(-32.1576325655698,34.1164018488584,45.0369872287475));
#38844=CARTESIAN_POINT('Ctrl Pts',(-33.8635256585285,33.0155180606887,45.148117017967));
#38845=CARTESIAN_POINT('Ctrl Pts',(-33.8639402778962,30.9852431562115,45.259246807187));
#38846=CARTESIAN_POINT('Ctrl Pts',(-32.1584969685238,29.8836627105899,45.3703765964065));
#38847=CARTESIAN_POINT('Ctrl Pts',(-30.3079989523865,30.718931201514,45.4815063856263));
#38848=CARTESIAN_POINT('Ctrl Pts',(-30.0060019460378,32.7266199642001,45.592636174846));
#38849=CARTESIAN_POINT('Ctrl Pts',(-31.5288903346668,34.0693140155155,45.7037659640658));
#38850=CARTESIAN_POINT('Ctrl Pts',(-33.4829331800372,33.5181943206072,45.8148957532854));
#38851=CARTESIAN_POINT('Ctrl Pts',(-34.0798116607782,31.577639647611,45.9260255425052));
#38852=CARTESIAN_POINT('Ctrl Pts',(-32.7732690641933,30.0236245888139,46.0371553317249));
#38853=CARTESIAN_POINT('Ctrl Pts',(-30.7590390058124,30.2783668734355,46.1482851209447));
#38854=CARTESIAN_POINT('Ctrl Pts',(-29.8805229916505,32.108729125155,46.2594149101643));
#38855=CARTESIAN_POINT('Ctrl Pts',(-30.9417293507589,33.839583660651,46.3705446993842));
#38856=CARTESIAN_POINT('Ctrl Pts',(-32.9714535315855,33.8868711793732,46.4816744886038));
#38857=CARTESIAN_POINT('Ctrl Pts',(-34.1121139752799,32.207314656999,46.5928042778236));
#38858=CARTESIAN_POINT('Ctrl Pts',(-33.3197906137204,30.3380260087731,46.7039340670433));
#38859=CARTESIAN_POINT('Ctrl Pts',(-31.3196091950172,29.9897579339606,46.8150638562631));
#38860=CARTESIAN_POINT('Ctrl Pts',(-29.9421140625033,31.4812415978201,46.9261936454828));
#38861=CARTESIAN_POINT('Ctrl Pts',(-30.4479738231426,33.4474873256539,47.0373234347025));
#38862=CARTESIAN_POINT('Ctrl Pts',(-32.3742311098188,34.0890083503957,47.1484532239222));
#38863=CARTESIAN_POINT('Ctrl Pts',(-33.9579961431562,32.8186915872076,47.259583013142));
#38864=CARTESIAN_POINT('Ctrl Pts',(-33.7498243398611,30.7991171617476,47.3707128023616));
#38865=CARTESIAN_POINT('Ctrl Pts',(-31.9402322767798,29.8785776868242,47.4818425915814));
#38866=CARTESIAN_POINT('Ctrl Pts',(-30.1853389858357,30.8995409070522,47.5929723808011));
#38867=CARTESIAN_POINT('Ctrl Pts',(-30.0912037758755,32.9276323551642,47.7041021700208));
#38868=CARTESIAN_POINT('Ctrl Pts',(-31.743978170201,34.1067647315839,47.8152319592406));
#38869=CARTESIAN_POINT('Ctrl Pts',(-33.6310609667174,33.3578088725702,47.9263617484603));
#38870=CARTESIAN_POINT('Ctrl Pts',(-34.0254144546136,31.3662010582043,48.03749153768));
#38871=CARTESIAN_POINT('Ctrl Pts',(-32.5661305983527,29.9546391621066,48.1486213268998));
#38872=CARTESIAN_POINT('Ctrl Pts',(-30.58873015791,30.4149693238342,48.2597511161195));
#38873=CARTESIAN_POINT('Ctrl Pts',(-29.9029085723639,32.3259023714469,48.3708809053392));
#38874=CARTESIAN_POINT('Ctrl Pts',(-31.1363223193809,33.9385731029754,48.4820106945589));
#38875=CARTESIAN_POINT('Ctrl Pts',(-33.160164513506,33.7770827536107,48.5931404837786));
#38876=CARTESIAN_POINT('Ctrl Pts',(-34.1222367263307,31.9892255398015,48.7042702729984));
#38877=CARTESIAN_POINT('Ctrl Pts',(-33.1420609019164,30.2112289951218,48.8154000622181));
#38878=CARTESIAN_POINT('Ctrl Pts',(-31.1166833252031,30.0702962756928,48.9265298514378));
#38879=CARTESIAN_POINT('Ctrl Pts',(-29.8997075900934,31.6954074779844,49.0376596406576));
#38880=CARTESIAN_POINT('Ctrl Pts',(-30.6048966918075,33.5992784532562,49.1487894298772));
#38881=CARTESIAN_POINT('Ctrl Pts',(-32.586869211914,34.0395071315606,49.259919219097));
#38882=CARTESIAN_POINT('Ctrl Pts',(-34.0317453936084,32.6132010005946,49.3710490083167));
#38883=CARTESIAN_POINT('Ctrl Pts',(-33.6171902244337,30.6256999637723,49.4821787975365));
#38884=CARTESIAN_POINT('Ctrl Pts',(-31.7226000995549,29.8959434164423,49.5933085867562));
#38885=CARTESIAN_POINT('Ctrl Pts',(-30.0818833552869,31.0917966368408,49.7044383759759));
#38886=CARTESIAN_POINT('Ctrl Pts',(-30.1966061631514,33.1188277261472,49.8155681651957));
#38887=CARTESIAN_POINT('Ctrl Pts',(-31.961775453508,34.1219198136651,49.9266979544153));
#38888=CARTESIAN_POINT('Ctrl Pts',(-33.7619274342862,33.183053898979,50.0378277436351));
#38889=CARTESIAN_POINT('Ctrl Pts',(-33.9495825345129,31.1614698856324,50.1489575328548));
#38890=CARTESIAN_POINT('Ctrl Pts',(-32.353000841496,29.9072995394748,50.2600873220746));
#38891=CARTESIAN_POINT('Ctrl Pts',(-30.433356606476,30.5683459603981,50.3712171112943));
#38892=CARTESIAN_POINT('Ctrl Pts',(-29.9474874156704,32.539626632724,50.482346900514));
#38893=CARTESIAN_POINT('Ctrl Pts',(-31.3400554834685,34.0170468627869,50.5934766897337));
#38894=CARTESIAN_POINT('Ctrl Pts',(-33.3365976160012,33.6484876779921,50.7046064789535));
#38895=CARTESIAN_POINT('Ctrl Pts',(-34.1099001051568,31.7712504473981,50.8157362681732));
#38896=CARTESIAN_POINT('Ctrl Pts',(-32.9522448990074,30.1033623266704,50.9268660573929));
#38897=CARTESIAN_POINT('Ctrl Pts',(-30.9231054879113,30.1712564363739,51.0379958466126));
#38898=CARTESIAN_POINT('Ctrl Pts',(-29.8795282559254,31.9127968236512,51.1491256358324));
#38899=CARTESIAN_POINT('Ctrl Pts',(-30.7765837683972,33.7341446121621,51.2602554250521));
#38900=CARTESIAN_POINT('Ctrl Pts',(-32.7932965489535,33.9684220577994,51.3713852142719));
#38901=CARTESIAN_POINT('Ctrl Pts',(-34.0839929302207,32.4012209824662,51.4825150034915));
#38902=CARTESIAN_POINT('Ctrl Pts',(-33.4674415829586,30.4668268156755,51.5936447927113));
#38903=CARTESIAN_POINT('Ctrl Pts',(-31.5079036102468,29.9355761193503,51.7047745819309));
#38904=CARTESIAN_POINT('Ctrl Pts',(-29.9987269217578,31.29366377334,51.8159043711508));
#38905=CARTESIAN_POINT('Ctrl Pts',(-30.321093641906,33.2981826771447,51.9270341603704));
#38906=CARTESIAN_POINT('Ctrl Pts',(-32.1799772731366,34.1146188827839,52.0381639495902));
#38907=CARTESIAN_POINT('Ctrl Pts',(-33.8741476178852,32.9957787996815,52.1492937388098));
#38908=CARTESIAN_POINT('Ctrl Pts',(-33.853118462012,30.9656127960953,52.2604235280297));
#38909=CARTESIAN_POINT('Ctrl Pts',(-32.1361352375125,29.882106668418,52.3715533172493));
#38910=CARTESIAN_POINT('Ctrl Pts',(-30.294562813773,30.736873699941,52.4826831064691));
#38911=CARTESIAN_POINT('Ctrl Pts',(-30.0137874265877,32.7476399268491,52.5938128956888));
#38912=CARTESIAN_POINT('Ctrl Pts',(-31.5507733982484,34.0741747872307,52.7049426849085));
#38913=CARTESIAN_POINT('Ctrl Pts',(-33.4988844053163,33.5024462144477,52.8160724741283));
#38914=CARTESIAN_POINT('Ctrl Pts',(-34.0752371703226,31.5556974584861,52.927202263348));
#38915=CARTESIAN_POINT('Ctrl Pts',(-32.7523464526881,30.0155650195559,53.0383320525678));
#38916=CARTESIAN_POINT('Ctrl Pts',(-30.7409340959589,30.2915749624683,53.1494618417874));
#38917=CARTESIAN_POINT('Ctrl Pts',(-29.8817702121404,32.1310991413546,53.2605916310072));
#38918=CARTESIAN_POINT('Ctrl Pts',(-30.9612565180695,33.8506781045533,53.3717214202268));
#38919=CARTESIAN_POINT('Ctrl Pts',(-32.9912524961666,33.8764666663383,53.4828512094467));
#38920=CARTESIAN_POINT('Ctrl Pts',(-34.1143363274486,32.185071596936,53.5939809986663));
#38921=CARTESIAN_POINT('Ctrl Pts',(-33.301865211337,30.3240271489152,53.7051107878861));
#38922=CARTESIAN_POINT('Ctrl Pts',(-31.2990054246639,29.9973578554558,53.8162405771058));
#38923=CARTESIAN_POINT('Ctrl Pts',(-29.9355727524405,31.5023995839451,53.9273703663255));
#38924=CARTESIAN_POINT('Ctrl Pts',(-30.4657743158319,33.465111084104,54.0385001555453));
#38925=CARTESIAN_POINT('Ctrl Pts',(-31.7487452602333,33.8754829148801,54.1125866816917));
#38926=CARTESIAN_POINT('Ctrl Pts',(-32.3352757582493,33.7640038755272,54.149629944765));
#38927=CARTESIAN_POINT('Ctrl Pts',(-33.4664903694653,33.2472660865709,40.850370055235));
#38928=CARTESIAN_POINT('Ctrl Pts',(-33.8812057842465,32.75965869598,40.8874133183083));
#38929=CARTESIAN_POINT('Ctrl Pts',(-34.1785778824356,31.3463913602508,40.9614998444547));
#38930=CARTESIAN_POINT('Ctrl Pts',(-32.6301738478915,29.8121449341238,41.0726296336745));
#38931=CARTESIAN_POINT('Ctrl Pts',(-30.5048836840657,30.2854044655623,41.1837594228942));
#38932=CARTESIAN_POINT('Ctrl Pts',(-29.7480171879371,32.3252963037301,41.294889212114));
#38933=CARTESIAN_POINT('Ctrl Pts',(-31.0520830646837,34.0687601701639,41.4060190013336));
#38934=CARTESIAN_POINT('Ctrl Pts',(-33.2237016930687,33.918271274101,41.5171487905534));
#38935=CARTESIAN_POINT('Ctrl Pts',(-34.2753869058308,32.0125275542285,41.6282785797731));
#38936=CARTESIAN_POINT('Ctrl Pts',(-33.2446702249182,30.095153944236,41.7394083689928));
#38937=CARTESIAN_POINT('Ctrl Pts',(-31.0748410494174,29.9211580451847,41.8505381582126));
#38938=CARTESIAN_POINT('Ctrl Pts',(-29.7517092335898,31.649653698699,41.9616679474322));
#38939=CARTESIAN_POINT('Ctrl Pts',(-30.4861877750113,33.6988037359677,42.0727977366521));
#38940=CARTESIAN_POINT('Ctrl Pts',(-32.6060913383974,34.1932162826512,42.1839275258717));
#38941=CARTESIAN_POINT('Ctrl Pts',(-34.171306433996,32.6804264946123,42.2950573150915));
#38942=CARTESIAN_POINT('Ctrl Pts',(-33.7493655531593,30.544915018161,42.4061871043112));
#38943=CARTESIAN_POINT('Ctrl Pts',(-31.7264242259422,29.7410829212761,42.5173168935309));
#38944=CARTESIAN_POINT('Ctrl Pts',(-29.9538565122688,31.0045865387686,42.6284466827506));
#38945=CARTESIAN_POINT('Ctrl Pts',(-30.0538971129336,33.1790821143611,42.7395764719704));
#38946=CARTESIAN_POINT('Ctrl Pts',(-31.9349899793838,34.2744943470779,42.8507062611901));
#38947=CARTESIAN_POINT('Ctrl Pts',(-33.8755793075807,33.2883141093505,42.9618360504098));
#38948=CARTESIAN_POINT('Ctrl Pts',(-34.0996587953703,31.1230827243945,43.0729658396296));
#38949=CARTESIAN_POINT('Ctrl Pts',(-32.4021533224376,29.7603965433046,43.1840956288492));
#38950=CARTESIAN_POINT('Ctrl Pts',(-30.3366014905122,30.4473711466732,43.2952254180691));
#38951=CARTESIAN_POINT('Ctrl Pts',(-29.793373935396,32.5552948449183,43.4063552072887));
#38952=CARTESIAN_POINT('Ctrl Pts',(-31.2696266248778,34.1550187200504,43.5174849965085));
#38953=CARTESIAN_POINT('Ctrl Pts',(-33.4143091066335,33.7824928342954,43.6286147857282));
#38954=CARTESIAN_POINT('Ctrl Pts',(-34.2646312315764,31.7786488361662,43.7397445749479));
#38955=CARTESIAN_POINT('Ctrl Pts',(-33.0423874122662,29.9773830231067,43.8508743641677));
#38956=CARTESIAN_POINT('Ctrl Pts',(-30.8661619374796,30.027194332739,43.9620041533873));
#38957=CARTESIAN_POINT('Ctrl Pts',(-29.7276127615454,31.8824959949596,44.0731339426071));
#38958=CARTESIAN_POINT('Ctrl Pts',(-30.6687277432337,33.845336048266,44.1842637318268));
#38959=CARTESIAN_POINT('Ctrl Pts',(-32.8282086572669,34.1193445620604,44.2953935210466));
#38960=CARTESIAN_POINT('Ctrl Pts',(-34.2297219897189,32.4537519159793,44.4065233102662));
#38961=CARTESIAN_POINT('Ctrl Pts',(-33.590617937508,30.3728904371349,44.517653099486));
#38962=CARTESIAN_POINT('Ctrl Pts',(-31.4957975984231,29.781141984953,44.6287828887056));
#38963=CARTESIAN_POINT('Ctrl Pts',(-29.862417829414,31.2200683256305,44.7399126779256));
#38964=CARTESIAN_POINT('Ctrl Pts',(-30.1853300818118,33.3727796766834,44.8510424671451));
#38965=CARTESIAN_POINT('Ctrl Pts',(-32.1690085640597,34.2691379548117,44.962172256365));
#38966=CARTESIAN_POINT('Ctrl Pts',(-33.9980122413016,33.0888057844725,45.0733020455846));
#38967=CARTESIAN_POINT('Ctrl Pts',(-33.9984567828449,30.9120103677913,45.1844318348044));
#38968=CARTESIAN_POINT('Ctrl Pts',(-32.1699353490897,29.7309312637511,45.295561624024));
#38969=CARTESIAN_POINT('Ctrl Pts',(-30.1858909267199,30.6264792601002,45.4066914132438));
#38970=CARTESIAN_POINT('Ctrl Pts',(-29.8620994550223,32.7790585423934,45.5178212024635));
#38971=CARTESIAN_POINT('Ctrl Pts',(-31.4948913775223,34.2186518952262,45.6289509916833));
#38972=CARTESIAN_POINT('Ctrl Pts',(-33.589953233639,33.627759093826,45.740080780903));
#38973=CARTESIAN_POINT('Ctrl Pts',(-34.2299071326541,31.5471588220685,45.8512105701227));
#38974=CARTESIAN_POINT('Ctrl Pts',(-32.8290742062001,29.8809938854959,45.9623403593424));
#38975=CARTESIAN_POINT('Ctrl Pts',(-30.6694815571671,30.154120365253,46.0734701485622));
#38976=CARTESIAN_POINT('Ctrl Pts',(-29.7275649581431,32.1165758689995,46.1845999377818));
#38977=CARTESIAN_POINT('Ctrl Pts',(-30.8653562658947,33.9723424016504,46.2957297270017));
#38978=CARTESIAN_POINT('Ctrl Pts',(-33.0415612144005,34.0230425574734,46.4068595162213));
#38979=CARTESIAN_POINT('Ctrl Pts',(-34.2645406347481,32.2222761036798,46.5179893054411));
#38980=CARTESIAN_POINT('Ctrl Pts',(-33.4150370240947,30.2180849702824,46.6291190946608));
#38981=CARTESIAN_POINT('Ctrl Pts',(-31.2705068744274,29.8446831480187,46.7402488838805));
#38982=CARTESIAN_POINT('Ctrl Pts',(-29.7936009222607,31.4438039352503,46.8513786731003));
#38983=CARTESIAN_POINT('Ctrl Pts',(-30.3359674786392,33.5519493292456,46.96250846232));
#38984=CARTESIAN_POINT('Ctrl Pts',(-32.401238552886,34.2397675273051,47.0736382515397));
#38985=CARTESIAN_POINT('Ctrl Pts',(-34.0993004547824,32.8777747736423,47.1847680407595));
#38986=CARTESIAN_POINT('Ctrl Pts',(-33.8761053464274,30.7124520662131,47.2958978299791));
#38987=CARTESIAN_POINT('Ctrl Pts',(-31.9359189705373,29.7254792649098,47.4070276191989));
#38988=CARTESIAN_POINT('Ctrl Pts',(-30.0543788578817,30.8201231742108,47.5181574084186));
#38989=CARTESIAN_POINT('Ctrl Pts',(-29.95345011511,32.9945775592427,47.6292871976383));
#38990=CARTESIAN_POINT('Ctrl Pts',(-31.7255016330804,34.2588053478002,47.7404169868581));
#38991=CARTESIAN_POINT('Ctrl Pts',(-33.7487710796447,33.4557989777749,47.8515467760777));
#38992=CARTESIAN_POINT('Ctrl Pts',(-34.1715841987509,31.3204611707726,47.9626765652976));
#38993=CARTESIAN_POINT('Ctrl Pts',(-32.6069870090102,29.8070299309874,48.0738063545172));
#38994=CARTESIAN_POINT('Ctrl Pts',(-30.4868818911235,30.3005811165925,48.184936143737));
#38995=CARTESIAN_POINT('Ctrl Pts',(-29.7515660573979,32.3494220348617,48.2960659329567));
#38996=CARTESIAN_POINT('Ctrl Pts',(-31.073992584691,34.0784756961497,48.4071957221765));
#38997=CARTESIAN_POINT('Ctrl Pts',(-33.2438910563427,33.9053309404518,48.5183255113961));
#38998=CARTESIAN_POINT('Ctrl Pts',(-34.2753939226663,31.988447970506,48.6294553006159));
#38999=CARTESIAN_POINT('Ctrl Pts',(-33.2244809465853,30.0821372926766,48.7405850898356));
#39000=CARTESIAN_POINT('Ctrl Pts',(-31.0529362871324,29.9310337662346,48.8517148790553));
#39001=CARTESIAN_POINT('Ctrl Pts',(-29.7481340672176,31.6734256999301,48.9628446682751));
#39002=CARTESIAN_POINT('Ctrl Pts',(-30.5042151285161,33.7146948914988,49.0739744574948));
#39003=CARTESIAN_POINT('Ctrl Pts',(-32.6292222830852,34.1866939134596,49.1851042467145));
#39004=CARTESIAN_POINT('Ctrl Pts',(-34.1783720278063,32.6574543795302,49.2962340359342));
#39005=CARTESIAN_POINT('Ctrl Pts',(-33.7338993161399,30.5265197272506,49.407363825154));
#39006=CARTESIAN_POINT('Ctrl Pts',(-31.7025807536974,29.7440982413631,49.5184936143737));
#39007=CARTESIAN_POINT('Ctrl Pts',(-29.9434570600936,31.0262535807442,49.6296234035934));
#39008=CARTESIAN_POINT('Ctrl Pts',(-30.0664591628126,33.199571083188,49.7407531928132));
#39009=CARTESIAN_POINT('Ctrl Pts',(-31.9590168713483,34.2750541391048,49.8518829820328));
#39010=CARTESIAN_POINT('Ctrl Pts',(-33.8890818947825,33.2684323188477,49.9630127712527));
#39011=CARTESIAN_POINT('Ctrl Pts',(-34.0902796543517,31.1009549959568,50.0741425604723));
#39012=CARTESIAN_POINT('Ctrl Pts',(-32.3784761423976,29.7562739110293,50.1852723496921));
#39013=CARTESIAN_POINT('Ctrl Pts',(-30.3202953693232,30.4650266105312,50.2964021389118));
#39014=CARTESIAN_POINT('Ctrl Pts',(-29.7993620586076,32.5785703099824,50.4075319281315));
#39015=CARTESIAN_POINT('Ctrl Pts',(-31.2924287269267,34.1626127360701,50.5186617173513));
#39016=CARTESIAN_POINT('Ctrl Pts',(-33.4330569510772,33.7674554386677,50.629791506571));
#39017=CARTESIAN_POINT('Ctrl Pts',(-34.2621669944462,31.7547420910471,50.7409212957907));
#39018=CARTESIAN_POINT('Ctrl Pts',(-33.0209663366997,29.9664861220002,50.8520510850105));
#39019=CARTESIAN_POINT('Ctrl Pts',(-30.8453883594806,30.0392800015366,50.9631808742301));
#39020=CARTESIAN_POINT('Ctrl Pts',(-29.72649843451,31.9065035605881,51.0743106634499));
#39021=CARTESIAN_POINT('Ctrl Pts',(-30.6882924870058,33.8592940469749,51.1854404526696));
#39022=CARTESIAN_POINT('Ctrl Pts',(-32.8505470308592,34.1104787849484,51.2965702418894));
#39023=CARTESIAN_POINT('Ctrl Pts',(-34.2343901551937,32.4301762257824,51.407700031109));
#39024=CARTESIAN_POINT('Ctrl Pts',(-33.5733436417835,30.3561810505284,51.5188298203289));
#39025=CARTESIAN_POINT('Ctrl Pts',(-31.472390086969,29.7865911500084,51.6299596095484));
#39026=CARTESIAN_POINT('Ctrl Pts',(-29.8542994081055,31.2426890282499,51.7410893987682));
#39027=CARTESIAN_POINT('Ctrl Pts',(-30.1999306314249,33.3918696898592,51.852219187988));
#39028=CARTESIAN_POINT('Ctrl Pts',(-32.1929658404419,34.2672263159639,51.9633489772077));
#39029=CARTESIAN_POINT('Ctrl Pts',(-34.0094007643006,33.0676419840461,52.0744787664274));
#39030=CARTESIAN_POINT('Ctrl Pts',(-33.9868539801086,30.8909633273957,52.1856085556472));
#39031=CARTESIAN_POINT('Ctrl Pts',(-32.1459598207181,29.7292629254092,52.2967383448669));
#39032=CARTESIAN_POINT('Ctrl Pts',(-30.1714851312844,30.6457166295093,52.4078681340866));
#39033=CARTESIAN_POINT('Ctrl Pts',(-29.8704467967248,32.8015954699061,52.5189979233063));
#39034=CARTESIAN_POINT('Ctrl Pts',(-31.5183536940796,34.2238634582357,52.630127712526));
#39035=CARTESIAN_POINT('Ctrl Pts',(-33.6070556240599,33.6108744811885,52.7412575017458));
#39036=CARTESIAN_POINT('Ctrl Pts',(-34.2250025111984,31.5236331130063,52.8523872909654));
#39037=CARTESIAN_POINT('Ctrl Pts',(-32.8066416554509,29.8723526747009,52.9635170801853));
#39038=CARTESIAN_POINT('Ctrl Pts',(-30.6500700554528,30.168281653267,53.0746468694049));
#39039=CARTESIAN_POINT('Ctrl Pts',(-29.7289021878159,32.1405602804833,53.1857766586248));
#39040=CARTESIAN_POINT('Ctrl Pts',(-30.8862926662849,33.9842375073741,53.2969064478443));
#39041=CARTESIAN_POINT('Ctrl Pts',(-33.0627890270775,34.0118871734231,53.4080362370642));
#39042=CARTESIAN_POINT('Ctrl Pts',(-34.2669233692262,32.1984278104801,53.5191660262838));
#39043=CARTESIAN_POINT('Ctrl Pts',(-33.3958179845133,30.2030758432375,53.6302958155037));
#39044=CARTESIAN_POINT('Ctrl Pts',(-31.2484161749007,29.8528315392741,53.7414256047233));
#39045=CARTESIAN_POINT('Ctrl Pts',(-29.786587540116,31.4664888470924,53.8525553939431));
#39046=CARTESIAN_POINT('Ctrl Pts',(-30.3550525940664,33.5708449559089,53.9636851831627));
#39047=CARTESIAN_POINT('Ctrl Pts',(-31.7306127536042,34.0108324267675,54.0377717093093));
#39048=CARTESIAN_POINT('Ctrl Pts',(-32.359471878548,33.8913081882596,54.0748149723825));
#39049=CARTESIAN_POINT('Ctrl Pts',(-33.5652001142718,33.3312198033321,40.7755550828525));
#39050=CARTESIAN_POINT('Ctrl Pts',(-34.0078301022494,32.8107914668331,40.8125983459258));
#39051=CARTESIAN_POINT('Ctrl Pts',(-34.3252183727475,31.3023968387891,40.8866848720723));
#39052=CARTESIAN_POINT('Ctrl Pts',(-32.6725909690703,29.6648799948355,40.997814661292));
#39053=CARTESIAN_POINT('Ctrl Pts',(-30.4042471213751,30.1699947150623,41.1089444505117));
#39054=CARTESIAN_POINT('Ctrl Pts',(-29.5964357978947,32.3471920596084,41.2200742397314));
#39055=CARTESIAN_POINT('Ctrl Pts',(-30.9882785960482,34.2080088094421,41.3312040289512));
#39056=CARTESIAN_POINT('Ctrl Pts',(-33.3060692860357,34.0473904772534,41.4423338181709));
#39057=CARTESIAN_POINT('Ctrl Pts',(-34.4285436298619,32.0133707862788,41.5534636073906));
#39058=CARTESIAN_POINT('Ctrl Pts',(-33.3284492137394,29.9669383950752,41.6645933966104));
#39059=CARTESIAN_POINT('Ctrl Pts',(-31.0125684250491,29.7812307990702,41.7757231858301));
#39060=CARTESIAN_POINT('Ctrl Pts',(-29.6003763558403,31.6260718227349,41.8868529750497));
#39061=CARTESIAN_POINT('Ctrl Pts',(-30.3842927871376,33.8131505375187,41.9979827642696));
#39062=CARTESIAN_POINT('Ctrl Pts',(-32.6468874612962,34.3408420864571,42.1091125534892));
#39063=CARTESIAN_POINT('Ctrl Pts',(-34.3174574817349,32.7262261309694,42.220242342709));
#39064=CARTESIAN_POINT('Ctrl Pts',(-33.8671156802116,30.446972972158,42.3313721319287));
#39065=CARTESIAN_POINT('Ctrl Pts',(-31.708009788722,29.5890347844302,42.4425019211484));
#39066=CARTESIAN_POINT('Ctrl Pts',(-29.8161302061732,30.9375850699686,42.5536317103681));
#39067=CARTESIAN_POINT('Ctrl Pts',(-29.9229045586358,33.2584463550257,42.6647614995879));
#39068=CARTESIAN_POINT('Ctrl Pts',(-31.9306141425706,34.4275909928101,42.7758912888076));
#39069=CARTESIAN_POINT('Ctrl Pts',(-34.0018249063725,33.3750307763075,42.8870210780274));
#39070=CARTESIAN_POINT('Ctrl Pts',(-34.2409872269693,31.0640572563152,42.998150867247));
#39071=CARTESIAN_POINT('Ctrl Pts',(-32.4292223388168,29.6096484100191,43.1092806564668));
#39072=CARTESIAN_POINT('Ctrl Pts',(-30.2246378214682,30.3428634041866,43.2204104456865));
#39073=CARTESIAN_POINT('Ctrl Pts',(-29.6448455166245,32.5926718462104,43.3315402349062));
#39074=CARTESIAN_POINT('Ctrl Pts',(-31.2204650545239,34.3000734386756,43.442670024126));
#39075=CARTESIAN_POINT('Ctrl Pts',(-33.5095065207455,33.9024727649217,43.5537998133457));
#39076=CARTESIAN_POINT('Ctrl Pts',(-34.4170639891342,31.7637496473617,43.6649296025654));
#39077=CARTESIAN_POINT('Ctrl Pts',(-33.1125507066162,29.841240290916,43.7760593917852));
#39078=CARTESIAN_POINT('Ctrl Pts',(-30.7898430825224,29.8944044092436,43.8871891810048));
#39079=CARTESIAN_POINT('Ctrl Pts',(-29.5746579456941,31.8745867781023,43.9983189702246));
#39080=CARTESIAN_POINT('Ctrl Pts',(-30.5791195552295,33.9695459675394,44.1094487594443));
#39081=CARTESIAN_POINT('Ctrl Pts',(-32.883955539011,34.2619980463476,44.2205785486641));
#39082=CARTESIAN_POINT('Ctrl Pts',(-34.3798049995887,32.4842940434725,44.3317083378838));
#39083=CARTESIAN_POINT('Ctrl Pts',(-33.6976827324532,30.2633693839683,44.4428381271035));
#39084=CARTESIAN_POINT('Ctrl Pts',(-31.4618596391792,29.6317902312781,44.5539679163232));
#39085=CARTESIAN_POINT('Ctrl Pts',(-29.7185367682392,31.1675709767584,44.665097705543));
#39086=CARTESIAN_POINT('Ctrl Pts',(-30.0631843055681,33.4651817369917,44.7762274947626));
#39087=CARTESIAN_POINT('Ctrl Pts',(-32.1803845625496,34.421874060765,44.8873572839825));
#39088=CARTESIAN_POINT('Ctrl Pts',(-34.1324988240748,33.1620935082564,44.9984870732021));
#39089=CARTESIAN_POINT('Ctrl Pts',(-34.1329732877935,30.8387775793711,45.109616862422));
#39090=CARTESIAN_POINT('Ctrl Pts',(-32.1813737296557,29.5781998169125,45.2207466516415));
#39091=CARTESIAN_POINT('Ctrl Pts',(-30.0637829010532,30.5340273186863,45.3318764408613));
#39092=CARTESIAN_POINT('Ctrl Pts',(-29.7181969640068,32.8314971205867,45.4430062300811));
#39093=CARTESIAN_POINT('Ctrl Pts',(-31.4608924203777,34.3679897749369,45.5541360193008));
#39094=CARTESIAN_POINT('Ctrl Pts',(-33.6969732872408,33.7373238670447,45.6652658085205));
#39095=CARTESIAN_POINT('Ctrl Pts',(-34.38000260453,31.5166779965259,45.7763955977402));
#39096=CARTESIAN_POINT('Ctrl Pts',(-32.8848793482069,29.7383631821778,45.88752538696));
#39097=CARTESIAN_POINT('Ctrl Pts',(-30.5799241085217,30.0298738570706,45.9986551761797));
#39098=CARTESIAN_POINT('Ctrl Pts',(-29.5746069246357,32.1244226128439,46.1097849653993));
#39099=CARTESIAN_POINT('Ctrl Pts',(-30.7889831810305,34.1051011426497,46.2209147546192));
#39100=CARTESIAN_POINT('Ctrl Pts',(-33.1116688972156,34.1592139355736,46.3320445438388));
#39101=CARTESIAN_POINT('Ctrl Pts',(-34.4169672942162,32.2372375503608,46.4431743330586));
#39102=CARTESIAN_POINT('Ctrl Pts',(-33.510283434469,30.0981439317918,46.5543041222783));
#39103=CARTESIAN_POINT('Ctrl Pts',(-31.2214045538376,29.6996083620767,46.665433911498));
#39104=CARTESIAN_POINT('Ctrl Pts',(-29.645087782018,31.4063662726806,46.7765637007178));
#39105=CARTESIAN_POINT('Ctrl Pts',(-30.223961134136,33.6564113328374,46.8876934899375));
#39106=CARTESIAN_POINT('Ctrl Pts',(-32.4282459959531,34.3905267042144,46.9988232791572));
#39107=CARTESIAN_POINT('Ctrl Pts',(-34.2406047664085,32.9368579600769,47.109953068377));
#39108=CARTESIAN_POINT('Ctrl Pts',(-34.0023863529936,30.6257869706786,47.2210828575967));
#39109=CARTESIAN_POINT('Ctrl Pts',(-31.9316056642948,29.5723808429954,47.3322126468164));
#39110=CARTESIAN_POINT('Ctrl Pts',(-29.9234187299276,30.7407054413694,47.4433424360361));
#39111=CARTESIAN_POINT('Ctrl Pts',(-29.8156964543446,33.0615227633212,47.5544722252558));
#39112=CARTESIAN_POINT('Ctrl Pts',(-31.7070250959598,34.4108459640165,47.6656020144756));
#39113=CARTESIAN_POINT('Ctrl Pts',(-33.8664811925721,33.5537890829796,47.7767318036953));
#39114=CARTESIAN_POINT('Ctrl Pts',(-34.317753942888,31.2747212833408,47.8878615929151));
#39115=CARTESIAN_POINT('Ctrl Pts',(-32.6478434196678,29.6594206998682,47.9989913821348));
#39116=CARTESIAN_POINT('Ctrl Pts',(-30.3850336243369,30.1861929093508,48.1101211713545));
#39117=CARTESIAN_POINT('Ctrl Pts',(-29.6002235424318,32.3729416982765,48.2212509605743));
#39118=CARTESIAN_POINT('Ctrl Pts',(-31.0116628500012,34.2183782893241,48.3323807497939));
#39119=CARTESIAN_POINT('Ctrl Pts',(-33.3276175991793,34.0335791272928,48.4435105390137));
#39120=CARTESIAN_POINT('Ctrl Pts',(-34.4285511190019,31.9876704012107,48.5546403282334));
#39121=CARTESIAN_POINT('Ctrl Pts',(-33.3069009912542,29.9530455902315,48.6657701174531));
#39122=CARTESIAN_POINT('Ctrl Pts',(-30.9891892490617,29.7917712567763,48.7768999066728));
#39123=CARTESIAN_POINT('Ctrl Pts',(-29.5965605443418,31.6514439218759,48.8880296958926));
#39124=CARTESIAN_POINT('Ctrl Pts',(-30.4035335652247,33.8301113297414,48.9991594851123));
#39125=CARTESIAN_POINT('Ctrl Pts',(-32.6715753542565,34.3338806953585,49.110289274332));
#39126=CARTESIAN_POINT('Ctrl Pts',(-34.3249986620041,32.7017077584658,49.2214190635518));
#39127=CARTESIAN_POINT('Ctrl Pts',(-33.8506084078462,30.4273394907288,49.3325488527714));
#39128=CARTESIAN_POINT('Ctrl Pts',(-31.6825614078399,29.5922530662839,49.4436786419912));
#39129=CARTESIAN_POINT('Ctrl Pts',(-29.8050307649004,30.9607105246476,49.554808431211));
#39130=CARTESIAN_POINT('Ctrl Pts',(-29.9363121624739,33.2803144402289,49.6659382204307));
#39131=CARTESIAN_POINT('Ctrl Pts',(-31.9562582891885,34.4281884645445,49.7770680096504));
#39132=CARTESIAN_POINT('Ctrl Pts',(-34.0162363552789,33.3538107387165,49.8881977988702));
#39133=CARTESIAN_POINT('Ctrl Pts',(-34.2309767741905,31.040440106281,49.9993275880898));
#39134=CARTESIAN_POINT('Ctrl Pts',(-32.4039514432991,29.6052482825838,50.1104573773096));
#39135=CARTESIAN_POINT('Ctrl Pts',(-30.2072341321705,30.3617072606643,50.2215871665293));
#39136=CARTESIAN_POINT('Ctrl Pts',(-29.6512367015448,32.6175139872409,50.332716955749));
#39137=CARTESIAN_POINT('Ctrl Pts',(-31.2448019703849,34.3081786093532,50.4438467449688));
#39138=CARTESIAN_POINT('Ctrl Pts',(-33.5295162861532,33.8864231993434,50.5549765341884));
#39139=CARTESIAN_POINT('Ctrl Pts',(-34.4144338837356,31.738233734696,50.6661063234082));
#39140=CARTESIAN_POINT('Ctrl Pts',(-33.0896877743921,29.8296099173301,50.7772361126279));
#39141=CARTESIAN_POINT('Ctrl Pts',(-30.7676712310498,29.9073035666993,50.8883659018476));
#39142=CARTESIAN_POINT('Ctrl Pts',(-29.5734686130947,31.9002102975249,50.9994956910674));
#39143=CARTESIAN_POINT('Ctrl Pts',(-30.6000012056143,33.9844434817877,51.110625480287));
#39144=CARTESIAN_POINT('Ctrl Pts',(-32.907797512765,34.2525355120973,51.2217552695069));
#39145=CARTESIAN_POINT('Ctrl Pts',(-34.3847873801667,32.4591314690988,51.3328850587265));
#39146=CARTESIAN_POINT('Ctrl Pts',(-33.6792457006084,30.2455352853812,51.4440148479464));
#39147=CARTESIAN_POINT('Ctrl Pts',(-31.4368765636913,29.6376061806665,51.5551446371659));
#39148=CARTESIAN_POINT('Ctrl Pts',(-29.7098718944532,31.1917142831597,51.6662744263858));
#39149=CARTESIAN_POINT('Ctrl Pts',(-30.0787676209438,33.4855567025737,51.7774042156054));
#39150=CARTESIAN_POINT('Ctrl Pts',(-32.2059544077473,34.4198337491439,51.8885340048253));
#39151=CARTESIAN_POINT('Ctrl Pts',(-34.1446539107159,33.1395051684107,51.9996637940449));
#39152=CARTESIAN_POINT('Ctrl Pts',(-34.1205894982053,30.816313858696,52.1107935832648));
#39153=CARTESIAN_POINT('Ctrl Pts',(-32.1557844039238,29.5764191824004,52.2219233724843));
#39154=CARTESIAN_POINT('Ctrl Pts',(-30.0484074487957,30.5545595590777,52.3330531617041));
#39155=CARTESIAN_POINT('Ctrl Pts',(-29.7271061668619,32.8555510129632,52.4441829509238));
#39156=CARTESIAN_POINT('Ctrl Pts',(-31.4859339899109,34.3735521292407,52.5553127401435));
#39157=CARTESIAN_POINT('Ctrl Pts',(-33.7152268428034,33.7193027479294,52.6664425293632));
#39158=CARTESIAN_POINT('Ctrl Pts',(-34.3747678520742,31.4915687675265,52.777572318583));
#39159=CARTESIAN_POINT('Ctrl Pts',(-32.8609368582137,29.729140329846,52.8887021078027));
#39160=CARTESIAN_POINT('Ctrl Pts',(-30.5592060149468,30.0449883440656,52.9998318970225));
#39161=CARTESIAN_POINT('Ctrl Pts',(-29.5760341634913,32.150021419612,53.1109616862422));
#39162=CARTESIAN_POINT('Ctrl Pts',(-30.8113288145004,34.117796910195,53.2220914754619));
#39163=CARTESIAN_POINT('Ctrl Pts',(-33.1343255579885,34.1473076805079,53.3332212646816));
#39164=CARTESIAN_POINT('Ctrl Pts',(-34.4195104110039,32.2117840240242,53.4443510539014));
#39165=CARTESIAN_POINT('Ctrl Pts',(-33.4897707576895,30.0821245375598,53.5554808431211));
#39166=CARTESIAN_POINT('Ctrl Pts',(-31.1978269251376,29.7083052230924,53.6666106323408));
#39167=CARTESIAN_POINT('Ctrl Pts',(-29.6376023277916,31.4305781102398,53.7777404215605));
#39168=CARTESIAN_POINT('Ctrl Pts',(-30.2443308723009,33.6765788277138,53.8888702107803));
#39169=CARTESIAN_POINT('Ctrl Pts',(-31.7124802469751,34.146181938655,53.9629567369268));
#39170=CARTESIAN_POINT('Ctrl Pts',(-32.3836679988468,34.0186125009919,54.));
#39171=CARTESIAN_POINT('Ctrl Pts',(-33.2690708798524,33.0793586530485,41.));
#39172=CARTESIAN_POINT('Ctrl Pts',(-33.3144021367584,33.0370694015056,41.));
#39173=CARTESIAN_POINT('Ctrl Pts',(-33.357003518039,32.9922111868308,41.));
#39174=CARTESIAN_POINT('Ctrl Pts',(-33.396876415392,32.9451289935681,41.));
#39175=CARTESIAN_POINT('Ctrl Pts',(-33.4393774108012,32.8949435239245,41.));
#39176=CARTESIAN_POINT('Ctrl Pts',(-33.478779113966,32.8422310065705,41.));
#39177=CARTESIAN_POINT('Ctrl Pts',(-33.5150543890132,32.7873545360889,41.));
#39178=CARTESIAN_POINT('Ctrl Pts',(-33.5467952546795,32.7393376244174,41.));
#39179=CARTESIAN_POINT('Ctrl Pts',(-33.5761422056407,32.689662710961,41.));
#39180=CARTESIAN_POINT('Ctrl Pts',(-33.6030541769026,32.6385454943499,41.));
#39181=CARTESIAN_POINT('Ctrl Pts',(-33.6165537545645,32.6129040863392,41.));
#39182=CARTESIAN_POINT('Ctrl Pts',(-33.6294402762058,32.5868994069059,41.));
#39183=CARTESIAN_POINT('Ctrl Pts',(-33.641706218416,32.5605568410562,41.));
#39184=CARTESIAN_POINT('Ctrl Pts',(-33.6473173816178,32.5485062024991,41.));
#39185=CARTESIAN_POINT('Ctrl Pts',(-33.6527992584238,32.5363831634529,41.));
#39186=CARTESIAN_POINT('Ctrl Pts',(-33.6581426077326,32.5242101295597,41.));
#39187=CARTESIAN_POINT('Ctrl Pts',(-33.685064215522,32.4628782522786,41.));
#39188=CARTESIAN_POINT('Ctrl Pts',(-33.7085245448721,32.4001709264115,41.));
#39189=CARTESIAN_POINT('Ctrl Pts',(-33.728499993566,32.3364458568814,41.));
#39190=CARTESIAN_POINT('Ctrl Pts',(-33.7488294565481,32.2715914217246,41.));
#39191=CARTESIAN_POINT('Ctrl Pts',(-33.7655499805244,32.205682007983,41.));
#39192=CARTESIAN_POINT('Ctrl Pts',(-33.778597371195,32.139058167292,41.));
#39193=CARTESIAN_POINT('Ctrl Pts',(-33.7895089756291,32.0833402836288,41.));
#39194=CARTESIAN_POINT('Ctrl Pts',(-33.7978510101904,32.0271217838561,41.));
#39195=CARTESIAN_POINT('Ctrl Pts',(-33.8035611097405,31.97058958092,41.));
#39196=CARTESIAN_POINT('Ctrl Pts',(-33.8061908976541,31.9445536593552,41.));
#39197=CARTESIAN_POINT('Ctrl Pts',(-33.8082620999711,31.9184510862623,41.));
#39198=CARTESIAN_POINT('Ctrl Pts',(-33.8097668241107,31.8922997194398,41.));
#39199=CARTESIAN_POINT('Ctrl Pts',(-33.8104248596001,31.880863385687,41.));
#39200=CARTESIAN_POINT('Ctrl Pts',(-33.8109744437721,31.8694179108277,41.));
#39201=CARTESIAN_POINT('Ctrl Pts',(-33.8114145802126,31.8579789498471,41.));
#39202=CARTESIAN_POINT('Ctrl Pts',(-33.8141127536739,31.7878545563686,41.));
#39203=CARTESIAN_POINT('Ctrl Pts',(-33.8127099564223,31.7178435879866,41.));
#39204=CARTESIAN_POINT('Ctrl Pts',(-33.8071514622337,31.6483067461029,41.));
#39205=CARTESIAN_POINT('Ctrl Pts',(-33.8021840858831,31.5861647968351,41.));
#39206=CARTESIAN_POINT('Ctrl Pts',(-33.7938975383786,31.524400531023,41.));
#39207=CARTESIAN_POINT('Ctrl Pts',(-33.7822196781911,31.4632592560481,41.));
#39208=CARTESIAN_POINT('Ctrl Pts',(-33.769491639951,31.3966196085928,41.));
#39209=CARTESIAN_POINT('Ctrl Pts',(-33.7527359979084,31.3307192075773,41.));
#39210=CARTESIAN_POINT('Ctrl Pts',(-33.732198040194,31.2657716978078,41.));
#39211=CARTESIAN_POINT('Ctrl Pts',(-33.7242658128154,31.2406874892254,41.));
#39212=CARTESIAN_POINT('Ctrl Pts',(-33.7157688301419,31.2157454686801,41.));
#39213=CARTESIAN_POINT('Ctrl Pts',(-33.7067192107323,31.1909582653564,41.));
#39214=CARTESIAN_POINT('Ctrl Pts',(-33.7027507419357,31.1800884996244,41.));
#39215=CARTESIAN_POINT('Ctrl Pts',(-33.698676095927,31.1692490592239,41.));
#39216=CARTESIAN_POINT('Ctrl Pts',(-33.6945013882907,31.1584535681983,41.));
#39217=CARTESIAN_POINT('Ctrl Pts',(-33.6692787473599,31.0932296489372,41.));
#39218=CARTESIAN_POINT('Ctrl Pts',(-33.6403651885278,31.0294907437057,41.));
#39219=CARTESIAN_POINT('Ctrl Pts',(-33.6080734174902,30.9674557344658,41.));
#39220=CARTESIAN_POINT('Ctrl Pts',(-33.5750332658763,30.9039830278043,41.));
#39221=CARTESIAN_POINT('Ctrl Pts',(-33.5384562013509,30.8422932904506,41.));
#39222=CARTESIAN_POINT('Ctrl Pts',(-33.4986210386776,30.7826246842389,41.));
#39223=CARTESIAN_POINT('Ctrl Pts',(-33.4681150414624,30.7369301216272,41.));
#39224=CARTESIAN_POINT('Ctrl Pts',(-33.4356970894283,30.6924208354612,41.));
#39225=CARTESIAN_POINT('Ctrl Pts',(-33.401472825112,30.6492098980629,41.));
#39226=CARTESIAN_POINT('Ctrl Pts',(-33.3801641910076,30.6223060018733,41.));
#39227=CARTESIAN_POINT('Ctrl Pts',(-33.3581550105309,30.5959055373049,41.));
#39228=CARTESIAN_POINT('Ctrl Pts',(-33.3354678681772,30.5700374883911,41.));
#39229=CARTESIAN_POINT('Ctrl Pts',(-33.3228125346432,30.5556077827115,41.));
#39230=CARTESIAN_POINT('Ctrl Pts',(-33.3099418038776,30.5413392395066,41.));
#39231=CARTESIAN_POINT('Ctrl Pts',(-33.2968831946259,30.5272622022597,41.));
#39232=CARTESIAN_POINT('Ctrl Pts',(-33.2460103743684,30.4724218611623,41.));
#39233=CARTESIAN_POINT('Ctrl Pts',(-33.1922409878963,30.4204264438423,41.));
#39234=CARTESIAN_POINT('Ctrl Pts',(-33.1358600523127,30.3715399649794,41.));
#39235=CARTESIAN_POINT('Ctrl Pts',(-33.0937060828269,30.3349893274824,41.));
#39236=CARTESIAN_POINT('Ctrl Pts',(-33.0500910988085,30.3001767875303,41.));
#39237=CARTESIAN_POINT('Ctrl Pts',(-33.0051178417279,30.2672224267123,41.));
#39238=CARTESIAN_POINT('Ctrl Pts',(-32.991033633089,30.2569021581027,41.));
#39239=CARTESIAN_POINT('Ctrl Pts',(-32.9768161196749,30.2467642066019,41.));
#39240=CARTESIAN_POINT('Ctrl Pts',(-32.9624682145604,30.2368124882568,41.));
#39241=CARTESIAN_POINT('Ctrl Pts',(-32.9486861836171,30.2272532606847,41.));
#39242=CARTESIAN_POINT('Ctrl Pts',(-32.9347908994425,30.217870822758,41.));
#39243=CARTESIAN_POINT('Ctrl Pts',(-32.9207902789774,30.2086713607756,41.));
#39244=CARTESIAN_POINT('Ctrl Pts',(-32.8578346023933,30.1673047402921,41.));
#39245=CARTESIAN_POINT('Ctrl Pts',(-32.7927216169288,30.1296140460093,41.));
#39246=CARTESIAN_POINT('Ctrl Pts',(-32.7257126755435,30.095878544712,41.));
#39247=CARTESIAN_POINT('Ctrl Pts',(-32.6745222019714,30.0701068155682,41.));
#39248=CARTESIAN_POINT('Ctrl Pts',(-32.6222242810127,30.046643732657,41.));
#39249=CARTESIAN_POINT('Ctrl Pts',(-32.5689215997279,30.0256290168506,41.));
#39250=CARTESIAN_POINT('Ctrl Pts',(-32.5564364835041,30.0207067284604,41.));
#39251=CARTESIAN_POINT('Ctrl Pts',(-32.5438961977317,30.0159188346434,41.));
#39252=CARTESIAN_POINT('Ctrl Pts',(-32.5313026984106,30.0112647410448,41.));
#39253=CARTESIAN_POINT('Ctrl Pts',(-30.3326930047543,31.9986962112692,42.1285196366098));
#39254=CARTESIAN_POINT('Ctrl Pts',(-30.3319567964985,31.9130463864536,42.1227790551389));
#39255=CARTESIAN_POINT('Ctrl Pts',(-30.3379868569258,31.8275005632038,42.1170384736681));
#39256=CARTESIAN_POINT('Ctrl Pts',(-30.3511440008779,31.7430654121314,42.1112978921973));
#39257=CARTESIAN_POINT('Ctrl Pts',(-30.4360454254438,31.1982158128894,42.074254629124));
#39258=CARTESIAN_POINT('Ctrl Pts',(-30.8177158617989,30.6996141751516,42.0372113660508));
#39259=CARTESIAN_POINT('Ctrl Pts',(-31.32150540483,30.4754087738067,42.0001681029776));
#39260=CARTESIAN_POINT('Ctrl Pts',(-31.8252949478612,30.2512033724617,41.9631248399043));
#39261=CARTESIAN_POINT('Ctrl Pts',(-32.4512035975684,30.3013942075097,41.9260815768311));
#39262=CARTESIAN_POINT('Ctrl Pts',(-32.9128181241709,30.6030322996287,41.8890383137578));
#39263=CARTESIAN_POINT('Ctrl Pts',(-33.3744326507733,30.9046703917478,41.8519950506846));
#39264=CARTESIAN_POINT('Ctrl Pts',(-33.671753054271,31.4577557409379,41.8149517876113));
#39265=CARTESIAN_POINT('Ctrl Pts',(-33.6687287642475,32.009163711811,41.7779085245381));
#39266=CARTESIAN_POINT('Ctrl Pts',(-33.665704474224,32.5605716826841,41.7408652614648));
#39267=CARTESIAN_POINT('Ctrl Pts',(-33.3623354906794,33.1103022752402,41.7038219983916));
#39268=CARTESIAN_POINT('Ctrl Pts',(-32.8974385813771,33.4068725754867,41.6667787353184));
#39269=CARTESIAN_POINT('Ctrl Pts',(-32.4325416720748,33.7034428757333,41.6297354722451));
#39270=CARTESIAN_POINT('Ctrl Pts',(-31.8061168370147,33.7468528836704,41.5926922091719));
#39271=CARTESIAN_POINT('Ctrl Pts',(-31.3048190804959,33.5170982043666,41.5556489460986));
#39272=CARTESIAN_POINT('Ctrl Pts',(-30.803521323977,33.2873435250628,41.5186056830254));
#39273=CARTESIAN_POINT('Ctrl Pts',(-30.4273506459994,32.7844241585182,41.4815624199522));
#39274=CARTESIAN_POINT('Ctrl Pts',(-30.3484281139147,32.238751004344,41.4445191568789));
#39275=CARTESIAN_POINT('Ctrl Pts',(-30.3370655201346,32.1601896325297,41.4391859834559));
#39276=CARTESIAN_POINT('Ctrl Pts',(-30.3318642226577,32.080742069305,41.4338528100328));
#39277=CARTESIAN_POINT('Ctrl Pts',(-30.3325261571163,32.001210199007,41.4285196366098));
#39278=CARTESIAN_POINT('Ctrl Pts',(-31.4698297828114,30.0148256743283,41.));
#39279=CARTESIAN_POINT('Ctrl Pts',(-30.8097602092473,30.1911070339301,41.0370432630732));
#39280=CARTESIAN_POINT('Ctrl Pts',(-29.6907568006176,31.251212957076,41.1111297892197));
#39281=CARTESIAN_POINT('Ctrl Pts',(-30.1186158644953,33.5380364303402,41.2222595784395));
#39282=CARTESIAN_POINT('Ctrl Pts',(-32.2715961695763,34.4127962262488,41.3333893676592));
#39283=CARTESIAN_POINT('Ctrl Pts',(-34.1743722121293,33.0815585185448,41.4445191568789));
#39284=CARTESIAN_POINT('Ctrl Pts',(-34.088014018114,30.7594030715832,41.5556489460986));
#39285=CARTESIAN_POINT('Ctrl Pts',(-32.0903101568642,29.5731769531958,41.6667787353184));
#39286=CARTESIAN_POINT('Ctrl Pts',(-30.0101664816534,30.6076759834516,41.777908524538));
#39287=CARTESIAN_POINT('Ctrl Pts',(-29.7509902552198,32.9165547583188,41.8890383137579));
#39288=CARTESIAN_POINT('Ctrl Pts',(-31.5501372064992,34.3865418916543,42.0001681029775));
#39289=CARTESIAN_POINT('Ctrl Pts',(-33.7609665083167,33.6724274609132,42.1112978921974));
#39290=CARTESIAN_POINT('Ctrl Pts',(-34.3601920973369,31.4277075251964,42.2224276814169));
#39291=CARTESIAN_POINT('Ctrl Pts',(-32.7993885345327,29.7067525630187,42.3335574706368));
#39292=CARTESIAN_POINT('Ctrl Pts',(-30.5069967591677,30.0845481859775,42.4446872598564));
#39293=CARTESIAN_POINT('Ctrl Pts',(-29.5809835883393,32.2153468604003,42.5558170490762));
#39294=CARTESIAN_POINT('Ctrl Pts',(-30.8688288986318,34.1490612499125,42.6669468382959));
#39295=CARTESIAN_POINT('Ctrl Pts',(-33.1919092821327,34.1159786819058,42.7780766275156));
#39296=CARTESIAN_POINT('Ctrl Pts',(-34.4241674445136,32.1463750716222,42.8892064167354));
#39297=CARTESIAN_POINT('Ctrl Pts',(-33.4378537354262,30.0428107344064,43.0003362059551));
#39298=CARTESIAN_POINT('Ctrl Pts',(-31.1356319387654,29.7304447118329,43.1114659951747));
#39299=CARTESIAN_POINT('Ctrl Pts',(-29.6244703886607,31.4951511152756,43.2225957843946));
#39300=CARTESIAN_POINT('Ctrl Pts',(-30.2873677921603,33.7218897236688,43.3337255736142));
#39301=CARTESIAN_POINT('Ctrl Pts',(-32.5176476120498,34.372773539922,43.4448553628341));
#39302=CARTESIAN_POINT('Ctrl Pts',(-34.2741819548352,32.8521207391232,43.5559851520537));
#39303=CARTESIAN_POINT('Ctrl Pts',(-33.9494096331178,30.5516162812554,43.6671149412735));
#39304=CARTESIAN_POINT('Ctrl Pts',(-31.8405587566049,29.5766568944465,43.7782447304931));
#39305=CARTESIAN_POINT('Ctrl Pts',(-29.8776267764906,30.8195148384194,43.889374519713));
#39306=CARTESIAN_POINT('Ctrl Pts',(-29.8570677545995,33.1427400001187,44.0005043089325));
#39307=CARTESIAN_POINT('Ctrl Pts',(-31.7976970844419,34.4201419063721,44.1116340981524));
#39308=CARTESIAN_POINT('Ctrl Pts',(-33.9234718487822,33.4826561851773,44.2227638873721));
#39309=CARTESIAN_POINT('Ctrl Pts',(-34.2889060362689,31.1882596020868,44.3338936765918));
#39310=CARTESIAN_POINT('Ctrl Pts',(-32.5595582415307,29.6367590281872,44.4450234658115));
#39311=CARTESIAN_POINT('Ctrl Pts',(-30.3181088122919,30.2480709634203,44.5561532550313));
#39312=CARTESIAN_POINT('Ctrl Pts',(-29.6159079586973,32.4627293540464,44.6672830442509));
#39313=CARTESIAN_POINT('Ctrl Pts',(-31.0956022868993,34.2539028579429,44.7784128334708));
#39314=CARTESIAN_POINT('Ctrl Pts',(-33.4029915943473,33.9823289088073,44.8895426226903));
#39315=CARTESIAN_POINT('Ctrl Pts',(-34.4263782094584,31.8965490397939,45.0006724119102));
#39316=CARTESIAN_POINT('Ctrl Pts',(-33.2291698002495,29.9054463676817,45.1118022011298));
#39317=CARTESIAN_POINT('Ctrl Pts',(-30.9070385196435,29.8312564653792,45.2229319903496));
#39318=CARTESIAN_POINT('Ctrl Pts',(-29.5851737331861,31.7418771269173,45.3340617795693));
#39319=CARTESIAN_POINT('Ctrl Pts',(-30.4733317584164,33.8887290426746,45.4451915687891));
#39320=CARTESIAN_POINT('Ctrl Pts',(-32.7586800023163,34.3070366209898,45.5563213580088));
#39321=CARTESIAN_POINT('Ctrl Pts',(-34.3496925356383,32.6139693025454,45.6674511472286));
#39322=CARTESIAN_POINT('Ctrl Pts',(-33.7902919416986,30.3590039366313,45.7785809364482));
#39323=CARTESIAN_POINT('Ctrl Pts',(-31.592435577624,29.605860372051,45.889710725668));
#39324=CARTESIAN_POINT('Ctrl Pts',(-29.7675777530558,31.0438074316064,46.0008405148877));
#39325=CARTESIAN_POINT('Ctrl Pts',(-29.9858085592797,33.3568515602791,46.1119703041074));
#39326=CARTESIAN_POINT('Ctrl Pts',(-32.0474055290543,34.4281198554267,46.2231000933271));
#39327=CARTESIAN_POINT('Ctrl Pts',(-34.0656174727299,33.2771991907512,46.3342298825469));
#39328=CARTESIAN_POINT('Ctrl Pts',(-34.1933987060518,30.9573996773486,46.4453596717666));
#39329=CARTESIAN_POINT('Ctrl Pts',(-32.3138052300136,29.5917766727069,46.5564894609864));
#39330=CARTESIAN_POINT('Ctrl Pts',(-30.1470206105429,30.4301335411094,46.667619250206));
#39331=CARTESIAN_POINT('Ctrl Pts',(-29.6760626335787,32.7052151681957,46.7787490394258));
#39332=CARTESIAN_POINT('Ctrl Pts',(-31.3319469323119,34.3348915210894,46.8898788286455));
#39333=CARTESIAN_POINT('Ctrl Pts',(-33.5992261538594,33.8277004747262,47.0010086178653));
#39334=CARTESIAN_POINT('Ctrl Pts',(-34.4029109422803,31.64781777448,47.1121384070849));
#39335=CARTESIAN_POINT('Ctrl Pts',(-33.0074776948103,29.7902484277724,47.2232681963048));
#39336=CARTESIAN_POINT('Ctrl Pts',(-30.6900117866906,29.9550197562096,47.3343979855244));
#39337=CARTESIAN_POINT('Ctrl Pts',(-29.571432885161,31.9913348268765,47.4455277747442));
#39338=CARTESIAN_POINT('Ctrl Pts',(-30.6754522704185,34.0355801700161,47.5566575639638));
#39339=CARTESIAN_POINT('Ctrl Pts',(-32.9916833736669,34.2168846165047,47.6677873531836));
#39340=CARTESIAN_POINT('Ctrl Pts',(-34.4003366076938,32.3693203030807,47.7789171424033));
#39341=CARTESIAN_POINT('Ctrl Pts',(-33.6122278089259,30.1837580533892,47.890046931623));
#39342=CARTESIAN_POINT('Ctrl Pts',(-31.3486256033116,29.6604007369121,48.0011767208428));
#39343=CARTESIAN_POINT('Ctrl Pts',(-29.6811541816853,31.2782192941156,48.1123065100625));
#39344=CARTESIAN_POINT('Ctrl Pts',(-30.1358653061449,33.5566037259586,48.2234362992823));
#39345=CARTESIAN_POINT('Ctrl Pts',(-32.2966122867217,34.4104013084688,48.3345660885019));
#39346=CARTESIAN_POINT('Ctrl Pts',(-34.1859029191172,33.0582257531821,48.4456958777217));
#39347=CARTESIAN_POINT('Ctrl Pts',(-34.0746789050666,30.7375734645635,48.5568256669414));
#39348=CARTESIAN_POINT('Ctrl Pts',(-32.064731256055,29.5722802507307,48.6679554561612));
#39349=CARTESIAN_POINT('Ctrl Pts',(-29.995542263483,30.6288098239048,48.7790852453808));
#39350=CARTESIAN_POINT('Ctrl Pts',(-29.7608112539325,32.940237776303,48.8902150346006));
#39351=CARTESIAN_POINT('Ctrl Pts',(-31.5753615017921,34.3911703122827,49.0013448238203));
#39352=CARTESIAN_POINT('Ctrl Pts',(-33.7785362981989,33.6537297096236,49.1124746130401));
#39353=CARTESIAN_POINT('Ctrl Pts',(-34.354013961917,31.4028136106688,49.2236044022597));
#39354=CARTESIAN_POINT('Ctrl Pts',(-32.7751235759071,29.6984360190133,49.3347341914796));
#39355=CARTESIAN_POINT('Ctrl Pts',(-30.4868484990922,30.1004248233347,49.4458639806991));
#39356=CARTESIAN_POINT('Ctrl Pts',(-29.5833932664634,32.2408842293052,49.556993769919));
#39357=CARTESIAN_POINT('Ctrl Pts',(-30.8915903093585,34.1608890008963,49.6681235591386));
#39358=CARTESIAN_POINT('Ctrl Pts',(-33.2141918809262,34.1032715927325,49.7792533483584));
#39359=CARTESIAN_POINT('Ctrl Pts',(-34.4255782104328,32.1207628319306,49.8903831375781));
#39360=CARTESIAN_POINT('Ctrl Pts',(-33.4171016660518,30.0277332369641,50.0015129267978));
#39361=CARTESIAN_POINT('Ctrl Pts',(-31.1117090447276,29.7397007951857,50.1126427160176));
#39362=CARTESIAN_POINT('Ctrl Pts',(-29.6192706725547,31.5202696737293,50.2237725052373));
#39363=CARTESIAN_POINT('Ctrl Pts',(-30.3056499629249,33.7398825444167,50.334902294457));
#39364=CARTESIAN_POINT('Ctrl Pts',(-32.5426800327657,34.3671737786953,50.4460320836768));
#39365=CARTESIAN_POINT('Ctrl Pts',(-34.2830552217384,32.828053241641,50.5571618728965));
#39366=CARTESIAN_POINT('Ctrl Pts',(-33.9340030304806,30.5311073577035,50.6682916621162));
#39367=CARTESIAN_POINT('Ctrl Pts',(-31.8149722391133,29.5784760905123,50.779421451336));
#39368=CARTESIAN_POINT('Ctrl Pts',(-29.8652768479733,30.8419972449628,50.8905512405557));
#39369=CARTESIAN_POINT('Ctrl Pts',(-29.869256935447,33.1653099627831,51.0016810297754));
#39370=CARTESIAN_POINT('Ctrl Pts',(-31.8232699686781,34.4221436399707,51.1128108189951));
#39371=CARTESIAN_POINT('Ctrl Pts',(-33.9390244099684,33.4622577248198,51.2239406082149));
#39372=CARTESIAN_POINT('Ctrl Pts',(-34.2802047391973,31.1641293976194,51.3350703974346));
#39373=CARTESIAN_POINT('Ctrl Pts',(-32.5345664187102,29.6309807807203,51.4462001866543));
#39374=CARTESIAN_POINT('Ctrl Pts',(-30.2996987093337,30.2659328630714,51.557329975874));
#39375=CARTESIAN_POINT('Ctrl Pts',(-29.6209283014176,32.4878843825608,51.6684597650938));
#39376=CARTESIAN_POINT('Ctrl Pts',(-31.1194585135859,34.2633294087954,51.7795895543135));
#39377=CARTESIAN_POINT('Ctrl Pts',(-33.423850742076,33.9673998993839,51.8907193435332));
#39378=CARTESIAN_POINT('Ctrl Pts',(-34.4251502183154,31.8709273485123,52.001849132753));
#39379=CARTESIAN_POINT('Ctrl Pts',(-33.2069785027727,29.8925806669829,52.1129789219727));
#39380=CARTESIAN_POINT('Ctrl Pts',(-30.8841931736715,29.8429213477129,52.2241087111924));
#39381=CARTESIAN_POINT('Ctrl Pts',(-29.5825821059866,31.7673969339495,52.3352385004122));
#39382=CARTESIAN_POINT('Ctrl Pts',(-30.4933657694112,33.9047484910958,52.4463682896318));
#39383=CARTESIAN_POINT('Ctrl Pts',(-32.7830045631024,34.2988945540426,52.5574980788516));
#39384=CARTESIAN_POINT('Ctrl Pts',(-34.3560464259567,32.5891179074725,52.6686278680713));
#39385=CARTESIAN_POINT('Ctrl Pts',(-33.7728594492291,30.3401856422308,52.7797576572911));
#39386=CARTESIAN_POINT('Ctrl Pts',(-31.5671721178615,29.6103000479543,52.8908874465108));
#39387=CARTESIAN_POINT('Ctrl Pts',(-29.7576014236038,31.0674368452352,53.0020172357304));
#39388=CARTESIAN_POINT('Ctrl Pts',(-30.0002550266955,33.3780554042465,53.1131470249502));
#39389=CARTESIAN_POINT('Ctrl Pts',(-32.0730427769752,34.4274726540847,53.2242768141699));
#39390=CARTESIAN_POINT('Ctrl Pts',(-34.0790038841791,33.2553327473947,53.3354066033897));
#39391=CARTESIAN_POINT('Ctrl Pts',(-34.182240985042,30.9342477393896,53.4465363926094));
#39392=CARTESIAN_POINT('Ctrl Pts',(-32.288398343005,29.5886824305611,53.5576661818291));
#39393=CARTESIAN_POINT('Ctrl Pts',(-30.130451271847,30.4496223583594,53.6687959710488));
#39394=CARTESIAN_POINT('Ctrl Pts',(-29.6838223728037,32.7300579053691,53.7799257602686));
#39395=CARTESIAN_POINT('Ctrl Pts',(-31.3562857209018,34.3411497251595,53.8910555494883));
#39396=CARTESIAN_POINT('Ctrl Pts',(-33.6191545377039,33.8120432967827,54.002185338708));
#39397=CARTESIAN_POINT('Ctrl Pts',(-34.3976274079488,31.6196462144305,54.1133151279277));
#39398=CARTESIAN_POINT('Ctrl Pts',(-33.4572031808897,30.3983372977455,54.1874016540742));
#39399=CARTESIAN_POINT('Ctrl Pts',(-32.8326019491389,30.121497522815,54.2244449171475));
#39400=CARTESIAN_POINT('Ctrl Pts',(-31.5032651029123,30.1400211999972,40.9251850276175));
#39401=CARTESIAN_POINT('Ctrl Pts',(-30.8848229855226,30.3051853306507,40.9622282906908));
#39402=CARTESIAN_POINT('Ctrl Pts',(-29.8363898125428,31.2984354031054,41.0363148168372));
#39403=CARTESIAN_POINT('Ctrl Pts',(-30.2372658353235,33.4410397701959,41.147444606057));
#39404=CARTESIAN_POINT('Ctrl Pts',(-32.2544678878028,34.2606326162469,41.2585743952767));
#39405=CARTESIAN_POINT('Ctrl Pts',(-34.0372448734482,33.0133497544479,41.3697041844965));
#39406=CARTESIAN_POINT('Ctrl Pts',(-33.956332880986,30.8376416336016,41.4808339737161));
#39407=CARTESIAN_POINT('Ctrl Pts',(-32.0846147237652,29.7262251682171,41.5919637629359));
#39408=CARTESIAN_POINT('Ctrl Pts',(-30.1356558404978,30.6954832530194,41.7030935521556));
#39409=CARTESIAN_POINT('Ctrl Pts',(-29.8928246289527,32.8587519984865,41.8142233413753));
#39410=CARTESIAN_POINT('Ctrl Pts',(-31.5785079184226,34.2360340179664,41.9253531305951));
#39411=CARTESIAN_POINT('Ctrl Pts',(-33.6499107058901,33.5669553961153,42.0364829198148));
#39412=CARTESIAN_POINT('Ctrl Pts',(-34.2113459801549,31.4637992962278,42.1476127090345));
#39413=CARTESIAN_POINT('Ctrl Pts',(-32.7489748925163,29.8513767981043,42.2587424982542));
#39414=CARTESIAN_POINT('Ctrl Pts',(-30.6011533897186,30.205346643649,42.3698722874739));
#39415=CARTESIAN_POINT('Ctrl Pts',(-29.7335394759222,32.2017659556705,42.4810020766937));
#39416=CARTESIAN_POINT('Ctrl Pts',(-30.9401664929307,34.0135301535256,42.5921318659134));
#39417=CARTESIAN_POINT('Ctrl Pts',(-33.1167412189572,33.9825339461162,42.7032616551331));
#39418=CARTESIAN_POINT('Ctrl Pts',(-34.2712867057287,32.1371438903604,42.8143914443529));
#39419=CARTESIAN_POINT('Ctrl Pts',(-33.3471751225135,30.1662413751168,42.9255212335726));
#39420=CARTESIAN_POINT('Ctrl Pts',(-31.1901435312227,29.8735747955049,43.0366510227923));
#39421=CARTESIAN_POINT('Ctrl Pts',(-29.7742837700791,31.52698953908,43.1477808120121));
#39422=CARTESIAN_POINT('Ctrl Pts',(-30.3953753795874,33.6132983086424,43.2589106012317));
#39423=CARTESIAN_POINT('Ctrl Pts',(-32.485002033239,34.2231339708512,43.3700403904516));
#39424=CARTESIAN_POINT('Ctrl Pts',(-34.1307600892487,32.7983815271616,43.4811701796711));
#39425=CARTESIAN_POINT('Ctrl Pts',(-33.8264696169156,30.6429589702544,43.5922999688911));
#39426=CARTESIAN_POINT('Ctrl Pts',(-31.8506139593254,29.7294856460844,43.7034297581105));
#39427=CARTESIAN_POINT('Ctrl Pts',(-30.0114747856789,30.8939624365156,43.8145595473305));
#39428=CARTESIAN_POINT('Ctrl Pts',(-29.9922123237522,33.0706728102665,43.92568933655));
#39429=CARTESIAN_POINT('Ctrl Pts',(-31.8104553694601,34.2675150391779,44.0368191257699));
#39430=CARTESIAN_POINT('Ctrl Pts',(-33.8021676055711,33.3891520943329,44.1479489149895));
#39431=CARTESIAN_POINT('Ctrl Pts',(-34.1445555927276,31.2394522175207,44.2590787042094));
#39432=CARTESIAN_POINT('Ctrl Pts',(-32.5242695581717,29.7857974234166,44.370208493429));
#39433=CARTESIAN_POINT('Ctrl Pts',(-30.4241777094362,30.3585568153845,44.4813382826488));
#39434=CARTESIAN_POINT('Ctrl Pts',(-29.7662613319473,32.4335472091974,44.5924680718684));
#39435=CARTESIAN_POINT('Ctrl Pts',(-31.1526383595712,34.1117598987791,44.7035978610883));
#39436=CARTESIAN_POINT('Ctrl Pts',(-33.3145115712621,33.8573128300793,44.8147276503079));
#39437=CARTESIAN_POINT('Ctrl Pts',(-34.2733580482179,31.9030732010106,44.9258574395277));
#39438=CARTESIAN_POINT('Ctrl Pts',(-33.1516518929863,30.0375399272492,45.0369872287473));
#39439=CARTESIAN_POINT('Ctrl Pts',(-30.9759664144383,29.9680288300763,45.1481170179672));
#39440=CARTESIAN_POINT('Ctrl Pts',(-29.7374653682146,31.7581557118077,45.2592468071868));
#39441=CARTESIAN_POINT('Ctrl Pts',(-30.5696114808345,33.7696158634006,45.3703765964066));
#39442=CARTESIAN_POINT('Ctrl Pts',(-32.7108336542772,34.1615427674943,45.4815063856263));
#39443=CARTESIAN_POINT('Ctrl Pts',(-34.2015085759953,32.5752491717323,45.592636174846));
#39444=CARTESIAN_POINT('Ctrl Pts',(-33.677386723329,30.4624937723185,45.7037659640658));
#39445=CARTESIAN_POINT('Ctrl Pts',(-31.6181387319734,29.756847398918,45.8148957532855));
#39446=CARTESIAN_POINT('Ctrl Pts',(-29.9083660320029,31.1041099600508,45.9260255425052));
#39447=CARTESIAN_POINT('Ctrl Pts',(-30.1128340567174,33.2712813702222,46.0371553317249));
#39448=CARTESIAN_POINT('Ctrl Pts',(-32.0444158872617,34.2749898568386,46.1482851209447));
#39449=CARTESIAN_POINT('Ctrl Pts',(-33.9353487794544,33.196652297714,46.2594149101644));
#39450=CARTESIAN_POINT('Ctrl Pts',(-34.0550714566739,31.0231515328753,46.3705446993841));
#39451=CARTESIAN_POINT('Ctrl Pts',(-32.2940150230675,29.7436518916687,46.4816744886039));
#39452=CARTESIAN_POINT('Ctrl Pts',(-30.2638792288098,30.5291375701305,46.5928042778235));
#39453=CARTESIAN_POINT('Ctrl Pts',(-29.8226223368996,32.6607405935701,46.7039340670433));
#39454=CARTESIAN_POINT('Ctrl Pts',(-31.3740778695814,34.1876409912076,46.815063856263));
#39455=CARTESIAN_POINT('Ctrl Pts',(-33.4983705481795,33.7124360776707,46.9261936454827));
#39456=CARTESIAN_POINT('Ctrl Pts',(-34.2513707502356,31.6700282364455,47.0373234347025));
#39457=CARTESIAN_POINT('Ctrl Pts',(-32.9439408567753,29.9296069748306,47.1484532239222));
#39458=CARTESIAN_POINT('Ctrl Pts',(-30.7726265278065,30.0839869573734,47.2595830131419));
#39459=CARTESIAN_POINT('Ctrl Pts',(-29.7245910902782,31.9918812982318,47.3707128023617));
#39460=CARTESIAN_POINT('Ctrl Pts',(-30.7589852111452,33.9072057869049,47.4818425915814));
#39461=CARTESIAN_POINT('Ctrl Pts',(-32.9291426085271,34.0770762221881,47.5929723808011));
#39462=CARTESIAN_POINT('Ctrl Pts',(-34.248958766717,32.3460290238784,47.7041021700208));
#39463=CARTESIAN_POINT('Ctrl Pts',(-33.5105522505498,30.2982998154438,47.8152319592406));
#39464=CARTESIAN_POINT('Ctrl Pts',(-31.3897046959364,29.8079481617449,47.9263617484603));
#39465=CARTESIAN_POINT('Ctrl Pts',(-29.8273927852251,31.3237385786048,48.0374915376801));
#39466=CARTESIAN_POINT('Ctrl Pts',(-30.2534274365316,33.4584361145758,48.1486213268997));
#39467=CARTESIAN_POINT('Ctrl Pts',(-32.2779063571337,34.2583887345682,48.2597511161195));
#39468=CARTESIAN_POINT('Ctrl Pts',(-34.048048393456,32.9914884758897,48.3708809053392));
#39469=CARTESIAN_POINT('Ctrl Pts',(-33.9438387502473,30.8171887163217,48.4820106945589));
#39470=CARTESIAN_POINT('Ctrl Pts',(-32.0606489628658,29.7253850165219,48.5931404837786));
#39471=CARTESIAN_POINT('Ctrl Pts',(-30.1219539023801,30.7152842824289,48.7042702729984));
#39472=CARTESIAN_POINT('Ctrl Pts',(-29.9020262638743,32.8809414408952,48.8154000622181));
#39473=CARTESIAN_POINT('Ctrl Pts',(-31.602141437093,34.2403705460662,48.9265298514378));
#39474=CARTESIAN_POINT('Ctrl Pts',(-33.6663724524877,33.5494368232845,49.0376596406576));
#39475=CARTESIAN_POINT('Ctrl Pts',(-34.2055574704225,31.4404753227754,49.1487894298773));
#39476=CARTESIAN_POINT('Ctrl Pts',(-32.7262402097014,29.8435847390698,49.259919219097));
#39477=CARTESIAN_POINT('Ctrl Pts',(-30.5822757848087,30.2202220168179,49.3710490083167));
#39478=CARTESIAN_POINT('Ctrl Pts',(-29.7357971870802,32.2256928038857,49.4821787975365));
#39479=CARTESIAN_POINT('Ctrl Pts',(-30.9614924494789,34.0246119843739,49.5933085867562));
#39480=CARTESIAN_POINT('Ctrl Pts',(-33.1376185599691,33.9706282327658,49.7044383759759));
#39481=CARTESIAN_POINT('Ctrl Pts',(-34.2726085013351,32.1131468931038,49.8155681651957));
#39482=CARTESIAN_POINT('Ctrl Pts',(-33.3277317876923,30.1521147439001,49.9266979544153));
#39483=CARTESIAN_POINT('Ctrl Pts',(-31.167729340605,29.8822471415979,50.0378277436351));
#39484=CARTESIAN_POINT('Ctrl Pts',(-29.7694119753968,31.550523989232,50.1489575328548));
#39485=CARTESIAN_POINT('Ctrl Pts',(-30.4125045805853,33.6301564075563,50.2600873220745));
#39486=CARTESIAN_POINT('Ctrl Pts',(-32.5084557779517,34.2178873599959,50.3712171112943));
#39487=CARTESIAN_POINT('Ctrl Pts',(-34.1390737613091,32.7758318525526,50.482346900514));
#39488=CARTESIAN_POINT('Ctrl Pts',(-33.8120346356071,30.6237434472022,50.5934766897338));
#39489=CARTESIAN_POINT('Ctrl Pts',(-31.8266410620917,29.7311901140859,50.7046064789534));
#39490=CARTESIAN_POINT('Ctrl Pts',(-29.9999037085566,30.9150269843506,50.8157362681732));
#39491=CARTESIAN_POINT('Ctrl Pts',(-30.0036327907976,33.0918193924733,50.9268660573929));
#39492=CARTESIAN_POINT('Ctrl Pts',(-31.8344154932231,34.2693905329361,51.0379958466127));
#39493=CARTESIAN_POINT('Ctrl Pts',(-33.8167393405155,33.3700400680856,51.1491256358324));
#39494=CARTESIAN_POINT('Ctrl Pts',(-34.1364030451772,31.2168437905586,51.2602554250521));
#39495=CARTESIAN_POINT('Ctrl Pts',(-32.5008538510381,29.7803835826013,51.3713852142718));
#39496=CARTESIAN_POINT('Ctrl Pts',(-30.4069286443211,30.3752922497739,51.4825150034915));
#39497=CARTESIAN_POINT('Ctrl Pts',(-29.7709650654724,32.4571158294164,51.5936447927113));
#39498=CARTESIAN_POINT('Ctrl Pts',(-31.1749900872312,34.1205919617954,51.704774581931));
#39499=CARTESIAN_POINT('Ctrl Pts',(-33.334055231514,33.8433253224467,51.8159043711508));
#39500=CARTESIAN_POINT('Ctrl Pts',(-34.2722075006498,31.879067348231,51.9270341603704));
#39501=CARTESIAN_POINT('Ctrl Pts',(-33.1308600953504,30.0254856052496,52.0381639495902));
#39502=CARTESIAN_POINT('Ctrl Pts',(-30.9545618160425,29.9789580636276,52.1492937388099));
#39503=CARTESIAN_POINT('Ctrl Pts',(-29.735037182646,31.7820661056942,52.2604235280297));
#39504=CARTESIAN_POINT('Ctrl Pts',(-30.5883820418111,33.7846250412173,52.3715533172493));
#39505=CARTESIAN_POINT('Ctrl Pts',(-32.733624180427,34.1539141820779,52.4826831064691));
#39506=CARTESIAN_POINT('Ctrl Pts',(-34.2074617565987,32.5519650362343,52.5938128956888));
#39507=CARTESIAN_POINT('Ctrl Pts',(-33.6610536154475,30.4448622584587,52.7049426849085));
#39508=CARTESIAN_POINT('Ctrl Pts',(-31.5944685187508,29.761007085527,52.8160724741283));
#39509=CARTESIAN_POINT('Ctrl Pts',(-29.8990188623148,31.1262491786764,52.927202263348));
#39510=CARTESIAN_POINT('Ctrl Pts',(-30.1263694539774,33.2911479883563,53.0383320525678));
#39511=CARTESIAN_POINT('Ctrl Pts',(-32.0684363155972,34.2743834714144,53.1494618417874));
#39512=CARTESIAN_POINT('Ctrl Pts',(-33.9478909734479,33.1761648671903,53.2605916310072));
#39513=CARTESIAN_POINT('Ctrl Pts',(-34.0446174001881,31.0014596777944,53.3717214202269));
#39514=CARTESIAN_POINT('Ctrl Pts',(-32.2702104278746,29.7407527886938,53.4828512094466));
#39515=CARTESIAN_POINT('Ctrl Pts',(-30.2483548396889,30.5473973201451,53.5939809986664));
#39516=CARTESIAN_POINT('Ctrl Pts',(-29.8298927061893,32.6840166171813,53.705110787886));
#39517=CARTESIAN_POINT('Ctrl Pts',(-31.3968817262552,34.1935045200403,53.8162405771059));
#39518=CARTESIAN_POINT('Ctrl Pts',(-33.517042143409,33.6977663236515,53.9273703663255));
#39519=CARTESIAN_POINT('Ctrl Pts',(-34.2464204233457,31.6436333230227,54.0385001555453));
#39520=CARTESIAN_POINT('Ctrl Pts',(-33.3653042902589,30.4993465649721,54.1125866816917));
#39521=CARTESIAN_POINT('Ctrl Pts',(-32.7800936946509,30.2399657611256,54.149629944765));
#39522=CARTESIAN_POINT('Ctrl Pts',(-31.5367004230132,30.2652167256662,40.850370055235));
#39523=CARTESIAN_POINT('Ctrl Pts',(-30.9598857617979,30.4192636273712,40.8874133183083));
#39524=CARTESIAN_POINT('Ctrl Pts',(-29.9820228244681,31.3456578491348,40.9614998444547));
#39525=CARTESIAN_POINT('Ctrl Pts',(-30.3559158061516,33.3440431100515,41.0726296336745));
#39526=CARTESIAN_POINT('Ctrl Pts',(-32.2373396060292,34.108469006245,41.1837594228942));
#39527=CARTESIAN_POINT('Ctrl Pts',(-33.900117534767,32.945140990351,41.2948892121139));
#39528=CARTESIAN_POINT('Ctrl Pts',(-33.8246517438579,30.91588019562,41.4060190013336));
#39529=CARTESIAN_POINT('Ctrl Pts',(-32.0789192906661,29.8792733832384,41.5171487905534));
#39530=CARTESIAN_POINT('Ctrl Pts',(-30.2611451993424,30.7832905225872,41.6282785797731));
#39531=CARTESIAN_POINT('Ctrl Pts',(-30.0346590026857,32.8009492386541,41.7394083689928));
#39532=CARTESIAN_POINT('Ctrl Pts',(-31.6068786303459,34.0855261442786,41.8505381582125));
#39533=CARTESIAN_POINT('Ctrl Pts',(-33.5388549034635,33.4614833313175,41.9616679474323));
#39534=CARTESIAN_POINT('Ctrl Pts',(-34.0624998629728,31.4998910672591,42.072797736652));
#39535=CARTESIAN_POINT('Ctrl Pts',(-32.6985612504999,29.9960010331899,42.1839275258717));
#39536=CARTESIAN_POINT('Ctrl Pts',(-30.6953100202696,30.3261451013204,42.2950573150915));
#39537=CARTESIAN_POINT('Ctrl Pts',(-29.8860953635051,32.1881850509407,42.4061871043112));
#39538=CARTESIAN_POINT('Ctrl Pts',(-31.0115040872296,33.8779990571385,42.5173168935309));
#39539=CARTESIAN_POINT('Ctrl Pts',(-33.0415731557818,33.8490892103266,42.6284466827506));
#39540=CARTESIAN_POINT('Ctrl Pts',(-34.1184059669438,32.1279127090986,42.7395764719704));
#39541=CARTESIAN_POINT('Ctrl Pts',(-33.2564965096008,30.2896720158273,42.8507062611901));
#39542=CARTESIAN_POINT('Ctrl Pts',(-31.24465512368,30.0167048791768,42.9618360504098));
#39543=CARTESIAN_POINT('Ctrl Pts',(-29.9240971514974,31.5588279628845,43.0729658396296));
#39544=CARTESIAN_POINT('Ctrl Pts',(-30.5033829670146,33.5047068936161,43.1840956288493));
#39545=CARTESIAN_POINT('Ctrl Pts',(-32.4523564544282,34.0734944017804,43.295225418069));
#39546=CARTESIAN_POINT('Ctrl Pts',(-33.9873382236621,32.7446423152,43.4063552072887));
#39547=CARTESIAN_POINT('Ctrl Pts',(-33.7035296007133,30.7343016592533,43.5174849965085));
#39548=CARTESIAN_POINT('Ctrl Pts',(-31.8606691620459,29.8823143977223,43.6286147857282));
#39549=CARTESIAN_POINT('Ctrl Pts',(-30.1453227948673,30.9684100346118,43.739744574948));
#39550=CARTESIAN_POINT('Ctrl Pts',(-30.1273568929049,32.9986056204144,43.8508743641676));
#39551=CARTESIAN_POINT('Ctrl Pts',(-31.8232136544782,34.1148881719836,43.9620041533874));
#39552=CARTESIAN_POINT('Ctrl Pts',(-33.68086336236,33.2956480034885,44.073133942607));
#39553=CARTESIAN_POINT('Ctrl Pts',(-34.0002051491863,31.2906448329547,44.1842637318269));
#39554=CARTESIAN_POINT('Ctrl Pts',(-32.4889808748128,29.9348358186458,44.2953935210465));
#39555=CARTESIAN_POINT('Ctrl Pts',(-30.5302466065805,30.4690426673488,44.4065233102663));
#39556=CARTESIAN_POINT('Ctrl Pts',(-29.9166147051972,32.4043650643483,44.5176530994859));
#39557=CARTESIAN_POINT('Ctrl Pts',(-31.2096744322432,33.9696169396154,44.6287828887058));
#39558=CARTESIAN_POINT('Ctrl Pts',(-33.226031548177,33.7322967513513,44.7399126779253));
#39559=CARTESIAN_POINT('Ctrl Pts',(-34.1203378869774,31.9095973622274,44.8510424671453));
#39560=CARTESIAN_POINT('Ctrl Pts',(-33.0741339857231,30.1696334868166,44.9621722563649));
#39561=CARTESIAN_POINT('Ctrl Pts',(-31.0448943092331,30.1048011947734,45.0733020455846));
#39562=CARTESIAN_POINT('Ctrl Pts',(-29.889757003243,31.7744342966981,45.1844318348044));
#39563=CARTESIAN_POINT('Ctrl Pts',(-30.6658912032526,33.6505026841267,45.2955616240241));
#39564=CARTESIAN_POINT('Ctrl Pts',(-32.662987306238,34.0160489139987,45.4066914132438));
#39565=CARTESIAN_POINT('Ctrl Pts',(-34.0533246163523,32.5365290409192,45.5178212024636));
#39566=CARTESIAN_POINT('Ctrl Pts',(-33.5644815049592,30.5659836080057,45.6289509916833));
#39567=CARTESIAN_POINT('Ctrl Pts',(-31.643841886323,29.907834425785,45.740080780903));
#39568=CARTESIAN_POINT('Ctrl Pts',(-30.0491543109499,31.1644124884951,45.8512105701227));
#39569=CARTESIAN_POINT('Ctrl Pts',(-30.2398595541551,33.1857111801652,45.9623403593424));
#39570=CARTESIAN_POINT('Ctrl Pts',(-32.0414262454691,34.1218598582504,46.0734701485622));
#39571=CARTESIAN_POINT('Ctrl Pts',(-33.8050800861789,33.1161054046768,46.1845999377819));
#39572=CARTESIAN_POINT('Ctrl Pts',(-33.916744207296,31.0889033884021,46.2957297270016));
#39573=CARTESIAN_POINT('Ctrl Pts',(-32.2742248161213,29.8955271106305,46.4068595162214));
#39574=CARTESIAN_POINT('Ctrl Pts',(-30.3807378470766,30.6281415991517,46.5179893054411));
#39575=CARTESIAN_POINT('Ctrl Pts',(-29.9691820402206,32.6162660189444,46.6291190946608));
#39576=CARTESIAN_POINT('Ctrl Pts',(-31.416208806851,34.0403904613259,46.7402488838805));
#39577=CARTESIAN_POINT('Ctrl Pts',(-33.3975149424995,33.5971716806151,46.8513786731002));
#39578=CARTESIAN_POINT('Ctrl Pts',(-34.0998305581909,31.692238698411,46.96250846232));
#39579=CARTESIAN_POINT('Ctrl Pts',(-32.8804040187402,30.0689655218888,47.0736382515397));
#39580=CARTESIAN_POINT('Ctrl Pts',(-30.8552412689225,30.2129541585371,47.1847680407594));
#39581=CARTESIAN_POINT('Ctrl Pts',(-29.8777492953954,31.9924277695871,47.2958978299792));
#39582=CARTESIAN_POINT('Ctrl Pts',(-30.842518151872,33.7788314037936,47.4070276191988));
#39583=CARTESIAN_POINT('Ctrl Pts',(-32.8666018433873,33.9372678278714,47.5181574084187));
#39584=CARTESIAN_POINT('Ctrl Pts',(-34.0975809257403,32.3227377446762,47.6292871976383));
#39585=CARTESIAN_POINT('Ctrl Pts',(-33.4088766921736,30.4128415774984,47.7404169868581));
#39586=CARTESIAN_POINT('Ctrl Pts',(-31.4307837885612,29.9554955865777,47.8515467760778));
#39587=CARTESIAN_POINT('Ctrl Pts',(-29.9736313887648,31.369257863094,47.9626765652975));
#39588=CARTESIAN_POINT('Ctrl Pts',(-30.3709895669183,33.360268503193,48.0738063545173));
#39589=CARTESIAN_POINT('Ctrl Pts',(-32.2592004275456,34.1063761606675,48.1849361437369));
#39590=CARTESIAN_POINT('Ctrl Pts',(-33.9101938677949,32.9247511985973,48.2960659329567));
#39591=CARTESIAN_POINT('Ctrl Pts',(-33.8129985954281,30.89680396808,48.4071957221764));
#39592=CARTESIAN_POINT('Ctrl Pts',(-32.0565666696766,29.8784897823131,48.5183255113962));
#39593=CARTESIAN_POINT('Ctrl Pts',(-30.2483655412771,30.801758740953,48.6294553006159));
#39594=CARTESIAN_POINT('Ctrl Pts',(-30.0432412738161,32.8216451054873,48.7405850898357));
#39595=CARTESIAN_POINT('Ctrl Pts',(-31.6289213723938,34.0895707798498,48.8517148790553));
#39596=CARTESIAN_POINT('Ctrl Pts',(-33.5542086067766,33.4451439369453,48.9628446682751));
#39597=CARTESIAN_POINT('Ctrl Pts',(-34.0571009789279,31.4781370348818,49.0739744574948));
#39598=CARTESIAN_POINT('Ctrl Pts',(-32.6773568434957,29.9887334591264,49.1851042467145));
#39599=CARTESIAN_POINT('Ctrl Pts',(-30.6777030705251,30.340019210301,49.2962340359342));
#39600=CARTESIAN_POINT('Ctrl Pts',(-29.8882011076971,32.2105013784662,49.407363825154));
#39601=CARTESIAN_POINT('Ctrl Pts',(-31.0313945895992,33.8883349678514,49.5184936143736));
#39602=CARTESIAN_POINT('Ctrl Pts',(-33.0610452390119,33.8379848727991,49.6296234035935));
#39603=CARTESIAN_POINT('Ctrl Pts',(-34.1196387922374,32.105530954277,49.7407531928131));
#39604=CARTESIAN_POINT('Ctrl Pts',(-33.2383619093327,30.2764962508361,49.8518829820329));
#39605=CARTESIAN_POINT('Ctrl Pts',(-31.2237496364824,30.0247934880102,49.9630127712526));
#39606=CARTESIAN_POINT('Ctrl Pts',(-29.9195532782388,31.5807783047347,50.0741425604724));
#39607=CARTESIAN_POINT('Ctrl Pts',(-30.5193591982457,33.5204302706958,50.185272349692));
#39608=CARTESIAN_POINT('Ctrl Pts',(-32.4742315231376,34.0686009412964,50.2964021389119));
#39609=CARTESIAN_POINT('Ctrl Pts',(-33.9950923008799,32.7236104634643,50.4075319281315));
#39610=CARTESIAN_POINT('Ctrl Pts',(-33.6900662407335,30.716379536701,50.5186617173513));
#39611=CARTESIAN_POINT('Ctrl Pts',(-31.8383098850701,29.8839041376594,50.6297915065709));
#39612=CARTESIAN_POINT('Ctrl Pts',(-30.1345305691399,30.9880567237383,50.7409212957907));
#39613=CARTESIAN_POINT('Ctrl Pts',(-30.1380086461482,33.0183288221635,50.8520510850104));
#39614=CARTESIAN_POINT('Ctrl Pts',(-31.8455610177681,34.1166374259014,50.9631808742302));
#39615=CARTESIAN_POINT('Ctrl Pts',(-33.6944542710625,33.2778224113514,51.0743106634499));
#39616=CARTESIAN_POINT('Ctrl Pts',(-33.9926013511572,31.2695581834978,51.1854404526696));
#39617=CARTESIAN_POINT('Ctrl Pts',(-32.4671412833658,29.9297863844823,51.2965702418893));
#39618=CARTESIAN_POINT('Ctrl Pts',(-30.5141585793086,30.4846516364765,51.4077000311091));
#39619=CARTESIAN_POINT('Ctrl Pts',(-29.921001829527,32.426347276272,51.5188298203287));
#39620=CARTESIAN_POINT('Ctrl Pts',(-31.2305216608766,33.9778545147955,51.6299596095485));
#39621=CARTESIAN_POINT('Ctrl Pts',(-33.2442597209519,33.7192507455094,51.7410893987682));
#39622=CARTESIAN_POINT('Ctrl Pts',(-34.1192647829842,31.8872073479497,51.8522191879879));
#39623=CARTESIAN_POINT('Ctrl Pts',(-33.0547416879281,30.1583905435162,51.9633489772077));
#39624=CARTESIAN_POINT('Ctrl Pts',(-31.0249304584134,30.1149947795421,52.0744787664274));
#39625=CARTESIAN_POINT('Ctrl Pts',(-29.8874922593055,31.7967352774389,52.1856085556472));
#39626=CARTESIAN_POINT('Ctrl Pts',(-30.6833983142111,33.6645015913388,52.2967383448669));
#39627=CARTESIAN_POINT('Ctrl Pts',(-32.6842437977518,34.0089338101131,52.4078681340866));
#39628=CARTESIAN_POINT('Ctrl Pts',(-34.0588770872406,32.5148121649961,52.5189979233063));
#39629=CARTESIAN_POINT('Ctrl Pts',(-33.549247781666,30.5495388746866,52.6301277125261));
#39630=CARTESIAN_POINT('Ctrl Pts',(-31.62176491964,29.9117141230998,52.7412575017458));
#39631=CARTESIAN_POINT('Ctrl Pts',(-30.0404363010257,31.1850615121176,52.8523872909655));
#39632=CARTESIAN_POINT('Ctrl Pts',(-30.2524838812592,33.2042405724662,52.9635170801852));
#39633=CARTESIAN_POINT('Ctrl Pts',(-32.0638298542192,34.1212942887441,53.074646869405));
#39634=CARTESIAN_POINT('Ctrl Pts',(-33.8167780627168,33.0969969869859,53.1857766586247));
#39635=CARTESIAN_POINT('Ctrl Pts',(-33.9069938153344,31.0686716161993,53.2969064478444));
#39636=CARTESIAN_POINT('Ctrl Pts',(-32.252022512744,29.8928231468264,53.4080362370641));
#39637=CARTESIAN_POINT('Ctrl Pts',(-30.3662584075308,30.6451722819308,53.5191660262839));
#39638=CARTESIAN_POINT('Ctrl Pts',(-29.975963039575,32.6379753289934,53.6302958155036));
#39639=CARTESIAN_POINT('Ctrl Pts',(-31.4374777316085,34.0458593149211,53.7414256047233));
#39640=CARTESIAN_POINT('Ctrl Pts',(-33.4149297491141,33.5834893505202,53.8525553939431));
#39641=CARTESIAN_POINT('Ctrl Pts',(-34.0952134387425,31.6676204316151,53.9636851831627));
#39642=CARTESIAN_POINT('Ctrl Pts',(-33.2734053996281,30.6003558321987,54.0377717093093));
#39643=CARTESIAN_POINT('Ctrl Pts',(-32.7275854401629,30.3584339994361,54.0748149723825));
#39644=CARTESIAN_POINT('Ctrl Pts',(-31.5701357431141,30.3904122513352,40.7755550828525));
#39645=CARTESIAN_POINT('Ctrl Pts',(-31.0349485380732,30.5333419240918,40.8125983459258));
#39646=CARTESIAN_POINT('Ctrl Pts',(-30.1276558363932,31.3928802951642,40.8866848720723));
#39647=CARTESIAN_POINT('Ctrl Pts',(-30.4745657769798,33.2470464499072,40.997814661292));
#39648=CARTESIAN_POINT('Ctrl Pts',(-32.2202113242556,33.9563053962431,41.1089444505117));
#39649=CARTESIAN_POINT('Ctrl Pts',(-33.7629901960859,32.8769322262541,41.2200742397314));
#39650=CARTESIAN_POINT('Ctrl Pts',(-33.6929706067298,30.9941187576385,41.3312040289512));
#39651=CARTESIAN_POINT('Ctrl Pts',(-32.073223857567,30.0323215982597,41.4423338181709));
#39652=CARTESIAN_POINT('Ctrl Pts',(-30.3866345581869,30.871097792155,41.5534636073906));
#39653=CARTESIAN_POINT('Ctrl Pts',(-30.1764933764186,32.7431464788218,41.6645933966103));
#39654=CARTESIAN_POINT('Ctrl Pts',(-31.6352493422693,33.9350182705907,41.7757231858301));
#39655=CARTESIAN_POINT('Ctrl Pts',(-33.4277991010369,33.3560112665197,41.8868529750498));
#39656=CARTESIAN_POINT('Ctrl Pts',(-33.9136537457907,31.5359828382904,41.9979827642695));
#39657=CARTESIAN_POINT('Ctrl Pts',(-32.6481476084835,30.1406252682755,42.1091125534893));
#39658=CARTESIAN_POINT('Ctrl Pts',(-30.7894666508205,30.4469435589918,42.2202423427089));
#39659=CARTESIAN_POINT('Ctrl Pts',(-30.0386512510881,32.174604146211,42.3313721319287));
#39660=CARTESIAN_POINT('Ctrl Pts',(-31.0828416815284,33.7424679607515,42.4425019211484));
#39661=CARTESIAN_POINT('Ctrl Pts',(-32.9664050926064,33.7156444745371,42.5536317103681));
#39662=CARTESIAN_POINT('Ctrl Pts',(-33.965525228159,32.1186815278368,42.6647614995879));
#39663=CARTESIAN_POINT('Ctrl Pts',(-33.1658178966882,30.4131026565378,42.7758912888076));
#39664=CARTESIAN_POINT('Ctrl Pts',(-31.2991667161373,30.1598349628488,42.8870210780273));
#39665=CARTESIAN_POINT('Ctrl Pts',(-30.0739105329158,31.590666386689,42.9981508672471));
#39666=CARTESIAN_POINT('Ctrl Pts',(-30.6113905544417,33.3961154785897,43.1092806564667));
#39667=CARTESIAN_POINT('Ctrl Pts',(-32.4197108756174,33.9238548327095,43.2204104456866));
#39668=CARTESIAN_POINT('Ctrl Pts',(-33.8439163580755,32.6909031032385,43.3315402349062));
#39669=CARTESIAN_POINT('Ctrl Pts',(-33.5805895845112,30.8256443482523,43.442670024126));
#39670=CARTESIAN_POINT('Ctrl Pts',(-31.8707243647664,30.0351431493602,43.5537998133457));
#39671=CARTESIAN_POINT('Ctrl Pts',(-30.2791708040556,31.042857632708,43.6649296025655));
#39672=CARTESIAN_POINT('Ctrl Pts',(-30.2625014620576,32.9265384305622,43.7760593917851));
#39673=CARTESIAN_POINT('Ctrl Pts',(-31.8359719394964,33.9622613047893,43.8871891810049));
#39674=CARTESIAN_POINT('Ctrl Pts',(-33.5595591191489,33.2021439126441,43.9983189702245));
#39675=CARTESIAN_POINT('Ctrl Pts',(-33.855854705645,31.3418374483886,44.1094487594444));
#39676=CARTESIAN_POINT('Ctrl Pts',(-32.453692191454,30.0838742138751,44.220578548664));
#39677=CARTESIAN_POINT('Ctrl Pts',(-30.6363155037247,30.5795285193129,44.3317083378839));
#39678=CARTESIAN_POINT('Ctrl Pts',(-30.0669680784473,32.3751829194994,44.4428381271034));
#39679=CARTESIAN_POINT('Ctrl Pts',(-31.266710504915,33.8274739804516,44.5539679163233));
#39680=CARTESIAN_POINT('Ctrl Pts',(-33.1375515250919,33.6072806726234,44.6650977055429));
#39681=CARTESIAN_POINT('Ctrl Pts',(-33.9673177257368,31.916121523444,44.7762274947628));
#39682=CARTESIAN_POINT('Ctrl Pts',(-32.99661607846,30.3017270463841,44.8873572839823));
#39683=CARTESIAN_POINT('Ctrl Pts',(-31.1138222040278,30.2415735594704,44.9984870732022));
#39684=CARTESIAN_POINT('Ctrl Pts',(-30.0420486382714,31.7907128815886,45.1096168624219));
#39685=CARTESIAN_POINT('Ctrl Pts',(-30.7621709256707,33.5313895048526,45.2207466516415));
#39686=CARTESIAN_POINT('Ctrl Pts',(-32.6151409581988,33.8705550605032,45.3318764408614));
#39687=CARTESIAN_POINT('Ctrl Pts',(-33.9051406567093,32.4978089101062,45.443006230081));
#39688=CARTESIAN_POINT('Ctrl Pts',(-33.4515762865896,30.6694734436928,45.5541360193008));
#39689=CARTESIAN_POINT('Ctrl Pts',(-31.6695450406724,30.0588214526521,45.6652658085205));
#39690=CARTESIAN_POINT('Ctrl Pts',(-30.189942589897,31.2247150169395,45.7763955977402));
#39691=CARTESIAN_POINT('Ctrl Pts',(-30.3668850515927,33.1001409901083,45.88752538696));
#39692=CARTESIAN_POINT('Ctrl Pts',(-32.0384366036765,33.9687298596622,45.9986551761797));
#39693=CARTESIAN_POINT('Ctrl Pts',(-33.6748113929033,33.0355585116396,46.1097849653994));
#39694=CARTESIAN_POINT('Ctrl Pts',(-33.7784169579181,31.1546552439288,46.2209147546192));
#39695=CARTESIAN_POINT('Ctrl Pts',(-32.2544346091752,30.0474023295923,46.3320445438389));
#39696=CARTESIAN_POINT('Ctrl Pts',(-30.4975964653435,30.7271456281728,46.4431743330586));
#39697=CARTESIAN_POINT('Ctrl Pts',(-30.1157417435415,32.5717914443188,46.5543041222783));
#39698=CARTESIAN_POINT('Ctrl Pts',(-31.4583397441205,33.8931399314442,46.665433911498));
#39699=CARTESIAN_POINT('Ctrl Pts',(-33.2966593368194,33.4819072835595,46.7765637007178));
#39700=CARTESIAN_POINT('Ctrl Pts',(-33.9482903661463,31.7144491603765,46.8876934899375));
#39701=CARTESIAN_POINT('Ctrl Pts',(-32.8168671807052,30.208324068947,46.9988232791572));
#39702=CARTESIAN_POINT('Ctrl Pts',(-30.9378560100384,30.3419213597008,47.109953068377));
#39703=CARTESIAN_POINT('Ctrl Pts',(-30.0309075005126,31.9929742409423,47.2210828575967));
#39704=CARTESIAN_POINT('Ctrl Pts',(-30.9260510925986,33.6504570206823,47.3322126468164));
#39705=CARTESIAN_POINT('Ctrl Pts',(-32.8040610782476,33.7974594335549,47.4433424360362));
#39706=CARTESIAN_POINT('Ctrl Pts',(-33.9462030847635,32.2994464654739,47.5544722252558));
#39707=CARTESIAN_POINT('Ctrl Pts',(-33.3072011337976,30.5273833395529,47.6656020144756));
#39708=CARTESIAN_POINT('Ctrl Pts',(-31.471862881186,30.1030430114104,47.7767318036953));
#39709=CARTESIAN_POINT('Ctrl Pts',(-30.1198699923045,31.4147771475832,47.887861592915));
#39710=CARTESIAN_POINT('Ctrl Pts',(-30.488551697305,33.2621008918102,47.9989913821348));
#39711=CARTESIAN_POINT('Ctrl Pts',(-32.2404944979576,33.9543635867668,48.1101211713545));
#39712=CARTESIAN_POINT('Ctrl Pts',(-33.7723393421336,32.8580139213049,48.2212509605742));
#39713=CARTESIAN_POINT('Ctrl Pts',(-33.6821584406089,30.9764192198383,48.332380749794));
#39714=CARTESIAN_POINT('Ctrl Pts',(-32.0524843764874,30.0315945481044,48.4435105390137));
#39715=CARTESIAN_POINT('Ctrl Pts',(-30.3747771801741,30.888233199477,48.5546403282334));
#39716=CARTESIAN_POINT('Ctrl Pts',(-30.1844562837579,32.7623487700795,48.6657701174531));
#39717=CARTESIAN_POINT('Ctrl Pts',(-31.6557013076947,33.9387710136333,48.7768999066728));
#39718=CARTESIAN_POINT('Ctrl Pts',(-33.4420447610655,33.3408510506062,48.8880296958927));
#39719=CARTESIAN_POINT('Ctrl Pts',(-33.9086444874334,31.5157987469883,48.9991594851123));
#39720=CARTESIAN_POINT('Ctrl Pts',(-32.6284734772899,30.1338821791829,49.110289274332));
#39721=CARTESIAN_POINT('Ctrl Pts',(-30.7731303562417,30.4598164037842,49.2214190635518));
#39722=CARTESIAN_POINT('Ctrl Pts',(-30.0406050283139,32.1953099530466,49.3325488527715));
#39723=CARTESIAN_POINT('Ctrl Pts',(-31.1012967297195,33.752057951329,49.4436786419912));
#39724=CARTESIAN_POINT('Ctrl Pts',(-32.9844719180548,33.7053415128324,49.5548084312109));
#39725=CARTESIAN_POINT('Ctrl Pts',(-33.9666690831396,32.0979150154502,49.6659382204306));
#39726=CARTESIAN_POINT('Ctrl Pts',(-33.1489920309732,30.4008777577721,49.7770680096504));
#39727=CARTESIAN_POINT('Ctrl Pts',(-31.2797699323598,30.1673398344224,49.8881977988701));
#39728=CARTESIAN_POINT('Ctrl Pts',(-30.0696945810809,31.6110326202375,49.9993275880899));
#39729=CARTESIAN_POINT('Ctrl Pts',(-30.6262138159061,33.4107041338354,50.1104573773096));
#39730=CARTESIAN_POINT('Ctrl Pts',(-32.4400072683235,33.9193145225971,50.2215871665293));
#39731=CARTESIAN_POINT('Ctrl Pts',(-33.8511108404508,32.6713890743759,50.332716955749));
#39732=CARTESIAN_POINT('Ctrl Pts',(-33.5680978458599,30.8090156261998,50.4438467449687));
#39733=CARTESIAN_POINT('Ctrl Pts',(-31.8499787080486,30.036618161233,50.5549765341885));
#39734=CARTESIAN_POINT('Ctrl Pts',(-30.2691574297231,31.061086463126,50.6661063234082));
#39735=CARTESIAN_POINT('Ctrl Pts',(-30.2723845014988,32.9448382518538,50.777236112628));
#39736=CARTESIAN_POINT('Ctrl Pts',(-31.8567065423131,33.9638843188666,50.8883659018476));
#39737=CARTESIAN_POINT('Ctrl Pts',(-33.5721692016096,33.1856047546172,50.9994956910675));
#39738=CARTESIAN_POINT('Ctrl Pts',(-33.8487996571372,31.322272576437,51.110625480287));
#39739=CARTESIAN_POINT('Ctrl Pts',(-32.4334287156935,30.0791891863634,51.2217552695069));
#39740=CARTESIAN_POINT('Ctrl Pts',(-30.6213885142961,30.594011023179,51.3328850587265));
#39741=CARTESIAN_POINT('Ctrl Pts',(-30.0710385935816,32.3955787231275,51.4440148479463));
#39742=CARTESIAN_POINT('Ctrl Pts',(-31.286053234522,33.8351170677957,51.555144637166));
#39743=CARTESIAN_POINT('Ctrl Pts',(-33.1544642103899,33.5951761685721,51.6662744263858));
#39744=CARTESIAN_POINT('Ctrl Pts',(-33.9663220653187,31.8953473476683,51.7774042156054));
#39745=CARTESIAN_POINT('Ctrl Pts',(-32.9786232805058,30.291295481783,51.8885340048253));
#39746=CARTESIAN_POINT('Ctrl Pts',(-31.0952991007844,30.2510314954568,51.9996637940449));
#39747=CARTESIAN_POINT('Ctrl Pts',(-30.0399473359648,31.8114044491835,52.1107935832646));
#39748=CARTESIAN_POINT('Ctrl Pts',(-30.778414586611,33.5443781414603,52.2219233724844));
#39749=CARTESIAN_POINT('Ctrl Pts',(-32.6348634150766,33.8639534381483,52.3330531617041));
#39750=CARTESIAN_POINT('Ctrl Pts',(-33.9102924178824,32.4776592937579,52.4441829509238));
#39751=CARTESIAN_POINT('Ctrl Pts',(-33.4374419478845,30.6542154909145,52.5553127401436));
#39752=CARTESIAN_POINT('Ctrl Pts',(-31.6490613205292,30.0624211606725,52.6664425293633));
#39753=CARTESIAN_POINT('Ctrl Pts',(-30.1818537397367,31.2438738455587,52.777572318583));
#39754=CARTESIAN_POINT('Ctrl Pts',(-30.378598308541,33.1173331565761,52.8887021078027));
#39755=CARTESIAN_POINT('Ctrl Pts',(-32.0592233928413,33.9682051060738,52.9998318970225));
#39756=CARTESIAN_POINT('Ctrl Pts',(-33.6856651519856,33.0178291067816,53.1109616862421));
#39757=CARTESIAN_POINT('Ctrl Pts',(-33.7693702304806,31.1358835546042,53.222091475462));
#39758=CARTESIAN_POINT('Ctrl Pts',(-32.2338345976135,30.0448935049591,53.3332212646815));
#39759=CARTESIAN_POINT('Ctrl Pts',(-30.4841619753727,30.7429472437166,53.4443510539014));
#39760=CARTESIAN_POINT('Ctrl Pts',(-30.1220333729607,32.5919340408055,53.555480843121));
#39761=CARTESIAN_POINT('Ctrl Pts',(-31.4780737369618,33.898214109802,53.6666106323408));
#39762=CARTESIAN_POINT('Ctrl Pts',(-33.3128173548192,33.469212377389,53.7777404215606));
#39763=CARTESIAN_POINT('Ctrl Pts',(-33.9440064541393,31.6916075402074,53.8888702107803));
#39764=CARTESIAN_POINT('Ctrl Pts',(-33.1815065089974,30.7013650994253,53.9629567369268));
#39765=CARTESIAN_POINT('Ctrl Pts',(-32.6750771856749,30.4769022377466,54.));
#39766=CARTESIAN_POINT('Ctrl Pts',(-30.3361589164137,32.0009454232939,41.6214803633902));
#39767=CARTESIAN_POINT('Ctrl Pts',(-30.3350387322945,32.2165036755626,41.6358513744636));
#39768=CARTESIAN_POINT('Ctrl Pts',(-30.3739091166134,32.4316746076715,41.6502223855369));
#39769=CARTESIAN_POINT('Ctrl Pts',(-30.4546429010218,32.6297836630055,41.6645933966103));
#39770=CARTESIAN_POINT('Ctrl Pts',(-30.6627453650355,33.1404370760781,41.7016366596836));
#39771=CARTESIAN_POINT('Ctrl Pts',(-31.1489973536524,33.5377276733344,41.7386799227568));
#39772=CARTESIAN_POINT('Ctrl Pts',(-31.6908816410888,33.6398718046173,41.7757231858301));
#39773=CARTESIAN_POINT('Ctrl Pts',(-32.2327659285252,33.7420159359003,41.8127664489033));
#39774=CARTESIAN_POINT('Ctrl Pts',(-32.830282514781,33.54901360121,41.8498097119766));
#39775=CARTESIAN_POINT('Ctrl Pts',(-33.2100165820346,33.1491743624933,41.8868529750498));
#39776=CARTESIAN_POINT('Ctrl Pts',(-33.5897506492881,32.7493351237766,41.9238962381231));
#39777=CARTESIAN_POINT('Ctrl Pts',(-33.7517021975394,32.1426589810335,41.9609395011963));
#39778=CARTESIAN_POINT('Ctrl Pts',(-33.6217602821139,31.6067613146595,41.9979827642695));
#39779=CARTESIAN_POINT('Ctrl Pts',(-33.4918183666883,31.0708636482855,42.0350260273428));
#39780=CARTESIAN_POINT('Ctrl Pts',(-33.0699829875859,30.6057444582805,42.072069290416));
#39781=CARTESIAN_POINT('Ctrl Pts',(-32.5492851384242,30.4242379117307,42.1091125534893));
#39782=CARTESIAN_POINT('Ctrl Pts',(-32.0285872892625,30.242731365181,42.1461558165625));
#39783=CARTESIAN_POINT('Ctrl Pts',(-31.4090269700415,30.3448374620864,42.1831990796357));
#39784=CARTESIAN_POINT('Ctrl Pts',(-30.9741109104756,30.6838339417423,42.220242342709));
#39785=CARTESIAN_POINT('Ctrl Pts',(-30.5779071442121,30.9926560213956,42.2539883496027));
#39786=CARTESIAN_POINT('Ctrl Pts',(-30.3349398414768,31.4980736765861,42.2877343564965));
#39787=CARTESIAN_POINT('Ctrl Pts',(-30.3317921991812,32.000855278924,42.3214803633902));
#39788=CARTESIAN_POINT('Ctrl Pts',(-31.4698297828114,30.0148256743283,41.));
#39789=CARTESIAN_POINT('Ctrl Pts',(-31.4011629084353,30.0402504721211,41.));
#39790=CARTESIAN_POINT('Ctrl Pts',(-31.3341993832291,30.0695646102219,41.));
#39791=CARTESIAN_POINT('Ctrl Pts',(-31.2691281870165,30.1024741661484,41.));
#39792=CARTESIAN_POINT('Ctrl Pts',(-31.2022478796466,30.136298674439,41.));
#39793=CARTESIAN_POINT('Ctrl Pts',(-31.1373658136216,30.1739219879674,41.));
#39794=CARTESIAN_POINT('Ctrl Pts',(-31.0747183883007,30.2150696221828,41.));
#39795=CARTESIAN_POINT('Ctrl Pts',(-31.0217877302761,30.2498351587395,41.));
#39796=CARTESIAN_POINT('Ctrl Pts',(-30.9704526091484,30.2871175891263,41.));
#39797=CARTESIAN_POINT('Ctrl Pts',(-30.9208783414071,30.3267693724872,41.));
#39798=CARTESIAN_POINT('Ctrl Pts',(-30.8988476211705,30.3443905575476,41.));
#39799=CARTESIAN_POINT('Ctrl Pts',(-30.877164954821,30.3624798447009,41.));
#39800=CARTESIAN_POINT('Ctrl Pts',(-30.8558464048857,30.3810250092555,41.));
#39801=CARTESIAN_POINT('Ctrl Pts',(-30.8441323268764,30.3912151725146,41.));
#39802=CARTESIAN_POINT('Ctrl Pts',(-30.8325282028598,30.4015429837462,41.));
#39803=CARTESIAN_POINT('Ctrl Pts',(-30.8210368319428,30.4120064565416,41.));
#39804=CARTESIAN_POINT('Ctrl Pts',(-30.8104448512627,30.421650989165,41.));
#39805=CARTESIAN_POINT('Ctrl Pts',(-30.799947233707,30.4314122915714,41.));
#39806=CARTESIAN_POINT('Ctrl Pts',(-30.7895620525903,30.4412733595479,41.));
#39807=CARTESIAN_POINT('Ctrl Pts',(-30.7364770065195,30.4916793411058,41.));
#39808=CARTESIAN_POINT('Ctrl Pts',(-30.6862319428219,30.5447736155129,41.));
#39809=CARTESIAN_POINT('Ctrl Pts',(-30.6390455537104,30.6002968491221,41.));
#39810=CARTESIAN_POINT('Ctrl Pts',(-30.5922257365251,30.6553887452401,41.));
#39811=CARTESIAN_POINT('Ctrl Pts',(-30.5484167469741,30.7128728910456,41.));
#39812=CARTESIAN_POINT('Ctrl Pts',(-30.5078770105767,30.7725201905801,41.));
#39813=CARTESIAN_POINT('Ctrl Pts',(-30.4741908999485,30.8220835501218,41.));
#39814=CARTESIAN_POINT('Ctrl Pts',(-30.4427627290454,30.8731411370933,41.));
#39815=CARTESIAN_POINT('Ctrl Pts',(-30.4137683610081,30.9255679879711,41.));
#39816=CARTESIAN_POINT('Ctrl Pts',(-30.4016604837945,30.9474611319191,41.));
#39817=CARTESIAN_POINT('Ctrl Pts',(-30.3899773466439,30.9695930938703,41.));
#39818=CARTESIAN_POINT('Ctrl Pts',(-30.3787331983111,30.9919548569239,41.));
#39819=CARTESIAN_POINT('Ctrl Pts',(-30.3735336034124,31.0022955341953,41.));
#39820=CARTESIAN_POINT('Ctrl Pts',(-30.3684278936195,31.0126853517444,41.));
#39821=CARTESIAN_POINT('Ctrl Pts',(-30.363417543091,31.0231234159713,41.));
#39822=CARTESIAN_POINT('Ctrl Pts',(-30.3581837446205,31.0340269893391,41.));
#39823=CARTESIAN_POINT('Ctrl Pts',(-30.3530576063202,31.0449757645301,41.));
#39824=CARTESIAN_POINT('Ctrl Pts',(-30.348042198309,31.0559644120955,41.));
#39825=CARTESIAN_POINT('Ctrl Pts',(-30.3195018402902,31.1184957026626,41.));
#39826=CARTESIAN_POINT('Ctrl Pts',(-30.2945224741136,31.182360381032,41.));
#39827=CARTESIAN_POINT('Ctrl Pts',(-30.2733275766249,31.2473541148403,41.));
#39828=CARTESIAN_POINT('Ctrl Pts',(-30.2541304118743,31.3062218407325,41.));
#39829=CARTESIAN_POINT('Ctrl Pts',(-30.2380382479865,31.3660164111607,41.));
#39830=CARTESIAN_POINT('Ctrl Pts',(-30.2252538021287,31.4265908222046,41.));
#39831=CARTESIAN_POINT('Ctrl Pts',(-30.2101196168207,31.4982986124253,41.));
#39832=CARTESIAN_POINT('Ctrl Pts',(-30.1996201783637,31.5711007701871,41.));
#39833=CARTESIAN_POINT('Ctrl Pts',(-30.1936803374547,31.644574102922,41.));
#39834=CARTESIAN_POINT('Ctrl Pts',(-30.192373397395,31.6607404015391,41.));
#39835=CARTESIAN_POINT('Ctrl Pts',(-30.1912874246838,31.6769391120234,41.));
#39836=CARTESIAN_POINT('Ctrl Pts',(-30.1904219877599,31.6931655622086,41.));
#39837=CARTESIAN_POINT('Ctrl Pts',(-30.1895243490928,31.7099957767667,41.));
#39838=CARTESIAN_POINT('Ctrl Pts',(-30.1888639529652,31.72686206175,41.));
#39839=CARTESIAN_POINT('Ctrl Pts',(-30.1884408807954,31.7437248028176,41.));
#39840=CARTESIAN_POINT('Ctrl Pts',(-30.1867207010254,31.8122874455965,41.));
#39841=CARTESIAN_POINT('Ctrl Pts',(-30.1889121483104,31.8808779859611,41.));
#39842=CARTESIAN_POINT('Ctrl Pts',(-30.1948946421042,31.9491579840471,41.));
#39843=CARTESIAN_POINT('Ctrl Pts',(-30.2008758629234,32.0174234532929,41.));
#39844=CARTESIAN_POINT('Ctrl Pts',(-30.2106469707899,32.0853795842456,41.));
#39845=CARTESIAN_POINT('Ctrl Pts',(-30.2241370660968,32.1526731205519,41.));
#39846=CARTESIAN_POINT('Ctrl Pts',(-30.2338950540172,32.2013495382838,41.));
#39847=CARTESIAN_POINT('Ctrl Pts',(-30.2455999681403,32.2496790024792,41.));
#39848=CARTESIAN_POINT('Ctrl Pts',(-30.2592391639345,32.2975181738642,41.));
#39849=CARTESIAN_POINT('Ctrl Pts',(-30.269473786622,32.333415881925,41.));
#39850=CARTESIAN_POINT('Ctrl Pts',(-30.2807978036095,32.3690373637504,41.));
#39851=CARTESIAN_POINT('Ctrl Pts',(-30.293209784769,32.404317881334,41.));
#39852=CARTESIAN_POINT('Ctrl Pts',(-30.2973424899566,32.4160649164095,41.));
#39853=CARTESIAN_POINT('Ctrl Pts',(-30.3015926249635,32.4277649816303,41.));
#39854=CARTESIAN_POINT('Ctrl Pts',(-30.3059595224773,32.4394154501761,41.));
#39855=CARTESIAN_POINT('Ctrl Pts',(-30.3290832908114,32.501107471751,41.));
#39856=CARTESIAN_POINT('Ctrl Pts',(-30.355479582176,32.5614159713376,41.));
#39857=CARTESIAN_POINT('Ctrl Pts',(-30.3850984013863,32.6200067698823,41.));
#39858=CARTESIAN_POINT('Ctrl Pts',(-30.4059238288755,32.6612028222288,41.));
#39859=CARTESIAN_POINT('Ctrl Pts',(-30.4283432331492,32.7015491648088,41.));
#39860=CARTESIAN_POINT('Ctrl Pts',(-30.4523496254102,32.7409183022664,41.));
#39861=CARTESIAN_POINT('Ctrl Pts',(-30.4600634641435,32.7535685653344,41.));
#39862=CARTESIAN_POINT('Ctrl Pts',(-30.4679423056765,32.7661195241672,41.));
#39863=CARTESIAN_POINT('Ctrl Pts',(-30.4759826277317,32.7785613658112,41.));
#39864=CARTESIAN_POINT('Ctrl Pts',(-30.5102255857725,32.8315499722927,41.));
#39865=CARTESIAN_POINT('Ctrl Pts',(-30.5473242553461,32.8824546989078,41.));
#39866=CARTESIAN_POINT('Ctrl Pts',(-30.5872443914682,32.9309602517629,41.));
#39867=CARTESIAN_POINT('Ctrl Pts',(-30.6240203591527,32.9756454361735,41.));
#39868=CARTESIAN_POINT('Ctrl Pts',(-30.6631914372638,33.0182945811671,41.));
#39869=CARTESIAN_POINT('Ctrl Pts',(-30.7047522727162,33.0586283114149,41.));
#39870=CARTESIAN_POINT('Ctrl Pts',(-30.7125941112345,33.0662386155871,41.));
#39871=CARTESIAN_POINT('Ctrl Pts',(-30.720521081831,33.073766383874,41.));
#39872=CARTESIAN_POINT('Ctrl Pts',(-30.728531577822,33.081210944453,41.));
#39873=CARTESIAN_POINT('Origin',(-32.,32.,48.));
#39874=CARTESIAN_POINT('Origin',(32.,32.,54.));
#39875=CARTESIAN_POINT('Ctrl Pts',(31.3249228143251,30.4769022377466,54.));
#39876=CARTESIAN_POINT('Ctrl Pts',(31.2652392925755,30.4954885225906,54.));
#39877=CARTESIAN_POINT('Ctrl Pts',(31.2068683211469,30.5176493909919,54.));
#39878=CARTESIAN_POINT('Ctrl Pts',(31.1499664526549,30.5430859698249,54.));
#39879=CARTESIAN_POINT('Ctrl Pts',(31.1138836855836,30.5592158821362,54.));
#39880=CARTESIAN_POINT('Ctrl Pts',(31.0783916111174,30.5766640975224,54.));
#39881=CARTESIAN_POINT('Ctrl Pts',(31.0435310469341,30.5953648451471,54.));
#39882=CARTESIAN_POINT('Ctrl Pts',(31.0197684746904,30.6081121393132,54.));
#39883=CARTESIAN_POINT('Ctrl Pts',(30.996299346444,30.6214415774298,54.));
#39884=CARTESIAN_POINT('Ctrl Pts',(30.9731370541742,30.6353342860965,54.));
#39885=CARTESIAN_POINT('Ctrl Pts',(30.9607881815602,30.6427411216371,54.));
#39886=CARTESIAN_POINT('Ctrl Pts',(30.9485266882192,30.6503081374092,54.));
#39887=CARTESIAN_POINT('Ctrl Pts',(30.9363666889478,30.6580245755571,54.));
#39888=CARTESIAN_POINT('Ctrl Pts',(30.8806648540549,30.6933715977137,54.));
#39889=CARTESIAN_POINT('Ctrl Pts',(30.8270267921164,30.7318880347813,54.));
#39890=CARTESIAN_POINT('Ctrl Pts',(30.7756343274519,30.773271408358,54.));
#39891=CARTESIAN_POINT('Ctrl Pts',(30.7385655425372,30.8031207526961,54.));
#39892=CARTESIAN_POINT('Ctrl Pts',(30.7026651301385,30.8344628590285,54.));
#39893=CARTESIAN_POINT('Ctrl Pts',(30.6680066073461,30.8672000886409,54.));
#39894=CARTESIAN_POINT('Ctrl Pts',(30.6585374859811,30.876144289818,54.));
#39895=CARTESIAN_POINT('Ctrl Pts',(30.6491610994594,30.8851926993893,54.));
#39896=CARTESIAN_POINT('Ctrl Pts',(30.639879031127,30.8943434783427,54.));
#39897=CARTESIAN_POINT('Ctrl Pts',(30.6303154851562,30.9037717535995,54.));
#39898=CARTESIAN_POINT('Ctrl Pts',(30.6208577720802,30.9133031307529,54.));
#39899=CARTESIAN_POINT('Ctrl Pts',(30.6115111155573,30.922931187383,54.));
#39900=CARTESIAN_POINT('Ctrl Pts',(30.5642487582623,30.9716164740835,54.));
#39901=CARTESIAN_POINT('Ctrl Pts',(30.5197932859356,31.0228006877741,54.));
#39902=CARTESIAN_POINT('Ctrl Pts',(30.4783284042593,31.0761767372777,54.));
#39903=CARTESIAN_POINT('Ctrl Pts',(30.436264293657,31.1303241497162,54.));
#39904=CARTESIAN_POINT('Ctrl Pts',(30.3972769445889,31.1867277877173,54.));
#39905=CARTESIAN_POINT('Ctrl Pts',(30.3615825003683,31.2451139635999,54.));
#39906=CARTESIAN_POINT('Ctrl Pts',(30.3394718058714,31.2812809057101,54.));
#39907=CARTESIAN_POINT('Ctrl Pts',(30.3186251627735,31.3182094602772,54.));
#39908=CARTESIAN_POINT('Ctrl Pts',(30.2991008591822,31.3558418492927,54.));
#39909=CARTESIAN_POINT('Ctrl Pts',(30.2831165799908,31.3866509693133,54.));
#39910=CARTESIAN_POINT('Ctrl Pts',(30.2680186762366,31.417931948164,54.));
#39911=CARTESIAN_POINT('Ctrl Pts',(30.2538424561611,31.4496552941849,54.));
#39912=CARTESIAN_POINT('Ctrl Pts',(30.2480304578859,31.4626613022304,54.));
#39913=CARTESIAN_POINT('Ctrl Pts',(30.2423725282932,31.4757441614276,54.));
#39914=CARTESIAN_POINT('Ctrl Pts',(30.2368802697065,31.4888793524524,54.));
#39915=CARTESIAN_POINT('Ctrl Pts',(30.209689682674,31.5539078920073,54.));
#39916=CARTESIAN_POINT('Ctrl Pts',(30.1865048065016,31.6203282670227,54.));
#39917=CARTESIAN_POINT('Ctrl Pts',(30.1675372143216,31.6878453452323,54.));
#39918=CARTESIAN_POINT('Ctrl Pts',(30.165437190741,31.695320593276,54.));
#39919=CARTESIAN_POINT('Ctrl Pts',(30.1633888988524,31.7028093234633,54.));
#39920=CARTESIAN_POINT('Ctrl Pts',(30.1613926538322,31.7103111628798,54.));
#39921=CARTESIAN_POINT('Ctrl Pts',(30.1440545227347,31.7754674307538,54.));
#39922=CARTESIAN_POINT('Ctrl Pts',(30.1306386910357,31.8416105480239,54.));
#39923=CARTESIAN_POINT('Ctrl Pts',(30.1209911133228,31.9084360573021,54.));
#39924=CARTESIAN_POINT('Ctrl Pts',(30.1106126487227,31.9803241729591,54.));
#39925=CARTESIAN_POINT('Ctrl Pts',(30.1045944012331,32.0530027832628,54.));
#39926=CARTESIAN_POINT('Ctrl Pts',(30.1028047404686,32.1261154066584,54.));
#39927=CARTESIAN_POINT('Ctrl Pts',(30.1024846698419,32.139191182611,54.));
#39928=CARTESIAN_POINT('Ctrl Pts',(30.1023000105237,32.1522808750456,54.));
#39929=CARTESIAN_POINT('Ctrl Pts',(30.1022502162009,32.1653824793981,54.));
#39930=CARTESIAN_POINT('Ctrl Pts',(30.1022052492636,32.1772139290201,54.));
#39931=CARTESIAN_POINT('Ctrl Pts',(30.1022703199631,32.1890464872063,54.));
#39932=CARTESIAN_POINT('Ctrl Pts',(30.1024444765937,32.2008751816772,54.));
#39933=CARTESIAN_POINT('Ctrl Pts',(30.1034907073006,32.2719350278467,54.));
#39934=CARTESIAN_POINT('Ctrl Pts',(30.1084695156064,32.3428927641364,54.));
#39935=CARTESIAN_POINT('Ctrl Pts',(30.1172007707484,32.413412787761,54.));
#39936=CARTESIAN_POINT('Ctrl Pts',(30.1261162611738,32.4854208307286,54.));
#39937=CARTESIAN_POINT('Ctrl Pts',(30.1389441735648,32.5569734294332,54.));
#39938=CARTESIAN_POINT('Ctrl Pts',(30.1555454304087,32.6277294754119,54.));
#39939=CARTESIAN_POINT('Ctrl Pts',(30.1722476063644,32.6989156476985,54.));
#39940=CARTESIAN_POINT('Ctrl Pts',(30.1927692213023,32.7692966238086,54.));
#39941=CARTESIAN_POINT('Ctrl Pts',(30.2170210478913,32.8385259647519,54.));
#39942=CARTESIAN_POINT('Ctrl Pts',(30.2230020581078,32.8555993754471,54.));
#39943=CARTESIAN_POINT('Ctrl Pts',(30.2292101918566,32.8726027019187,54.));
#39944=CARTESIAN_POINT('Ctrl Pts',(30.2356445879338,32.8895306376608,54.));
#39945=CARTESIAN_POINT('Ctrl Pts',(30.2407135830383,32.9028664072306,54.));
#39946=CARTESIAN_POINT('Ctrl Pts',(30.2459237771072,32.9161569899756,54.));
#39947=CARTESIAN_POINT('Ctrl Pts',(30.2512663088271,32.9293795887561,54.));
#39948=CARTESIAN_POINT('Ctrl Pts',(30.2794914917943,32.9992360331264,54.));
#39949=CARTESIAN_POINT('Ctrl Pts',(30.3114529069637,33.0673215315237,54.));
#39950=CARTESIAN_POINT('Ctrl Pts',(30.3469924470567,33.1332787426213,54.));
#39951=CARTESIAN_POINT('Ctrl Pts',(30.3825709958759,33.1993083493318,54.));
#39952=CARTESIAN_POINT('Ctrl Pts',(30.4217357000898,33.2632061094673,54.));
#39953=CARTESIAN_POINT('Ctrl Pts',(30.4643796980224,33.3246090804382,54.));
#39954=CARTESIAN_POINT('Ctrl Pts',(30.5060535747287,33.3846151766228,54.));
#39955=CARTESIAN_POINT('Ctrl Pts',(30.5510505813055,33.4422396847995,54.));
#39956=CARTESIAN_POINT('Ctrl Pts',(30.5993163191418,33.4971242544356,54.));
#39957=CARTESIAN_POINT('Ctrl Pts',(30.6096515303738,33.5088767655541,54.));
#39958=CARTESIAN_POINT('Ctrl Pts',(30.6201367787392,33.5205035406757,54.));
#39959=CARTESIAN_POINT('Ctrl Pts',(30.6307717865001,33.5320008742866,54.));
#39960=CARTESIAN_POINT('Ctrl Pts',(30.6398828337217,33.5418506789889,54.));
#39961=CARTESIAN_POINT('Ctrl Pts',(30.6491037972993,33.5516054798596,54.));
#39962=CARTESIAN_POINT('Ctrl Pts',(30.6584328166059,33.5612648614874,54.));
#39963=CARTESIAN_POINT('Ctrl Pts',(31.6163320011532,34.0186125009919,54.));
#39964=CARTESIAN_POINT('Ctrl Pts',(31.6906496900554,34.0256330925326,54.));
#39965=CARTESIAN_POINT('Ctrl Pts',(31.7652154809392,34.0282517372431,54.));
#39966=CARTESIAN_POINT('Ctrl Pts',(31.8397072565627,34.0266320313122,54.));
#39967=CARTESIAN_POINT('Ctrl Pts',(31.9122409523519,34.0250549007326,54.));
#39968=CARTESIAN_POINT('Ctrl Pts',(31.9847052554167,34.0194586585716,54.));
#39969=CARTESIAN_POINT('Ctrl Pts',(32.0567895869437,34.009950480074,54.));
#39970=CARTESIAN_POINT('Ctrl Pts',(32.0728797642137,34.0078281287349,54.));
#39971=CARTESIAN_POINT('Ctrl Pts',(32.0889530628615,34.0055103754858,54.));
#39972=CARTESIAN_POINT('Ctrl Pts',(32.1049990603174,34.0029992289119,54.));
#39973=CARTESIAN_POINT('Ctrl Pts',(32.1786326365799,33.9914758129782,54.));
#39974=CARTESIAN_POINT('Ctrl Pts',(32.2515465637322,33.9759078826664,54.));
#39975=CARTESIAN_POINT('Ctrl Pts',(32.3234089085464,33.9564349301845,54.));
#39976=CARTESIAN_POINT('Ctrl Pts',(32.3738561644734,33.9427649473854,54.));
#39977=CARTESIAN_POINT('Ctrl Pts',(32.4237849247872,33.9271694712033,54.));
#39978=CARTESIAN_POINT('Ctrl Pts',(32.4730724197954,33.9096836167836,54.));
#39979=CARTESIAN_POINT('Ctrl Pts',(32.4917998071078,33.9030396522617,54.));
#39980=CARTESIAN_POINT('Ctrl Pts',(32.5104345309238,33.896122668595,54.));
#39981=CARTESIAN_POINT('Ctrl Pts',(32.5289695229777,33.8889342296203,54.));
#39982=CARTESIAN_POINT('Ctrl Pts',(32.5466571100482,33.8820744403149,54.));
#39983=CARTESIAN_POINT('Ctrl Pts',(32.5642593377296,33.874964996238,54.));
#39984=CARTESIAN_POINT('Ctrl Pts',(32.5817391496632,33.8676204838936,54.));
#39985=CARTESIAN_POINT('Ctrl Pts',(32.6486663172982,33.8394996201947,54.));
#39986=CARTESIAN_POINT('Ctrl Pts',(32.7138733597198,33.8079107127814,54.));
#39987=CARTESIAN_POINT('Ctrl Pts',(32.7770520704153,33.7729809129467,54.));
#39988=CARTESIAN_POINT('Ctrl Pts',(32.8388737816019,33.7388013614265,54.));
#39989=CARTESIAN_POINT('Ctrl Pts',(32.8987540539514,33.7014222659878,54.));
#39990=CARTESIAN_POINT('Ctrl Pts',(32.9563717527268,33.6609259427107,54.));
#39991=CARTESIAN_POINT('Ctrl Pts',(33.0127259983595,33.6213176314161,54.));
#39992=CARTESIAN_POINT('Ctrl Pts',(33.0669163726691,33.5787267777315,54.));
#39993=CARTESIAN_POINT('Ctrl Pts',(33.1186019715482,33.5332031777472,54.));
#39994=CARTESIAN_POINT('Ctrl Pts',(33.1354287832063,33.5183824721823,54.));
#39995=CARTESIAN_POINT('Ctrl Pts',(33.1519897538664,33.5032507388309,54.));
#39996=CARTESIAN_POINT('Ctrl Pts',(33.1682720164058,33.4878091927252,54.));
#39997=CARTESIAN_POINT('Ctrl Pts',(33.1774026318648,33.4791500263936,54.));
#39998=CARTESIAN_POINT('Ctrl Pts',(33.1864464242868,33.4703924724357,54.));
#39999=CARTESIAN_POINT('Ctrl Pts',(33.1953886696531,33.4615493621301,54.));
#40000=CARTESIAN_POINT('Ctrl Pts',(33.2439541235006,33.4135223121193,54.));
#40001=CARTESIAN_POINT('Ctrl Pts',(33.2896152685707,33.3628927157441,54.));
#40002=CARTESIAN_POINT('Ctrl Pts',(33.332079740635,33.3097415636927,54.));
#40003=CARTESIAN_POINT('Ctrl Pts',(33.3381856709119,33.3020990048009,54.));
#40004=CARTESIAN_POINT('Ctrl Pts',(33.3442254363888,33.2944042619705,54.));
#40005=CARTESIAN_POINT('Ctrl Pts',(33.3501980920418,33.2866575274568,54.));
#40006=CARTESIAN_POINT('Ctrl Pts',(33.3925565636038,33.2317171704926,54.));
#40007=CARTESIAN_POINT('Ctrl Pts',(33.4315436482843,33.1741631439773,54.));
#40008=CARTESIAN_POINT('Ctrl Pts',(33.4670921079473,33.1143576586055,54.));
#40009=CARTESIAN_POINT('Ctrl Pts',(33.5002539400628,33.058567351957,54.));
#40010=CARTESIAN_POINT('Ctrl Pts',(33.5304229661912,33.0008167747747,54.));
#40011=CARTESIAN_POINT('Ctrl Pts',(33.557504889555,32.9413945291346,54.));
#40012=CARTESIAN_POINT('Ctrl Pts',(33.563398708835,32.9284625090446,54.));
#40013=CARTESIAN_POINT('Ctrl Pts',(33.5691461688042,32.9154513223191,54.));
#40014=CARTESIAN_POINT('Ctrl Pts',(33.5747460519361,32.9023639711173,54.));
#40015=CARTESIAN_POINT('Ctrl Pts',(33.5792733485958,32.8917833357747,54.));
#40016=CARTESIAN_POINT('Ctrl Pts',(33.5837039631642,32.8811532170269,54.));
#40017=CARTESIAN_POINT('Ctrl Pts',(33.588032228022,32.870488236425,54.));
#40018=CARTESIAN_POINT('Ctrl Pts',(33.6137449952032,32.8071311702053,54.));
#40019=CARTESIAN_POINT('Ctrl Pts',(33.6359004658581,32.7424283875045,54.));
#40020=CARTESIAN_POINT('Ctrl Pts',(33.6544523724797,32.6767299554583,54.));
#40021=CARTESIAN_POINT('Ctrl Pts',(33.6729186410861,32.6113347959239,54.));
#40022=CARTESIAN_POINT('Ctrl Pts',(33.6878145454425,32.5449520220622,54.));
#40023=CARTESIAN_POINT('Ctrl Pts',(33.6990433939503,32.4779242445738,54.));
#40024=CARTESIAN_POINT('Ctrl Pts',(33.7100316622983,32.4123325496376,54.));
#40025=CARTESIAN_POINT('Ctrl Pts',(33.7175081962818,32.3461222296304,54.));
#40026=CARTESIAN_POINT('Ctrl Pts',(33.7213344983069,32.2796272244155,54.));
#40027=CARTESIAN_POINT('Ctrl Pts',(33.7224477961555,32.2602798896349,54.));
#40028=CARTESIAN_POINT('Ctrl Pts',(33.7232517671042,32.2409085892293,54.));
#40029=CARTESIAN_POINT('Ctrl Pts',(33.7237422384393,32.2215219353351,54.));
#40030=CARTESIAN_POINT('Ctrl Pts',(33.72401437674,32.2107652393375,54.));
#40031=CARTESIAN_POINT('Ctrl Pts',(33.7241897483875,32.2000135675735,54.));
#40032=CARTESIAN_POINT('Ctrl Pts',(33.7242681224748,32.1892683767583,54.));
#40033=CARTESIAN_POINT('Ctrl Pts',(33.7247442520814,32.1239903792229,54.));
#40034=CARTESIAN_POINT('Ctrl Pts',(33.7216445871738,32.0589495683597,54.));
#40035=CARTESIAN_POINT('Ctrl Pts',(33.7148888928212,31.9944557738682,54.));
#40036=CARTESIAN_POINT('Ctrl Pts',(33.7079758523754,31.9284598618934,54.));
#40037=CARTESIAN_POINT('Ctrl Pts',(33.6972346951092,31.8630356000403,54.));
#40038=CARTESIAN_POINT('Ctrl Pts',(33.6825255118463,31.798535704284,54.));
#40039=CARTESIAN_POINT('Ctrl Pts',(33.668893202805,31.7387579112976,54.));
#40040=CARTESIAN_POINT('Ctrl Pts',(33.6518520502579,31.6797736424106,54.));
#40041=CARTESIAN_POINT('Ctrl Pts',(33.6312489013858,31.6218918727598,54.));
#40042=CARTESIAN_POINT('Ctrl Pts',(33.6296213708013,31.6173195449581,54.));
#40043=CARTESIAN_POINT('Ctrl Pts',(33.6279715922876,31.6127541143676,54.));
#40044=CARTESIAN_POINT('Ctrl Pts',(33.6262994796833,31.6081957426667,54.));
#40045=CARTESIAN_POINT('Ctrl Pts',(33.6225368250294,31.5979383123658,54.));
#40046=CARTESIAN_POINT('Ctrl Pts',(33.6186610809759,31.587716623037,54.));
#40047=CARTESIAN_POINT('Ctrl Pts',(33.614673303851,31.5775320375437,54.));
#40048=CARTESIAN_POINT('Origin',(32.,32.,39.4540747194623));
#40049=CARTESIAN_POINT('Ctrl Pts',(34.0565678449602,32.0014926321758,41.2040747194623));
#40050=CARTESIAN_POINT('Ctrl Pts',(34.0573842294279,32.0995827500376,41.2094078928854));
#40051=CARTESIAN_POINT('Ctrl Pts',(34.0064118509519,32.8781629596678,41.2517843293816));
#40052=CARTESIAN_POINT('Ctrl Pts',(33.0117215203461,34.2080087873732,41.3312040289512));
#40053=CARTESIAN_POINT('Ctrl Pts',(30.693930615665,34.0473906585599,41.4423338181709));
#40054=CARTESIAN_POINT('Ctrl Pts',(29.5714562640958,32.0133707418711,41.5534636073906));
#40055=CARTESIAN_POINT('Ctrl Pts',(30.6715507113449,29.9669383183226,41.6645933966104));
#40056=CARTESIAN_POINT('Ctrl Pts',(32.9874316286532,29.7812306730564,41.7757231858301));
#40057=CARTESIAN_POINT('Ctrl Pts',(34.0018420245732,31.1064228934244,41.8555502934474));
#40058=CARTESIAN_POINT('Ctrl Pts',(34.0572700743595,31.8927563372387,41.8983341379915));
#40059=CARTESIAN_POINT('Ctrl Pts',(34.0563620767522,31.9983919833491,41.9040747194623));
#40060=CARTESIAN_POINT('Ctrl Pts',(34.052676219088,31.9976391197375,41.1459252805377));
#40061=CARTESIAN_POINT('Ctrl Pts',(34.0491258389796,32.4677617736048,41.1713700465049));
#40062=CARTESIAN_POINT('Ctrl Pts',(33.6566798069838,33.6293344104736,41.2338580755454));
#40063=CARTESIAN_POINT('Ctrl Pts',(31.7284038427318,34.4127959913661,41.3333893676592));
#40064=CARTESIAN_POINT('Ctrl Pts',(29.8256278405404,33.0815586024407,41.4445191568789));
#40065=CARTESIAN_POINT('Ctrl Pts',(29.9119860164316,30.7594030366271,41.5556489460986));
#40066=CARTESIAN_POINT('Ctrl Pts',(31.9096898523802,29.5731770382926,41.6667787353184));
#40067=CARTESIAN_POINT('Ctrl Pts',(33.7208347882445,30.4738973185028,41.7635375134647));
#40068=CARTESIAN_POINT('Ctrl Pts',(34.0499076510441,31.5817394238508,41.8232530285378));
#40069=CARTESIAN_POINT('Ctrl Pts',(34.0520872716434,32.0011660295939,41.8459252805377));
#40070=CARTESIAN_POINT('Ctrl Pts',(30.7309291201476,33.0793586530485,41.));
#40071=CARTESIAN_POINT('Ctrl Pts',(30.3720428517593,32.6573931542737,41.0370432630732));
#40072=CARTESIAN_POINT('Ctrl Pts',(30.114703984369,31.4343794756361,41.1111297892197));
#40073=CARTESIAN_POINT('Ctrl Pts',(31.4546599251405,30.1066751817884,41.2222595784394));
#40074=CARTESIAN_POINT('Ctrl Pts',(33.2938434714149,30.5162236027394,41.3333893676592));
#40075=CARTESIAN_POINT('Ctrl Pts',(33.9488200232574,32.2815049853891,41.4445191568789));
#40076=CARTESIAN_POINT('Ctrl Pts',(32.8203080924183,33.7902628737138,41.5556489460987));
#40077=CARTESIAN_POINT('Ctrl Pts',(30.9410334131636,33.6600330148003,41.6667787353184));
#40078=CARTESIAN_POINT('Ctrl Pts',(30.0309264562519,32.010841054122,41.7779085245381));
#40079=CARTESIAN_POINT('Ctrl Pts',(30.9228876919823,30.3515849803264,41.8890383137579));
#40080=CARTESIAN_POINT('Ctrl Pts',(32.8006137453881,30.2010124352413,42.0001681029775));
#40081=CARTESIAN_POINT('Ctrl Pts',(33.9456251072274,31.6968174418197,42.1112978921973));
#40082=CARTESIAN_POINT('Ctrl Pts',(33.3100223159796,33.4701102033079,42.222427681417));
#40083=CARTESIAN_POINT('Ctrl Pts',(31.4755008806028,33.897964772512,42.3335574706367));
#40084=CARTESIAN_POINT('Ctrl Pts',(30.1209955671039,32.5888272504792,42.4446872598565));
#40085=CARTESIAN_POINT('Ctrl Pts',(30.4861346246503,30.740799047359,42.5558170490762));
#40086=CARTESIAN_POINT('Ctrl Pts',(32.2367469115823,30.0451790962689,42.6669468382959));
#40087=CARTESIAN_POINT('Ctrl Pts',(33.7706909646394,31.1385894331762,42.7780766275156));
#40088=CARTESIAN_POINT('Ctrl Pts',(33.6841178632491,33.0203536843011,42.8892064167355));
#40089=CARTESIAN_POINT('Ctrl Pts',(32.0562583498155,33.9683011547304,43.000336205955));
#40090=CARTESIAN_POINT('Ctrl Pts',(30.3769118083114,33.1148808315266,43.1114659951749));
#40091=CARTESIAN_POINT('Ctrl Pts',(30.1829979763716,31.2411336223703,43.2225957843945));
#40092=CARTESIAN_POINT('Ctrl Pts',(31.6519846928047,30.0618927123183,43.3337255736143));
#40093=CARTESIAN_POINT('Ctrl Pts',(33.4394712438521,30.6563865640221,43.444855362834));
#40094=CARTESIAN_POINT('Ctrl Pts',(33.909569323175,32.4805408665194,43.5559851520537));
#40095=CARTESIAN_POINT('Ctrl Pts',(32.6320502662273,33.8649093766671,43.6671149412734));
#40096=CARTESIAN_POINT('Ctrl Pts',(30.7760856599876,33.5425330506821,43.7782447304932));
#40097=CARTESIAN_POINT('Ctrl Pts',(30.0402341848989,31.8084472041341,43.8893745197128));
#40098=CARTESIAN_POINT('Ctrl Pts',(31.0979391310306,30.2496683993889,44.0005043089327));
#40099=CARTESIAN_POINT('Ctrl Pts',(32.9812004019927,30.2927740938005,44.1116340981523));
#40100=CARTESIAN_POINT('Ctrl Pts',(33.9664777057302,31.8983144235561,44.2227638873721));
#40101=CARTESIAN_POINT('Ctrl Pts',(33.1520559387442,33.5969162900964,44.3338936765918));
#40102=CARTESIAN_POINT('Ctrl Pts',(31.2832850701469,33.8340376857981,44.4450234658115));
#40103=CARTESIAN_POINT('Ctrl Pts',(30.0704439329009,32.3926676807569,44.5561532550313));
#40104=CARTESIAN_POINT('Ctrl Pts',(30.6235115831001,30.5919324725962,44.667283044251));
#40105=CARTESIAN_POINT('Ctrl Pts',(32.4363265050506,30.0798453956562,44.7784128334707));
#40106=CARTESIAN_POINT('Ctrl Pts',(33.8498201413429,31.3250629894034,44.8895426226904));
#40107=CARTESIAN_POINT('Ctrl Pts',(33.5703784447421,33.1879756158609,45.0006724119101));
#40108=CARTESIAN_POINT('Ctrl Pts',(31.8537434255585,33.9636658417418,45.1118022011299));
#40109=CARTESIAN_POINT('Ctrl Pts',(30.2709608372172,32.9422303843299,45.2229319903496));
#40110=CARTESIAN_POINT('Ctrl Pts',(30.2705761400058,31.0584758972423,45.3340617795693));
#40111=CARTESIAN_POINT('Ctrl Pts',(31.8529414046403,30.0363940585948,45.4451915687891));
#40112=CARTESIAN_POINT('Ctrl Pts',(33.5698931009639,30.8113830831017,45.5563213580088));
#40113=CARTESIAN_POINT('Ctrl Pts',(33.8500956560671,32.6741814199402,45.6674511472285));
#40114=CARTESIAN_POINT('Ctrl Pts',(32.4371107301896,33.9199762324424,45.7785809364483));
#40115=CARTESIAN_POINT('Ctrl Pts',(30.6240868043111,33.4086296182887,45.8897107256679));
#40116=CARTESIAN_POINT('Ctrl Pts',(30.0702837139698,31.6081204534292,46.0008405148878));
#40117=CARTESIAN_POINT('Ctrl Pts',(31.2825360417016,30.1662551998346,46.1119703041074));
#40118=CARTESIAN_POINT('Ctrl Pts',(33.1514036034955,30.4026133012171,46.2231000933272));
#40119=CARTESIAN_POINT('Ctrl Pts',(33.9665190738225,32.1008823863883,46.3342298825469));
#40120=CARTESIAN_POINT('Ctrl Pts',(32.9818976137984,33.7068250055609,46.4453596717666));
#40121=CARTESIAN_POINT('Ctrl Pts',(31.0986541058623,33.7506998893905,46.5564894609863));
#40122=CARTESIAN_POINT('Ctrl Pts',(30.0403125855518,32.1923532199997,46.6676192502061));
#40123=CARTESIAN_POINT('Ctrl Pts',(30.7754557350193,30.457966969649,46.7787490394258));
#40124=CARTESIAN_POINT('Ctrl Pts',(32.6312885161675,30.1348326260236,46.8898788286455));
#40125=CARTESIAN_POINT('Ctrl Pts',(33.9093728933581,31.5186792361636,47.0010086178653));
#40126=CARTESIAN_POINT('Ctrl Pts',(33.4400199048342,33.3430253896603,47.112138407085));
#40127=CARTESIAN_POINT('Ctrl Pts',(31.6527763157716,33.9382492710438,47.2232681963047));
#40128=CARTESIAN_POINT('Ctrl Pts',(30.1833080770308,32.7596084390061,47.3343979855245));
#40129=CARTESIAN_POINT('Ctrl Pts',(30.3764565849878,30.8857822012005,47.4455277747441));
#40130=CARTESIAN_POINT('Ctrl Pts',(32.0554544197689,30.0316760096674,47.5566575639639));
#40131=CARTESIAN_POINT('Ctrl Pts',(33.6837009709555,30.9789585885018,47.6677873531836));
#40132=CARTESIAN_POINT('Ctrl Pts',(33.7710426525005,32.8606871944064,47.7789171424033));
#40133=CARTESIAN_POINT('Ctrl Pts',(32.2375453046347,33.9547242137542,47.890046931623));
#40134=CARTESIAN_POINT('Ctrl Pts',(30.4866490700389,33.2598188307756,48.0011767208428));
#40135=CARTESIAN_POINT('Ctrl Pts',(30.120755194936,31.4119409160375,48.1123065100625));
#40136=CARTESIAN_POINT('Ctrl Pts',(31.4747257858664,30.1022482977067,48.2234362992822));
#40137=CARTESIAN_POINT('Ctrl Pts',(33.3094216412102,30.5293574570545,48.334566088502));
#40138=CARTESIAN_POINT('Ctrl Pts',(33.9457490106048,32.3023827232517,48.4456958777217));
#40139=CARTESIAN_POINT('Ctrl Pts',(32.8013479862633,33.7986706003332,48.5568256669415));
#40140=CARTESIAN_POINT('Ctrl Pts',(30.9235619751506,33.64883464976,48.6679554561611));
#40141=CARTESIAN_POINT('Ctrl Pts',(30.0309203708958,31.9900031085938,48.7790852453808));
#40142=CARTESIAN_POINT('Ctrl Pts',(30.9403590894178,30.3403206140307,48.8902150346006));
#40143=CARTESIAN_POINT('Ctrl Pts',(32.8195696779774,30.2095586950333,49.0013448238203));
#40144=CARTESIAN_POINT('Ctrl Pts',(33.9487189851152,31.717389241814,49.1124746130401));
#40145=CARTESIAN_POINT('Ctrl Pts',(33.2944218100529,33.4838620897005,49.2236044022597));
#40146=CARTESIAN_POINT('Ctrl Pts',(31.4554838318502,33.8923204449074,49.3347341914795));
#40147=CARTESIAN_POINT('Ctrl Pts',(30.1148811457062,32.5689476502957,49.4458639806992));
#40148=CARTESIAN_POINT('Ctrl Pts',(30.4995187917492,30.7248801361138,49.5569937699189));
#40149=CARTESIAN_POINT('Ctrl Pts',(32.2573805675422,30.0477884932614,49.6681235591387));
#40150=CARTESIAN_POINT('Ctrl Pts',(33.7796904390966,31.1573396505239,49.7792533483584));
#40151=CARTESIAN_POINT('Ctrl Pts',(33.673246920729,33.038084421356,49.8903831375781));
#40152=CARTESIAN_POINT('Ctrl Pts',(32.0354659661174,33.9687855873198,50.0015129267978));
#40153=CARTESIAN_POINT('Ctrl Pts',(30.3652269439276,33.0976755343592,50.1126427160176));
#40154=CARTESIAN_POINT('Ctrl Pts',(30.1911144942798,31.2219847361484,50.2237725052373));
#40155=CARTESIAN_POINT('Ctrl Pts',(31.6724744429204,30.0583250701906,50.334902294457));
#40156=CARTESIAN_POINT('Ctrl Pts',(33.4535822295341,30.6716652434062,50.4460320836768));
#40157=CARTESIAN_POINT('Ctrl Pts',(33.9043873231198,32.5006829806665,50.5571618728964));
#40158=CARTESIAN_POINT('Ctrl Pts',(32.6123177908093,33.8714810837004,50.6682916621163));
#40159=CARTESIAN_POINT('Ctrl Pts',(30.7598616566552,33.5295199943014,50.7794214513359));
#40160=CARTESIAN_POINT('Ctrl Pts',(30.0423666855995,31.7877587930665,50.8905512405557));
#40161=CARTESIAN_POINT('Ctrl Pts',(31.1164764942148,30.2402384427668,51.0016810297754));
#40162=CARTESIAN_POINT('Ctrl Pts',(32.9991774339491,30.3032327858082,51.1128108189951));
#40163=CARTESIAN_POINT('Ctrl Pts',(33.9674420216862,31.9190900826419,51.2239406082149));
#40164=CARTESIAN_POINT('Ctrl Pts',(33.135125007345,33.6089952583346,51.3350703974345));
#40165=CARTESIAN_POINT('Ctrl Pts',(31.2639538959055,33.8263654225762,51.4462001866543));
#40166=CARTESIAN_POINT('Ctrl Pts',(30.0664041974282,32.3722657578878,51.557329975874));
#40167=CARTESIAN_POINT('Ctrl Pts',(30.638460407338,30.5774725092217,51.6684597650938));
#40168=CARTESIAN_POINT('Ctrl Pts',(32.4565828894534,30.0845609922851,51.7795895543135));
#40169=CARTESIAN_POINT('Ctrl Pts',(33.8568456580557,31.3446384854398,51.8907193435332));
#40170=CARTESIAN_POINT('Ctrl Pts',(33.5577434260076,33.2044957250635,52.0018491327529));
#40171=CARTESIAN_POINT('Ctrl Pts',(31.833011285784,33.9620115483424,52.1129789219727));
#40172=CARTESIAN_POINT('Ctrl Pts',(30.2611054409688,32.9239156618485,52.2241087111923));
#40173=CARTESIAN_POINT('Ctrl Pts',(30.2806169696143,31.0402622164347,52.3352385004122));
#40174=CARTESIAN_POINT('Ctrl Pts',(31.873689339204,30.034950312623,52.4463682896318));
#40175=CARTESIAN_POINT('Ctrl Pts',(33.5823595836263,30.8280307111899,52.5574980788517));
#40176=CARTESIAN_POINT('Ctrl Pts',(33.842872035858,32.6936844190747,52.6686278680713));
#40177=CARTESIAN_POINT('Ctrl Pts',(32.4168069193824,33.9244862123967,52.7797576572911));
#40178=CARTESIAN_POINT('Ctrl Pts',(30.6092867419366,33.3940180191776,52.8908874465107));
#40179=CARTESIAN_POINT('Ctrl Pts',(30.0745280763313,31.5877617807645,53.0020172357305));
#40180=CARTESIAN_POINT('Ctrl Pts',(31.3019487101277,30.1587772763281,53.1131470249502));
#40181=CARTESIAN_POINT('Ctrl Pts',(33.1682019308355,30.4148681833194,53.2242768141699));
#40182=CARTESIAN_POINT('Ctrl Pts',(33.9653618476556,32.1216380242729,53.3354066033897));
#40183=CARTESIAN_POINT('Ctrl Pts',(32.9637797039416,33.7171187586807,53.4465363926094));
#40184=CARTESIAN_POINT('Ctrl Pts',(31.0802839463425,33.7410463011958,53.5576661818291));
#40185=CARTESIAN_POINT('Ctrl Pts',(30.038250683241,32.1717152925075,53.6687959710489));
#40186=CARTESIAN_POINT('Ctrl Pts',(30.7920873980091,30.4449785577687,53.7799257602685));
#40187=CARTESIAN_POINT('Ctrl Pts',(32.6504055030379,30.1418837476604,53.8910555494883));
#40188=CARTESIAN_POINT('Ctrl Pts',(33.9154419463401,31.538310911213,54.002185338708));
#40189=CARTESIAN_POINT('Ctrl Pts',(33.4235043307428,33.3593759834911,54.1133151279278));
#40190=CARTESIAN_POINT('Ctrl Pts',(32.2331222331376,33.7401334029927,54.1874016540742));
#40191=CARTESIAN_POINT('Ctrl Pts',(31.6889203620495,33.6366995627948,54.2244449171475));
#40192=CARTESIAN_POINT('Ctrl Pts',(30.6322193753411,33.1633123698097,40.9251850276175));
#40193=CARTESIAN_POINT('Ctrl Pts',(30.2454185337564,32.7085259251269,40.9622282906908));
#40194=CARTESIAN_POINT('Ctrl Pts',(29.9680635629852,31.3903848820294,41.0363148168373));
#40195=CARTESIAN_POINT('Ctrl Pts',(31.412242767457,29.9594102712082,41.1474446060569));
#40196=CARTESIAN_POINT('Ctrl Pts',(33.3944800559513,30.4008138239409,41.2585743952767));
#40197=CARTESIAN_POINT('Ctrl Pts',(34.1004014126213,32.3034007563114,41.3697041844964));
#40198=CARTESIAN_POINT('Ctrl Pts',(32.8841125683943,33.9295115116003,41.4808339737162));
#40199=CARTESIAN_POINT('Ctrl Pts',(30.8586658139974,33.7891522293869,41.5919637629359));
#40200=CARTESIAN_POINT('Ctrl Pts',(29.8777697255332,32.0116842833717,41.7030935521556));
#40201=CARTESIAN_POINT('Ctrl Pts',(30.8391086984365,30.2233694263251,41.8142233413754));
#40202=CARTESIAN_POINT('Ctrl Pts',(32.8628863731431,30.0610851811797,41.925353130595));
#40203=CARTESIAN_POINT('Ctrl Pts',(34.0969579924684,31.6732355651705,42.0364829198148));
#40204=CARTESIAN_POINT('Ctrl Pts',(33.4119173090442,33.5844570103379,42.1476127090345));
#40205=CARTESIAN_POINT('Ctrl Pts',(31.4347047556197,34.0455905838994,42.2587424982542));
#40206=CARTESIAN_POINT('Ctrl Pts',(29.9748445120241,32.6346268890594,42.369872287474));
#40207=CARTESIAN_POINT('Ctrl Pts',(30.3683844916637,30.6428569964709,42.4810020766937));
#40208=CARTESIAN_POINT('Ctrl Pts',(32.2551613497331,29.893130951746,42.5921318659135));
#40209=CARTESIAN_POINT('Ctrl Pts',(33.9084172776653,31.0715879610168,42.7032616551331));
#40210=CARTESIAN_POINT('Ctrl Pts',(33.815110424141,33.0997179289533,42.8143914443529));
#40211=CARTESIAN_POINT('Ctrl Pts',(32.0606341868485,34.1213978081722,42.9255212335726));
#40212=CARTESIAN_POINT('Ctrl Pts',(30.2506662031655,33.2015975028463,43.0366510227923));
#40213=CARTESIAN_POINT('Ctrl Pts',(30.0416695376591,31.1821081513212,43.147780812012));
#40214=CARTESIAN_POINT('Ctrl Pts',(31.6249156750632,29.9111445714447,43.2589106012318));
#40215=CARTESIAN_POINT('Ctrl Pts',(33.5514349185315,30.5518788162757,43.3700403904515));
#40216=CARTESIAN_POINT('Ctrl Pts',(34.0580977494224,32.5179178696926,43.4811701796712));
#40217=CARTESIAN_POINT('Ctrl Pts',(32.6812118390555,34.0099641025933,43.592299968891));
#40218=CARTESIAN_POINT('Ctrl Pts',(30.680888241084,33.6625129873473,43.7034297581107));
#40219=CARTESIAN_POINT('Ctrl Pts',(29.8878014196687,31.7935480145797,43.8145595473304));
#40220=CARTESIAN_POINT('Ctrl Pts',(31.0277758331491,30.1135256603458,43.9256893365501));
#40221=CARTESIAN_POINT('Ctrl Pts',(33.0575192607911,30.1599841636214,44.0368191257698));
#40222=CARTESIAN_POINT('Ctrl Pts',(34.1194325292802,31.8904052063007,44.1479489149897));
#40223=CARTESIAN_POINT('Ctrl Pts',(33.2416641312585,33.7211262156216,44.2590787042093));
#40224=CARTESIAN_POINT('Ctrl Pts',(31.227538185597,33.9766911772654,44.3702084934291));
#40225=CARTESIAN_POINT('Ctrl Pts',(29.920360915477,32.4232098097874,44.4813382826487));
#40226=CARTESIAN_POINT('Ctrl Pts',(30.516446782766,30.4824114139171,44.5924680718685));
#40227=CARTESIAN_POINT('Ctrl Pts',(32.4702644660027,29.930493634464,44.7035978610882));
#40228=CARTESIAN_POINT('Ctrl Pts',(33.9937012097596,31.2725656378889,44.814727650308));
#40229=CARTESIAN_POINT('Ctrl Pts',(33.6925242271338,33.28037768082,44.9258574395276));
#40230=CARTESIAN_POINT('Ctrl Pts',(31.8423674264961,34.1164019553827,45.0369872287474));
#40231=CARTESIAN_POINT('Ctrl Pts',(30.1364742476751,33.0155181118025,45.1481170179671));
#40232=CARTESIAN_POINT('Ctrl Pts',(30.1360596282866,30.985243105136,45.2592468071869));
#40233=CARTESIAN_POINT('Ctrl Pts',(31.8415030234986,29.8836626040688,45.3703765964065));
#40234=CARTESIAN_POINT('Ctrl Pts',(33.6920011327766,30.7189311370344,45.4815063856263));
#40235=CARTESIAN_POINT('Ctrl Pts',(33.9939981543256,32.7266200007729,45.592636174846));
#40236=CARTESIAN_POINT('Ctrl Pts',(32.4711096890454,34.0693141196697,45.7037659640657));
#40237=CARTESIAN_POINT('Ctrl Pts',(30.5170667453227,33.5181943970221,45.8148957532855));
#40238=CARTESIAN_POINT('Ctrl Pts',(29.9201882345391,31.5776396263525,45.9260255425052));
#40239=CARTESIAN_POINT('Ctrl Pts',(31.226730896886,30.0236244893375,46.0371553317249));
#40240=CARTESIAN_POINT('Ctrl Pts',(33.2409610566485,30.278366786781,46.1482851209446));
#40241=CARTESIAN_POINT('Ctrl Pts',(34.1194771150287,32.1087291306277,46.2594149101644));
#40242=CARTESIAN_POINT('Ctrl Pts',(33.0582707025067,33.8395837532423,46.3705446993841));
#40243=CARTESIAN_POINT('Ctrl Pts',(31.0285464195185,33.8868712743446,46.4816744886038));
#40244=CARTESIAN_POINT('Ctrl Pts',(29.8878859184116,32.2073146674336,46.5928042778236));
#40245=CARTESIAN_POINT('Ctrl Pts',(30.6802093198509,30.3380259251214,46.7039340670433));
#40246=CARTESIAN_POINT('Ctrl Pts',(32.6803908392287,29.9897578327796,46.815063856263));
#40247=CARTESIAN_POINT('Ctrl Pts',(34.0578860410758,31.4812415717095,46.9261936454828));
#40248=CARTESIAN_POINT('Ctrl Pts',(33.5520262549751,33.4474873985099,47.0373234347025));
#40249=CARTESIAN_POINT('Ctrl Pts',(31.6257688713451,34.0890084555412,47.1484532239222));
#40250=CARTESIAN_POINT('Ctrl Pts',(30.0420037582924,32.8186916284146,47.2595830131419));
#40251=CARTESIAN_POINT('Ctrl Pts',(30.2501755720655,30.7991171013039,47.3707128023616));
#40252=CARTESIAN_POINT('Ctrl Pts',(32.0597677262285,29.8785775800472,47.4818425915814));
#40253=CARTESIAN_POINT('Ctrl Pts',(33.8146611055012,30.8995408516631,47.5929723808011));
#40254=CARTESIAN_POINT('Ctrl Pts',(33.9087963201994,32.9276324018544,47.7041021700208));
#40255=CARTESIAN_POINT('Ctrl Pts',(32.2560218426853,34.1067648376231,47.8152319592405));
#40256=CARTESIAN_POINT('Ctrl Pts',(30.3689389511868,33.3578089409124,47.9263617484603));
#40257=CARTESIAN_POINT('Ctrl Pts',(29.9745854434417,31.3662010263035,48.03749153768));
#40258=CARTESIAN_POINT('Ctrl Pts',(31.4338693731524,29.9546390591579,48.1486213268997));
#40259=CARTESIAN_POINT('Ctrl Pts',(33.4112699131231,30.4149692440553,48.2597511161195));
#40260=CARTESIAN_POINT('Ctrl Pts',(34.0970915331884,32.3259023878504,48.3708809053391));
#40261=CARTESIAN_POINT('Ctrl Pts',(32.8636777240904,33.9385732005491,48.482010694559));
#40262=CARTESIAN_POINT('Ctrl Pts',(30.8398354280997,33.7770828430561,48.5931404837786));
#40263=CARTESIAN_POINT('Ctrl Pts',(29.8777631668513,31.9892255392592,48.7042702729984));
#40264=CARTESIAN_POINT('Ctrl Pts',(30.8579390406005,30.211228905088,48.815400062218));
#40265=CARTESIAN_POINT('Ctrl Pts',(32.8833167192567,30.0702961785655,48.9265298514379));
#40266=CARTESIAN_POINT('Ctrl Pts',(34.1002925156201,31.6954074626534,49.0376596406576));
#40267=CARTESIAN_POINT('Ctrl Pts',(33.3951033784119,33.5992785337523,49.1487894298773));
#40268=CARTESIAN_POINT('Ctrl Pts',(31.4131307585472,34.0395072342147,49.259919219097));
#40269=CARTESIAN_POINT('Ctrl Pts',(29.9682545041283,32.6132010314587,49.3710490083168));
#40270=CARTESIAN_POINT('Ctrl Pts',(30.3828096941687,30.6256998946,49.4821787975364));
#40271=CARTESIAN_POINT('Ctrl Pts',(32.2773999144073,29.8959433105394,49.5933085867562));
#40272=CARTESIAN_POINT('Ctrl Pts',(33.9181167412572,31.0917965911284,49.7044383759758));
#40273=CARTESIAN_POINT('Ctrl Pts',(33.8033939276184,33.1188277824609,49.8155681651957));
#40274=CARTESIAN_POINT('Ctrl Pts',(32.0382245484159,34.1219199204672,49.9266979544153));
#40275=CARTESIAN_POINT('Ctrl Pts',(30.2380724770312,33.1830539585253,50.0378277436352));
#40276=CARTESIAN_POINT('Ctrl Pts',(30.0504173673593,31.1614698434269,50.1489575328547));
#40277=CARTESIAN_POINT('Ctrl Pts',(31.6469991407365,29.9072994341435,50.2600873220747));
#40278=CARTESIAN_POINT('Ctrl Pts',(33.5666434723775,30.568345888339,50.3712171112942));
#40279=CARTESIAN_POINT('Ctrl Pts',(34.0525126876382,32.539626659885,50.4823469005141));
#40280=CARTESIAN_POINT('Ctrl Pts',(32.6599445497484,34.0170469643103,50.5934766897337));
#40281=CARTESIAN_POINT('Ctrl Pts',(30.6634023167241,33.648487760965,50.7046064789535));
#40282=CARTESIAN_POINT('Ctrl Pts',(29.8900997886462,31.7712504358846,50.8157362681732));
#40283=CARTESIAN_POINT('Ctrl Pts',(31.0477550530635,30.1033622312073,50.926866057393));
#40284=CARTESIAN_POINT('Ctrl Pts',(33.0768945662916,30.1712563443283,51.0379958466126));
#40285=CARTESIAN_POINT('Ctrl Pts',(34.120471850804,31.912796819262,51.1491256358324));
#40286=CARTESIAN_POINT('Ctrl Pts',(33.2234162931804,33.7341446994465,51.260255425052));
#40287=CARTESIAN_POINT('Ctrl Pts',(31.2067034111182,33.9684221568752,51.3713852142719));
#40288=CARTESIAN_POINT('Ctrl Pts',(29.9160069648852,32.4012210026614,51.4825150034915));
#40289=CARTESIAN_POINT('Ctrl Pts',(30.5325583431829,30.4668267385054,51.5936447927113));
#40290=CARTESIAN_POINT('Ctrl Pts',(32.4920964145184,29.9355760154445,51.7047745819309));
#40291=CARTESIAN_POINT('Ctrl Pts',(34.001273178978,31.2936637377837,51.8159043711508));
#40292=CARTESIAN_POINT('Ctrl Pts',(33.6789064425863,33.2981827424942,51.9270341603704));
#40293=CARTESIAN_POINT('Ctrl Pts',(31.8200227178265,34.1146189892024,52.0381639495902));
#40294=CARTESIAN_POINT('Ctrl Pts',(30.1258522877428,32.9957788498324,52.1492937388099));
#40295=CARTESIAN_POINT('Ctrl Pts',(30.1468814447919,30.9656127439735,52.2604235280297));
#40296=CARTESIAN_POINT('Ctrl Pts',(31.8638647554936,29.8821065619291,52.3715533172493));
#40297=CARTESIAN_POINT('Ctrl Pts',(33.7054372723287,30.7368736361549,52.4826831064692));
#40298=CARTESIAN_POINT('Ctrl Pts',(33.9862126729008,32.7476399648761,52.5938128956888));
#40299=CARTESIAN_POINT('Ctrl Pts',(32.4492266252468,34.074174890882,52.7049426849086));
#40300=CARTESIAN_POINT('Ctrl Pts',(30.5011155176325,33.5024462914775,52.8160724741282));
#40301=CARTESIAN_POINT('Ctrl Pts',(29.9247627281268,31.5556974334801,52.927202263348));
#40302=CARTESIAN_POINT('Ctrl Pts',(31.2476535042578,30.0155649246219,53.0383320525677));
#40303=CARTESIAN_POINT('Ctrl Pts',(33.2590659765762,30.291574867246,53.1494618417874));
#40304=CARTESIAN_POINT('Ctrl Pts',(34.1182298785232,32.1310991651164,53.2605916310072));
#40305=CARTESIAN_POINT('Ctrl Pts',(33.0387435614661,33.850678165931,53.3717214202268));
#40306=CARTESIAN_POINT('Ctrl Pts',(31.0087474085555,33.876466819321,53.4828512094467));
#40307=CARTESIAN_POINT('Ctrl Pts',(29.8856636390453,32.1850714989825,53.5939809986663));
#40308=CARTESIAN_POINT('Ctrl Pts',(30.6981346120899,30.3240272601162,53.7051107878861));
#40309=CARTESIAN_POINT('Ctrl Pts',(32.7009947666045,29.9973573985013,53.8162405771057));
#40310=CARTESIAN_POINT('Ctrl Pts',(34.0644271517501,31.5024002202835,53.9273703663256));
#40311=CARTESIAN_POINT('Ctrl Pts',(33.5342260811582,33.465109759718,54.0385001555452));
#40312=CARTESIAN_POINT('Ctrl Pts',(32.2512547397667,33.8754829148801,54.1125866816917));
#40313=CARTESIAN_POINT('Ctrl Pts',(31.6647242417507,33.7640038755272,54.149629944765));
#40314=CARTESIAN_POINT('Ctrl Pts',(30.5335096305347,33.2472660865709,40.850370055235));
#40315=CARTESIAN_POINT('Ctrl Pts',(30.1187942157535,32.75965869598,40.8874133183083));
#40316=CARTESIAN_POINT('Ctrl Pts',(29.8214231416013,31.3463902884227,40.9614998444548));
#40317=CARTESIAN_POINT('Ctrl Pts',(31.3698256097737,29.812145360628,41.0726296336744));
#40318=CARTESIAN_POINT('Ctrl Pts',(33.4951166404876,30.2854040451424,41.1837594228943));
#40319=CARTESIAN_POINT('Ctrl Pts',(34.2519828019854,32.3252965272338,41.2948892121139));
#40320=CARTESIAN_POINT('Ctrl Pts',(32.9479170443701,34.0687601494867,41.4060190013337));
#40321=CARTESIAN_POINT('Ctrl Pts',(30.7762982148312,33.9182714439734,41.5171487905533));
#40322=CARTESIAN_POINT('Ctrl Pts',(29.7246129948145,32.0125275126214,41.6282785797731));
#40323=CARTESIAN_POINT('Ctrl Pts',(30.7553297048906,30.0951538723239,41.7394083689928));
#40324=CARTESIAN_POINT('Ctrl Pts',(32.9251590008982,29.9211579271181,41.8505381582126));
#40325=CARTESIAN_POINT('Ctrl Pts',(34.2482908777094,31.6496536885213,41.9616679474323));
#40326=CARTESIAN_POINT('Ctrl Pts',(33.5138123021089,33.698803817368,42.072797736652));
#40327=CARTESIAN_POINT('Ctrl Pts',(31.3939086306365,34.1932163952868,42.1839275258717));
#40328=CARTESIAN_POINT('Ctrl Pts',(29.8286934569445,32.6804265276396,42.2950573150915));
#40329=CARTESIAN_POINT('Ctrl Pts',(30.250634358677,30.5449149455827,42.4061871043112));
#40330=CARTESIAN_POINT('Ctrl Pts',(32.2735757878839,29.7410828072231,42.5173168935309));
#40331=CARTESIAN_POINT('Ctrl Pts',(34.0461435906913,31.0045864888574,42.6284466827506));
#40332=CARTESIAN_POINT('Ctrl Pts',(33.946102985033,33.1790821736056,42.7395764719704));
#40333=CARTESIAN_POINT('Ctrl Pts',(32.0650100238815,34.2744944616138,42.8507062611901));
#40334=CARTESIAN_POINT('Ctrl Pts',(30.1244205980196,33.288314174166,42.9618360504099));
#40335=CARTESIAN_POINT('Ctrl Pts',(29.9003410989465,31.1230826802721,43.0729658396295));
#40336=CARTESIAN_POINT('Ctrl Pts',(31.5978466573217,29.7603964305711,43.1840956288493));
#40337=CARTESIAN_POINT('Ctrl Pts',(33.6633985932109,30.4473710685293,43.295225418069));
#40338=CARTESIAN_POINT('Ctrl Pts',(34.2066261756697,32.5552948728657,43.4063552072888));
#40339=CARTESIAN_POINT('Ctrl Pts',(32.7303734118838,34.1550188285196,43.5174849965084));
#40340=CARTESIAN_POINT('Ctrl Pts',(30.5856908221805,33.7824929240125,43.6286147857282));
#40341=CARTESIAN_POINT('Ctrl Pts',(29.7353686544384,31.7786488250253,43.7397445749479));
#40342=CARTESIAN_POINT('Ctrl Pts',(30.9576125352676,29.9773829213026,43.8508743641677));
#40343=CARTESIAN_POINT('Ctrl Pts',(33.1338381195896,30.0271942334423,43.9620041533873));
#40344=CARTESIAN_POINT('Ctrl Pts',(34.2723873528301,31.8824959890453,44.0731339426071));
#40345=CARTESIAN_POINT('Ctrl Pts',(33.3312723237729,33.8453361411468,44.1842637318268));
#40346=CARTESIAN_POINT('Ctrl Pts',(31.1717913010471,34.1193446687329,44.2953935210466));
#40347=CARTESIAN_POINT('Ctrl Pts',(29.770277898053,32.4537519388178,44.4065233102662));
#40348=CARTESIAN_POINT('Ctrl Pts',(30.4093819824319,30.372890355238,44.5176530994861));
#40349=CARTESIAN_POINT('Ctrl Pts',(32.5042024269548,29.7811418732718,44.6287828887057));
#40350=CARTESIAN_POINT('Ctrl Pts',(34.1375822781764,31.2200682863745,44.7399126779255));
#40351=CARTESIAN_POINT('Ctrl Pts',(33.8146700095254,33.3727797457791,44.8510424671451));
#40352=CARTESIAN_POINT('Ctrl Pts',(31.8309914274337,34.2691380690237,44.9621722563649));
#40353=CARTESIAN_POINT('Ctrl Pts',(30.0019876581329,33.0888058392751,45.0733020455846));
#40354=CARTESIAN_POINT('Ctrl Pts',(30.0015431165673,30.9120103130298,45.1844318348044));
#40355=CARTESIAN_POINT('Ctrl Pts',(31.8300646423569,29.7309311495427,45.2955616240241));
#40356=CARTESIAN_POINT('Ctrl Pts',(33.8141091645892,30.6264791909671,45.4066914132438));
#40357=CARTESIAN_POINT('Ctrl Pts',(34.1379006525841,32.7790585816055,45.5178212024635));
#40358=CARTESIAN_POINT('Ctrl Pts',(32.5051086479012,34.2186520068971,45.6289509916833));
#40359=CARTESIAN_POINT('Ctrl Pts',(30.4100466863343,33.6277591757555,45.740080780903));
#40360=CARTESIAN_POINT('Ctrl Pts',(29.7700927551085,31.5471587992758,45.8512105701227));
#40361=CARTESIAN_POINT('Ctrl Pts',(31.1709257520704,29.8809937788405,45.9623403593425));
#40362=CARTESIAN_POINT('Ctrl Pts',(33.3305185098015,30.1541202723448,46.0734701485622));
#40363=CARTESIAN_POINT('Ctrl Pts',(34.2724351562348,32.1165758748671,46.1845999377819));
#40364=CARTESIAN_POINT('Ctrl Pts',(33.134643791215,33.9723425009238,46.2957297270016));
#40365=CARTESIAN_POINT('Ctrl Pts',(30.9584387331748,34.0230426592987,46.4068595162213));
#40366=CARTESIAN_POINT('Ctrl Pts',(29.7354592512714,32.2222761148676,46.5179893054411));
#40367=CARTESIAN_POINT('Ctrl Pts',(30.5849629046826,30.2180848805937,46.6291190946608));
#40368=CARTESIAN_POINT('Ctrl Pts',(32.72949316229,29.8446830395357,46.7402488838805));
#40369=CARTESIAN_POINT('Ctrl Pts',(34.2063991887935,31.4438039072554,46.8513786731003));
#40370=CARTESIAN_POINT('Ctrl Pts',(33.6640326051161,33.5519494073595,46.96250846232));
#40371=CARTESIAN_POINT('Ctrl Pts',(31.5987614269185,34.2397676400387,47.0736382515397));
#40372=CARTESIAN_POINT('Ctrl Pts',(29.9006994395541,32.8777748178231,47.1847680407595));
#40373=CARTESIAN_POINT('Ctrl Pts',(30.1238945591431,30.7124520014073,47.2958978299791));
#40374=CARTESIAN_POINT('Ctrl Pts',(32.0640810326881,29.725479150427,47.4070276191989));
#40375=CARTESIAN_POINT('Ctrl Pts',(33.9456212400468,30.8201231148243,47.5181574084186));
#40376=CARTESIAN_POINT('Ctrl Pts',(34.0465499878984,32.9945776093026,47.6292871976383));
#40377=CARTESIAN_POINT('Ctrl Pts',(32.2744983807359,34.258805461492,47.7404169868581));
#40378=CARTESIAN_POINT('Ctrl Pts',(30.2512288323348,33.4557990510493,47.8515467760777));
#40379=CARTESIAN_POINT('Ctrl Pts',(29.8284156919473,31.3204611365695,47.9626765652976));
#40380=CARTESIAN_POINT('Ctrl Pts',(31.3930129604384,29.8070298206093,48.0738063545172));
#40381=CARTESIAN_POINT('Ctrl Pts',(33.513118185036,30.300581031056,48.184936143737));
#40382=CARTESIAN_POINT('Ctrl Pts',(34.2484340557719,32.3494220524491,48.2960659329567));
#40383=CARTESIAN_POINT('Ctrl Pts',(32.9260074619175,34.0784758007651,48.4071957221765));
#40384=CARTESIAN_POINT('Ctrl Pts',(30.7561088810489,33.9053310363523,48.5183255113961));
#40385=CARTESIAN_POINT('Ctrl Pts',(29.7246059628069,31.9884479699246,48.6294553006159));
#40386=CARTESIAN_POINT('Ctrl Pts',(30.7755189917832,30.0821371961453,48.7405850898356));
#40387=CARTESIAN_POINT('Ctrl Pts',(32.9470637605359,29.9310336620978,48.8517148790554));
#40388=CARTESIAN_POINT('Ctrl Pts',(34.251866046125,31.6734256834927,48.962844668275));
#40389=CARTESIAN_POINT('Ctrl Pts',(33.4957849467709,33.7146949778041,49.0739744574948));
#40390=CARTESIAN_POINT('Ctrl Pts',(31.3707776852443,34.1866940235219,49.1851042467145));
#40391=CARTESIAN_POINT('Ctrl Pts',(29.8216278625503,32.6574544126216,49.2962340359343));
#40392=CARTESIAN_POINT('Ctrl Pts',(30.2661005965881,30.5265196530863,49.4073638251539));
#40393=CARTESIAN_POINT('Ctrl Pts',(32.2974192612725,29.7440981278174,49.5184936143737));
#40394=CARTESIAN_POINT('Ctrl Pts',(34.0565430434178,31.0262535317329,49.6296234035934));
#40395=CARTESIAN_POINT('Ctrl Pts',(33.9335409345078,33.1995711435658,49.7407531928132));
#40396=CARTESIAN_POINT('Ctrl Pts',(32.0409831307145,34.2750542536145,49.8518829820329));
#40397=CARTESIAN_POINT('Ctrl Pts',(30.1109180101348,33.2684323826914,49.9630127712527));
#40398=CARTESIAN_POINT('Ctrl Pts',(29.9097202404387,31.1009549507053,50.0741425604723));
#40399=CARTESIAN_POINT('Ctrl Pts',(31.6215238385528,29.7562737980964,50.1852723496921));
#40400=CARTESIAN_POINT('Ctrl Pts',(33.6797047152209,30.4650265332718,50.2964021389118));
#40401=CARTESIAN_POINT('Ctrl Pts',(34.2006380521566,32.5785703391035,50.4075319281315));
#40402=CARTESIAN_POINT('Ctrl Pts',(32.7075713086873,34.1626128449203,50.5186617173513));
#40403=CARTESIAN_POINT('Ctrl Pts',(30.5669429767931,33.7674555276286,50.6297915065709));
#40404=CARTESIAN_POINT('Ctrl Pts',(29.7378328916927,31.7547420787026,50.7409212957907));
#40405=CARTESIAN_POINT('Ctrl Pts',(30.9790336119123,29.9664860196478,50.8520510850104));
#40406=CARTESIAN_POINT('Ctrl Pts',(33.1546116986341,30.0392799028483,50.9631808742301));
#40407=CARTESIAN_POINT('Ctrl Pts',(34.2735016799217,31.906503555882,51.0743106634499));
#40408=CARTESIAN_POINT('Ctrl Pts',(33.3117075790158,33.8592941405585,51.1854404526696));
#40409=CARTESIAN_POINT('Ctrl Pts',(31.1494529263309,34.1104788911743,51.2965702418893));
#40410=CARTESIAN_POINT('Ctrl Pts',(29.7656097323423,32.4301762474351,51.4077000311091));
#40411=CARTESIAN_POINT('Ctrl Pts',(30.4266562790277,30.3561809677892,51.5188298203287));
#40412=CARTESIAN_POINT('Ctrl Pts',(32.5276099395835,29.7865910386039,51.6299596095486));
#40413=CARTESIAN_POINT('Ctrl Pts',(34.1457006999001,31.2426889901276,51.7410893987682));
#40414=CARTESIAN_POINT('Ctrl Pts',(33.8000694591651,33.3918697599249,51.852219187988));
#40415=CARTESIAN_POINT('Ctrl Pts',(31.807034149869,34.2672264300624,51.9633489772076));
#40416=CARTESIAN_POINT('Ctrl Pts',(29.9905991345169,33.0676420378163,52.0744787664275));
#40417=CARTESIAN_POINT('Ctrl Pts',(30.0131459199694,30.8909632715124,52.1856085556471));
#40418=CARTESIAN_POINT('Ctrl Pts',(31.8540401717833,29.7292628112352,52.2967383448669));
#40419=CARTESIAN_POINT('Ctrl Pts',(33.8285149610311,30.6457165611199,52.4078681340866));
#40420=CARTESIAN_POINT('Ctrl Pts',(34.1295533099436,32.8015955106775,52.5189979233063));
#40421=CARTESIAN_POINT('Ctrl Pts',(32.4816463311111,34.2238635693672,52.630127712526));
#40422=CARTESIAN_POINT('Ctrl Pts',(30.3929442933283,33.6108745637776,52.7412575017457));
#40423=CARTESIAN_POINT('Ctrl Pts',(29.7749973799223,31.5236330861956,52.8523872909655));
#40424=CARTESIAN_POINT('Ctrl Pts',(31.1933582983878,29.8723525729158,52.9635170801853));
#40425=CARTESIAN_POINT('Ctrl Pts',(33.349930022317,30.1682815511726,53.0746468694049));
#40426=CARTESIAN_POINT('Ctrl Pts',(34.2710979093908,32.14056030596,53.1857766586248));
#40427=CARTESIAN_POINT('Ctrl Pts',(33.1137074189905,33.9842375731813,53.2969064478443));
#40428=CARTESIAN_POINT('Ctrl Pts',(30.9372108707685,34.0118873374463,53.4080362370642));
#40429=CARTESIAN_POINT('Ctrl Pts',(29.7330765948496,32.1984277054576,53.5191660262838));
#40430=CARTESIAN_POINT('Ctrl Pts',(30.6041818261707,30.2030759624636,53.6302958155036));
#40431=CARTESIAN_POINT('Ctrl Pts',(32.7515840301711,29.8528310493422,53.7414256047234));
#40432=CARTESIAN_POINT('Ctrl Pts',(34.2134123571603,31.4664895293539,53.852555393943));
#40433=CARTESIAN_POINT('Ctrl Pts',(33.6449478315736,33.5708435359449,53.9636851831628));
#40434=CARTESIAN_POINT('Ctrl Pts',(32.2693872463958,34.0108324267675,54.0377717093093));
#40435=CARTESIAN_POINT('Ctrl Pts',(31.640528121452,33.8913081882596,54.0748149723825));
#40436=CARTESIAN_POINT('Ctrl Pts',(30.4347998857282,33.3312198033321,40.7755550828525));
#40437=CARTESIAN_POINT('Ctrl Pts',(29.9921698977506,32.8107914668331,40.8125983459258));
#40438=CARTESIAN_POINT('Ctrl Pts',(29.6747827202174,31.3023956948159,40.8866848720723));
#40439=CARTESIAN_POINT('Ctrl Pts',(31.3274084520903,29.6648804500478,40.9978146612919));
#40440=CARTESIAN_POINT('Ctrl Pts',(33.595753225024,30.1699942663438,41.1089444505117));
#40441=CARTESIAN_POINT('Ctrl Pts',(34.4035641913493,32.3471922981561,41.2200742397314));
#40442=CARTESIAN_POINT('Ctrl Pts',(33.0117215203461,34.2080087873732,41.3312040289512));
#40443=CARTESIAN_POINT('Ctrl Pts',(30.693930615665,34.0473906585599,41.4423338181709));
#40444=CARTESIAN_POINT('Ctrl Pts',(29.5714562640958,32.0133707418711,41.5534636073906));
#40445=CARTESIAN_POINT('Ctrl Pts',(30.6715507113449,29.9669383183226,41.6645933966104));
#40446=CARTESIAN_POINT('Ctrl Pts',(32.9874316286532,29.7812306730564,41.7757231858301));
#40447=CARTESIAN_POINT('Ctrl Pts',(34.3996237629505,31.6260718118722,41.8868529750498));
#40448=CARTESIAN_POINT('Ctrl Pts',(33.6157072951735,33.8131506243979,41.9979827642696));
#40449=CARTESIAN_POINT('Ctrl Pts',(31.3531125056534,34.3408422066741,42.1091125534892));
#40450=CARTESIAN_POINT('Ctrl Pts',(29.6825424018648,32.7262261662198,42.220242342709));
#40451=CARTESIAN_POINT('Ctrl Pts',(30.1328842256904,30.4469728946945,42.3313721319287));
#40452=CARTESIAN_POINT('Ctrl Pts',(32.2919902260347,29.5890346627002,42.4425019211484));
#40453=CARTESIAN_POINT('Ctrl Pts',(34.1838699037172,30.9375850166979,42.5536317103681));
#40454=CARTESIAN_POINT('Ctrl Pts',(34.0770955459249,33.2584464182579,42.6647614995879));
#40455=CARTESIAN_POINT('Ctrl Pts',(32.0693858609145,34.4275911150555,42.7758912888076));
#40456=CARTESIAN_POINT('Ctrl Pts',(29.9981749928738,33.3750308454857,42.8870210780274));
#40457=CARTESIAN_POINT('Ctrl Pts',(29.7590126602339,31.0640572092229,42.9981508672471));
#40458=CARTESIAN_POINT('Ctrl Pts',(31.5707776395802,29.6096482896975,43.1092806564668));
#40459=CARTESIAN_POINT('Ctrl Pts',(33.7753622678902,30.3428633207829,43.2204104456866));
#40460=CARTESIAN_POINT('Ctrl Pts',(34.3551546019171,32.5926718760388,43.3315402349062));
#40461=CARTESIAN_POINT('Ctrl Pts',(32.7795349847121,34.3000735544458,43.442670024126));
#40462=CARTESIAN_POINT('Ctrl Pts',(30.490493403277,33.9024728606777,43.5537998133457));
#40463=CARTESIAN_POINT('Ctrl Pts',(29.5829358892083,31.763749635471,43.6649296025654));
#40464=CARTESIAN_POINT('Ctrl Pts',(30.887449237386,29.8412401822595,43.7760593917852));
#40465=CARTESIAN_POINT('Ctrl Pts',(33.2101569783881,29.8944043032633,43.8871891810048));
#40466=CARTESIAN_POINT('Ctrl Pts',(34.42534217638,31.8745867717898,43.9983189702247));
#40467=CARTESIAN_POINT('Ctrl Pts',(33.4208805162873,33.9695460666721,44.1094487594443));
#40468=CARTESIAN_POINT('Ctrl Pts',(31.1160444164971,34.2619981602002,44.2205785486641));
#40469=CARTESIAN_POINT('Ctrl Pts',(29.6201948806291,32.4842940678484,44.3317083378838));
#40470=CARTESIAN_POINT('Ctrl Pts',(30.3023171820977,30.2633692965589,44.4428381271035));
#40471=CARTESIAN_POINT('Ctrl Pts',(32.5381403879069,29.6317901120796,44.5539679163233));
#40472=CARTESIAN_POINT('Ctrl Pts',(34.2814633465932,31.16757093486,44.6650977055429));
#40473=CARTESIAN_POINT('Ctrl Pts',(33.9368157919171,33.4651818107383,44.7762274947627));
#40474=CARTESIAN_POINT('Ctrl Pts',(31.8196154283712,34.4218741826645,44.8873572839824));
#40475=CARTESIAN_POINT('Ctrl Pts',(29.8675010685907,33.1620935667478,44.9984870732022));
#40476=CARTESIAN_POINT('Ctrl Pts',(29.8670266048481,30.8387775209235,45.1096168624218));
#40477=CARTESIAN_POINT('Ctrl Pts',(31.8186262612152,29.5781996950166,45.2207466516417));
#40478=CARTESIAN_POINT('Ctrl Pts',(33.9362171964019,30.5340272448998,45.3318764408613));
#40479=CARTESIAN_POINT('Ctrl Pts',(34.2818031508426,32.8314971624382,45.4430062300811));
#40480=CARTESIAN_POINT('Ctrl Pts',(32.539107606757,34.3679898941243,45.5541360193008));
#40481=CARTESIAN_POINT('Ctrl Pts',(30.3030266273459,33.737323954489,45.6652658085205));
#40482=CARTESIAN_POINT('Ctrl Pts',(29.6199972756779,31.516677972199,45.7763955977403));
#40483=CARTESIAN_POINT('Ctrl Pts',(31.1151206072547,29.7383630683434,45.88752538696));
#40484=CARTESIAN_POINT('Ctrl Pts',(33.4200759629546,30.0298737579086,45.9986551761796));
#40485=CARTESIAN_POINT('Ctrl Pts',(34.425393197441,32.1244226191065,46.1097849653995));
#40486=CARTESIAN_POINT('Ctrl Pts',(33.2110168799234,34.1051012486052,46.2209147546191));
#40487=CARTESIAN_POINT('Ctrl Pts',(30.8883310468311,34.1592140442528,46.3320445438389));
#40488=CARTESIAN_POINT('Ctrl Pts',(29.5830325841312,32.2372375623016,46.4431743330585));
#40489=CARTESIAN_POINT('Ctrl Pts',(30.4897164895143,30.0981438360661,46.5543041222784));
#40490=CARTESIAN_POINT('Ctrl Pts',(32.7785954853513,29.6996082462917,46.665433911498));
#40491=CARTESIAN_POINT('Ctrl Pts',(34.3549123365112,31.4063662428014,46.7765637007178));
#40492=CARTESIAN_POINT('Ctrl Pts',(33.776038955257,33.6564114162091,46.8876934899375));
#40493=CARTESIAN_POINT('Ctrl Pts',(31.571753982492,34.3905268245362,46.9988232791573));
#40494=CARTESIAN_POINT('Ctrl Pts',(29.7593951208157,32.9368580072316,47.1099530683769));
#40495=CARTESIAN_POINT('Ctrl Pts',(29.9976135462207,30.6257869015107,47.2210828575967));
#40496=CARTESIAN_POINT('Ctrl Pts',(32.0683943391477,29.5723807208067,47.3322126468164));
#40497=CARTESIAN_POINT('Ctrl Pts',(34.0765813745924,30.7407053779857,47.4433424360362));
#40498=CARTESIAN_POINT('Ctrl Pts',(34.1843036555974,33.0615228167506,47.5544722252558));
#40499=CARTESIAN_POINT('Ctrl Pts',(32.2929749187864,34.410846085361,47.6656020144756));
#40500=CARTESIAN_POINT('Ctrl Pts',(30.1335187134828,33.5537891611861,47.7767318036953));
#40501=CARTESIAN_POINT('Ctrl Pts',(29.682245940453,31.2747212468355,47.8878615929151));
#40502=CARTESIAN_POINT('Ctrl Pts',(31.3521565477245,29.6594205820605,47.9989913821348));
#40503=CARTESIAN_POINT('Ctrl Pts',(33.6149664569488,30.1861928180569,48.1101211713545));
#40504=CARTESIAN_POINT('Ctrl Pts',(34.3997765783555,32.3729417170477,48.2212509605742));
#40505=CARTESIAN_POINT('Ctrl Pts',(32.9883371997446,34.2183784009811,48.3323807497939));
#40506=CARTESIAN_POINT('Ctrl Pts',(30.672382333998,34.0335792296485,48.4435105390137));
#40507=CARTESIAN_POINT('Ctrl Pts',(29.5714487587624,31.98767040059,48.5546403282333));
#40508=CARTESIAN_POINT('Ctrl Pts',(30.6930989429659,29.9530454872026,48.6657701174531));
#40509=CARTESIAN_POINT('Ctrl Pts',(33.0108108018152,29.7917711456301,48.7768999066728));
#40510=CARTESIAN_POINT('Ctrl Pts',(34.40343957663,31.6514439043321,48.8880296958926));
#40511=CARTESIAN_POINT('Ctrl Pts',(33.5964665151298,33.830111421856,48.9991594851123));
#40512=CARTESIAN_POINT('Ctrl Pts',(31.3284246119414,34.3338808128292,49.1102892743321));
#40513=CARTESIAN_POINT('Ctrl Pts',(29.6750012209723,32.7017077937846,49.2214190635517));
#40514=CARTESIAN_POINT('Ctrl Pts',(30.1493914990076,30.4273394115725,49.3325488527715));
#40515=CARTESIAN_POINT('Ctrl Pts',(32.3174386081376,29.5922529450954,49.4436786419912));
#40516=CARTESIAN_POINT('Ctrl Pts',(34.1949693455785,30.9607104723374,49.554808431211));
#40517=CARTESIAN_POINT('Ctrl Pts',(34.0636879413972,33.2803145046706,49.6659382204306));
#40518=CARTESIAN_POINT('Ctrl Pts',(32.0437417130131,34.4281885867619,49.7770680096504));
#40519=CARTESIAN_POINT('Ctrl Pts',(29.9837635432384,33.3538108068575,49.8881977988701));
#40520=CARTESIAN_POINT('Ctrl Pts',(29.7690231135183,31.0404400579838,49.9993275880899));
#40521=CARTESIAN_POINT('Ctrl Pts',(31.5960485363689,29.6052481620493,50.1104573773095));
#40522=CARTESIAN_POINT('Ctrl Pts',(33.7927659580644,30.3617071782046,50.2215871665294));
#40523=CARTESIAN_POINT('Ctrl Pts',(34.348763416675,32.617514018322,50.3327169557489));
#40524=CARTESIAN_POINT('Ctrl Pts',(32.7551980676263,34.3081787255302,50.4438467449689));
#40525=CARTESIAN_POINT('Ctrl Pts',(30.4704836368621,33.8864232942922,50.5549765341884));
#40526=CARTESIAN_POINT('Ctrl Pts',(29.5855659947393,31.7382337215207,50.6661063234083));
#40527=CARTESIAN_POINT('Ctrl Pts',(30.910312170761,29.8296098080883,50.7772361126278));
#40528=CARTESIAN_POINT('Ctrl Pts',(33.2323288309766,29.9073034613682,50.8883659018477));
#40529=CARTESIAN_POINT('Ctrl Pts',(34.4265315090395,31.9002102925021,50.9994956910673));
#40530=CARTESIAN_POINT('Ctrl Pts',(33.3999988648512,33.9844435816704,51.1106254802872));
#40531=CARTESIAN_POINT('Ctrl Pts',(31.0922024415436,34.2525356254733,51.2217552695068));
#40532=CARTESIAN_POINT('Ctrl Pts',(29.6152124997993,32.4591314922087,51.3328850587266));
#40533=CARTESIAN_POINT('Ctrl Pts',(30.3207542148726,30.2455351970729,51.4440148479463));
#40534=CARTESIAN_POINT('Ctrl Pts',(32.5631234646485,29.6376060617633,51.5551446371661));
#40535=CARTESIAN_POINT('Ctrl Pts',(34.2901282208224,31.1917142424714,51.6662744263857));
#40536=CARTESIAN_POINT('Ctrl Pts',(33.9212324757437,33.4855567773556,51.7774042156055));
#40537=CARTESIAN_POINT('Ctrl Pts',(31.7940455819115,34.4198338709223,51.8885340048252));
#40538=CARTESIAN_POINT('Ctrl Pts',(29.8553459812909,33.1395052258002,51.9996637940449));
#40539=CARTESIAN_POINT('Ctrl Pts',(29.879410395147,30.8163137990511,52.1107935832647));
#40540=CARTESIAN_POINT('Ctrl Pts',(31.8442155880729,29.5764190605415,52.2219233724844));
#40541=CARTESIAN_POINT('Ctrl Pts',(33.9515926497335,30.5545594860849,52.3330531617041));
#40542=CARTESIAN_POINT('Ctrl Pts',(34.2728939469864,32.8555510564788,52.4441829509239));
#40543=CARTESIAN_POINT('Ctrl Pts',(32.5140660369754,34.3735522478524,52.5553127401435));
#40544=CARTESIAN_POINT('Ctrl Pts',(30.2847730690242,33.7193028360775,52.6664425293633));
#40545=CARTESIAN_POINT('Ctrl Pts',(29.6252320317178,31.4915687389112,52.7775723185829));
#40546=CARTESIAN_POINT('Ctrl Pts',(31.1390630925179,29.7291402212096,52.8887021078028));
#40547=CARTESIAN_POINT('Ctrl Pts',(33.4407940680577,30.0449882350993,52.9998318970224));
#40548=CARTESIAN_POINT('Ctrl Pts',(34.4239659402583,32.1500214468035,53.1109616862423));
#40549=CARTESIAN_POINT('Ctrl Pts',(33.188671276515,34.1177969804317,53.2220914754619));
#40550=CARTESIAN_POINT('Ctrl Pts',(30.8656743329815,34.1473078555715,53.3332212646817));
#40551=CARTESIAN_POINT('Ctrl Pts',(29.5804895506539,32.2117839119326,53.4443510539014));
#40552=CARTESIAN_POINT('Ctrl Pts',(30.5102290402516,30.0821246648111,53.5554808431211));
#40553=CARTESIAN_POINT('Ctrl Pts',(32.8021732937378,29.7083047001831,53.6666106323408));
#40554=CARTESIAN_POINT('Ctrl Pts',(34.3623975625704,31.4305788384244,53.7777404215606));
#40555=CARTESIAN_POINT('Ctrl Pts',(33.755669581989,33.6765773121718,53.8888702107803));
#40556=CARTESIAN_POINT('Ctrl Pts',(32.2875197530249,34.146181938655,53.9629567369268));
#40557=CARTESIAN_POINT('Ctrl Pts',(31.6163320011532,34.0186125009919,54.));
#40558=CARTESIAN_POINT('Ctrl Pts',(30.7309291201476,33.0793586530485,41.));
#40559=CARTESIAN_POINT('Ctrl Pts',(30.6855978938826,33.0370694300904,41.));
#40560=CARTESIAN_POINT('Ctrl Pts',(30.6429965450219,32.9922112417457,41.));
#40561=CARTESIAN_POINT('Ctrl Pts',(30.6031236806187,32.9451290731506,41.));
#40562=CARTESIAN_POINT('Ctrl Pts',(30.5606226882341,32.8949435919002,41.));
#40563=CARTESIAN_POINT('Ctrl Pts',(30.5212209933767,32.8422310572396,41.));
#40564=CARTESIAN_POINT('Ctrl Pts',(30.4849457305127,32.787354565294,41.));
#40565=CARTESIAN_POINT('Ctrl Pts',(30.4532048755067,32.7393376348417,41.));
#40566=CARTESIAN_POINT('Ctrl Pts',(30.4238579381761,32.6896626994178,41.));
#40567=CARTESIAN_POINT('Ctrl Pts',(30.3969459826243,32.6385454586234,41.));
#40568=CARTESIAN_POINT('Ctrl Pts',(30.3834464248084,32.6129040612093,41.));
#40569=CARTESIAN_POINT('Ctrl Pts',(30.3705599224503,32.5868993924579,41.));
#40570=CARTESIAN_POINT('Ctrl Pts',(30.3582939988302,32.560556837428,41.));
#40571=CARTESIAN_POINT('Ctrl Pts',(30.3526828221897,32.5485061566953,41.));
#40572=CARTESIAN_POINT('Ctrl Pts',(30.3472009327832,32.5363830748729,41.));
#40573=CARTESIAN_POINT('Ctrl Pts',(30.3418575717771,32.5242099978175,41.));
#40574=CARTESIAN_POINT('Ctrl Pts',(30.314936000612,32.4628781207701,41.));
#40575=CARTESIAN_POINT('Ctrl Pts',(30.2914757060973,32.4001707948082,41.));
#40576=CARTESIAN_POINT('Ctrl Pts',(30.2715002890511,32.3364457257782,41.));
#40577=CARTESIAN_POINT('Ctrl Pts',(30.2511708530155,32.2715912743439,41.));
#40578=CARTESIAN_POINT('Ctrl Pts',(30.2344503545547,32.2056818443951,41.));
#40579=CARTESIAN_POINT('Ctrl Pts',(30.2214029865264,32.139057988802,41.));
#40580=CARTESIAN_POINT('Ctrl Pts',(30.2104913962594,32.0833400683238,41.));
#40581=CARTESIAN_POINT('Ctrl Pts',(30.2021493761013,32.0271215322105,41.));
#40582=CARTESIAN_POINT('Ctrl Pts',(30.1964392904162,31.9705892943722,41.));
#40583=CARTESIAN_POINT('Ctrl Pts',(30.1938095119973,31.9445533875158,41.));
#40584=CARTESIAN_POINT('Ctrl Pts',(30.1917383177404,31.918450829594,41.));
#40585=CARTESIAN_POINT('Ctrl Pts',(30.1902336001224,31.8922994784363,41.));
#40586=CARTESIAN_POINT('Ctrl Pts',(30.1895755650056,31.8808631084452,41.));
#40587=CARTESIAN_POINT('Ctrl Pts',(30.1890259817236,31.8694175972641,41.));
#40588=CARTESIAN_POINT('Ctrl Pts',(30.1885858466957,31.8579786000936,41.));
#40589=CARTESIAN_POINT('Ctrl Pts',(30.1858876893862,31.7878541794764,41.));
#40590=CARTESIAN_POINT('Ctrl Pts',(30.1872904995807,31.7178431873908,41.));
#40591=CARTESIAN_POINT('Ctrl Pts',(30.1928490020739,31.6483063267634,41.));
#40592=CARTESIAN_POINT('Ctrl Pts',(30.1978163879672,31.5861643342093,41.));
#40593=CARTESIAN_POINT('Ctrl Pts',(30.206102944145,31.5244000293923,41.));
#40594=CARTESIAN_POINT('Ctrl Pts',(30.2177808112143,31.4632587210937,41.));
#40595=CARTESIAN_POINT('Ctrl Pts',(30.2305088547194,31.3966190490231,41.));
#40596=CARTESIAN_POINT('Ctrl Pts',(30.2472644984874,31.3307186298758,41.));
#40597=CARTESIAN_POINT('Ctrl Pts',(30.2678024552877,31.2657711075514,41.));
#40598=CARTESIAN_POINT('Ctrl Pts',(30.2757346768809,31.2406869112988,41.));
#40599=CARTESIAN_POINT('Ctrl Pts',(30.2842316526018,31.2157449037212,41.));
#40600=CARTESIAN_POINT('Ctrl Pts',(30.2932812639676,31.1909577139282,41.));
#40601=CARTESIAN_POINT('Ctrl Pts',(30.2972497295957,31.180087953147,41.));
#40602=CARTESIAN_POINT('Ctrl Pts',(30.3013243722381,31.1692485178295,41.));
#40603=CARTESIAN_POINT('Ctrl Pts',(30.3054990763298,31.158453031983,41.));
#40604=CARTESIAN_POINT('Ctrl Pts',(30.3307217120053,31.0932291022217,41.));
#40605=CARTESIAN_POINT('Ctrl Pts',(30.3596352637442,31.0294901920278,41.));
#40606=CARTESIAN_POINT('Ctrl Pts',(30.3919270267659,30.9674551823789,41.));
#40607=CARTESIAN_POINT('Ctrl Pts',(30.4249671644409,30.9039824863203,41.));
#40608=CARTESIAN_POINT('Ctrl Pts',(30.4615442128327,30.8422927637179,41.));
#40609=CARTESIAN_POINT('Ctrl Pts',(30.5013793582913,30.7826241753209,41.));
#40610=CARTESIAN_POINT('Ctrl Pts',(30.5318853054709,30.7369296815525,41.));
#40611=CARTESIAN_POINT('Ctrl Pts',(30.5643032022178,30.6924204631662,41.));
#40612=CARTESIAN_POINT('Ctrl Pts',(30.5985274068616,30.6492095916093,41.));
#40613=CARTESIAN_POINT('Ctrl Pts',(30.6198360174704,30.62230571917,41.));
#40614=CARTESIAN_POINT('Ctrl Pts',(30.6418451736476,30.5959052782455,41.));
#40615=CARTESIAN_POINT('Ctrl Pts',(30.6645322910513,30.5700372527086,41.));
#40616=CARTESIAN_POINT('Ctrl Pts',(30.6771876348299,30.555607532519,41.));
#40617=CARTESIAN_POINT('Ctrl Pts',(30.6900583764597,30.5413389753362,41.));
#40618=CARTESIAN_POINT('Ctrl Pts',(30.7031169971451,30.5272619247055,41.));
#40619=CARTESIAN_POINT('Ctrl Pts',(30.7539897854241,30.4724216139574,41.));
#40620=CARTESIAN_POINT('Ctrl Pts',(30.8077591398318,30.4204262274082,41.));
#40621=CARTESIAN_POINT('Ctrl Pts',(30.8641400445596,30.3715397784649,41.));
#40622=CARTESIAN_POINT('Ctrl Pts',(30.9062939887424,30.3349891652741,41.));
#40623=CARTESIAN_POINT('Ctrl Pts',(30.9499089479774,30.3001766489696,41.));
#40624=CARTESIAN_POINT('Ctrl Pts',(30.9948821813454,30.2672223105979,41.));
#40625=CARTESIAN_POINT('Ctrl Pts',(31.0089663888168,30.2569020444318,41.));
#40626=CARTESIAN_POINT('Ctrl Pts',(31.0231839012869,30.2467640954187,41.));
#40627=CARTESIAN_POINT('Ctrl Pts',(31.0375318056939,30.2368123795939,41.));
#40628=CARTESIAN_POINT('Ctrl Pts',(31.0513138251944,30.2272531619083,41.));
#40629=CARTESIAN_POINT('Ctrl Pts',(31.0652090979386,30.2178707336406,41.));
#40630=CARTESIAN_POINT('Ctrl Pts',(31.0792097070466,30.208671281042,41.));
#40631=CARTESIAN_POINT('Ctrl Pts',(31.1421653556993,30.167304687551,41.));
#40632=CARTESIAN_POINT('Ctrl Pts',(31.2072783160395,30.1296140175869,41.));
#40633=CARTESIAN_POINT('Ctrl Pts',(31.2742872364057,30.0958785366594,41.));
#40634=CARTESIAN_POINT('Ctrl Pts',(31.3254776883888,30.0701068258617,41.));
#40635=CARTESIAN_POINT('Ctrl Pts',(31.3777755899145,30.0466437584942,41.));
#40636=CARTESIAN_POINT('Ctrl Pts',(31.4310782545421,30.0256290548068,41.));
#40637=CARTESIAN_POINT('Ctrl Pts',(31.4435633682323,30.0207067687159,41.));
#40638=CARTESIAN_POINT('Ctrl Pts',(31.4561036516355,30.0159188770397,41.));
#40639=CARTESIAN_POINT('Ctrl Pts',(31.4686971487471,30.0112647854283,41.));
#40640=CARTESIAN_POINT('Ctrl Pts',(33.6673070786563,31.998696213291,42.1285196366098));
#40641=CARTESIAN_POINT('Ctrl Pts',(33.6680432869609,31.9130463841536,42.1227790551389));
#40642=CARTESIAN_POINT('Ctrl Pts',(33.6620132262641,31.8275005565021,42.1170384736681));
#40643=CARTESIAN_POINT('Ctrl Pts',(33.6488560817129,31.7430654009713,42.1112978921973));
#40644=CARTESIAN_POINT('Ctrl Pts',(33.563954653281,31.1982157729602,42.074254629124));
#40645=CARTESIAN_POINT('Ctrl Pts',(33.1822841993345,30.6996141041007,42.0372113660508));
#40646=CARTESIAN_POINT('Ctrl Pts',(32.678494630127,30.4754086938519,42.0001681029775));
#40647=CARTESIAN_POINT('Ctrl Pts',(32.1747050609195,30.251203283603,41.9631248399043));
#40648=CARTESIAN_POINT('Ctrl Pts',(31.5487963764509,30.3013941319647,41.9260815768311));
#40649=CARTESIAN_POINT('Ctrl Pts',(31.0871818282615,30.6030322351115,41.8890383137578));
#40650=CARTESIAN_POINT('Ctrl Pts',(30.6255672800722,30.9046703382582,41.8519950506846));
#40651=CARTESIAN_POINT('Ctrl Pts',(30.328246868162,31.4577556961901,41.8149517876113));
#40652=CARTESIAN_POINT('Ctrl Pts',(30.3312711550256,32.0091637019358,41.7779085245381));
#40653=CARTESIAN_POINT('Ctrl Pts',(30.3342954418892,32.5605717076814,41.7408652614648));
#40654=CARTESIAN_POINT('Ctrl Pts',(30.6376644275264,33.1103023612409,41.7038219983916));
#40655=CARTESIAN_POINT('Ctrl Pts',(31.1025613668874,33.4068726645062,41.6667787353184));
#40656=CARTESIAN_POINT('Ctrl Pts',(31.5674583062485,33.7034429677715,41.6297354722451));
#40657=CARTESIAN_POINT('Ctrl Pts',(32.1938831993334,33.7468529207427,41.5926922091719));
#40658=CARTESIAN_POINT('Ctrl Pts',(32.6951809676823,33.5170982491741,41.5556489460986));
#40659=CARTESIAN_POINT('Ctrl Pts',(33.1964787360313,33.2873435776056,41.5186056830254));
#40660=CARTESIAN_POINT('Ctrl Pts',(33.5726493796443,32.7844242814973,41.4815624199522));
#40661=CARTESIAN_POINT('Ctrl Pts',(33.6515719428105,32.2387510696683,41.4445191568789));
#40662=CARTESIAN_POINT('Ctrl Pts',(33.6629345410655,32.1601896895534,41.4391859834559));
#40663=CARTESIAN_POINT('Ctrl Pts',(33.6681358443738,32.080742115373,41.4338528100328));
#40664=CARTESIAN_POINT('Ctrl Pts',(33.6674739163907,32.0012102324881,41.4285196366098));
#40665=CARTESIAN_POINT('Ctrl Pts',(32.5301702171886,30.0148256743283,41.));
#40666=CARTESIAN_POINT('Ctrl Pts',(33.1902397907527,30.1911070339301,41.0370432630732));
#40667=CARTESIAN_POINT('Ctrl Pts',(34.3092433024178,31.2512123085144,41.1111297892197));
#40668=CARTESIAN_POINT('Ctrl Pts',(33.8813840453791,33.5380367222224,41.2222595784394));
#40669=CARTESIAN_POINT('Ctrl Pts',(31.7284038427318,34.4127959913661,41.3333893676592));
#40670=CARTESIAN_POINT('Ctrl Pts',(29.8256278405404,33.0815586024407,41.4445191568789));
#40671=CARTESIAN_POINT('Ctrl Pts',(29.9119860164316,30.7594030366271,41.5556489460986));
#40672=CARTESIAN_POINT('Ctrl Pts',(31.9096898523802,29.5731770382926,41.6667787353184));
#40673=CARTESIAN_POINT('Ctrl Pts',(33.9898334716449,30.6076759933568,41.7779085245381));
#40674=CARTESIAN_POINT('Ctrl Pts',(34.2490097010621,32.9165547497841,41.8890383137578));
#40675=CARTESIAN_POINT('Ctrl Pts',(32.4498627820811,34.3865418359406,42.0001681029776));
#40676=CARTESIAN_POINT('Ctrl Pts',(30.2390335296879,33.6724274291408,42.1112978921972));
#40677=CARTESIAN_POINT('Ctrl Pts',(29.6398079512964,31.4277075354308,42.222427681417));
#40678=CARTESIAN_POINT('Ctrl Pts',(31.2006114825729,29.706752611882,42.3335574706367));
#40679=CARTESIAN_POINT('Ctrl Pts',(33.4930032094031,30.0845482255105,42.4446872598564));
#40680=CARTESIAN_POINT('Ctrl Pts',(34.4190163612264,32.2153468561681,42.5558170490762));
#40681=CARTESIAN_POINT('Ctrl Pts',(33.1311710776567,34.1490612048519,42.6669468382959));
#40682=CARTESIAN_POINT('Ctrl Pts',(30.8080907428172,34.1159786377566,42.7780766275156));
#40683=CARTESIAN_POINT('Ctrl Pts',(29.5758326061327,32.1463750685223,42.8892064167354));
#40684=CARTESIAN_POINT('Ctrl Pts',(30.5621462946373,30.0428107753347,43.0003362059551));
#40685=CARTESIAN_POINT('Ctrl Pts',(32.8643680431626,29.7304447592571,43.1114659951748));
#40686=CARTESIAN_POINT('Ctrl Pts',(34.3755295616921,31.4951511258333,43.2225957843945));
#40687=CARTESIAN_POINT('Ctrl Pts',(33.7126321720426,33.7218896876768,43.3337255736143));
#40688=CARTESIAN_POINT('Ctrl Pts',(31.4823523987704,34.3727734903307,43.444855362834));
#40689=CARTESIAN_POINT('Ctrl Pts',(29.7258180926964,32.8521207213123,43.5559851520537));
#40690=CARTESIAN_POINT('Ctrl Pts',(30.0505904076267,30.5516163115282,43.6671149412734));
#40691=CARTESIAN_POINT('Ctrl Pts',(32.1594412400625,29.576656945096,43.7782447304932));
#40692=CARTESIAN_POINT('Ctrl Pts',(34.1223731791502,30.8195148630926,43.8893745197129));
#40693=CARTESIAN_POINT('Ctrl Pts',(34.1429322006114,33.1427399762344,44.0005043089326));
#40694=CARTESIAN_POINT('Ctrl Pts',(32.2023029113298,34.4201418557892,44.1116340981523));
#40695=CARTESIAN_POINT('Ctrl Pts',(30.0765281914199,33.4826561541886,44.2227638873721));
#40696=CARTESIAN_POINT('Ctrl Pts',(29.7110940115711,31.1882596190528,44.3338936765918));
#40697=CARTESIAN_POINT('Ctrl Pts',(31.4404417701646,29.6367590775809,44.4450234658115));
#40698=CARTESIAN_POINT('Ctrl Pts',(33.6818911525552,30.2480710000371,44.5561532550313));
#40699=CARTESIAN_POINT('Ctrl Pts',(34.3840919914733,32.462729344375,44.667283044251));
#40700=CARTESIAN_POINT('Ctrl Pts',(32.9043976941981,34.2539028108345,44.7784128334707));
#40701=CARTESIAN_POINT('Ctrl Pts',(30.5970084349764,33.9823288673751,44.8895426226904));
#40702=CARTESIAN_POINT('Ctrl Pts',(29.5736218412549,31.8965490419561,45.0006724119102));
#40703=CARTESIAN_POINT('Ctrl Pts',(30.7708302254411,29.9054464114596,45.1118022011299));
#40704=CARTESIAN_POINT('Ctrl Pts',(33.0929614575128,29.8312565107077,45.2229319903496));
#40705=CARTESIAN_POINT('Ctrl Pts',(34.414826216342,31.7418771323123,45.3340617795693));
#40706=CARTESIAN_POINT('Ctrl Pts',(33.526668209675,33.8887290031987,45.4451915687891));
#40707=CARTESIAN_POINT('Ctrl Pts',(31.2413200135407,34.3070365727709,45.5563213580088));
#40708=CARTESIAN_POINT('Ctrl Pts',(29.6503075134721,32.6139692897129,45.6674511472286));
#40709=CARTESIAN_POINT('Ctrl Pts',(30.2097080957199,30.3590039709295,45.7785809364483));
#40710=CARTESIAN_POINT('Ctrl Pts',(32.4075644138576,29.6058604220904,45.889710725668));
#40711=CARTESIAN_POINT('Ctrl Pts',(34.2324222002848,31.0438074515917,46.0008405148877));
#40712=CARTESIAN_POINT('Ctrl Pts',(34.014191398622,33.3568515319198,46.1119703041075));
#40713=CARTESIAN_POINT('Ctrl Pts',(31.9525944719365,34.4281198046771,46.2231000933271));
#40714=CARTESIAN_POINT('Ctrl Pts',(29.9343825704431,33.2771991640567,46.3342298825469));
#40715=CARTESIAN_POINT('Ctrl Pts',(29.806601339792,30.9573996991398,46.4453596717666));
#40716=CARTESIAN_POINT('Ctrl Pts',(31.6861947765452,29.5917767230407,46.5564894609864));
#40717=CARTESIAN_POINT('Ctrl Pts',(33.8529793507283,30.4301335739208,46.6676192502061));
#40718=CARTESIAN_POINT('Ctrl Pts',(34.3239373178492,32.7052151534561,46.7787490394258));
#40719=CARTESIAN_POINT('Ctrl Pts',(32.6680530537252,34.3348914722883,46.8898788286455));
#40720=CARTESIAN_POINT('Ctrl Pts',(30.4007738795658,33.8277004365258,47.0010086178653));
#40721=CARTESIAN_POINT('Ctrl Pts',(29.5970891079424,31.6478177818408,47.112138407085));
#40722=CARTESIAN_POINT('Ctrl Pts',(30.9925223262469,29.790248473958,47.2232681963047));
#40723=CARTESIAN_POINT('Ctrl Pts',(33.3099881859296,29.9550197989514,47.3343979855245));
#40724=CARTESIAN_POINT('Ctrl Pts',(34.42856706408,31.9913348270576,47.4455277747441));
#40725=CARTESIAN_POINT('Ctrl Pts',(33.3245477018974,34.0355801274709,47.556657563964));
#40726=CARTESIAN_POINT('Ctrl Pts',(31.0083166470601,34.21688457017,47.6677873531835));
#40727=CARTESIAN_POINT('Ctrl Pts',(29.5996634424752,32.3693202953617,47.7789171424034));
#40728=CARTESIAN_POINT('Ctrl Pts',(30.387772224771,30.1837580913501,47.890046931623));
#40729=CARTESIAN_POINT('Ctrl Pts',(32.6513743830742,29.6604007858116,48.0011767208428));
#40730=CARTESIAN_POINT('Ctrl Pts',(34.318845769849,31.2782193092014,48.1123065100625));
#40731=CARTESIAN_POINT('Ctrl Pts',(33.8641346548932,33.5566036934244,48.2234362992823));
#40732=CARTESIAN_POINT('Ctrl Pts',(31.7033877194777,34.4104012580895,48.3345660885019));
#40733=CARTESIAN_POINT('Ctrl Pts',(29.81409712657,33.0582257310643,48.4456958777218));
#40734=CARTESIAN_POINT('Ctrl Pts',(29.9253211382958,30.7375734909492,48.5568256669414));
#40735=CARTESIAN_POINT('Ctrl Pts',(31.935268745298,29.572280301472,48.6679554561612));
#40736=CARTESIAN_POINT('Ctrl Pts',(34.0044576946222,30.6288098525638,48.7790852453808));
#40737=CARTESIAN_POINT('Ctrl Pts',(34.2391886992667,32.9402377566512,48.8902150346007));
#40738=CARTESIAN_POINT('Ctrl Pts',(32.4246384893326,34.3911702623054,49.0013448238203));
#40739=CARTESIAN_POINT('Ctrl Pts',(30.221463738974,33.6537296750593,49.1124746130401));
#40740=CARTESIAN_POINT('Ctrl Pts',(29.6459860872837,31.4028136231505,49.2236044022597));
#40741=CARTESIAN_POINT('Ctrl Pts',(31.2248764402936,29.6984360671178,49.3347341914796));
#40742=CARTESIAN_POINT('Ctrl Pts',(33.5131514692818,30.1004248630373,49.4458639806992));
#40743=CARTESIAN_POINT('Ctrl Pts',(34.4166066830276,32.2408842242706,49.556993769919));
#40744=CARTESIAN_POINT('Ctrl Pts',(33.1084096674749,34.160888955732,49.6681235591387));
#40745=CARTESIAN_POINT('Ctrl Pts',(30.7858081444514,34.1032715487725,49.7792533483584));
#40746=CARTESIAN_POINT('Ctrl Pts',(29.5744218402637,32.1207628294065,49.8903831375782));
#40747=CARTESIAN_POINT('Ctrl Pts',(30.5828983635668,30.0277332781861,50.0015129267979));
#40748=CARTESIAN_POINT('Ctrl Pts',(32.8882909367063,29.7397008424277,50.1126427160176));
#40749=CARTESIAN_POINT('Ctrl Pts',(34.3807292776862,31.520269683756,50.2237725052373));
#40750=CARTESIAN_POINT('Ctrl Pts',(33.6943500016618,33.7398825080518,50.3349022944571));
#40751=CARTESIAN_POINT('Ctrl Pts',(31.4573199785767,34.3671737292195,50.4460320836768));
#40752=CARTESIAN_POINT('Ctrl Pts',(29.7169448259793,32.828053224334,50.5571618728965));
#40753=CARTESIAN_POINT('Ctrl Pts',(30.0659970099416,30.5311073884045,50.6682916621163));
#40754=CARTESIAN_POINT('Ctrl Pts',(32.1850277570195,29.5784761411241,50.7794214513359));
#40755=CARTESIAN_POINT('Ctrl Pts',(34.1347231074093,30.8419972691661,50.8905512405558));
#40756=CARTESIAN_POINT('Ctrl Pts',(34.1307430200187,33.1653099384271,51.0016810297753));
#40757=CARTESIAN_POINT('Ctrl Pts',(32.1767300276281,34.4221435893461,51.1128108189952));
#40758=CARTESIAN_POINT('Ctrl Pts',(30.0609756305588,33.4622576942574,51.2239406082148));
#40759=CARTESIAN_POINT('Ctrl Pts',(29.7197953084608,31.1641294150899,51.3350703974346));
#40760=CARTESIAN_POINT('Ctrl Pts',(31.4654335924627,29.6309808302345,51.4462001866543));
#40761=CARTESIAN_POINT('Ctrl Pts',(33.7003012551285,30.2659328993153,51.557329975874));
#40762=CARTESIAN_POINT('Ctrl Pts',(34.3790716488582,32.4878843723627,51.6684597650938));
#40763=CARTESIAN_POINT('Ctrl Pts',(32.8805414680095,34.2633293614917,51.7795895543134));
#40764=CARTESIAN_POINT('Ctrl Pts',(30.5761492876849,33.9673998582603,51.8907193435333));
#40765=CARTESIAN_POINT('Ctrl Pts',(29.5748498323699,31.8709273512164,52.0018491327529));
#40766=CARTESIAN_POINT('Ctrl Pts',(30.7930215224583,29.8925807110175,52.1129789219727));
#40767=CARTESIAN_POINT('Ctrl Pts',(33.1158068029996,29.8429213928206,52.2241087111924));
#40768=CARTESIAN_POINT('Ctrl Pts',(34.4174178435015,31.7673969387678,52.3352385004122));
#40769=CARTESIAN_POINT('Ctrl Pts',(33.5066341990735,33.9047484513664,52.4463682896318));
#40770=CARTESIAN_POINT('Ctrl Pts',(31.216995453309,34.2988945058415,52.5574980788517));
#40771=CARTESIAN_POINT('Ctrl Pts',(29.6439536232049,32.5891178954443,52.6686278680713));
#40772=CARTESIAN_POINT('Ctrl Pts',(30.2271405879685,30.340185676392,52.7797576572911));
#40773=CARTESIAN_POINT('Ctrl Pts',(32.4328278728442,29.6103000988841,52.8908874465108));
#40774=CARTESIAN_POINT('Ctrl Pts',(34.2423985299477,31.0674368629122,53.0020172357305));
#40775=CARTESIAN_POINT('Ctrl Pts',(33.9997449308191,33.3780553787745,53.1131470249502));
#40776=CARTESIAN_POINT('Ctrl Pts',(31.9269572256365,34.4274725972727,53.2242768141699));
#40777=CARTESIAN_POINT('Ctrl Pts',(29.9209961576786,33.2553327321614,53.3354066033897));
#40778=CARTESIAN_POINT('Ctrl Pts',(29.8177590626321,30.9342477419074,53.4465363926093));
#40779=CARTESIAN_POINT('Ctrl Pts',(31.7116016611041,29.5886825160599,53.5576661818292));
#40780=CARTESIAN_POINT('Ctrl Pts',(33.869548688589,30.4496223292041,53.6687959710489));
#40781=CARTESIAN_POINT('Ctrl Pts',(34.3161775882222,32.7300579964386,53.7799257602685));
#40782=CARTESIAN_POINT('Ctrl Pts',(32.6437142303927,34.3411494950526,53.8910555494883));
#40783=CARTESIAN_POINT('Ctrl Pts',(30.3808455967403,33.8120435710866,54.002185338708));
#40784=CARTESIAN_POINT('Ctrl Pts',(29.6023723893559,31.6196455898001,54.1133151279278));
#40785=CARTESIAN_POINT('Ctrl Pts',(30.5427968191103,30.3983372977455,54.1874016540742));
#40786=CARTESIAN_POINT('Ctrl Pts',(31.1673980508611,30.121497522815,54.2244449171475));
#40787=CARTESIAN_POINT('Ctrl Pts',(32.4967348970877,30.1400211999972,40.9251850276175));
#40788=CARTESIAN_POINT('Ctrl Pts',(33.1151770144774,30.3051853306507,40.9622282906908));
#40789=CARTESIAN_POINT('Ctrl Pts',(34.1636102839946,31.2984347954455,41.0363148168372));
#40790=CARTESIAN_POINT('Ctrl Pts',(33.7627340802347,33.4410400436705,41.147444606057));
#40791=CARTESIAN_POINT('Ctrl Pts',(31.7455321237292,34.2606323961771,41.2585743952767));
#40792=CARTESIAN_POINT('Ctrl Pts',(29.9627551758999,33.013349833053,41.3697041844964));
#40793=CARTESIAN_POINT('Ctrl Pts',(30.043667151381,30.8376416008499,41.4808339737161));
#40794=CARTESIAN_POINT('Ctrl Pts',(31.9153852848962,29.7262252479473,41.5919637629359));
#40795=CARTESIAN_POINT('Ctrl Pts',(33.8643441157457,30.6954832622999,41.7030935521556));
#40796=CARTESIAN_POINT('Ctrl Pts',(34.1071753300863,32.85875199049,41.8142233413754));
#40797=CARTESIAN_POINT('Ctrl Pts',(32.4214920708779,34.2360339657663,41.925353130595));
#40798=CARTESIAN_POINT('Ctrl Pts',(30.3500893297177,33.5669553663467,42.0364829198148));
#40799=CARTESIAN_POINT('Ctrl Pts',(29.7886540654114,31.4637993058167,42.1476127090344));
#40800=CARTESIAN_POINT('Ctrl Pts',(31.2510251235106,29.851376843886,42.2587424982543));
#40801=CARTESIAN_POINT('Ctrl Pts',(33.3988465808343,30.2053466806888,42.369872287474));
#40802=CARTESIAN_POINT('Ctrl Pts',(34.2664604768241,32.2017659517052,42.4810020766936));
#40803=CARTESIAN_POINT('Ctrl Pts',(33.0598334848532,34.0135301113067,42.5921318659135));
#40804=CARTESIAN_POINT('Ctrl Pts',(30.8832588044191,33.9825339047513,42.7032616551331));
#40805=CARTESIAN_POINT('Ctrl Pts',(29.7287133417236,32.1371438874559,42.8143914443529));
#40806=CARTESIAN_POINT('Ctrl Pts',(30.652824905654,30.1662414134641,42.9255212335726));
#40807=CARTESIAN_POINT('Ctrl Pts',(32.809856451845,29.8735748399382,43.0366510227923));
#40808=CARTESIAN_POINT('Ctrl Pts',(34.2257161834047,31.526989548972,43.1477808120121));
#40809=CARTESIAN_POINT('Ctrl Pts',(33.604624586873,33.6132982749202,43.2589106012318));
#40810=CARTESIAN_POINT('Ctrl Pts',(31.5149979768988,34.2231339243874,43.3700403904515));
#40811=CARTESIAN_POINT('Ctrl Pts',(29.8692399552855,32.798381510474,43.4811701796712));
#40812=CARTESIAN_POINT('Ctrl Pts',(30.1735304212594,30.642958998618,43.592299968891));
#40813=CARTESIAN_POINT('Ctrl Pts',(32.1493860375522,29.7294856935398,43.7034297581107));
#40814=CARTESIAN_POINT('Ctrl Pts',(33.9885251727594,30.8939624596328,43.8145595473304));
#40815=CARTESIAN_POINT('Ctrl Pts',(34.0077876342834,33.0706727878886,43.9256893365501));
#40816=CARTESIAN_POINT('Ctrl Pts',(32.1895446265783,34.267514991785,44.0368191257699));
#40817=CARTESIAN_POINT('Ctrl Pts',(30.1978324320956,33.3891520652985,44.1479489149896));
#40818=CARTESIAN_POINT('Ctrl Pts',(29.8554444520954,31.2394522334168,44.2590787042094));
#40819=CARTESIAN_POINT('Ctrl Pts',(31.4757304527859,29.7857974696952,44.370208493429));
#40820=CARTESIAN_POINT('Ctrl Pts',(33.5758222576279,30.358556849692,44.4813382826489));
#40821=CARTESIAN_POINT('Ctrl Pts',(34.2337386213657,32.4335472001359,44.5924680718684));
#40822=CARTESIAN_POINT('Ctrl Pts',(32.8473616227183,34.1117598546416,44.7035978610883));
#40823=CARTESIAN_POINT('Ctrl Pts',(30.6854884562122,33.85731279126,44.8147276503079));
#40824=CARTESIAN_POINT('Ctrl Pts',(29.7266419992971,31.9030732030364,44.9258574395277));
#40825=CARTESIAN_POINT('Ctrl Pts',(30.8483481310841,30.0375399682662,45.0369872287474));
#40826=CARTESIAN_POINT('Ctrl Pts',(33.0240335641586,29.9680288725461,45.1481170179672));
#40827=CARTESIAN_POINT('Ctrl Pts',(34.2625345844966,31.7581557168625,45.2592468071868));
#40828=CARTESIAN_POINT('Ctrl Pts',(33.4303884892692,33.7696158264143,45.3703765964066));
#40829=CARTESIAN_POINT('Ctrl Pts',(31.2891663605798,34.1615427223163,45.4815063856263));
#40830=CARTESIAN_POINT('Ctrl Pts',(29.798491470018,32.5752491597092,45.5926361748461));
#40831=CARTESIAN_POINT('Ctrl Pts',(30.3226133117298,30.4624938044536,45.7037659640658));
#40832=CARTESIAN_POINT('Ctrl Pts',(32.3818612600453,29.7568474458017,45.8148957532855));
#40833=CARTESIAN_POINT('Ctrl Pts',(34.0916339242804,31.1041099787756,45.9260255425052));
#40834=CARTESIAN_POINT('Ctrl Pts',(33.8871659038393,33.2712813436514,46.0371553317249));
#40835=CARTESIAN_POINT('Ctrl Pts',(31.9555841136666,34.2749898092894,46.1482851209447));
#40836=CARTESIAN_POINT('Ctrl Pts',(30.064651260996,33.1966522727031,46.2594149101643));
#40837=CARTESIAN_POINT('Ctrl Pts',(29.9449285862787,31.0231515532923,46.3705446993842));
#40838=CARTESIAN_POINT('Ctrl Pts',(31.7059849830777,29.7436519388281,46.4816744886038));
#40839=CARTESIAN_POINT('Ctrl Pts',(33.7361207349039,30.5291376008727,46.5928042778236));
#40840=CARTESIAN_POINT('Ctrl Pts',(34.1773776175914,32.6607405797601,46.7039340670433));
#40841=CARTESIAN_POINT('Ctrl Pts',(32.6259221173363,34.1876409454842,46.815063856263));
#40842=CARTESIAN_POINT('Ctrl Pts',(30.5016294831377,33.7124360418794,46.9261936454828));
#40843=CARTESIAN_POINT('Ctrl Pts',(29.7486292968198,31.6700282433421,47.0373234347025));
#40844=CARTESIAN_POINT('Ctrl Pts',(31.0560591629539,29.9296070181035,47.1484532239222));
#40845=CARTESIAN_POINT('Ctrl Pts',(33.2273734465404,30.0839869974196,47.2595830131419));
#40846=CARTESIAN_POINT('Ctrl Pts',(34.2754088621639,31.9918812984015,47.3707128023616));
#40847=CARTESIAN_POINT('Ctrl Pts',(33.2410147629166,33.9072057470427,47.4818425915815));
#40848=CARTESIAN_POINT('Ctrl Pts',(31.0708574108927,34.0770761787755,47.5929723808011));
#40849=CARTESIAN_POINT('Ctrl Pts',(29.751041280288,32.3460290166462,47.7041021700209));
#40850=CARTESIAN_POINT('Ctrl Pts',(30.489447781022,30.2982998510106,47.8152319592405));
#40851=CARTESIAN_POINT('Ctrl Pts',(32.610295291308,29.8079482075606,47.9263617484603));
#40852=CARTESIAN_POINT('Ctrl Pts',(34.1726071693657,31.3237385927392,48.03749153768));
#40853=CARTESIAN_POINT('Ctrl Pts',(33.7465725269636,33.4584360840934,48.1486213268998));
#40854=CARTESIAN_POINT('Ctrl Pts',(31.7220936486748,34.258388687366,48.2597511161194));
#40855=CARTESIAN_POINT('Ctrl Pts',(29.9519516493499,32.9914884551668,48.3708809053392));
#40856=CARTESIAN_POINT('Ctrl Pts',(30.0561612903804,30.8171887410435,48.482010694559));
#40857=CARTESIAN_POINT('Ctrl Pts',(31.9393510384019,29.7253850640632,48.5931404837786));
#40858=CARTESIAN_POINT('Ctrl Pts',(33.8780460583672,30.7152843092805,48.7042702729984));
#40859=CARTESIAN_POINT('Ctrl Pts',(34.0979736922764,32.8809414224827,48.815400062218));
#40860=CARTESIAN_POINT('Ctrl Pts',(32.3978585545914,34.2403704992407,48.9265298514379));
#40861=CARTESIAN_POINT('Ctrl Pts',(30.3336275823409,33.5494367909,49.0376596406575));
#40862=CARTESIAN_POINT('Ctrl Pts',(29.7944425756754,31.4404753344699,49.1487894298773));
#40863=CARTESIAN_POINT('Ctrl Pts',(31.2737598054777,29.8435847841406,49.259919219097));
#40864=CARTESIAN_POINT('Ctrl Pts',(33.4177241855597,30.2202220540166,49.3710490083167));
#40865=CARTESIAN_POINT('Ctrl Pts',(34.2642027655962,32.2256927991686,49.4821787975365));
#40866=CARTESIAN_POINT('Ctrl Pts',(33.0385075288155,34.0246119420578,49.5933085867562));
#40867=CARTESIAN_POINT('Ctrl Pts',(30.8623814638081,33.9706281915781,49.7044383759759));
#40868=CARTESIAN_POINT('Ctrl Pts',(29.7273915461642,32.1131468907389,49.8155681651957));
#40869=CARTESIAN_POINT('Ctrl Pts',(30.6722682400584,30.1521147825225,49.9266979544154));
#40870=CARTESIAN_POINT('Ctrl Pts',(32.8322706419999,29.8822471858606,50.0378277436351));
#40871=CARTESIAN_POINT('Ctrl Pts',(34.2305879779822,31.5505239986264,50.1489575328548));
#40872=CARTESIAN_POINT('Ctrl Pts',(33.5874953862348,33.6301563734847,50.2600873220746));
#40873=CARTESIAN_POINT('Ctrl Pts',(31.4915442326755,34.2178873136402,50.3712171112943));
#40874=CARTESIAN_POINT('Ctrl Pts',(29.8609262833992,32.7758318363371,50.482346900514));
#40875=CARTESIAN_POINT('Ctrl Pts',(30.1879654022659,30.6237434759671,50.5934766897337));
#40876=CARTESIAN_POINT('Ctrl Pts',(32.173358934285,29.7311901615058,50.7046064789535));
#40877=CARTESIAN_POINT('Ctrl Pts',(34.0000962496398,30.9150270070274,50.8157362681732));
#40878=CARTESIAN_POINT('Ctrl Pts',(33.9963671674767,33.0918193696534,50.9268660573929));
#40879=CARTESIAN_POINT('Ctrl Pts',(32.165584503316,34.269390485504,51.0379958466126));
#40880=CARTESIAN_POINT('Ctrl Pts',(30.1832606974559,33.3700400394506,51.1491256358324));
#40881=CARTESIAN_POINT('Ctrl Pts',(29.8635969994753,31.2168438069273,51.2602554250521));
#40882=CARTESIAN_POINT('Ctrl Pts',(31.4991461594303,29.7803836289929,51.3713852142718));
#40883=CARTESIAN_POINT('Ctrl Pts',(33.5930713223822,30.3752922837321,51.4825150034915));
#40884=CARTESIAN_POINT('Ctrl Pts',(34.2290348879394,32.4571158198614,51.5936447927113));
#40885=CARTESIAN_POINT('Ctrl Pts',(32.8250098955248,34.1205919174751,51.704774581931));
#40886=CARTESIAN_POINT('Ctrl Pts',(30.66594479637,33.8433252839165,51.8159043711507));
#40887=CARTESIAN_POINT('Ctrl Pts',(29.727792546839,31.8790673507646,51.9270341603705));
#40888=CARTESIAN_POINT('Ctrl Pts',(30.8691399282894,30.0254856465071,52.0381639495901));
#40889=CARTESIAN_POINT('Ctrl Pts',(33.0454381620998,29.9789581058905,52.14929373881));
#40890=CARTESIAN_POINT('Ctrl Pts',(34.2649627700276,31.7820661102086,52.2604235280296));
#40891=CARTESIAN_POINT('Ctrl Pts',(33.411617928661,33.7846250039935,52.3715533172494));
#40892=CARTESIAN_POINT('Ctrl Pts',(31.2663758349493,34.1539141369164,52.4826831064691));
#40893=CARTESIAN_POINT('Ctrl Pts',(29.7925382894626,32.5519650249647,52.5938128956888));
#40894=CARTESIAN_POINT('Ctrl Pts',(30.3389464194041,30.4448622904655,52.7049426849086));
#40895=CARTESIAN_POINT('Ctrl Pts',(32.4055314725411,29.7610071332449,52.8160724741282));
#40896=CARTESIAN_POINT('Ctrl Pts',(34.100981094166,31.1262491952386,52.9272022633481));
#40897=CARTESIAN_POINT('Ctrl Pts',(33.8736305062165,33.2911479644908,53.0383320525677));
#40898=CARTESIAN_POINT('Ctrl Pts',(31.9315636868498,34.2743834181852,53.1494618417875));
#40899=CARTESIAN_POINT('Ctrl Pts',(30.0521090657699,33.1761648529178,53.2605916310072));
#40900=CARTESIAN_POINT('Ctrl Pts',(29.9553826444794,31.0014596801536,53.3717214202268));
#40901=CARTESIAN_POINT('Ctrl Pts',(31.7297895759754,29.7407528688005,53.4828512094467));
#40902=CARTESIAN_POINT('Ctrl Pts',(33.7516451232423,30.5473972928286,53.5939809986663));
#40903=CARTESIAN_POINT('Ctrl Pts',(34.1701072572945,32.6840167025074,53.7051107878861));
#40904=CARTESIAN_POINT('Ctrl Pts',(32.6031182281109,34.1935043044452,53.8162405771058));
#40905=CARTESIAN_POINT('Ctrl Pts',(30.4829579825565,33.6977665806563,53.9273703663255));
#40906=CARTESIAN_POINT('Ctrl Pts',(29.7535793867421,31.6436327377849,54.0385001555453));
#40907=CARTESIAN_POINT('Ctrl Pts',(30.6346957097411,30.4993465649721,54.1125866816917));
#40908=CARTESIAN_POINT('Ctrl Pts',(31.2199063053491,30.2399657611256,54.149629944765));
#40909=CARTESIAN_POINT('Ctrl Pts',(32.4632995769868,30.2652167256662,40.850370055235));
#40910=CARTESIAN_POINT('Ctrl Pts',(33.0401142382021,30.4192636273712,40.8874133183083));
#40911=CARTESIAN_POINT('Ctrl Pts',(34.0179772655714,31.3456572823766,40.9614998444547));
#40912=CARTESIAN_POINT('Ctrl Pts',(33.6440841150904,33.3440433651185,41.0726296336745));
#40913=CARTESIAN_POINT('Ctrl Pts',(31.7626604047266,34.1084688009882,41.1837594228942));
#40914=CARTESIAN_POINT('Ctrl Pts',(30.0998825112594,32.9451410636651,41.294889212114));
#40915=CARTESIAN_POINT('Ctrl Pts',(30.1753482863305,30.9158801650729,41.4060190013336));
#40916=CARTESIAN_POINT('Ctrl Pts',(31.9210807174123,29.8792734576019,41.5171487905534));
#40917=CARTESIAN_POINT('Ctrl Pts',(33.7388547598464,30.7832905312431,41.6282785797731));
#40918=CARTESIAN_POINT('Ctrl Pts',(33.9653409591104,32.8009492311959,41.7394083689928));
#40919=CARTESIAN_POINT('Ctrl Pts',(32.3931213596747,34.085526095592,41.8505381582126));
#40920=CARTESIAN_POINT('Ctrl Pts',(30.4611451297475,33.4614833035526,41.9616679474322));
#40921=CARTESIAN_POINT('Ctrl Pts',(29.9375001795264,31.4998910762026,42.0727977366521));
#40922=CARTESIAN_POINT('Ctrl Pts',(31.3014387644482,29.9960010758901,42.1839275258717));
#40923=CARTESIAN_POINT('Ctrl Pts',(33.3046899522655,30.326145135867,42.2950573150915));
#40924=CARTESIAN_POINT('Ctrl Pts',(34.1139045924217,32.1881850472423,42.4061871043112));
#40925=CARTESIAN_POINT('Ctrl Pts',(32.9884958920498,33.8779990177615,42.5173168935309));
#40926=CARTESIAN_POINT('Ctrl Pts',(30.958426866021,33.849089171746,42.6284466827506));
#40927=CARTESIAN_POINT('Ctrl Pts',(29.8815940773145,32.1279127063896,42.7395764719704));
#40928=CARTESIAN_POINT('Ctrl Pts',(30.7435035166707,30.2896720515934,42.8507062611901));
#40929=CARTESIAN_POINT('Ctrl Pts',(32.7553448605274,30.0167049206194,42.9618360504098));
#40930=CARTESIAN_POINT('Ctrl Pts',(34.0759028051174,31.5588279721106,43.0729658396296));
#40931=CARTESIAN_POINT('Ctrl Pts',(33.4966170017034,33.5047068621638,43.1840956288492));
#40932=CARTESIAN_POINT('Ctrl Pts',(31.5476435550272,34.0734943584441,43.2952254180691));
#40933=CARTESIAN_POINT('Ctrl Pts',(30.0126618178744,32.7446422996357,43.4063552072887));
#40934=CARTESIAN_POINT('Ctrl Pts',(30.296470434892,30.7343016857078,43.5174849965085));
#40935=CARTESIAN_POINT('Ctrl Pts',(32.1393308350419,29.8823144419834,43.6286147857282));
#40936=CARTESIAN_POINT('Ctrl Pts',(33.8546771663686,30.968410056173,43.739744574948));
#40937=CARTESIAN_POINT('Ctrl Pts',(33.8726430679553,32.9986055995426,43.8508743641676));
#40938=CARTESIAN_POINT('Ctrl Pts',(32.1767863418268,34.1148881277808,43.9620041533874));
#40939=CARTESIAN_POINT('Ctrl Pts',(30.3191366727714,33.2956479764084,44.0731339426071));
#40940=CARTESIAN_POINT('Ctrl Pts',(29.9997948926197,31.2906448477808,44.1842637318268));
#40941=CARTESIAN_POINT('Ctrl Pts',(31.5110191354072,29.9348358618094,44.2953935210465));
#40942=CARTESIAN_POINT('Ctrl Pts',(33.4697533627006,30.469042699347,44.4065233102663));
#40943=CARTESIAN_POINT('Ctrl Pts',(34.0833852512582,32.4043650558968,44.517653099486));
#40944=CARTESIAN_POINT('Ctrl Pts',(32.7903255512385,33.9696168984488,44.6287828887058));
#40945=CARTESIAN_POINT('Ctrl Pts',(30.773968477448,33.732296715145,44.7399126779254));
#40946=CARTESIAN_POINT('Ctrl Pts',(29.8796621573394,31.9095973641168,44.8510424671452));
#40947=CARTESIAN_POINT('Ctrl Pts',(30.9258660367271,30.1696335250728,44.9621722563649));
#40948=CARTESIAN_POINT('Ctrl Pts',(32.9551056708045,30.1048012343845,45.0733020455847));
#40949=CARTESIAN_POINT('Ctrl Pts',(34.1102429526512,31.7744343014126,45.1844318348043));
#40950=CARTESIAN_POINT('Ctrl Pts',(33.3341087688635,33.6505026496298,45.2955616240241));
#40951=CARTESIAN_POINT('Ctrl Pts',(31.337012707619,34.0160488718617,45.4066914132438));
#40952=CARTESIAN_POINT('Ctrl Pts',(29.9466754265638,32.5365290297053,45.5178212024635));
#40953=CARTESIAN_POINT('Ctrl Pts',(30.4355185277397,30.5659836379777,45.6289509916833));
#40954=CARTESIAN_POINT('Ctrl Pts',(32.3561581062331,29.907834469513,45.7400807809029));
#40955=CARTESIAN_POINT('Ctrl Pts',(33.9508456482759,31.1644125059596,45.8512105701228));
#40956=CARTESIAN_POINT('Ctrl Pts',(33.7601404090566,33.1857111553829,45.9623403593423));
#40957=CARTESIAN_POINT('Ctrl Pts',(31.9585737553967,34.1218598139018,46.0734701485622));
#40958=CARTESIAN_POINT('Ctrl Pts',(30.1949199515488,33.1161053813493,46.1845999377819));
#40959=CARTESIAN_POINT('Ctrl Pts',(30.0832558327655,31.0889034074447,46.2957297270016));
#40960=CARTESIAN_POINT('Ctrl Pts',(31.7257751896102,29.8955271546156,46.4068595162213));
#40961=CARTESIAN_POINT('Ctrl Pts',(33.6192621190795,30.6281416278246,46.5179893054411));
#40962=CARTESIAN_POINT('Ctrl Pts',(34.0308179173337,32.616266006064,46.6291190946608));
#40963=CARTESIAN_POINT('Ctrl Pts',(32.5837911809473,34.0403904186801,46.7402488838805));
#40964=CARTESIAN_POINT('Ctrl Pts',(30.6024850867097,33.5971716472329,46.8513786731003));
#40965=CARTESIAN_POINT('Ctrl Pts',(29.9001694856972,31.6922387048434,46.96250846232));
#40966=CARTESIAN_POINT('Ctrl Pts',(31.119595999661,30.068965562249,47.0736382515397));
#40967=CARTESIAN_POINT('Ctrl Pts',(33.1447587071512,30.2129541958878,47.1847680407594));
#40968=CARTESIAN_POINT('Ctrl Pts',(34.1222506602479,31.9924277697453,47.2958978299792));
#40969=CARTESIAN_POINT('Ctrl Pts',(33.1574818239358,33.7788313666146,47.4070276191989));
#40970=CARTESIAN_POINT('Ctrl Pts',(31.1333981747253,33.937267787381,47.5181574084186));
#40971=CARTESIAN_POINT('Ctrl Pts',(29.9024191181009,32.3227377379307,47.6292871976384));
#40972=CARTESIAN_POINT('Ctrl Pts',(30.591123337273,30.4128416106712,47.740416986858));
#40973=CARTESIAN_POINT('Ctrl Pts',(32.5692161995418,29.9554956293095,47.8515467760779));
#40974=CARTESIAN_POINT('Ctrl Pts',(34.0263685688824,31.369257876277,47.9626765652974));
#40975=CARTESIAN_POINT('Ctrl Pts',(33.6290103990342,33.3602684747623,48.0738063545174));
#40976=CARTESIAN_POINT('Ctrl Pts',(31.7407995778718,34.1063761166425,48.1849361437369));
#40977=CARTESIAN_POINT('Ctrl Pts',(30.0898061721298,32.9247511792693,48.2960659329568));
#40978=CARTESIAN_POINT('Ctrl Pts',(30.187001442465,30.8968039911378,48.4071957221765));
#40979=CARTESIAN_POINT('Ctrl Pts',(31.9434333315057,29.8784898266544,48.5183255113961));
#40980=CARTESIAN_POINT('Ctrl Pts',(33.7516344221123,30.8017587659972,48.6294553006159));
#40981=CARTESIAN_POINT('Ctrl Pts',(33.9567586852861,32.8216450883142,48.7405850898356));
#40982=CARTESIAN_POINT('Ctrl Pts',(32.3710786198504,34.0895707361761,48.8517148790554));
#40983=CARTESIAN_POINT('Ctrl Pts',(30.4457914257076,33.4451439067406,48.9628446682751));
#40984=CARTESIAN_POINT('Ctrl Pts',(29.9428990640671,31.4781370457892,49.0739744574948));
#40985=CARTESIAN_POINT('Ctrl Pts',(31.3226431706617,29.9887335011634,49.1851042467146));
#40986=CARTESIAN_POINT('Ctrl Pts',(33.3222969018377,30.340019244996,49.2962340359342));
#40987=CARTESIAN_POINT('Ctrl Pts',(34.1117988481647,32.2105013740665,49.407363825154));
#40988=CARTESIAN_POINT('Ctrl Pts',(32.9686053901562,33.8883349283837,49.5184936143737));
#40989=CARTESIAN_POINT('Ctrl Pts',(30.9389547831648,33.8379848343838,49.6296234035935));
#40990=CARTESIAN_POINT('Ctrl Pts',(29.8803612520648,32.1055309520713,49.7407531928131));
#40991=CARTESIAN_POINT('Ctrl Pts',(30.76163811655,30.2764962868588,49.851882982033));
#40992=CARTESIAN_POINT('Ctrl Pts',(32.7762503472934,30.0247935292935,49.9630127712526));
#40993=CARTESIAN_POINT('Ctrl Pts',(34.0804466782781,31.5807783134968,50.0741425604724));
#40994=CARTESIAN_POINT('Ctrl Pts',(33.4806407708078,33.5204302389176,50.1852723496921));
#40995=CARTESIAN_POINT('Ctrl Pts',(31.5257684867742,34.068600898061,50.2964021389118));
#40996=CARTESIAN_POINT('Ctrl Pts',(30.0049077408191,32.7236104483403,50.4075319281315));
#40997=CARTESIAN_POINT('Ctrl Pts',(30.3099337945902,30.7163795635297,50.5186617173512));
#40998=CARTESIAN_POINT('Ctrl Pts',(32.1616901115504,29.8839041818875,50.629791506571));
#40999=CARTESIAN_POINT('Ctrl Pts',(33.8654693918704,30.9880567448887,50.7409212957908));
#41000=CARTESIAN_POINT('Ctrl Pts',(33.8619913149347,33.0183288008796,50.8520510850104));
#41001=CARTESIAN_POINT('Ctrl Pts',(32.154438979004,34.116637381662,50.9631808742302));
#41002=CARTESIAN_POINT('Ctrl Pts',(30.305545764353,33.2778223846438,51.0743106634499));
#41003=CARTESIAN_POINT('Ctrl Pts',(30.0073986904897,31.2695581987648,51.1854404526696));
#41004=CARTESIAN_POINT('Ctrl Pts',(31.5328587263979,29.9297864277512,51.2965702418893));
#41005=CARTESIAN_POINT('Ctrl Pts',(33.4858413896359,30.4846516681489,51.407700031109));
#41006=CARTESIAN_POINT('Ctrl Pts',(34.0789981270206,32.4263472673601,51.5188298203288));
#41007=CARTESIAN_POINT('Ctrl Pts',(32.7694783230401,33.9778544734584,51.6299596095485));
#41008=CARTESIAN_POINT('Ctrl Pts',(30.7557403050552,33.7192507095727,51.7410893987683));
#41009=CARTESIAN_POINT('Ctrl Pts',(29.8807352613081,31.8872073503127,51.8522191879879));
#41010=CARTESIAN_POINT('Ctrl Pts',(30.9452583341205,30.1583905819967,51.9633489772077));
#41011=CARTESIAN_POINT('Ctrl Pts',(32.9750695212001,30.1149948189604,52.0744787664274));
#41012=CARTESIAN_POINT('Ctrl Pts',(34.1125076965538,31.7967352816494,52.1856085556472));
#41013=CARTESIAN_POINT('Ctrl Pts',(33.3166016582486,33.6645015566205,52.2967383448668));
#41014=CARTESIAN_POINT('Ctrl Pts',(31.3157562165896,34.0089337679915,52.4078681340867));
#41015=CARTESIAN_POINT('Ctrl Pts',(29.9411229557203,32.5148121544851,52.5189979233063));
#41016=CARTESIAN_POINT('Ctrl Pts',(30.4507522508398,30.549538904539,52.6301277125261));
#41017=CARTESIAN_POINT('Ctrl Pts',(32.378235072238,29.9117141676057,52.7412575017457));
#41018=CARTESIAN_POINT('Ctrl Pts',(33.9595636583843,31.185061527565,52.8523872909655));
#41019=CARTESIAN_POINT('Ctrl Pts',(33.7475160816141,33.204240550207,52.9635170801852));
#41020=CARTESIAN_POINT('Ctrl Pts',(31.936170148063,34.1212942390978,53.074646869405));
#41021=CARTESIAN_POINT('Ctrl Pts',(30.1832219738614,33.0969969736741,53.1857766586247));
#41022=CARTESIAN_POINT('Ctrl Pts',(30.0930062263266,31.0686716183996,53.2969064478444));
#41023=CARTESIAN_POINT('Ctrl Pts',(31.7479774908468,29.8928232215412,53.4080362370642));
#41024=CARTESIAN_POINT('Ctrl Pts',(33.6337415578955,30.645172256453,53.5191660262839));
#41025=CARTESIAN_POINT('Ctrl Pts',(34.0240369263667,32.6379754085762,53.6302958155036));
#41026=CARTESIAN_POINT('Ctrl Pts',(32.5625222258292,34.0458591138378,53.7414256047233));
#41027=CARTESIAN_POINT('Ctrl Pts',(30.5850703683726,33.583489590226,53.8525553939431));
#41028=CARTESIAN_POINT('Ctrl Pts',(29.9047863841283,31.6676198857696,53.9636851831627));
#41029=CARTESIAN_POINT('Ctrl Pts',(30.7265946003719,30.6003558321987,54.0377717093093));
#41030=CARTESIAN_POINT('Ctrl Pts',(31.2724145598371,30.3584339994361,54.0748149723825));
#41031=CARTESIAN_POINT('Ctrl Pts',(32.4298642568859,30.3904122513352,40.7755550828525));
#41032=CARTESIAN_POINT('Ctrl Pts',(32.9650514619268,30.5333419240918,40.8125983459258));
#41033=CARTESIAN_POINT('Ctrl Pts',(33.8723442471483,31.3928797693077,40.8866848720722));
#41034=CARTESIAN_POINT('Ctrl Pts',(33.525434149946,33.2470466865665,40.997814661292));
#41035=CARTESIAN_POINT('Ctrl Pts',(31.7797886857239,33.9563052057992,41.1089444505117));
#41036=CARTESIAN_POINT('Ctrl Pts',(30.2370098466189,32.8769322942773,41.2200742397314));
#41037=CARTESIAN_POINT('Ctrl Pts',(30.3070294212799,30.9941187292959,41.3312040289512));
#41038=CARTESIAN_POINT('Ctrl Pts',(31.9267761499284,30.0323216672566,41.4423338181709));
#41039=CARTESIAN_POINT('Ctrl Pts',(33.6133654039472,30.8710978001861,41.5534636073906));
#41040=CARTESIAN_POINT('Ctrl Pts',(33.8235065881346,32.7431464719018,41.6645933966104));
#41041=CARTESIAN_POINT('Ctrl Pts',(32.3647506484716,33.9350182254177,41.7757231858301));
#41042=CARTESIAN_POINT('Ctrl Pts',(30.5722009297773,33.3560112407585,41.8868529750498));
#41043=CARTESIAN_POINT('Ctrl Pts',(30.0863462936415,31.5359828465885,41.9979827642696));
#41044=CARTESIAN_POINT('Ctrl Pts',(31.3518524053858,30.1406253078941,42.1091125534893));
#41045=CARTESIAN_POINT('Ctrl Pts',(33.2105333236966,30.4469435910453,42.220242342709));
#41046=CARTESIAN_POINT('Ctrl Pts',(33.9613487080195,32.1746041427795,42.3313721319287));
#41047=CARTESIAN_POINT('Ctrl Pts',(32.9171582992462,33.7424679242163,42.4425019211484));
#41048=CARTESIAN_POINT('Ctrl Pts',(31.033594927623,33.7156444387407,42.5536317103682));
#41049=CARTESIAN_POINT('Ctrl Pts',(30.0344748129053,32.1186815253233,42.6647614995878));
#41050=CARTESIAN_POINT('Ctrl Pts',(30.8341821276874,30.4131026897227,42.7758912888076));
#41051=CARTESIAN_POINT('Ctrl Pts',(32.7008332692098,30.1598350013005,42.8870210780273));
#41052=CARTESIAN_POINT('Ctrl Pts',(33.9260894268301,31.5906663952492,42.9981508672471));
#41053=CARTESIAN_POINT('Ctrl Pts',(33.3886094165338,33.3961154494072,43.1092806564668));
#41054=CARTESIAN_POINT('Ctrl Pts',(31.5802891331557,33.9238547925008,43.2204104456866));
#41055=CARTESIAN_POINT('Ctrl Pts',(30.1560836804634,32.6909030887974,43.3315402349062));
#41056=CARTESIAN_POINT('Ctrl Pts',(30.4194104485247,30.8256443727976,43.442670024126));
#41057=CARTESIAN_POINT('Ctrl Pts',(32.1292756325315,30.0351431904271,43.5537998133457));
#41058=CARTESIAN_POINT('Ctrl Pts',(33.7208291599778,31.0428576527132,43.6649296025654));
#41059=CARTESIAN_POINT('Ctrl Pts',(33.7374985016273,32.9265384111968,43.7760593917852));
#41060=CARTESIAN_POINT('Ctrl Pts',(32.1640280570753,33.9622612637765,43.8871891810049));
#41061=CARTESIAN_POINT('Ctrl Pts',(30.4404409134472,33.2021438875183,43.9983189702246));
#41062=CARTESIAN_POINT('Ctrl Pts',(30.1441453331439,31.3418374621448,44.1094487594444));
#41063=CARTESIAN_POINT('Ctrl Pts',(31.5463078180286,30.0838742539237,44.220578548664));
#41064=CARTESIAN_POINT('Ctrl Pts',(33.3636844677732,30.579528549002,44.3317083378838));
#41065=CARTESIAN_POINT('Ctrl Pts',(33.9330318811508,32.3751829116577,44.4428381271035));
#41066=CARTESIAN_POINT('Ctrl Pts',(32.7332894797586,33.8274739422559,44.5539679163233));
#41067=CARTESIAN_POINT('Ctrl Pts',(30.8624484986839,33.6072806390299,44.665097705543));
#41068=CARTESIAN_POINT('Ctrl Pts',(30.0326823153817,31.9161215251971,44.7762274947627));
#41069=CARTESIAN_POINT('Ctrl Pts',(31.0033839423701,30.3017270818794,44.8873572839824));
#41070=CARTESIAN_POINT('Ctrl Pts',(32.8861777774504,30.2415735962229,44.9984870732022));
#41071=CARTESIAN_POINT('Ctrl Pts',(33.9579513208059,31.7907128859628,45.1096168624218));
#41072=CARTESIAN_POINT('Ctrl Pts',(33.2378290484577,33.5313894728454,45.2207466516416));
#41073=CARTESIAN_POINT('Ctrl Pts',(31.3848590546582,33.8705550214071,45.3318764408613));
#41074=CARTESIAN_POINT('Ctrl Pts',(30.0948593831097,32.4978088997016,45.4430062300811));
#41075=CARTESIAN_POINT('Ctrl Pts',(30.5484237437495,30.6694734715018,45.5541360193008));
#41076=CARTESIAN_POINT('Ctrl Pts',(32.3304549524208,30.0588214932243,45.6652658085205));
#41077=CARTESIAN_POINT('Ctrl Pts',(33.8100573722714,31.2247150331435,45.7763955977402));
#41078=CARTESIAN_POINT('Ctrl Pts',(33.6331149142739,33.1001409671145,45.88752538696));
#41079=CARTESIAN_POINT('Ctrl Pts',(31.9615633971268,33.9687298185142,45.9986551761796));
#41080=CARTESIAN_POINT('Ctrl Pts',(30.3251886421016,33.0355584899957,46.1097849653995));
#41081=CARTESIAN_POINT('Ctrl Pts',(30.2215830792522,31.1546552615972,46.2209147546191));
#41082=CARTESIAN_POINT('Ctrl Pts',(31.7455653961428,30.0474023704031,46.3320445438389));
#41083=CARTESIAN_POINT('Ctrl Pts',(33.5024035032551,30.7271456547765,46.4431743330586));
#41084=CARTESIAN_POINT('Ctrl Pts',(33.884258217076,32.5717914323679,46.5543041222783));
#41085=CARTESIAN_POINT('Ctrl Pts',(32.5416602445583,33.893139891876,46.665433911498));
#41086=CARTESIAN_POINT('Ctrl Pts',(30.7033406902817,33.4819072525865,46.7765637007178));
#41087=CARTESIAN_POINT('Ctrl Pts',(30.0517096745746,31.7144491663447,46.8876934899375));
#41088=CARTESIAN_POINT('Ctrl Pts',(31.183132836368,30.2083241063945,46.9988232791572));
#41089=CARTESIAN_POINT('Ctrl Pts',(33.0621439677619,30.341921394356,47.109953068377));
#41090=CARTESIAN_POINT('Ctrl Pts',(33.9690924583318,31.9929742410892,47.2210828575967));
#41091=CARTESIAN_POINT('Ctrl Pts',(33.073948884955,33.6504569861864,47.3322126468164));
#41092=CARTESIAN_POINT('Ctrl Pts',(31.195938938558,33.7974593959865,47.4433424360361));
#41093=CARTESIAN_POINT('Ctrl Pts',(30.0537969559137,32.2994464592152,47.5544722252559));
#41094=CARTESIAN_POINT('Ctrl Pts',(30.6927988935239,30.5273833703318,47.6656020144756));
#41095=CARTESIAN_POINT('Ctrl Pts',(32.5281371077755,30.1030430510584,47.7767318036953));
#41096=CARTESIAN_POINT('Ctrl Pts',(33.8801299683993,31.4147771598148,47.887861592915));
#41097=CARTESIAN_POINT('Ctrl Pts',(33.5114482711046,33.2621008654313,47.9989913821348));
#41098=CARTESIAN_POINT('Ctrl Pts',(31.7595055070689,33.954363545919,48.1101211713544));
#41099=CARTESIAN_POINT('Ctrl Pts',(30.2276606949097,32.8580139033718,48.2212509605743));
#41100=CARTESIAN_POINT('Ctrl Pts',(30.3178415945496,30.976419241232,48.3323807497939));
#41101=CARTESIAN_POINT('Ctrl Pts',(31.9475156246096,30.0315945892456,48.4435105390137));
#41102=CARTESIAN_POINT('Ctrl Pts',(33.6252227858574,30.8882332227139,48.5546403282333));
#41103=CARTESIAN_POINT('Ctrl Pts',(33.8155436782958,32.7623487541457,48.6657701174532));
#41104=CARTESIAN_POINT('Ctrl Pts',(32.3442986851092,33.9387709731115,48.7768999066728));
#41105=CARTESIAN_POINT('Ctrl Pts',(30.5579552690744,33.3408510225813,48.8880296958926));
#41106=CARTESIAN_POINT('Ctrl Pts',(30.0913555524588,31.5157987571086,48.9991594851122));
#41107=CARTESIAN_POINT('Ctrl Pts',(31.3715265358458,30.1338822181863,49.1102892743321));
#41108=CARTESIAN_POINT('Ctrl Pts',(33.2268696181157,30.4598164359753,49.2214190635517));
#41109=CARTESIAN_POINT('Ctrl Pts',(33.9593949307332,32.1953099489645,49.3325488527716));
#41110=CARTESIAN_POINT('Ctrl Pts',(32.8987032514968,33.7520579147096,49.4436786419912));
#41111=CARTESIAN_POINT('Ctrl Pts',(31.0155281025215,33.7053414771894,49.554808431211));
#41112=CARTESIAN_POINT('Ctrl Pts',(30.0333309579654,32.0979150134037,49.6659382204306));
#41113=CARTESIAN_POINT('Ctrl Pts',(30.8510079930416,30.4008777911951,49.7770680096504));
#41114=CARTESIAN_POINT('Ctrl Pts',(32.7202300525869,30.1673398727264,49.8881977988701));
#41115=CARTESIAN_POINT('Ctrl Pts',(33.9303053785741,31.6110326283673,49.9993275880898));
#41116=CARTESIAN_POINT('Ctrl Pts',(33.3737861553808,33.4107041043505,50.1104573773096));
#41117=CARTESIAN_POINT('Ctrl Pts',(31.559992740873,33.9193144824819,50.2215871665293));
#41118=CARTESIAN_POINT('Ctrl Pts',(30.148889198239,32.6713890603434,50.332716955749));
#41119=CARTESIAN_POINT('Ctrl Pts',(30.4319021869145,30.8090156510923,50.4438467449687));
#41120=CARTESIAN_POINT('Ctrl Pts',(32.1500212888159,30.0366182022692,50.5549765341885));
#41121=CARTESIAN_POINT('Ctrl Pts',(33.7308425341009,31.06108648275,50.6661063234082));
#41122=CARTESIAN_POINT('Ctrl Pts',(33.7276154623926,32.9448382321059,50.7772361126279));
#41123=CARTESIAN_POINT('Ctrl Pts',(32.143293454692,33.96388427782,50.8883659018477));
#41124=CARTESIAN_POINT('Ctrl Pts',(30.42783083125,33.1856047298371,50.9994956910674));
#41125=CARTESIAN_POINT('Ctrl Pts',(30.1512003815042,31.3222725906022,51.1106254802871));
#41126=CARTESIAN_POINT('Ctrl Pts',(31.5665712933655,30.0791892265096,51.2217552695068));
#41127=CARTESIAN_POINT('Ctrl Pts',(33.3786114568897,30.5940110525657,51.3328850587266));
#41128=CARTESIAN_POINT('Ctrl Pts',(33.9289613661019,32.3955787148589,51.4440148479463));
#41129=CARTESIAN_POINT('Ctrl Pts',(32.7139467505554,33.8351170294417,51.555144637166));
#41130=CARTESIAN_POINT('Ctrl Pts',(30.8455358137404,33.5951761352289,51.6662744263858));
#41131=CARTESIAN_POINT('Ctrl Pts',(30.0336779757772,31.8953473498609,51.7774042156054));
#41132=CARTESIAN_POINT('Ctrl Pts',(31.0213767399516,30.2912955174864,51.8885340048252));
#41133=CARTESIAN_POINT('Ctrl Pts',(32.9047008803004,30.2510315320302,51.9996637940449));
#41134=CARTESIAN_POINT('Ctrl Pts',(33.9600526230799,31.8114044530902,52.1107935832647));
#41135=CARTESIAN_POINT('Ctrl Pts',(33.2215853878362,33.5443781092476,52.2219233724843));
#41136=CARTESIAN_POINT('Ctrl Pts',(31.3651365982299,33.8639533990665,52.3330531617042));
#41137=CARTESIAN_POINT('Ctrl Pts',(30.089707621978,32.4776592840055,52.4441829509237));
#41138=CARTESIAN_POINT('Ctrl Pts',(30.5625580822755,30.6542155186125,52.5553127401437));
#41139=CARTESIAN_POINT('Ctrl Pts',(32.350938671935,30.0624212019666,52.6664425293632));
#41140=CARTESIAN_POINT('Ctrl Pts',(33.8181462226027,31.2438738598914,52.7775723185831));
#41141=CARTESIAN_POINT('Ctrl Pts',(33.6214016570116,33.1173331359233,52.8887021078027));
#41142=CARTESIAN_POINT('Ctrl Pts',(31.9407766092763,33.9682050600104,52.9998318970225));
#41143=CARTESIAN_POINT('Ctrl Pts',(30.3143348819528,33.0178290944304,53.1109616862422));
#41144=CARTESIAN_POINT('Ctrl Pts',(30.2306298081738,31.1358835566457,53.2220914754619));
#41145=CARTESIAN_POINT('Ctrl Pts',(31.7661654057182,30.0448935742819,53.3332212646817));
#41146=CARTESIAN_POINT('Ctrl Pts',(33.5158379925487,30.7429472200775,53.4443510539014));
#41147=CARTESIAN_POINT('Ctrl Pts',(33.877966595439,32.5919341146449,53.5554808431211));
#41148=CARTESIAN_POINT('Ctrl Pts',(32.5219262235475,33.8982139232304,53.6666106323408));
#41149=CARTESIAN_POINT('Ctrl Pts',(30.6871827541888,33.4692125997957,53.7777404215606));
#41150=CARTESIAN_POINT('Ctrl Pts',(30.0559933815144,31.6916070337544,53.8888702107803));
#41151=CARTESIAN_POINT('Ctrl Pts',(30.8184934910026,30.7013650994253,53.9629567369268));
#41152=CARTESIAN_POINT('Ctrl Pts',(31.3249228143251,30.4769022377466,54.));
#41153=CARTESIAN_POINT('Ctrl Pts',(33.6638410485742,32.0009454217316,41.6214803633902));
#41154=CARTESIAN_POINT('Ctrl Pts',(33.664961233117,32.2165036710547,41.6358513744636));
#41155=CARTESIAN_POINT('Ctrl Pts',(33.6260908500516,32.431674600308,41.650222385537));
#41156=CARTESIAN_POINT('Ctrl Pts',(33.5453570674928,32.6297836522019,41.6645933966103));
#41157=CARTESIAN_POINT('Ctrl Pts',(33.3372546082469,33.1404370564071,41.7016366596836));
#41158=CARTESIAN_POINT('Ctrl Pts',(32.8510026283593,33.5377276409124,41.7386799227568));
#41159=CARTESIAN_POINT('Ctrl Pts',(32.3091183519664,33.6398717690552,41.7757231858301));
#41160=CARTESIAN_POINT('Ctrl Pts',(31.7672340755735,33.742015897198,41.8127664489033));
#41161=CARTESIAN_POINT('Ctrl Pts',(31.1697175026754,33.5490135689782,41.8498097119765));
#41162=CARTESIAN_POINT('Ctrl Pts',(30.7899834435371,33.1491743391734,41.8868529750498));
#41163=CARTESIAN_POINT('Ctrl Pts',(30.4102493843987,32.7493351093685,41.923896238123));
#41164=CARTESIAN_POINT('Ctrl Pts',(30.2482978390201,32.1426589779785,41.9609395011963));
#41165=CARTESIAN_POINT('Ctrl Pts',(30.3782397516215,31.6067613225011,41.9979827642696));
#41166=CARTESIAN_POINT('Ctrl Pts',(30.5081816642229,31.0708636670237,42.0350260273428));
#41167=CARTESIAN_POINT('Ctrl Pts',(30.9300170348044,30.6057444874589,42.072069290416));
#41168=CARTESIAN_POINT('Ctrl Pts',(31.4507148731469,30.4242379448684,42.1091125534893));
#41169=CARTESIAN_POINT('Ctrl Pts',(31.9714127114894,30.2427314022778,42.1461558165625));
#41170=CARTESIAN_POINT('Ctrl Pts',(32.590973017593,30.3448374966616,42.1831990796357));
#41171=CARTESIAN_POINT('Ctrl Pts',(33.025889068032,30.6838339691425,42.220242342709));
#41172=CARTESIAN_POINT('Ctrl Pts',(33.422092825981,30.9926560422594,42.2539883496027));
#41173=CARTESIAN_POINT('Ctrl Pts',(33.6650601237133,31.4980736870518,42.2877343564965));
#41174=CARTESIAN_POINT('Ctrl Pts',(33.6682077659727,32.0008552789479,42.3214803633902));
#41175=CARTESIAN_POINT('Ctrl Pts',(32.5301702171886,30.0148256743283,41.));
#41176=CARTESIAN_POINT('Ctrl Pts',(32.5988371051268,30.0402504771426,41.));
#41177=CARTESIAN_POINT('Ctrl Pts',(32.6658006438088,30.0695646181114,41.));
#41178=CARTESIAN_POINT('Ctrl Pts',(32.7308718531578,30.1024741754033,41.));
#41179=CARTESIAN_POINT('Ctrl Pts',(32.7977521620216,30.1362986790245,41.));
#41180=CARTESIAN_POINT('Ctrl Pts',(32.8626342298991,30.1739219849321,41.));
#41181=CARTESIAN_POINT('Ctrl Pts',(32.9252816572652,30.2150696094253,41.));
#41182=CARTESIAN_POINT('Ctrl Pts',(32.9782123144213,30.2498351360624,41.));
#41183=CARTESIAN_POINT('Ctrl Pts',(33.0295474349744,30.2871175547814,41.));
#41184=CARTESIAN_POINT('Ctrl Pts',(33.0791217023575,30.3267693252569,41.));
#41185=CARTESIAN_POINT('Ctrl Pts',(33.101152415551,30.3443904990851,41.));
#41186=CARTESIAN_POINT('Ctrl Pts',(33.1228350751178,30.3624797744732,41.));
#41187=CARTESIAN_POINT('Ctrl Pts',(33.144153618539,30.381024926788,41.));
#41188=CARTESIAN_POINT('Ctrl Pts',(33.1558677004653,30.3912150898427,41.));
#41189=CARTESIAN_POINT('Ctrl Pts',(33.1674718283393,30.4015429009028,41.));
#41190=CARTESIAN_POINT('Ctrl Pts',(33.1789632030502,30.4120063735654,41.));
#41191=CARTESIAN_POINT('Ctrl Pts',(33.1895551793566,30.4216508988997,41.));
#41192=CARTESIAN_POINT('Ctrl Pts',(33.2000527926184,30.43141219387,41.));
#41193=CARTESIAN_POINT('Ctrl Pts',(33.2104379695418,30.4412732542948,41.));
#41194=CARTESIAN_POINT('Ctrl Pts',(33.2635230176514,30.4916792195395,41.));
#41195=CARTESIAN_POINT('Ctrl Pts',(33.3137680834773,30.544773476948,41.));
#41196=CARTESIAN_POINT('Ctrl Pts',(33.3609544746693,30.6002966936962,41.));
#41197=CARTESIAN_POINT('Ctrl Pts',(33.4077742912829,30.6553885699823,41.));
#41198=CARTESIAN_POINT('Ctrl Pts',(33.4515832805539,30.7128726958201,41.));
#41199=CARTESIAN_POINT('Ctrl Pts',(33.4921230168721,30.7725199761025,41.));
#41200=CARTESIAN_POINT('Ctrl Pts',(33.5258091298193,30.8220833231556,41.));
#41201=CARTESIAN_POINT('Ctrl Pts',(33.5572373028608,30.8731408983435,41.));
#41202=CARTESIAN_POINT('Ctrl Pts',(33.5862316727688,30.9255677386219,41.));
#41203=CARTESIAN_POINT('Ctrl Pts',(33.5983395518361,30.947460880083,41.));
#41204=CARTESIAN_POINT('Ctrl Pts',(33.6100226907185,30.9695928397964,41.));
#41205=CARTESIAN_POINT('Ctrl Pts',(33.6212668406506,30.9919546008952,41.));
#41206=CARTESIAN_POINT('Ctrl Pts',(33.6264664374306,31.0022952795331,41.));
#41207=CARTESIAN_POINT('Ctrl Pts',(33.6315721490351,31.0126850985308,41.));
#41208=CARTESIAN_POINT('Ctrl Pts',(33.6365825013037,31.0231231642912,41.));
#41209=CARTESIAN_POINT('Ctrl Pts',(33.6418162986447,31.0340267331209,41.));
#41210=CARTESIAN_POINT('Ctrl Pts',(33.6469424358502,31.0449755037995,41.));
#41211=CARTESIAN_POINT('Ctrl Pts',(33.6519578428112,31.0559641469038,41.));
#41212=CARTESIAN_POINT('Ctrl Pts',(33.6804982000358,31.1184954234379,41.));
#41213=CARTESIAN_POINT('Ctrl Pts',(33.705477565471,31.1823600897106,41.));
#41214=CARTESIAN_POINT('Ctrl Pts',(33.72667246219,31.2473538141253,41.));
#41215=CARTESIAN_POINT('Ctrl Pts',(33.7458696283766,31.3062215380506,41.));
#41216=CARTESIAN_POINT('Ctrl Pts',(33.7619617929881,31.3660161089348,41.));
#41217=CARTESIAN_POINT('Ctrl Pts',(33.7747462387311,31.4265905234075,41.));
#41218=CARTESIAN_POINT('Ctrl Pts',(33.7898804231815,31.4982983142678,41.));
#41219=CARTESIAN_POINT('Ctrl Pts',(33.8003798600472,31.571100476734,41.));
#41220=CARTESIAN_POINT('Ctrl Pts',(33.8063196987879,31.6445738174103,41.));
#41221=CARTESIAN_POINT('Ctrl Pts',(33.8076266382734,31.6607401165739,41.));
#41222=CARTESIAN_POINT('Ctrl Pts',(33.8087126104153,31.6769388277567,41.));
#41223=CARTESIAN_POINT('Ctrl Pts',(33.8095780467764,31.6931652787845,41.));
#41224=CARTESIAN_POINT('Ctrl Pts',(33.8104756849897,31.7099954966529,41.));
#41225=CARTESIAN_POINT('Ctrl Pts',(33.8111360806015,31.7268617851126,41.));
#41226=CARTESIAN_POINT('Ctrl Pts',(33.8115591521967,31.7437245298023,41.));
#41227=CARTESIAN_POINT('Ctrl Pts',(33.8132793295231,31.8122871830253,41.));
#41228=CARTESIAN_POINT('Ctrl Pts',(33.8110878793106,31.8808777362401,41.));
#41229=CARTESIAN_POINT('Ctrl Pts',(33.8051053822439,31.9491577488549,41.));
#41230=CARTESIAN_POINT('Ctrl Pts',(33.7991241582521,32.0174232314892,41.));
#41231=CARTESIAN_POINT('Ctrl Pts',(33.7893530469936,32.0853793775203,41.));
#41232=CARTESIAN_POINT('Ctrl Pts',(33.7758629482066,32.1526729298985,41.));
#41233=CARTESIAN_POINT('Ctrl Pts',(33.7661049603147,32.2013493465565,41.));
#41234=CARTESIAN_POINT('Ctrl Pts',(33.7544000471896,32.2496788103789,41.));
#41235=CARTESIAN_POINT('Ctrl Pts',(33.7407608534051,32.2975179819387,41.));
#41236=CARTESIAN_POINT('Ctrl Pts',(33.7305262323088,32.3334156898394,41.));
#41237=CARTESIAN_POINT('Ctrl Pts',(33.7192022175004,32.3690371718178,41.));
#41238=CARTESIAN_POINT('Ctrl Pts',(33.7067902391303,32.4043176898062,41.));
#41239=CARTESIAN_POINT('Ctrl Pts',(33.7026575280213,32.4160647444878,41.));
#41240=CARTESIAN_POINT('Ctrl Pts',(33.6984073867442,32.42776482926,41.));
#41241=CARTESIAN_POINT('Ctrl Pts',(33.6940404826521,32.4394153171815,41.));
#41242=CARTESIAN_POINT('Ctrl Pts',(33.6709167132624,32.5011073512387,41.));
#41243=CARTESIAN_POINT('Ctrl Pts',(33.6445204214222,32.5614158634302,41.));
#41244=CARTESIAN_POINT('Ctrl Pts',(33.6149016024334,32.6200066741332,41.));
#41245=CARTESIAN_POINT('Ctrl Pts',(33.5940761769243,32.6612027314195,41.));
#41246=CARTESIAN_POINT('Ctrl Pts',(33.5716567752548,32.7015490788674,41.));
#41247=CARTESIAN_POINT('Ctrl Pts',(33.5476503862663,32.7409182209529,41.));
#41248=CARTESIAN_POINT('Ctrl Pts',(33.5399365462045,32.7535684894111,41.));
#41249=CARTESIAN_POINT('Ctrl Pts',(33.532057703321,32.7661194535318,41.));
#41250=CARTESIAN_POINT('Ctrl Pts',(33.5240173798602,32.778561300404,41.));
#41251=CARTESIAN_POINT('Ctrl Pts',(33.4897744251705,32.8315499147026,41.));
#41252=CARTESIAN_POINT('Ctrl Pts',(33.4526757599804,32.882454648408,41.));
#41253=CARTESIAN_POINT('Ctrl Pts',(33.412755629387,32.9309602071557,41.));
#41254=CARTESIAN_POINT('Ctrl Pts',(33.3759796454528,32.9756454229281,41.));
#41255=CARTESIAN_POINT('Ctrl Pts',(33.3368085492858,33.0182945959076,41.));
#41256=CARTESIAN_POINT('Ctrl Pts',(33.2952476940792,33.0586283498916,41.));
#41257=CARTESIAN_POINT('Ctrl Pts',(33.2874058553447,33.0662386551351,41.));
#41258=CARTESIAN_POINT('Ctrl Pts',(33.2794788845476,33.0737664244156,41.));
#41259=CARTESIAN_POINT('Ctrl Pts',(33.2714683883714,33.0812109859128,41.));
#41260=CARTESIAN_POINT('Origin',(32.,32.,48.));
#41261=CARTESIAN_POINT('Origin',(32.,-32.,54.));
#41262=CARTESIAN_POINT('Ctrl Pts',(31.3249228143251,-33.5230977622534,54.));
#41263=CARTESIAN_POINT('Ctrl Pts',(31.265239275159,-33.5045114719856,54.));
#41264=CARTESIAN_POINT('Ctrl Pts',(31.206868285946,-33.482350599571,54.));
#41265=CARTESIAN_POINT('Ctrl Pts',(31.1499663996996,-33.4569140176145,54.));
#41266=CARTESIAN_POINT('Ctrl Pts',(31.1138836062791,-33.4407840965766,54.));
#41267=CARTESIAN_POINT('Ctrl Pts',(31.0783915059693,-33.4233358717196,54.));
#41268=CARTESIAN_POINT('Ctrl Pts',(31.0435309165988,-33.4046351138275,54.));
#41269=CARTESIAN_POINT('Ctrl Pts',(31.0197680190607,-33.3918876473705,54.));
#41270=CARTESIAN_POINT('Ctrl Pts',(30.9962985734341,-33.3785580214987,54.));
#41271=CARTESIAN_POINT('Ctrl Pts',(30.973135972271,-33.3646651103166,54.));
#41272=CARTESIAN_POINT('Ctrl Pts',(30.9607872858049,-33.357258377235,54.));
#41273=CARTESIAN_POINT('Ctrl Pts',(30.9485259765169,-33.3496914691038,54.));
#41274=CARTESIAN_POINT('Ctrl Pts',(30.9363661582946,-33.3419751431426,54.));
#41275=CARTESIAN_POINT('Ctrl Pts',(30.8806643177476,-33.3066281050175,54.));
#41276=CARTESIAN_POINT('Ctrl Pts',(30.8270262511519,-33.2681116533153,54.));
#41277=CARTESIAN_POINT('Ctrl Pts',(30.7756337832862,-33.2267282656662,54.));
#41278=CARTESIAN_POINT('Ctrl Pts',(30.7385650270783,-33.196878936153,54.));
#41279=CARTESIAN_POINT('Ctrl Pts',(30.7026646421898,-33.1655368474349,54.));
#41280=CARTESIAN_POINT('Ctrl Pts',(30.6680061457107,-33.1327996377017,54.));
#41281=CARTESIAN_POINT('Ctrl Pts',(30.6585368474332,-33.12385526806,54.));
#41282=CARTESIAN_POINT('Ctrl Pts',(30.6491602875156,-33.1148066861414,54.));
#41283=CARTESIAN_POINT('Ctrl Pts',(30.6398780493963,-33.1056557310545,54.));
#41284=CARTESIAN_POINT('Ctrl Pts',(30.6303147814348,-33.0962277208618,54.));
#41285=CARTESIAN_POINT('Ctrl Pts',(30.6208573412613,-33.0866966156126,54.));
#41286=CARTESIAN_POINT('Ctrl Pts',(30.6115109509391,-33.0770688360442,54.));
#41287=CARTESIAN_POINT('Ctrl Pts',(30.564248583844,-33.0283835536427,54.));
#41288=CARTESIAN_POINT('Ctrl Pts',(30.5197931029259,-32.977199343729,54.));
#41289=CARTESIAN_POINT('Ctrl Pts',(30.4783282142722,-32.9238232967636,54.));
#41290=CARTESIAN_POINT('Ctrl Pts',(30.4362641057054,-32.869675898632,54.));
#41291=CARTESIAN_POINT('Ctrl Pts',(30.397276759,-32.8132722746407,54.));
#41292=CARTESIAN_POINT('Ctrl Pts',(30.3615823177727,-32.7548861115473,54.));
#41293=CARTESIAN_POINT('Ctrl Pts',(30.3394716332882,-32.7187191907038,54.));
#41294=CARTESIAN_POINT('Ctrl Pts',(30.3186249995123,-32.6817906574975,54.));
#41295=CARTESIAN_POINT('Ctrl Pts',(30.2991007045613,-32.6441582896561,54.));
#41296=CARTESIAN_POINT('Ctrl Pts',(30.2831164151376,-32.6133491536137,54.));
#41297=CARTESIAN_POINT('Ctrl Pts',(30.2680185026127,-32.5820681575949,54.));
#41298=CARTESIAN_POINT('Ctrl Pts',(30.2538422753457,-32.5503447932022,54.));
#41299=CARTESIAN_POINT('Ctrl Pts',(30.2480302988927,-32.537338833056,54.));
#41300=CARTESIAN_POINT('Ctrl Pts',(30.2423723901086,-32.5242560222887,54.));
#41301=CARTESIAN_POINT('Ctrl Pts',(30.2368801512033,-32.5111208799825,54.));
#41302=CARTESIAN_POINT('Ctrl Pts',(30.2096895647203,-32.446092349906,54.));
#41303=CARTESIAN_POINT('Ctrl Pts',(30.1865046901109,-32.3796719815527,54.));
#41304=CARTESIAN_POINT('Ctrl Pts',(30.1675371008066,-32.3121549062884,54.));
#41305=CARTESIAN_POINT('Ctrl Pts',(30.1654370835708,-32.3046796800225,54.));
#41306=CARTESIAN_POINT('Ctrl Pts',(30.1633887977462,-32.2971909716448,54.));
#41307=CARTESIAN_POINT('Ctrl Pts',(30.1613925585069,-32.2896891540652,54.));
#41308=CARTESIAN_POINT('Ctrl Pts',(30.1440544308544,-32.2245329001155,54.));
#41309=CARTESIAN_POINT('Ctrl Pts',(30.1306386024233,-32.1583897935046,54.));
#41310=CARTESIAN_POINT('Ctrl Pts',(30.1209910276371,-32.091564292141,54.));
#41311=CARTESIAN_POINT('Ctrl Pts',(30.1106125640439,-32.0196761701662,54.));
#41312=CARTESIAN_POINT('Ctrl Pts',(30.1045943189643,-31.9469975500423,54.));
#41313=CARTESIAN_POINT('Ctrl Pts',(30.1028046617085,-31.8738849141495,54.));
#41314=CARTESIAN_POINT('Ctrl Pts',(30.1024845931803,-31.8608091960565,54.));
#41315=CARTESIAN_POINT('Ctrl Pts',(30.1022999347513,-31.8477195615237,54.));
#41316=CARTESIAN_POINT('Ctrl Pts',(30.1022501401139,-31.834618015092,54.));
#41317=CARTESIAN_POINT('Ctrl Pts',(30.1022051724613,-31.8227865043478,54.));
#41318=CARTESIAN_POINT('Ctrl Pts',(30.1022702435749,-31.8109538847267,54.));
#41319=CARTESIAN_POINT('Ctrl Pts',(30.1024444017349,-31.7991251289033,54.));
#41320=CARTESIAN_POINT('Ctrl Pts',(30.1034906362357,-31.7280652805266,54.));
#41321=CARTESIAN_POINT('Ctrl Pts',(30.1084694479729,-31.657107539816,54.));
#41322=CARTESIAN_POINT('Ctrl Pts',(30.1172007059819,-31.5865875101679,54.));
#41323=CARTESIAN_POINT('Ctrl Pts',(30.1261162000589,-31.5145794552014,54.));
#41324=CARTESIAN_POINT('Ctrl Pts',(30.1389441161484,-31.4430268429001,54.));
#41325=CARTESIAN_POINT('Ctrl Pts',(30.1555453764766,-31.3722707824218,54.));
#41326=CARTESIAN_POINT('Ctrl Pts',(30.1722475569473,-31.3010845912446,54.));
#41327=CARTESIAN_POINT('Ctrl Pts',(30.1927691766452,-31.2307035954258,54.));
#41328=CARTESIAN_POINT('Ctrl Pts',(30.2170210079531,-31.1614742347,54.));
#41329=CARTESIAN_POINT('Ctrl Pts',(30.2230020127514,-31.1444008379149,54.));
#41330=CARTESIAN_POINT('Ctrl Pts',(30.2292101405796,-31.1273975251947,54.));
#41331=CARTESIAN_POINT('Ctrl Pts',(30.2356445302325,-31.1104696030387,54.));
#41332=CARTESIAN_POINT('Ctrl Pts',(30.2407135367379,-31.0971338008628,54.));
#41333=CARTESIAN_POINT('Ctrl Pts',(30.2459237428321,-31.0838431856506,54.));
#41334=CARTESIAN_POINT('Ctrl Pts',(30.2512662871439,-31.0706205546988,54.));
#41335=CARTESIAN_POINT('Ctrl Pts',(30.2794914752907,-31.0007640921922,54.));
#41336=CARTESIAN_POINT('Ctrl Pts',(30.3114528952479,-30.9326785760022,54.));
#41337=CARTESIAN_POINT('Ctrl Pts',(30.3469924394571,-30.8667213482137,54.));
#41338=CARTESIAN_POINT('Ctrl Pts',(30.3825709935462,-30.8006917226613,54.));
#41339=CARTESIAN_POINT('Ctrl Pts',(30.4217357025888,-30.7367939449245,54.));
#41340=CARTESIAN_POINT('Ctrl Pts',(30.4643797046174,-30.6753909583728,54.));
#41341=CARTESIAN_POINT('Ctrl Pts',(30.5060535838732,-30.6153848490545,54.));
#41342=CARTESIAN_POINT('Ctrl Pts',(30.5510505920688,-30.5577603295061,54.));
#41343=CARTESIAN_POINT('Ctrl Pts',(30.5993163303218,-30.5028757509615,54.));
#41344=CARTESIAN_POINT('Ctrl Pts',(30.6096515549672,-30.491123222784,54.));
#41345=CARTESIAN_POINT('Ctrl Pts',(30.6201368170775,-30.4794964310409,54.));
#41346=CARTESIAN_POINT('Ctrl Pts',(30.6307718389113,-30.4679990812668,54.));
#41347=CARTESIAN_POINT('Ctrl Pts',(30.6398828867194,-30.4581492751173,54.));
#41348=CARTESIAN_POINT('Ctrl Pts',(30.6491038508474,-30.448394472897,54.));
#41349=CARTESIAN_POINT('Ctrl Pts',(30.6584328706692,-30.4387350900139,54.));
#41350=CARTESIAN_POINT('Ctrl Pts',(31.6163320011532,-29.9813874990081,54.));
#41351=CARTESIAN_POINT('Ctrl Pts',(31.6906497010824,-29.9743669064257,54.));
#41352=CARTESIAN_POINT('Ctrl Pts',(31.7652155019048,-29.9717482581011,54.));
#41353=CARTESIAN_POINT('Ctrl Pts',(31.8397072864826,-29.973367958639,54.));
#41354=CARTESIAN_POINT('Ctrl Pts',(31.912240978847,-29.9749450837032,54.));
#41355=CARTESIAN_POINT('Ctrl Pts',(31.9847052775767,-29.9805413173162,54.));
#41356=CARTESIAN_POINT('Ctrl Pts',(32.0567896040968,-29.9900494850227,54.));
#41357=CARTESIAN_POINT('Ctrl Pts',(32.0728797819135,-29.9921718341726,54.));
#41358=CARTESIAN_POINT('Ctrl Pts',(32.0889530810813,-29.9944895851625,54.));
#41359=CARTESIAN_POINT('Ctrl Pts',(32.1049990789946,-29.9970007294107,54.));
#41360=CARTESIAN_POINT('Ctrl Pts',(32.1786326509453,-30.0085241336686,54.));
#41361=CARTESIAN_POINT('Ctrl Pts',(32.2515465731326,-30.0240920503004,54.));
#41362=CARTESIAN_POINT('Ctrl Pts',(32.3234089125773,-30.0435649879731,54.));
#41363=CARTESIAN_POINT('Ctrl Pts',(32.3738561635597,-30.0572349600577,54.));
#41364=CARTESIAN_POINT('Ctrl Pts',(32.4237849187537,-30.0728304248785,54.));
#41365=CARTESIAN_POINT('Ctrl Pts',(32.473072408561,-30.0903162675955,54.));
#41366=CARTESIAN_POINT('Ctrl Pts',(32.4917998053197,-30.0969602317232,54.));
#41367=CARTESIAN_POINT('Ctrl Pts',(32.5104345384574,-30.1038772152795,54.));
#41368=CARTESIAN_POINT('Ctrl Pts',(32.5289695397006,-30.1110656544418,54.));
#41369=CARTESIAN_POINT('Ctrl Pts',(32.5466571041536,-30.1179254317535,54.));
#41370=CARTESIAN_POINT('Ctrl Pts',(32.5642593093968,-30.1250348632197,54.));
#41371=CARTESIAN_POINT('Ctrl Pts',(32.5817390991713,-30.1323793623939,54.));
#41372=CARTESIAN_POINT('Ctrl Pts',(32.6486662599213,-30.1605002084223,54.));
#41373=CARTESIAN_POINT('Ctrl Pts',(32.7138732955257,-30.1920890980459,54.));
#41374=CARTESIAN_POINT('Ctrl Pts',(32.7770519997321,-30.2270188807991,54.));
#41375=CARTESIAN_POINT('Ctrl Pts',(32.8388737020017,-30.2611984141851,54.));
#41376=CARTESIAN_POINT('Ctrl Pts',(32.8987539659087,-30.2985774919006,54.));
#41377=CARTESIAN_POINT('Ctrl Pts',(32.9563716570095,-30.3390737986648,54.));
#41378=CARTESIAN_POINT('Ctrl Pts',(33.012725896401,-30.3786820946978,54.));
#41379=CARTESIAN_POINT('Ctrl Pts',(33.0669162651064,-30.4212729344113,54.));
#41380=CARTESIAN_POINT('Ctrl Pts',(33.1186018592923,-30.4667965224927,54.));
#41381=CARTESIAN_POINT('Ctrl Pts',(33.1354286838459,-30.4816172368864,54.));
#41382=CARTESIAN_POINT('Ctrl Pts',(33.1519896670425,-30.4967489798192,54.));
#41383=CARTESIAN_POINT('Ctrl Pts',(33.1682719417363,-30.5121905362843,54.));
#41384=CARTESIAN_POINT('Ctrl Pts',(33.1774025508037,-30.5208496958996,54.));
#41385=CARTESIAN_POINT('Ctrl Pts',(33.1864463369616,-30.5296072430981,54.));
#41386=CARTESIAN_POINT('Ctrl Pts',(33.1953885762173,-30.5384503466276,54.));
#41387=CARTESIAN_POINT('Ctrl Pts',(33.2439540244105,-30.5864773870649,54.));
#41388=CARTESIAN_POINT('Ctrl Pts',(33.2896151649663,-30.6371069762407,54.));
#41389=CARTESIAN_POINT('Ctrl Pts',(33.3320796339295,-30.6902581242221,54.));
#41390=CARTESIAN_POINT('Ctrl Pts',(33.33818556757,-30.6979006872969,54.));
#41391=CARTESIAN_POINT('Ctrl Pts',(33.3442253363571,-30.70559543444,54.));
#41392=CARTESIAN_POINT('Ctrl Pts',(33.3501979952662,-30.7133421733983,54.));
#41393=CARTESIAN_POINT('Ctrl Pts',(33.3925564663094,-30.76828253126,54.));
#41394=CARTESIAN_POINT('Ctrl Pts',(33.4315435515063,-30.8258365623855,54.));
#41395=CARTESIAN_POINT('Ctrl Pts',(33.4670920125223,-30.8856420553392,54.));
#41396=CARTESIAN_POINT('Ctrl Pts',(33.5002538459271,-30.9414323691067,54.));
#41397=CARTESIAN_POINT('Ctrl Pts',(33.5304228740683,-30.9991829559989,54.));
#41398=CARTESIAN_POINT('Ctrl Pts',(33.5575048000099,-31.0586052133472,54.));
#41399=CARTESIAN_POINT('Ctrl Pts',(33.5633986166787,-31.0715372290249,54.));
#41400=CARTESIAN_POINT('Ctrl Pts',(33.5691460742209,-31.0845484113474,54.));
#41401=CARTESIAN_POINT('Ctrl Pts',(33.5747459551106,-31.0976357581545,54.));
#41402=CARTESIAN_POINT('Ctrl Pts',(33.5792732531105,-31.1082163973129,54.));
#41403=CARTESIAN_POINT('Ctrl Pts',(33.5837038690107,-31.1188465199639,54.));
#41404=CARTESIAN_POINT('Ctrl Pts',(33.5880321351824,-31.1295115045319,54.));
#41405=CARTESIAN_POINT('Ctrl Pts',(33.613744906356,-31.1928685849159,54.));
#41406=CARTESIAN_POINT('Ctrl Pts',(33.6359003814639,-31.2575713836811,54.));
#41407=CARTESIAN_POINT('Ctrl Pts',(33.6544522928069,-31.3232698329539,54.));
#41408=CARTESIAN_POINT('Ctrl Pts',(33.6729185655388,-31.3886650076021,54.));
#41409=CARTESIAN_POINT('Ctrl Pts',(33.6878144745088,-31.4550477976694,54.));
#41410=CARTESIAN_POINT('Ctrl Pts',(33.6990433279385,-31.5220755917657,54.));
#41411=CARTESIAN_POINT('Ctrl Pts',(33.7100316003106,-31.5876672982249,54.));
#41412=CARTESIAN_POINT('Ctrl Pts',(33.7175081391197,-31.6538776300524,54.));
#41413=CARTESIAN_POINT('Ctrl Pts',(33.7213344466344,-31.7203726467958,54.));
#41414=CARTESIAN_POINT('Ctrl Pts',(33.7224477448494,-31.7397199635403,54.));
#41415=CARTESIAN_POINT('Ctrl Pts',(33.7232517169047,-31.7590912458322,54.));
#41416=CARTESIAN_POINT('Ctrl Pts',(33.7237421900973,-31.7784778815483,54.));
#41417=CARTESIAN_POINT('Ctrl Pts',(33.7240143304393,-31.7892346074059,54.));
#41418=CARTESIAN_POINT('Ctrl Pts',(33.7241897036422,-31.7999863091244,54.));
#41419=CARTESIAN_POINT('Ctrl Pts',(33.7242680787914,-31.8107315297782,54.));
#41420=CARTESIAN_POINT('Ctrl Pts',(33.7247442136253,-31.8760095407784,54.));
#41421=CARTESIAN_POINT('Ctrl Pts',(33.7216445542006,-31.9410503644791,54.));
#41422=CARTESIAN_POINT('Ctrl Pts',(33.7148888654324,-32.0055441705781,54.));
#41423=CARTESIAN_POINT('Ctrl Pts',(33.7079758296589,-32.0715401043794,54.));
#41424=CARTESIAN_POINT('Ctrl Pts',(33.6972346760188,-32.1369643866012,54.));
#41425=CARTESIAN_POINT('Ctrl Pts',(33.6825254951079,-32.2014643004376,54.));
#41426=CARTESIAN_POINT('Ctrl Pts',(33.6688931922852,-32.2612420924698,54.));
#41427=CARTESIAN_POINT('Ctrl Pts',(33.6518520468801,-32.3202263589063,54.));
#41428=CARTESIAN_POINT('Ctrl Pts',(33.6312489060068,-32.3781081241769,54.));
#41429=CARTESIAN_POINT('Ctrl Pts',(33.6296213694678,-32.3826804701361,54.));
#41430=CARTESIAN_POINT('Ctrl Pts',(33.6279715848248,-32.3872459188163,54.));
#41431=CARTESIAN_POINT('Ctrl Pts',(33.6262994659155,-32.3918043085367,54.));
#41432=CARTESIAN_POINT('Ctrl Pts',(33.6225368115429,-32.4020617399414,54.));
#41433=CARTESIAN_POINT('Ctrl Pts',(33.6186610677504,-32.4122834302941,54.));
#41434=CARTESIAN_POINT('Ctrl Pts',(33.6146732908669,-32.4224680167337,54.));
#41435=CARTESIAN_POINT('Origin',(32.,-32.,39.4540747194623));
#41436=CARTESIAN_POINT('Ctrl Pts',(34.0565678057143,-31.9985073856871,41.2040747194623));
#41437=CARTESIAN_POINT('Ctrl Pts',(34.057384193637,-31.9004172745425,41.2094078928853));
#41438=CARTESIAN_POINT('Ctrl Pts',(34.006411839884,-31.1218371113704,41.2517843293816));
#41439=CARTESIAN_POINT('Ctrl Pts',(33.0117214699854,-29.7919912031069,41.3312040289512));
#41440=CARTESIAN_POINT('Ctrl Pts',(30.6939306582022,-29.9526094198962,41.4423338181709));
#41441=CARTESIAN_POINT('Ctrl Pts',(29.5714563100008,-31.9866292389199,41.5534636073906));
#41442=CARTESIAN_POINT('Ctrl Pts',(30.6715507437682,-34.0330616484485,41.6645933966103));
#41443=CARTESIAN_POINT('Ctrl Pts',(32.9874316054104,-34.2187692724043,41.7757231858301));
#41444=CARTESIAN_POINT('Ctrl Pts',(34.0018419810914,-32.893577087834,41.8555502934474));
#41445=CARTESIAN_POINT('Ctrl Pts',(34.0572700298053,-32.1072436615327,41.8983341379915));
#41446=CARTESIAN_POINT('Ctrl Pts',(34.056362032224,-32.0016080177294,41.9040747194623));
#41447=CARTESIAN_POINT('Ctrl Pts',(34.0526762468981,-32.0023611642388,41.1459252805377));
#41448=CARTESIAN_POINT('Ctrl Pts',(34.0491258424523,-31.5322384053065,41.1713700465049));
#41449=CARTESIAN_POINT('Ctrl Pts',(33.656679719616,-30.3706653288645,41.2338580755454));
#41450=CARTESIAN_POINT('Ctrl Pts',(31.7284038562778,-29.5872042670172,41.3333893676592));
#41451=CARTESIAN_POINT('Ctrl Pts',(29.825627898444,-30.918441305227,41.4445191568789));
#41452=CARTESIAN_POINT('Ctrl Pts',(29.9119860544063,-33.2405970018638,41.5556489460987));
#41453=CARTESIAN_POINT('Ctrl Pts',(31.9096898625478,-34.4268228681169,41.6667787353183));
#41454=CARTESIAN_POINT('Ctrl Pts',(33.7208347448527,-33.5261026599319,41.7635375134647));
#41455=CARTESIAN_POINT('Ctrl Pts',(34.0499076026638,-32.4182605719717,41.8232530285378));
#41456=CARTESIAN_POINT('Ctrl Pts',(34.0520872241698,-31.9988339725263,41.8459252805377));
#41457=CARTESIAN_POINT('Ctrl Pts',(30.7309291201476,-30.9206413469515,41.));
#41458=CARTESIAN_POINT('Ctrl Pts',(30.3720428517593,-31.3426068457262,41.0370432630732));
#41459=CARTESIAN_POINT('Ctrl Pts',(30.1147036008868,-32.565620122978,41.1111297892197));
#41460=CARTESIAN_POINT('Ctrl Pts',(31.4546601281911,-33.8933249778742,41.2222595784395));
#41461=CARTESIAN_POINT('Ctrl Pts',(33.293843349898,-33.4837762398447,41.3333893676592));
#41462=CARTESIAN_POINT('Ctrl Pts',(33.9488200270038,-31.7184950982882,41.4445191568789));
#41463=CARTESIAN_POINT('Ctrl Pts',(32.8203080515856,-30.2097371185673,41.5556489460986));
#41464=CARTESIAN_POINT('Ctrl Pts',(30.941033447653,-30.3399670488123,41.6667787353184));
#41465=CARTESIAN_POINT('Ctrl Pts',(30.0309264934718,-31.9891589303032,41.7779085245381));
#41466=CARTESIAN_POINT('Ctrl Pts',(30.9228877182713,-33.6484149927315,41.8890383137578));
#41467=CARTESIAN_POINT('Ctrl Pts',(32.8006137265428,-33.7989875205381,42.0001681029776));
#41468=CARTESIAN_POINT('Ctrl Pts',(33.9456250655374,-32.303182554366,42.1112978921973));
#41469=CARTESIAN_POINT('Ctrl Pts',(33.3100222870931,-30.5298898271833,42.222427681417));
#41470=CARTESIAN_POINT('Ctrl Pts',(31.4755008922015,-30.1020352696771,42.3335574706367));
#41471=CARTESIAN_POINT('Ctrl Pts',(30.1209956079544,-31.4111727618922,42.4446872598565));
#41472=CARTESIAN_POINT('Ctrl Pts',(30.4861346576737,-33.2592009254551,42.5558170490762));
#41473=CARTESIAN_POINT('Ctrl Pts',(32.2367469064035,-33.9548208610104,42.6669468382959));
#41474=CARTESIAN_POINT('Ctrl Pts',(33.7706909260737,-32.8614105481285,42.7780766275156));
#41475=CARTESIAN_POINT('Ctrl Pts',(33.6841178265537,-30.9796463378902,42.8892064167354));
#41476=CARTESIAN_POINT('Ctrl Pts',(32.0562583485925,-30.0316988881712,43.0003362059551));
#41477=CARTESIAN_POINT('Ctrl Pts',(30.3769118436706,-30.8851191927514,43.1114659951748));
#41478=CARTESIAN_POINT('Ctrl Pts',(30.1829980159574,-32.7588663611027,43.2225957843945));
#41479=CARTESIAN_POINT('Ctrl Pts',(31.6519847003862,-33.9381072454552,43.3337255736142));
#41480=CARTESIAN_POINT('Ctrl Pts',(33.439471212492,-33.3436134067076,43.444855362834));
#41481=CARTESIAN_POINT('Ctrl Pts',(33.9095692815731,-31.5194591439489,43.5559851520537));
#41482=CARTESIAN_POINT('Ctrl Pts',(32.6320502524575,-30.1350906639621,43.6671149412734));
#41483=CARTESIAN_POINT('Ctrl Pts',(30.7760856866517,-30.4574669829232,43.7782447304932));
#41484=CARTESIAN_POINT('Ctrl Pts',(30.0402342275943,-32.1915527916928,43.8893745197128));
#41485=CARTESIAN_POINT('Ctrl Pts',(31.0979391506829,-33.7503315624784,44.0005043089327));
#41486=CARTESIAN_POINT('Ctrl Pts',(32.9812003806163,-33.707225869006,44.1116340981523));
#41487=CARTESIAN_POINT('Ctrl Pts',(33.9664776628886,-32.1016855742286,44.2227638873721));
#41488=CARTESIAN_POINT('Ctrl Pts',(33.1520559136455,-30.4030837446939,44.3338936765918));
#41489=CARTESIAN_POINT('Ctrl Pts',(31.2832850857612,-30.1659623541582,44.4450234658115));
#41490=CARTESIAN_POINT('Ctrl Pts',(30.0704439749381,-31.6073323277977,44.5561532550313));
#41491=CARTESIAN_POINT('Ctrl Pts',(30.6235116130882,-33.4080674967277,44.6672830442509));
#41492=CARTESIAN_POINT('Ctrl Pts',(32.4363264955448,-33.9201545625114,44.7784128334708));
#41493=CARTESIAN_POINT('Ctrl Pts',(33.8498201010428,-32.6749369958924,44.8895426226904));
#41494=CARTESIAN_POINT('Ctrl Pts',(33.5703784105299,-30.8120244100204,45.0006724119102));
#41495=CARTESIAN_POINT('Ctrl Pts',(31.8537434287449,-30.0363342010384,45.1118022011298));
#41496=CARTESIAN_POINT('Ctrl Pts',(30.270960874886,-31.0577696361976,45.2229319903497));
#41497=CARTESIAN_POINT('Ctrl Pts',(30.270576177683,-32.9415240822457,45.3340617795693));
#41498=CARTESIAN_POINT('Ctrl Pts',(31.852941407844,-33.9636058986261,45.4451915687891));
#41499=CARTESIAN_POINT('Ctrl Pts',(33.5698930667622,-33.1886168910032,45.5563213580087));
#41500=CARTESIAN_POINT('Ctrl Pts',(33.850095615761,-31.3258185947475,45.6674511472286));
#41501=CARTESIAN_POINT('Ctrl Pts',(32.4371107206668,-30.0800238093861,45.7785809364483));
#41502=CARTESIAN_POINT('Ctrl Pts',(30.6240868342867,-30.5913704123997,45.8897107256679));
#41503=CARTESIAN_POINT('Ctrl Pts',(30.0702837560105,-32.3918795380334,46.0008405148877));
#41504=CARTESIAN_POINT('Ctrl Pts',(31.2825360573322,-33.8337447602155,46.1119703041074));
#41505=CARTESIAN_POINT('Ctrl Pts',(33.151403578411,-33.5973866639823,46.2231000933271));
#41506=CARTESIAN_POINT('Ctrl Pts',(33.9665190309799,-31.8991176158095,46.3342298825469));
#41507=CARTESIAN_POINT('Ctrl Pts',(32.9818975924069,-30.293175031624,46.4453596717666));
#41508=CARTESIAN_POINT('Ctrl Pts',(31.098654125499,-30.2493001487501,46.5564894609863));
#41509=CARTESIAN_POINT('Ctrl Pts',(30.0403126282455,-31.8076467841909,46.6676192502061));
#41510=CARTESIAN_POINT('Ctrl Pts',(30.7754557616971,-33.5420329967564,46.7787490394258));
#41511=CARTESIAN_POINT('Ctrl Pts',(32.6312885024143,-33.8651673333419,46.8898788286455));
#41512=CARTESIAN_POINT('Ctrl Pts',(33.9093728517606,-32.4813207533504,47.0010086178652));
#41513=CARTESIAN_POINT('Ctrl Pts',(33.4400198734621,-30.6569746395988,47.1121384070849));
#41514=CARTESIAN_POINT('Ctrl Pts',(31.6527763233362,-30.0617507711828,47.2232681963047));
#41515=CARTESIAN_POINT('Ctrl Pts',(30.1833081166092,-31.2403915775427,47.3343979855244));
#41516=CARTESIAN_POINT('Ctrl Pts',(30.3764566203582,-33.1142177745252,47.4455277747442));
#41517=CARTESIAN_POINT('Ctrl Pts',(32.0554544185607,-33.9683239474508,47.5566575639638));
#41518=CARTESIAN_POINT('Ctrl Pts',(33.6837009342745,-33.0210413892538,47.6677873531837));
#41519=CARTESIAN_POINT('Ctrl Pts',(33.7710426139166,-31.1393128243445,47.7789171424032));
#41520=CARTESIAN_POINT('Ctrl Pts',(32.2375452994596,-30.0452758288314,47.8900469316231));
#41521=CARTESIAN_POINT('Ctrl Pts',(30.4866491030086,-30.7401811966708,48.0011767208427));
#41522=CARTESIAN_POINT('Ctrl Pts',(30.1207552358772,-32.5880590711511,48.1123065100626));
#41523=CARTESIAN_POINT('Ctrl Pts',(31.47472579731,-33.897751660949,48.2234362992821));
#41524=CARTESIAN_POINT('Ctrl Pts',(33.3094216126832,-33.4706425109062,48.3345660885021));
#41525=CARTESIAN_POINT('Ctrl Pts',(33.9457489682148,-31.6976172833359,48.4456958777216));
#41526=CARTESIAN_POINT('Ctrl Pts',(32.8013479688052,-30.2013294388527,48.5568256669415));
#41527=CARTESIAN_POINT('Ctrl Pts',(30.9235619986018,-30.3511653861614,48.6679554561611));
#41528=CARTESIAN_POINT('Ctrl Pts',(30.0309204137941,-32.0099968911885,48.7790852453809));
#41529=CARTESIAN_POINT('Ctrl Pts',(30.9403591125031,-33.6596793498116,48.8902150346005));
#41530=CARTESIAN_POINT('Ctrl Pts',(32.8195696601223,-33.7904412659602,49.0013448238204));
#41531=CARTESIAN_POINT('Ctrl Pts',(33.9487189426605,-32.2826107520291,49.11247461304));
#41532=CARTESIAN_POINT('Ctrl Pts',(33.2944217818527,-30.5161379426269,49.2236044022598));
#41533=CARTESIAN_POINT('Ctrl Pts',(31.455483843713,-30.1076795963187,49.3347341914795));
#41534=CARTESIAN_POINT('Ctrl Pts',(30.1148811867754,-31.4310523620993,49.4458639806992));
#41535=CARTESIAN_POINT('Ctrl Pts',(30.4995188244386,-33.2751198361065,49.556993769919));
#41536=CARTESIAN_POINT('Ctrl Pts',(32.2573805619349,-33.9522114642078,49.6681235591386));
#41537=CARTESIAN_POINT('Ctrl Pts',(33.7796904003243,-32.8426603311179,49.7792533483585));
#41538=CARTESIAN_POINT('Ctrl Pts',(33.6732468842757,-30.9619156012597,49.8903831375781));
#41539=CARTESIAN_POINT('Ctrl Pts',(32.0354659653448,-30.0312144555721,50.0015129267979));
#41540=CARTESIAN_POINT('Ctrl Pts',(30.3652269795427,-30.9023244895547,50.1126427160176));
#41541=CARTESIAN_POINT('Ctrl Pts',(30.1911145336881,-32.7780152469018,50.2237725052374));
#41542=CARTESIAN_POINT('Ctrl Pts',(31.6724744500558,-33.9416748875081,50.334902294457));
#41543=CARTESIAN_POINT('Ctrl Pts',(33.4535821978664,-33.3283347276548,50.4460320836768));
#41544=CARTESIAN_POINT('Ctrl Pts',(33.9043872816309,-31.4993170302414,50.5571618728964));
#41545=CARTESIAN_POINT('Ctrl Pts',(32.6123177774694,-30.1285189570716,50.6682916621163));
#41546=CARTESIAN_POINT('Ctrl Pts',(30.7598616836728,-30.4704800390206,50.7794214513359));
#41547=CARTESIAN_POINT('Ctrl Pts',(30.0423667282485,-32.2122412023096,50.8905512405557));
#41548=CARTESIAN_POINT('Ctrl Pts',(31.1164765134632,-33.7597615188951,51.0016810297753));
#41549=CARTESIAN_POINT('Ctrl Pts',(32.9991774121812,-33.696767177226,51.1128108189952));
#41550=CARTESIAN_POINT('Ctrl Pts',(33.9674419788235,-32.0809099155954,51.2239406082148));
#41551=CARTESIAN_POINT('Ctrl Pts',(33.1351249826154,-30.391004776719,51.3350703974346));
#41552=CARTESIAN_POINT('Ctrl Pts',(31.2639539119407,-30.1736346172128,51.4462001866543));
#41553=CARTESIAN_POINT('Ctrl Pts',(30.0664042395539,-31.6277342502227,51.5573299758739));
#41554=CARTESIAN_POINT('Ctrl Pts',(30.6384604369997,-33.4225274597867,51.6684597650938));
#41555=CARTESIAN_POINT('Ctrl Pts',(32.4565828795076,-33.9154389659862,51.7795895543135));
#41556=CARTESIAN_POINT('Ctrl Pts',(33.8568456176001,-32.6553615002807,51.8907193435332));
#41557=CARTESIAN_POINT('Ctrl Pts',(33.5577433920753,-30.7955043011809,52.0018491327529));
#41558=CARTESIAN_POINT('Ctrl Pts',(31.8330112894132,-30.0379884943954,52.1129789219727));
#41559=CARTESIAN_POINT('Ctrl Pts',(30.2611054788687,-31.0760843582921,52.2241087111923));
#41560=CARTESIAN_POINT('Ctrl Pts',(30.2806170070421,-32.9597377626332,52.3352385004122));
#41561=CARTESIAN_POINT('Ctrl Pts',(31.8736893420127,-33.9650496446109,52.4463682896318));
#41562=CARTESIAN_POINT('Ctrl Pts',(33.5823595490477,-33.1719692631936,52.5574980788516));
#41563=CARTESIAN_POINT('Ctrl Pts',(33.8428719959032,-31.3063155961969,52.6686278680713));
#41564=CARTESIAN_POINT('Ctrl Pts',(32.416806909947,-30.0755138292301,52.7797576572911));
#41565=CARTESIAN_POINT('Ctrl Pts',(30.6092867728801,-30.6059820117572,52.8908874465107));
#41566=CARTESIAN_POINT('Ctrl Pts',(30.074528117115,-32.4122382091939,53.0020172357305));
#41567=CARTESIAN_POINT('Ctrl Pts',(31.3019487274169,-33.8412226855446,53.1131470249502));
#41568=CARTESIAN_POINT('Ctrl Pts',(33.1682019017076,-33.5851317784421,53.2242768141699));
#41569=CARTESIAN_POINT('Ctrl Pts',(33.965361811241,-31.8783619852648,53.3354066033896));
#41570=CARTESIAN_POINT('Ctrl Pts',(32.9637796720064,-30.2828812659777,53.4465363926094));
#41571=CARTESIAN_POINT('Ctrl Pts',(31.0802839845962,-30.2589537602268,53.557666181829));
#41572=CARTESIAN_POINT('Ctrl Pts',(30.0382506967122,-31.8282846681807,53.6687959710489));
#41573=CARTESIAN_POINT('Ctrl Pts',(30.7920874688999,-33.5550214868453,53.7799257602685));
#41574=CARTESIAN_POINT('Ctrl Pts',(32.6504054262519,-33.8581160689002,53.8910555494883));
#41575=CARTESIAN_POINT('Ctrl Pts',(33.9154419847816,-32.461689344216,54.002185338708));
#41576=CARTESIAN_POINT('Ctrl Pts',(33.4235041713429,-30.6406234847563,54.1133151279277));
#41577=CARTESIAN_POINT('Ctrl Pts',(32.2331222331376,-30.2598665970073,54.1874016540742));
#41578=CARTESIAN_POINT('Ctrl Pts',(31.6889203620495,-30.3633004372052,54.2244449171475));
#41579=CARTESIAN_POINT('Ctrl Pts',(30.6322193753411,-30.8366876301903,40.9251850276175));
#41580=CARTESIAN_POINT('Ctrl Pts',(30.2454185337564,-31.2914740748731,40.9622282906908));
#41581=CARTESIAN_POINT('Ctrl Pts',(29.9680631496753,-32.6096146853645,41.0363148168372));
#41582=CARTESIAN_POINT('Ctrl Pts',(31.4122429863013,-34.0405899008731,41.147444606057));
#41583=CARTESIAN_POINT('Ctrl Pts',(33.3944799249825,-33.5991860063993,41.2585743952767));
#41584=CARTESIAN_POINT('Ctrl Pts',(34.1004014166593,-31.6965993338744,41.3697041844964));
#41585=CARTESIAN_POINT('Ctrl Pts',(32.8841125243855,-30.0704884800805,41.4808339737162));
#41586=CARTESIAN_POINT('Ctrl Pts',(30.8586658511694,-30.2108478391736,41.5919637629359));
#41587=CARTESIAN_POINT('Ctrl Pts',(29.8777697656481,-31.9883156998422,41.7030935521556));
#41588=CARTESIAN_POINT('Ctrl Pts',(30.8391087267702,-33.7766305446372,41.8142233413754));
#41589=CARTESIAN_POINT('Ctrl Pts',(32.862886352832,-33.9389147711602,41.925353130595));
#41590=CARTESIAN_POINT('Ctrl Pts',(34.0969579475357,-32.3267644307185,42.0364829198148));
#41591=CARTESIAN_POINT('Ctrl Pts',(33.4119172779109,-30.415543022525,42.1476127090345));
#41592=CARTESIAN_POINT('Ctrl Pts',(31.4347047681205,-29.9544094615713,42.2587424982542));
#41593=CARTESIAN_POINT('Ctrl Pts',(29.9748445560521,-31.3653731242743,42.369872287474));
#41594=CARTESIAN_POINT('Ctrl Pts',(30.3683845272556,-33.3571429742288,42.4810020766937));
#41595=CARTESIAN_POINT('Ctrl Pts',(32.2551613441515,-34.1068690022105,42.5921318659134));
#41596=CARTESIAN_POINT('Ctrl Pts',(33.9084172360999,-32.9284120188338,42.7032616551332));
#41597=CARTESIAN_POINT('Ctrl Pts',(33.8151103845915,-30.900282094964,42.8143914443528));
#41598=CARTESIAN_POINT('Ctrl Pts',(32.0606341855303,-29.8786022380665,42.9255212335726));
#41599=CARTESIAN_POINT('Ctrl Pts',(30.250666241275,-30.79840252332,43.0366510227923));
#41600=CARTESIAN_POINT('Ctrl Pts',(30.0416695803239,-32.8178918308664,43.1477808120121));
#41601=CARTESIAN_POINT('Ctrl Pts',(31.6249156832344,-34.0888553830443,43.2589106012317));
#41602=CARTESIAN_POINT('Ctrl Pts',(33.5514348847322,-33.4481211521773,43.3700403904515));
#41603=CARTESIAN_POINT('Ctrl Pts',(34.0580977045846,-31.4820821415899,43.4811701796712));
#41604=CARTESIAN_POINT('Ctrl Pts',(32.6812118242147,-29.9900359411961,43.592299968891));
#41605=CARTESIAN_POINT('Ctrl Pts',(30.6808882698222,-30.3374870488719,43.7034297581107));
#41606=CARTESIAN_POINT('Ctrl Pts',(29.8878014656849,-32.2064519809226,43.8145595473304));
#41607=CARTESIAN_POINT('Ctrl Pts',(31.02777585433,-33.8864742985555,43.9256893365501));
#41608=CARTESIAN_POINT('Ctrl Pts',(33.0575192377521,-33.8400157962921,44.0368191257698));
#41609=CARTESIAN_POINT('Ctrl Pts',(34.1194324831063,-32.1095947913117,44.1479489149896));
#41610=CARTESIAN_POINT('Ctrl Pts',(33.2416641042077,-30.2788738218748,44.2590787042093));
#41611=CARTESIAN_POINT('Ctrl Pts',(31.2275382024258,-30.0233088657986,44.3702084934291));
#41612=CARTESIAN_POINT('Ctrl Pts',(29.9203609607839,-31.5767901994327,44.4813382826487));
#41613=CARTESIAN_POINT('Ctrl Pts',(30.5164468150866,-33.5175885530207,44.5924680718685));
#41614=CARTESIAN_POINT('Ctrl Pts',(32.4702644557575,-34.0695063204498,44.7035978610882));
#41615=CARTESIAN_POINT('Ctrl Pts',(33.9937011663249,-32.7274343462632,44.814727650308));
#41616=CARTESIAN_POINT('Ctrl Pts',(33.6925241902605,-30.7196223470743,44.9258574395277));
#41617=CARTESIAN_POINT('Ctrl Pts',(31.8423674299303,-29.8835980907251,45.0369872287474));
#41618=CARTESIAN_POINT('Ctrl Pts',(30.1364742882738,-30.9844819103215,45.1481170179671));
#41619=CARTESIAN_POINT('Ctrl Pts',(30.1360596688943,-33.0147568727565,45.2592468071868));
#41620=CARTESIAN_POINT('Ctrl Pts',(31.8415030269516,-34.1163373498248,45.3703765964066));
#41621=CARTESIAN_POINT('Ctrl Pts',(33.6920010959146,-33.2810688350563,45.4815063856262));
#41622=CARTESIAN_POINT('Ctrl Pts',(33.9939981108845,-31.2733800150573,45.5926361748461));
#41623=CARTESIAN_POINT('Ctrl Pts',(32.4711096787818,-29.9306859254122,45.7037659640657));
#41624=CARTESIAN_POINT('Ctrl Pts',(30.5170667776298,-30.4818056360532,45.8148957532856));
#41625=CARTESIAN_POINT('Ctrl Pts',(29.9201882798498,-32.422360364446,45.9260255425052));
#41626=CARTESIAN_POINT('Ctrl Pts',(31.2267309137324,-33.9763754676053,46.037155331725));
#41627=CARTESIAN_POINT('Ctrl Pts',(33.240961029613,-33.7216331757116,46.1482851209446));
#41628=CARTESIAN_POINT('Ctrl Pts',(34.1194770688537,-31.8912708717411,46.2594149101644));
#41629=CARTESIAN_POINT('Ctrl Pts',(33.0582706794513,-30.1604162868348,46.3705446993841));
#41630=CARTESIAN_POINT('Ctrl Pts',(31.0285464406826,-30.1131287667627,46.4816744886039));
#41631=CARTESIAN_POINT('Ctrl Pts',(29.8878859644261,-31.7926853370829,46.5928042778235));
#41632=CARTESIAN_POINT('Ctrl Pts',(30.6802093486038,-33.661974038671,46.7039340670433));
#41633=CARTESIAN_POINT('Ctrl Pts',(32.6803908244057,-34.0102421234253,46.815063856263));
#41634=CARTESIAN_POINT('Ctrl Pts',(34.0578859962428,-32.5187584169888,46.9261936454828));
#41635=CARTESIAN_POINT('Ctrl Pts',(33.5520262211627,-30.552512633025,47.0373234347024));
#41636=CARTESIAN_POINT('Ctrl Pts',(31.6257688794981,-29.9109915899698,47.1484532239222));
#41637=CARTESIAN_POINT('Ctrl Pts',(30.0420038009492,-31.1813083894214,47.2595830131419));
#41638=CARTESIAN_POINT('Ctrl Pts',(30.2501756101871,-33.2008828725337,47.3707128023617));
#41639=CARTESIAN_POINT('Ctrl Pts',(32.0597677249264,-34.1214223737356,47.4818425915814));
#41640=CARTESIAN_POINT('Ctrl Pts',(33.814661065967,-33.1004591243624,47.5929723808012));
#41641=CARTESIAN_POINT('Ctrl Pts',(33.9087962786145,-31.0723676183549,47.7041021700208));
#41642=CARTESIAN_POINT('Ctrl Pts',(32.2560218371077,-29.8932352082748,47.8152319592406));
#41643=CARTESIAN_POINT('Ctrl Pts',(30.3689389867211,-30.6421910886687,47.9263617484603));
#41644=CARTESIAN_POINT('Ctrl Pts',(29.9745854875673,-32.6337989598886,48.03749153768));
#41645=CARTESIAN_POINT('Ctrl Pts',(31.4338693854861,-34.0453608962819,48.1486213268997));
#41646=CARTESIAN_POINT('Ctrl Pts',(33.4112698823772,-33.5850307214133,48.2597511161195));
#41647=CARTESIAN_POINT('Ctrl Pts',(34.0970914875013,-31.6740976192497,48.3708809053391));
#41648=CARTESIAN_POINT('Ctrl Pts',(32.8636777052743,-30.0614268416845,48.4820106945589));
#41649=CARTESIAN_POINT('Ctrl Pts',(30.839835453375,-30.2229171956593,48.5931404837787));
#41650=CARTESIAN_POINT('Ctrl Pts',(29.8777632130863,-32.010774460506,48.7042702729984));
#41651=CARTESIAN_POINT('Ctrl Pts',(30.8579390654813,-33.7887710559419,48.8154000622181));
#41652=CARTESIAN_POINT('Ctrl Pts',(32.8833167000128,-33.929703779394,48.9265298514378));
#41653=CARTESIAN_POINT('Ctrl Pts',(34.1002924698632,-32.3045925307108,49.0376596406576));
#41654=CARTESIAN_POINT('Ctrl Pts',(33.3951033480182,-30.4007215010895,49.1487894298773));
#41655=CARTESIAN_POINT('Ctrl Pts',(31.4131307713328,-29.960492810218,49.259919219097));
#41656=CARTESIAN_POINT('Ctrl Pts',(29.9682545483917,-31.3867989819005,49.3710490083168));
#41657=CARTESIAN_POINT('Ctrl Pts',(30.3828097294008,-33.3743000754595,49.4821787975364));
#41658=CARTESIAN_POINT('Ctrl Pts',(32.2773999083639,-34.1040566436217,49.5933085867562));
#41659=CARTESIAN_POINT('Ctrl Pts',(33.9181166994692,-32.9082033890855,49.7044383759759));
#41660=CARTESIAN_POINT('Ctrl Pts',(33.8033938883297,-30.8811722419139,49.8155681651957));
#41661=CARTESIAN_POINT('Ctrl Pts',(32.0382245475832,-29.8780801257608,49.9266979544153));
#41662=CARTESIAN_POINT('Ctrl Pts',(30.2380725154165,-30.8169460672487,50.0378277436351));
#41663=CARTESIAN_POINT('Ctrl Pts',(30.0504174098328,-32.8385301383049,50.1489575328548));
#41664=CARTESIAN_POINT('Ctrl Pts',(31.646999148427,-34.092700520265,50.2600873220746));
#41665=CARTESIAN_POINT('Ctrl Pts',(33.5666434382467,-33.431654080471,50.3712171112942));
#41666=CARTESIAN_POINT('Ctrl Pts',(34.0525126429222,-31.4603733518713,50.4823469005141));
#41667=CARTESIAN_POINT('Ctrl Pts',(32.6599445353708,-29.982953079633,50.5934766897336));
#41668=CARTESIAN_POINT('Ctrl Pts',(30.6634023458432,-30.3515122749489,50.7046064789535));
#41669=CARTESIAN_POINT('Ctrl Pts',(29.8900998346124,-32.2287495591319,50.8157362681731));
#41670=CARTESIAN_POINT('Ctrl Pts',(31.0477550738091,-33.8966377274726,50.926866057393));
#41671=CARTESIAN_POINT('Ctrl Pts',(33.0768945428305,-33.8287436158309,51.0379958466126));
#41672=CARTESIAN_POINT('Ctrl Pts',(34.1204718046074,-32.0872031788381,51.1491256358324));
#41673=CARTESIAN_POINT('Ctrl Pts',(33.2234162665272,-30.2658553383336,51.2602554250521));
#41674=CARTESIAN_POINT('Ctrl Pts',(31.2067034284007,-30.0315778860086,51.3713852142719));
#41675=CARTESIAN_POINT('Ctrl Pts',(29.9160070102875,-31.5987790060798,51.4825150034915));
#41676=CARTESIAN_POINT('Ctrl Pts',(30.5325583751517,-33.5331732280924,51.5936447927113));
#41677=CARTESIAN_POINT('Ctrl Pts',(32.4920964037991,-34.064423939581,51.704774581931));
#41678=CARTESIAN_POINT('Ctrl Pts',(34.0012731353756,-32.7063362468262,51.8159043711507));
#41679=CARTESIAN_POINT('Ctrl Pts',(33.6789064060147,-30.7018172857916,51.9270341603705));
#41680=CARTESIAN_POINT('Ctrl Pts',(31.820022721738,-29.8853810568597,52.0381639495902));
#41681=CARTESIAN_POINT('Ctrl Pts',(30.1258523285906,-31.0042211718748,52.1492937388099));
#41682=CARTESIAN_POINT('Ctrl Pts',(30.1468814851308,-33.0343872334662,52.2604235280297));
#41683=CARTESIAN_POINT('Ctrl Pts',(31.8638647585208,-34.1178933919783,52.3715533172493));
#41684=CARTESIAN_POINT('Ctrl Pts',(33.7054372350606,-33.2631263362361,52.4826831064691));
#41685=CARTESIAN_POINT('Ctrl Pts',(33.9862126298382,-31.2523600515833,52.5938128956889));
#41686=CARTESIAN_POINT('Ctrl Pts',(32.4492266150774,-29.9258251539826,52.7049426849085));
#41687=CARTESIAN_POINT('Ctrl Pts',(30.5011155509827,-30.4975537418634,52.8160724741283));
#41688=CARTESIAN_POINT('Ctrl Pts',(29.9247627720828,-32.4443025556973,52.9272022633479));
#41689=CARTESIAN_POINT('Ctrl Pts',(31.2476535228917,-33.9844350342852,53.0383320525678));
#41690=CARTESIAN_POINT('Ctrl Pts',(33.2590659451828,-33.7084250915412,53.1494618417874));
#41691=CARTESIAN_POINT('Ctrl Pts',(34.1182298392761,-31.8689008451631,53.2605916310072));
#41692=CARTESIAN_POINT('Ctrl Pts',(33.038743527047,-30.1493218606453,53.3717214202269));
#41693=CARTESIAN_POINT('Ctrl Pts',(31.0087474497846,-30.1235332468791,53.4828512094467));
#41694=CARTESIAN_POINT('Ctrl Pts',(29.8856636535643,-31.8149284586479,53.5939809986663));
#41695=CARTESIAN_POINT('Ctrl Pts',(30.6981346884947,-33.6759727879679,53.7051107878861));
#41696=CARTESIAN_POINT('Ctrl Pts',(32.700994683846,-34.0026424037911,53.8162405771058));
#41697=CARTESIAN_POINT('Ctrl Pts',(34.0644271931817,-32.497600055013,53.9273703663256));
#41698=CARTESIAN_POINT('Ctrl Pts',(33.53422590936,-30.5348896671691,54.0385001555452));
#41699=CARTESIAN_POINT('Ctrl Pts',(32.2512547397667,-30.1245170851199,54.1125866816917));
#41700=CARTESIAN_POINT('Ctrl Pts',(31.6647242417508,-30.2359961244728,54.149629944765));
#41701=CARTESIAN_POINT('Ctrl Pts',(30.5335096305347,-30.7527339134291,40.850370055235));
#41702=CARTESIAN_POINT('Ctrl Pts',(30.1187942157535,-31.24034130402,40.8874133183083));
#41703=CARTESIAN_POINT('Ctrl Pts',(29.8214226984638,-32.653609247751,40.9614998444547));
#41704=CARTESIAN_POINT('Ctrl Pts',(31.3698258444113,-34.187854823872,41.0726296336745));
#41705=CARTESIAN_POINT('Ctrl Pts',(33.4951165000671,-33.7145957729538,41.1837594228942));
#41706=CARTESIAN_POINT('Ctrl Pts',(34.2519828063147,-31.6747035694605,41.2948892121139));
#41707=CARTESIAN_POINT('Ctrl Pts',(32.9479169971854,-29.9312398415937,41.4060190013337));
#41708=CARTESIAN_POINT('Ctrl Pts',(30.7762982546858,-30.0817286295349,41.5171487905534));
#41709=CARTESIAN_POINT('Ctrl Pts',(29.7246130378245,-31.9874724693811,41.6282785797731));
#41710=CARTESIAN_POINT('Ctrl Pts',(30.7553297352692,-33.9048460965428,41.7394083689928));
#41711=CARTESIAN_POINT('Ctrl Pts',(32.9251589791213,-34.0788420217823,41.8505381582126));
#41712=CARTESIAN_POINT('Ctrl Pts',(34.248290829534,-32.350346307071,41.9616679474322));
#41713=CARTESIAN_POINT('Ctrl Pts',(33.5138122687288,-30.3011962178666,42.0727977366521));
#41714=CARTESIAN_POINT('Ctrl Pts',(31.3939086440396,-29.8067836534655,42.1839275258717));
#41715=CARTESIAN_POINT('Ctrl Pts',(29.8286935041498,-31.3195734866563,42.2950573150915));
#41716=CARTESIAN_POINT('Ctrl Pts',(30.2506343968376,-33.4550850230024,42.4061871043112));
#41717=CARTESIAN_POINT('Ctrl Pts',(32.2735757818995,-34.2589171434105,42.5173168935309));
#41718=CARTESIAN_POINT('Ctrl Pts',(34.0461435461261,-32.9954134895391,42.6284466827507));
#41719=CARTESIAN_POINT('Ctrl Pts',(33.9461029426293,-30.8209178520377,42.7395764719703));
#41720=CARTESIAN_POINT('Ctrl Pts',(32.0650100224681,-29.7255055879618,42.8507062611902));
#41721=CARTESIAN_POINT('Ctrl Pts',(30.1244206388795,-30.7116858538886,42.9618360504098));
#41722=CARTESIAN_POINT('Ctrl Pts',(29.9003411446903,-32.8769173006301,43.0729658396296));
#41723=CARTESIAN_POINT('Ctrl Pts',(31.5978466660826,-34.2396035206334,43.1840956288493));
#41724=CARTESIAN_POINT('Ctrl Pts',(33.6633985569723,-33.5526288976471,43.295225418069));
#41725=CARTESIAN_POINT('Ctrl Pts',(34.2066261275962,-31.444705139231,43.4063552072888));
#41726=CARTESIAN_POINT('Ctrl Pts',(32.730373395972,-29.8449812184301,43.5174849965084));
#41727=CARTESIAN_POINT('Ctrl Pts',(30.5856908529926,-30.2175071148205,43.6286147857282));
#41728=CARTESIAN_POINT('Ctrl Pts',(29.7353687037756,-32.2213511701524,43.7397445749478));
#41729=CARTESIAN_POINT('Ctrl Pts',(30.957612557977,-34.0226170346326,43.8508743641677));
#41730=CARTESIAN_POINT('Ctrl Pts',(33.1338380948878,-33.9728057235782,43.9620041533873));
#41731=CARTESIAN_POINT('Ctrl Pts',(34.272387303324,-32.1175040083948,44.0731339426071));
#41732=CARTESIAN_POINT('Ctrl Pts',(33.3312722947699,-30.1546638990556,44.1842637318268));
#41733=CARTESIAN_POINT('Ctrl Pts',(31.1717913190904,-29.8806553774391,44.2953935210465));
#41734=CARTESIAN_POINT('Ctrl Pts',(29.7702779466297,-31.5462480710675,44.4065233102663));
#41735=CARTESIAN_POINT('Ctrl Pts',(30.409382017085,-33.6271096093139,44.517653099486));
#41736=CARTESIAN_POINT('Ctrl Pts',(32.5042024159702,-34.2188580783882,44.6287828887057));
#41737=CARTESIAN_POINT('Ctrl Pts',(34.1375822316071,-32.779931696634,44.7399126779255));
#41738=CARTESIAN_POINT('Ctrl Pts',(33.8146699699911,-30.6272202841281,44.8510424671452));
#41739=CARTESIAN_POINT('Ctrl Pts',(31.8309914311157,-29.7308619804117,44.9621722563648));
#41740=CARTESIAN_POINT('Ctrl Pts',(30.0019877016615,-30.9111941844455,45.0733020455847));
#41741=CARTESIAN_POINT('Ctrl Pts',(30.0015431601057,-33.0879896632673,45.1844318348043));
#41742=CARTESIAN_POINT('Ctrl Pts',(31.8300646460591,-34.2690688010235,45.2955616240241));
#41743=CARTESIAN_POINT('Ctrl Pts',(33.8141091250671,-33.3735207791094,45.4066914132438));
#41744=CARTESIAN_POINT('Ctrl Pts',(34.1379006060079,-31.2209414353671,45.5178212024636));
#41745=CARTESIAN_POINT('Ctrl Pts',(32.505108636897,-29.7813480414384,45.6289509916832));
#41746=CARTESIAN_POINT('Ctrl Pts',(30.4100467209729,-30.3722408597067,45.740080780903));
#41747=CARTESIAN_POINT('Ctrl Pts',(29.7700928036892,-32.4528411908587,45.8512105701227));
#41748=CARTESIAN_POINT('Ctrl Pts',(31.1709257701325,-34.1190061749949,45.9623403593425));
#41749=CARTESIAN_POINT('Ctrl Pts',(33.3305184808149,-33.8458796874409,46.0734701485621));
#41750=CARTESIAN_POINT('Ctrl Pts',(34.2724351067276,-31.8834241276727,46.1845999377819));
#41751=CARTESIAN_POINT('Ctrl Pts',(33.1346437664958,-30.0276575420456,46.2957297270016));
#41752=CARTESIAN_POINT('Ctrl Pts',(30.9584387558662,-29.9769573847752,46.4068595162214));
#41753=CARTESIAN_POINT('Ctrl Pts',(29.7354593006066,-31.7777238899748,46.517989305441));
#41754=CARTESIAN_POINT('Ctrl Pts',(30.5849629355105,-33.7819150805856,46.6291190946608));
#41755=CARTESIAN_POINT('Ctrl Pts',(32.7294931463973,-34.1553169135087,46.7402488838805));
#41756=CARTESIAN_POINT('Ctrl Pts',(34.2063991407249,-32.5561960806273,46.8513786731002));
#41757=CARTESIAN_POINT('Ctrl Pts',(33.6640325688636,-30.4480506264512,46.96250846232));
#41758=CARTESIAN_POINT('Ctrl Pts',(31.5987614356599,-29.7602324087568,47.0736382515397));
#41759=CARTESIAN_POINT('Ctrl Pts',(29.9006994852894,-31.1222252013001,47.1847680407595));
#41760=CARTESIAN_POINT('Ctrl Pts',(30.1238946000158,-33.2875479705422,47.2958978299791));
#41761=CARTESIAN_POINT('Ctrl Pts',(32.064081031292,-34.2745208000205,47.407027619199));
#41762=CARTESIAN_POINT('Ctrl Pts',(33.9456211976595,-33.1798768594709,47.5181574084186));
#41763=CARTESIAN_POINT('Ctrl Pts',(34.0465499433124,-31.0054224123653,47.6292871976384));
#41764=CARTESIAN_POINT('Ctrl Pts',(32.2744983747557,-29.7411945877182,47.740416986858));
#41765=CARTESIAN_POINT('Ctrl Pts',(30.2512288704335,-30.5442009806667,47.8515467760778));
#41766=CARTESIAN_POINT('Ctrl Pts',(29.8284157392574,-32.6795388486261,47.9626765652975));
#41767=CARTESIAN_POINT('Ctrl Pts',(31.3930129736622,-34.1929701316148,48.0738063545172));
#41768=CARTESIAN_POINT('Ctrl Pts',(33.5131181520712,-33.6994189319205,48.184936143737));
#41769=CARTESIAN_POINT('Ctrl Pts',(34.2484340067877,-31.6505779551634,48.2960659329566));
#41770=CARTESIAN_POINT('Ctrl Pts',(32.9260074417436,-29.9215242445165,48.4071957221765));
#41771=CARTESIAN_POINT('Ctrl Pts',(30.7561089081482,-30.0946690051571,48.5183255113961));
#41772=CARTESIAN_POINT('Ctrl Pts',(29.7246060123785,-32.0115520298237,48.6294553006159));
#41773=CARTESIAN_POINT('Ctrl Pts',(30.7755190184597,-33.9178627620722,48.7405850898356));
#41774=CARTESIAN_POINT('Ctrl Pts',(32.9470637399033,-34.0689662928278,48.8517148790554));
#41775=CARTESIAN_POINT('Ctrl Pts',(34.2518659970659,-32.3265743093926,48.962844668275));
#41776=CARTESIAN_POINT('Ctrl Pts',(33.4957849141838,-30.2853050595522,49.0739744574949));
#41777=CARTESIAN_POINT('Ctrl Pts',(31.3707776989525,-29.8133060241173,49.1851042467144));
#41778=CARTESIAN_POINT('Ctrl Pts',(29.8216279100082,-31.3425456017016,49.2962340359344));
#41779=CARTESIAN_POINT('Ctrl Pts',(30.2661006343628,-33.4734803148125,49.4073638251539));
#41780=CARTESIAN_POINT('Ctrl Pts',(32.2974192547929,-34.2559018230357,49.5184936143738));
#41781=CARTESIAN_POINT('Ctrl Pts',(34.056542998614,-32.9737464470531,49.6296234035933));
#41782=CARTESIAN_POINT('Ctrl Pts',(33.9335408923838,-30.8004288825681,49.7407531928132));
#41783=CARTESIAN_POINT('Ctrl Pts',(32.0409831298217,-29.7249457959496,49.8518829820328));
#41784=CARTESIAN_POINT('Ctrl Pts',(30.1109180512903,-30.7315676449427,49.9630127712527));
#41785=CARTESIAN_POINT('Ctrl Pts',(29.9097202859775,-32.8990450297081,50.0741425604723));
#41786=CARTESIAN_POINT('Ctrl Pts',(31.6215238467982,-34.2437261530219,50.1852723496921));
#41787=CARTESIAN_POINT('Ctrl Pts',(33.6797046786269,-33.5349734332873,50.2964021389118));
#41788=CARTESIAN_POINT('Ctrl Pts',(34.2006380042136,-31.4214296735012,50.4075319281315));
#41789=CARTESIAN_POINT('Ctrl Pts',(32.7075712932722,-29.8373872021944,50.5186617173513));
#41790=CARTESIAN_POINT('Ctrl Pts',(30.5669430080136,-30.2325445108771,50.6297915065709));
#41791=CARTESIAN_POINT('Ctrl Pts',(29.7378329409762,-32.2452579159542,50.7409212957907));
#41792=CARTESIAN_POINT('Ctrl Pts',(30.979033634155,-34.0335139360501,50.8520510850104));
#41793=CARTESIAN_POINT('Ctrl Pts',(33.1546116734798,-33.9607200544356,50.9631808742302));
#41794=CARTESIAN_POINT('Ctrl Pts',(34.2735016303912,-32.093496442081,51.0743106634498));
#41795=CARTESIAN_POINT('Ctrl Pts',(33.3117075504391,-30.1407058999481,51.1854404526696));
#41796=CARTESIAN_POINT('Ctrl Pts',(31.1494529448607,-29.8895211548044,51.2965702418893));
#41797=CARTESIAN_POINT('Ctrl Pts',(29.7656097810211,-31.5698237619369,51.4077000311091));
#41798=CARTESIAN_POINT('Ctrl Pts',(30.4266563133037,-33.6438189963982,51.5188298203287));
#41799=CARTESIAN_POINT('Ctrl Pts',(32.5276099280905,-34.2134089131759,51.6299596095486));
#41800=CARTESIAN_POINT('Ctrl Pts',(34.1457006531511,-32.7573109933717,51.7410893987682));
#41801=CARTESIAN_POINT('Ctrl Pts',(33.8000694199542,-30.6081302704023,51.852219187988));
#41802=CARTESIAN_POINT('Ctrl Pts',(31.8070341540629,-29.7327736193239,51.9633489772077));
#41803=CARTESIAN_POINT('Ctrl Pts',(29.9905991783125,-30.9323579854575,52.0744787664274));
#41804=CARTESIAN_POINT('Ctrl Pts',(30.0131459632196,-33.1090367042992,52.1856085556471));
#41805=CARTESIAN_POINT('Ctrl Pts',(31.8540401750289,-34.2707371393458,52.2967383448669));
#41806=CARTESIAN_POINT('Ctrl Pts',(33.8285149210735,-33.3542834092786,52.4078681340866));
#41807=CARTESIAN_POINT('Ctrl Pts',(34.1295532637732,-31.1984045069698,52.5189979233063));
#41808=CARTESIAN_POINT('Ctrl Pts',(32.4816463202079,-29.7761364787351,52.630127712526));
#41809=CARTESIAN_POINT('Ctrl Pts',(30.3929443290853,-30.3891254719696,52.7412575017458));
#41810=CARTESIAN_POINT('Ctrl Pts',(29.7749974270505,-32.4763669022007,52.8523872909655));
#41811=CARTESIAN_POINT('Ctrl Pts',(31.1933583183665,-34.1276473830258,52.9635170801852));
#41812=CARTESIAN_POINT('Ctrl Pts',(33.349929988658,-33.8317184046403,53.0746468694049));
#41813=CARTESIAN_POINT('Ctrl Pts',(34.2710978673113,-31.8594397050614,53.1857766586247));
#41814=CARTESIAN_POINT('Ctrl Pts',(33.1137073820875,-30.015762455313,53.2969064478444));
#41815=CARTESIAN_POINT('Ctrl Pts',(30.9372109149731,-29.9881127335314,53.4080362370641));
#41816=CARTESIAN_POINT('Ctrl Pts',(29.7330766104164,-31.8015722491152,53.5191660262839));
#41817=CARTESIAN_POINT('Ctrl Pts',(30.6041819080895,-33.7969240890906,53.6302958155036));
#41818=CARTESIAN_POINT('Ctrl Pts',(32.7515839414401,-34.1471687386821,53.7414256047233));
#41819=CARTESIAN_POINT('Ctrl Pts',(34.2134124015819,-32.5335107658101,53.852555393943));
#41820=CARTESIAN_POINT('Ctrl Pts',(33.6449476473772,-30.4291558495818,53.9636851831628));
#41821=CARTESIAN_POINT('Ctrl Pts',(32.2693872463958,-29.9891675732325,54.0377717093093));
#41822=CARTESIAN_POINT('Ctrl Pts',(31.640528121452,-30.1086918117405,54.0748149723825));
#41823=CARTESIAN_POINT('Ctrl Pts',(30.4347998857282,-30.6687801966678,40.7755550828525));
#41824=CARTESIAN_POINT('Ctrl Pts',(29.9921698977506,-31.1892085331669,40.8125983459258));
#41825=CARTESIAN_POINT('Ctrl Pts',(29.6747822472522,-32.6976038101375,40.8866848720723));
#41826=CARTESIAN_POINT('Ctrl Pts',(31.3274087025214,-34.3351197468709,40.997814661292));
#41827=CARTESIAN_POINT('Ctrl Pts',(33.5957530751518,-33.8300055395084,41.1089444505117));
#41828=CARTESIAN_POINT('Ctrl Pts',(34.40356419597,-31.6528078050466,41.2200742397314));
#41829=CARTESIAN_POINT('Ctrl Pts',(33.0117214699854,-29.7919912031069,41.3312040289512));
#41830=CARTESIAN_POINT('Ctrl Pts',(30.6939306582022,-29.9526094198962,41.4423338181709));
#41831=CARTESIAN_POINT('Ctrl Pts',(29.5714563100008,-31.9866292389199,41.5534636073906));
#41832=CARTESIAN_POINT('Ctrl Pts',(30.6715507437682,-34.0330616484485,41.6645933966103));
#41833=CARTESIAN_POINT('Ctrl Pts',(32.9874316054104,-34.2187692724043,41.7757231858301));
#41834=CARTESIAN_POINT('Ctrl Pts',(34.3996237115323,-32.3739281834235,41.8868529750498));
#41835=CARTESIAN_POINT('Ctrl Pts',(33.6157072595466,-30.1868494132083,41.9979827642695));
#41836=CARTESIAN_POINT('Ctrl Pts',(31.3531125199586,-29.6591578453596,42.1091125534892));
#41837=CARTESIAN_POINT('Ctrl Pts',(29.6825424522475,-31.2737738490384,42.220242342709));
#41838=CARTESIAN_POINT('Ctrl Pts',(30.1328842664196,-33.553027071776,42.3313721319287));
#41839=CARTESIAN_POINT('Ctrl Pts',(32.2919902196474,-34.4109652846105,42.4425019211484));
#41840=CARTESIAN_POINT('Ctrl Pts',(34.1838698561524,-33.0624149602443,42.5536317103682));
#41841=CARTESIAN_POINT('Ctrl Pts',(34.077095500667,-30.7415536091116,42.6647614995879));
#41842=CARTESIAN_POINT('Ctrl Pts',(32.0693858594061,-29.572408937857,42.7758912888076));
#41843=CARTESIAN_POINT('Ctrl Pts',(29.9981750364838,-30.6249691844573,42.8870210780273));
#41844=CARTESIAN_POINT('Ctrl Pts',(29.7590127090568,-32.9359427703937,42.9981508672471));
#41845=CARTESIAN_POINT('Ctrl Pts',(31.5707776489307,-34.3903516582226,43.1092806564667));
#41846=CARTESIAN_POINT('Ctrl Pts',(33.7753622292125,-33.6571366431167,43.2204104456866));
#41847=CARTESIAN_POINT('Ctrl Pts',(34.3551545506076,-31.4073281368721,43.3315402349062));
#41848=CARTESIAN_POINT('Ctrl Pts',(32.7795349677293,-29.699926495664,43.442670024126));
#41849=CARTESIAN_POINT('Ctrl Pts',(30.490493436163,-30.0975271807692,43.5537998133457));
#41850=CARTESIAN_POINT('Ctrl Pts',(29.5829359418664,-32.2362503593823,43.6649296025654));
#41851=CARTESIAN_POINT('Ctrl Pts',(30.887449261624,-34.1587597707098,43.7760593917852));
#41852=CARTESIAN_POINT('Ctrl Pts',(33.2101569520236,-34.1055956508643,43.8871891810049));
#41853=CARTESIAN_POINT('Ctrl Pts',(34.4253421235416,-32.1254132254779,43.9983189702246));
#41854=CARTESIAN_POINT('Ctrl Pts',(33.420880485332,-30.0304539762364,44.1094487594444));
#41855=CARTESIAN_POINT('Ctrl Pts',(31.116044435755,-29.7380018890796,44.220578548664));
#41856=CARTESIAN_POINT('Ctrl Pts',(29.6201949324755,-31.5157059427025,44.3317083378838));
#41857=CARTESIAN_POINT('Ctrl Pts',(30.3023172190834,-33.7366306656069,44.4428381271035));
#41858=CARTESIAN_POINT('Ctrl Pts',(32.538140376183,-34.3682098363267,44.5539679163233));
#41859=CARTESIAN_POINT('Ctrl Pts',(34.2814632968893,-32.8324290470048,44.6650977055429));
#41860=CARTESIAN_POINT('Ctrl Pts',(33.9368157497217,-30.5348182211821,44.7762274947627));
#41861=CARTESIAN_POINT('Ctrl Pts',(31.819615432301,-29.5781258700983,44.8873572839824));
#41862=CARTESIAN_POINT('Ctrl Pts',(29.8675011150493,-30.8379064585695,44.9984870732022));
#41863=CARTESIAN_POINT('Ctrl Pts',(29.867026651317,-33.1612224537781,45.1096168624218));
#41864=CARTESIAN_POINT('Ctrl Pts',(31.8186262651666,-34.4218002522221,45.2207466516416));
#41865=CARTESIAN_POINT('Ctrl Pts',(33.9362171542195,-33.4659727231625,45.3318764408613));
#41866=CARTESIAN_POINT('Ctrl Pts',(34.2818031011314,-31.1685028556768,45.443006230081));
#41867=CARTESIAN_POINT('Ctrl Pts',(32.539107595012,-29.6320101574646,45.5541360193008));
#41868=CARTESIAN_POINT('Ctrl Pts',(30.3030266643161,-30.2626760833603,45.6652658085204));
#41869=CARTESIAN_POINT('Ctrl Pts',(29.6199973275285,-32.4833220172713,45.7763955977403));
#41870=CARTESIAN_POINT('Ctrl Pts',(31.1151206265327,-34.2616368823846,45.88752538696));
#41871=CARTESIAN_POINT('Ctrl Pts',(33.4200759320169,-33.9701261991703,45.9986551761797));
#41872=CARTESIAN_POINT('Ctrl Pts',(34.4253931446014,-31.8755773836041,46.1097849653994));
#41873=CARTESIAN_POINT('Ctrl Pts',(33.2110168535402,-29.8948987972565,46.2209147546191));
#41874=CARTESIAN_POINT('Ctrl Pts',(30.8883310710498,-29.8407860027877,46.3320445438389));
#41875=CARTESIAN_POINT('Ctrl Pts',(29.5830326367871,-31.7627624428669,46.4431743330586));
#41876=CARTESIAN_POINT('Ctrl Pts',(30.4897165224173,-33.9018561225001,46.5543041222784));
#41877=CARTESIAN_POINT('Ctrl Pts',(32.7785954683888,-34.300391703592,46.665433911498));
#41878=CARTESIAN_POINT('Ctrl Pts',(34.3549122852071,-32.5936337442658,46.7765637007178));
#41879=CARTESIAN_POINT('Ctrl Pts',(33.7760389165643,-30.3435886198774,46.8876934899375));
#41880=CARTESIAN_POINT('Ctrl Pts',(31.5717539918218,-29.6094732275437,46.9988232791572));
#41881=CARTESIAN_POINT('Ctrl Pts',(29.7593951696295,-31.0631420131788,47.1099530683769));
#41882=CARTESIAN_POINT('Ctrl Pts',(29.9976135898446,-33.3742130685507,47.2210828575967));
#41883=CARTESIAN_POINT('Ctrl Pts',(32.0683943376577,-34.4276192263053,47.3322126468163));
#41884=CARTESIAN_POINT('Ctrl Pts',(34.0765813293521,-33.2592945945794,47.4433424360362));
#41885=CARTESIAN_POINT('Ctrl Pts',(34.1843036080103,-30.9384772063757,47.5544722252558));
#41886=CARTESIAN_POINT('Ctrl Pts',(32.2929749124037,-29.5891539671616,47.6656020144756));
#41887=CARTESIAN_POINT('Ctrl Pts',(30.1335187541459,-30.4462108726646,47.7767318036953));
#41888=CARTESIAN_POINT('Ctrl Pts',(29.6822459909475,-32.7252787373636,47.8878615929151));
#41889=CARTESIAN_POINT('Ctrl Pts',(31.3521565618384,-34.3405793669477,47.9989913821348));
#41890=CARTESIAN_POINT('Ctrl Pts',(33.6149664217652,-33.8138071424277,48.1101211713545));
#41891=CARTESIAN_POINT('Ctrl Pts',(34.3997765260741,-31.6270582910771,48.2212509605742));
#41892=CARTESIAN_POINT('Ctrl Pts',(32.9883371782127,-29.7816216473485,48.3323807497939));
#41893=CARTESIAN_POINT('Ctrl Pts',(30.6723823629214,-29.966420814655,48.4435105390137));
#41894=CARTESIAN_POINT('Ctrl Pts',(29.5714488116707,-32.0123295991414,48.5546403282333));
#41895=CARTESIAN_POINT('Ctrl Pts',(30.693098971438,-34.0469544682025,48.6657701174531));
#41896=CARTESIAN_POINT('Ctrl Pts',(33.0108107797937,-34.2082288062616,48.7768999066728));
#41897=CARTESIAN_POINT('Ctrl Pts',(34.4034395242687,-32.3485560880743,48.8880296958926));
#41898=CARTESIAN_POINT('Ctrl Pts',(33.5964664803493,-30.1698886180148,48.9991594851123));
#41899=CARTESIAN_POINT('Ctrl Pts',(31.3284246265722,-29.6661192380166,49.1102892743321));
#41900=CARTESIAN_POINT('Ctrl Pts',(29.6750012716246,-31.2982922215028,49.2214190635517));
#41901=CARTESIAN_POINT('Ctrl Pts',(30.1493915393249,-33.5726605541655,49.3325488527715));
#41902=CARTESIAN_POINT('Ctrl Pts',(32.317438601222,-34.4077470024496,49.4436786419912));
#41903=CARTESIAN_POINT('Ctrl Pts',(34.1949692977589,-33.0392895050207,49.5548084312109));
#41904=CARTESIAN_POINT('Ctrl Pts',(34.0636878964378,-30.7196855232223,49.6659382204306));
#41905=CARTESIAN_POINT('Ctrl Pts',(32.0437417120601,-29.5718114661385,49.7770680096504));
#41906=CARTESIAN_POINT('Ctrl Pts',(29.9837635871641,-30.6461892226366,49.8881977988701));
#41907=CARTESIAN_POINT('Ctrl Pts',(29.7690231621222,-32.9595599211113,49.9993275880899));
#41908=CARTESIAN_POINT('Ctrl Pts',(31.5960485451694,-34.3947517857787,50.1104573773095));
#41909=CARTESIAN_POINT('Ctrl Pts',(33.7927659190072,-33.6382927861036,50.2215871665294));
#41910=CARTESIAN_POINT('Ctrl Pts',(34.3487633655049,-31.3824859951311,50.332716955749));
#41911=CARTESIAN_POINT('Ctrl Pts',(32.7551980511737,-29.6918213247557,50.4438467449688));
#41912=CARTESIAN_POINT('Ctrl Pts',(30.470483670184,-30.1135767468053,50.5549765341884));
#41913=CARTESIAN_POINT('Ctrl Pts',(29.5855660473401,-32.2617662727765,50.6661063234083));
#41914=CARTESIAN_POINT('Ctrl Pts',(30.9103121945009,-34.1703901446276,50.7772361126279));
#41915=CARTESIAN_POINT('Ctrl Pts',(33.2323288041292,-34.0926964930404,50.8883659018477));
#41916=CARTESIAN_POINT('Ctrl Pts',(34.426531456175,-32.0997897053238,50.9994956910673));
#41917=CARTESIAN_POINT('Ctrl Pts',(33.399998834351,-30.0155564615627,51.1106254802872));
#41918=CARTESIAN_POINT('Ctrl Pts',(31.0922024613207,-29.7474644236002,51.2217552695068));
#41919=CARTESIAN_POINT('Ctrl Pts',(29.6152125517546,-31.5408685177941,51.3328850587265));
#41920=CARTESIAN_POINT('Ctrl Pts',(30.3207542514557,-33.7544647647039,51.4440148479463));
#41921=CARTESIAN_POINT('Ctrl Pts',(32.563123452382,-34.3623938867708,51.555144637166));
#41922=CARTESIAN_POINT('Ctrl Pts',(34.2901281709266,-32.8082857399171,51.6662744263857));
#41923=CARTESIAN_POINT('Ctrl Pts',(33.9212324338936,-30.5144432550129,51.7774042156054));
#41924=CARTESIAN_POINT('Ctrl Pts',(31.7940455863876,-29.5801661817881,51.8885340048252));
#41925=CARTESIAN_POINT('Ctrl Pts',(29.8553460280345,-30.8604947990401,51.9996637940449));
#41926=CARTESIAN_POINT('Ctrl Pts',(29.8794104413083,-33.1836861751323,52.1107935832647));
#41927=CARTESIAN_POINT('Ctrl Pts',(31.844215591537,-34.4235808867133,52.2219233724843));
#41928=CARTESIAN_POINT('Ctrl Pts',(33.9515926070864,-33.4454404823211,52.3330531617041));
#41929=CARTESIAN_POINT('Ctrl Pts',(34.2728938977083,-31.1444489623563,52.4441829509238));
#41930=CARTESIAN_POINT('Ctrl Pts',(32.5140660253384,-29.6264478034877,52.5553127401435));
#41931=CARTESIAN_POINT('Ctrl Pts',(30.284773107188,-30.2806972020757,52.6664425293633));
#41932=CARTESIAN_POINT('Ctrl Pts',(29.6252320820182,-32.5084312487041,52.777572318583));
#41933=CARTESIAN_POINT('Ctrl Pts',(31.1390631138414,-34.2708597317664,52.8887021078028));
#41934=CARTESIAN_POINT('Ctrl Pts',(33.4407940321331,-33.9550117177394,52.9998318970224));
#41935=CARTESIAN_POINT('Ctrl Pts',(34.4239658953466,-31.8499785649598,53.1109616862422));
#41936=CARTESIAN_POINT('Ctrl Pts',(33.188671237128,-29.8822030499806,53.2220914754619));
#41937=CARTESIAN_POINT('Ctrl Pts',(30.8656743801615,-29.8526922201837,53.3332212646816));
#41938=CARTESIAN_POINT('Ctrl Pts',(29.5804895672685,-31.7882160395824,53.4443510539014));
#41939=CARTESIAN_POINT('Ctrl Pts',(30.5102291276843,-33.9178753902133,53.5554808431211));
#41940=CARTESIAN_POINT('Ctrl Pts',(32.8021731990342,-34.291695073573,53.6666106323408));
#41941=CARTESIAN_POINT('Ctrl Pts',(34.362397609982,-32.5694214766073,53.7777404215605));
#41942=CARTESIAN_POINT('Ctrl Pts',(33.7556693853943,-30.3234220319946,53.8888702107803));
#41943=CARTESIAN_POINT('Ctrl Pts',(32.2875197530249,-29.8538180613451,53.9629567369268));
#41944=CARTESIAN_POINT('Ctrl Pts',(31.6163320011532,-29.9813874990081,54.));
#41945=CARTESIAN_POINT('Ctrl Pts',(30.7309291201476,-30.9206413469515,41.));
#41946=CARTESIAN_POINT('Ctrl Pts',(30.6855978806243,-30.9629305822782,41.));
#41947=CARTESIAN_POINT('Ctrl Pts',(30.6429965177354,-31.0077887820157,41.));
#41948=CARTESIAN_POINT('Ctrl Pts',(30.6031236390744,-31.0548709612839,41.));
#41949=CARTESIAN_POINT('Ctrl Pts',(30.5606226453807,-31.1050564375116,41.));
#41950=CARTESIAN_POINT('Ctrl Pts',(30.5212209469281,-31.1577689646829,41.));
#41951=CARTESIAN_POINT('Ctrl Pts',(30.4849456787917,-31.2126454473402,41.));
#41952=CARTESIAN_POINT('Ctrl Pts',(30.4532048191724,-31.2606623696652,41.));
#41953=CARTESIAN_POINT('Ctrl Pts',(30.4238578759431,-31.3103372955829,41.));
#41954=CARTESIAN_POINT('Ctrl Pts',(30.3969459135927,-31.3614545259121,41.));
#41955=CARTESIAN_POINT('Ctrl Pts',(30.383446347189,-31.3870959279109,41.));
#41956=CARTESIAN_POINT('Ctrl Pts',(30.3705598364866,-31.4131006012838,41.));
#41957=CARTESIAN_POINT('Ctrl Pts',(30.3582939048221,-31.4394431609949,41.));
#41958=CARTESIAN_POINT('Ctrl Pts',(30.3526827339958,-31.451493823479,41.));
#41959=CARTESIAN_POINT('Ctrl Pts',(30.3472008500408,-31.4636168867931,41.));
#41960=CARTESIAN_POINT('Ctrl Pts',(30.3418574940955,-31.4757899451731,41.));
#41961=CARTESIAN_POINT('Ctrl Pts',(30.3149359070818,-31.537121822321,41.));
#41962=CARTESIAN_POINT('Ctrl Pts',(30.2914755974925,-31.5998291482412,41.));
#41963=CARTESIAN_POINT('Ctrl Pts',(30.2715001667511,-31.6635542174867,41.));
#41964=CARTESIAN_POINT('Ctrl Pts',(30.2511707190549,-31.7284086618758,41.));
#41965=CARTESIAN_POINT('Ctrl Pts',(30.2344502095525,-31.7943180848097,41.));
#41966=CARTESIAN_POINT('Ctrl Pts',(30.2214028317259,-31.8609419339526,41.));
#41967=CARTESIAN_POINT('Ctrl Pts',(30.2104912353279,-31.9166598384991,41.));
#41968=CARTESIAN_POINT('Ctrl Pts',(30.2021492089366,-31.972878358886,41.));
#41969=CARTESIAN_POINT('Ctrl Pts',(30.1964391172512,-32.0294105816203,41.));
#41970=CARTESIAN_POINT('Ctrl Pts',(30.1938093347234,-32.055446494841,41.));
#41971=CARTESIAN_POINT('Ctrl Pts',(30.1917381369785,-32.0815490593274,41.));
#41972=CARTESIAN_POINT('Ctrl Pts',(30.1902334165381,-32.1077004172633,41.));
#41973=CARTESIAN_POINT('Ctrl Pts',(30.1895753812609,-32.1191367715564,41.));
#41974=CARTESIAN_POINT('Ctrl Pts',(30.1890257975943,-32.1305822670034,41.));
#41975=CARTESIAN_POINT('Ctrl Pts',(30.1885856619553,-32.1420212484968,41.));
#41976=CARTESIAN_POINT('Ctrl Pts',(30.1858874976538,-32.2121456573693,41.));
#41977=CARTESIAN_POINT('Ctrl Pts',(30.1872903022448,-32.2821566391967,41.));
#41978=CARTESIAN_POINT('Ctrl Pts',(30.1928488011416,-32.3516934917122,41.));
#41979=CARTESIAN_POINT('Ctrl Pts',(30.1978161829043,-32.4138354655506,41.));
#41980=CARTESIAN_POINT('Ctrl Pts',(30.2061027353294,-32.4755997535043,41.));
#41981=CARTESIAN_POINT('Ctrl Pts',(30.217780599423,-32.5367410473977,41.));
#41982=CARTESIAN_POINT('Ctrl Pts',(30.230508640649,-32.6033807088163,41.));
#41983=CARTESIAN_POINT('Ctrl Pts',(30.2472642836697,-32.6692811201171,41.));
#41984=CARTESIAN_POINT('Ctrl Pts',(30.267802240865,-32.7342286370083,41.));
#41985=CARTESIAN_POINT('Ctrl Pts',(30.2757344649613,-32.7593128385954,41.));
#41986=CARTESIAN_POINT('Ctrl Pts',(30.2842314436902,-32.7842548517836,41.));
#41987=CARTESIAN_POINT('Ctrl Pts',(30.2932810585363,-32.8090420474308,41.));
#41988=CARTESIAN_POINT('Ctrl Pts',(30.2972495255297,-32.8199118103387,41.));
#41989=CARTESIAN_POINT('Ctrl Pts',(30.3013241696228,-32.8307512478403,41.));
#41990=CARTESIAN_POINT('Ctrl Pts',(30.3054988752419,-32.8415467359126,41.));
#41991=CARTESIAN_POINT('Ctrl Pts',(30.3307215131888,-32.9067706611294,41.));
#41992=CARTESIAN_POINT('Ctrl Pts',(30.3596350679945,-32.9705095691753,41.));
#41993=CARTESIAN_POINT('Ctrl Pts',(30.3919268344823,-33.0325445786466,41.));
#41994=CARTESIAN_POINT('Ctrl Pts',(30.4249669781864,-33.0960172792927,41.));
#41995=CARTESIAN_POINT('Ctrl Pts',(30.461544033557,-33.1577070082778,41.));
#41996=CARTESIAN_POINT('Ctrl Pts',(30.5013791864624,-33.2173756043833,41.));
#41997=CARTESIAN_POINT('Ctrl Pts',(30.5318851553063,-33.2630701279634,41.));
#41998=CARTESIAN_POINT('Ctrl Pts',(30.5643030759919,-33.3075793757001,41.));
#41999=CARTESIAN_POINT('Ctrl Pts',(30.5985273064738,-33.3507902757675,41.));
#42000=CARTESIAN_POINT('Ctrl Pts',(30.6198359272625,-33.3776941584995,41.));
#42001=CARTESIAN_POINT('Ctrl Pts',(30.6418450939684,-33.4040946096701,41.));
#42002=CARTESIAN_POINT('Ctrl Pts',(30.6645322221831,-33.4299626453368,41.));
#42003=CARTESIAN_POINT('Ctrl Pts',(30.6771875615082,-33.444392359223,41.));
#42004=CARTESIAN_POINT('Ctrl Pts',(30.6900582984156,-33.4586609103331,41.));
#42005=CARTESIAN_POINT('Ctrl Pts',(30.7031169141315,-33.4727379551488,41.));
#42006=CARTESIAN_POINT('Ctrl Pts',(30.7539897162477,-33.527578279029,41.));
#42007=CARTESIAN_POINT('Ctrl Pts',(30.8077590845298,-33.5795736788928,41.));
#42008=CARTESIAN_POINT('Ctrl Pts',(30.8641400026091,-33.6284601407826,41.));
#42009=CARTESIAN_POINT('Ctrl Pts',(30.9062939577409,-33.665010764491,41.));
#42010=CARTESIAN_POINT('Ctrl Pts',(30.9499089277002,-33.6998232910283,41.));
#42011=CARTESIAN_POINT('Ctrl Pts',(30.9948821713292,-33.732777639113,41.));
#42012=CARTESIAN_POINT('Ctrl Pts',(31.008966379297,-33.74309790633,41.));
#42013=CARTESIAN_POINT('Ctrl Pts',(31.0231838921667,-33.7532358564134,41.));
#42014=CARTESIAN_POINT('Ctrl Pts',(31.0375317968707,-33.7631875733228,41.));
#42015=CARTESIAN_POINT('Ctrl Pts',(31.0513138213297,-33.7727467952917,41.));
#42016=CARTESIAN_POINT('Ctrl Pts',(31.0652090990272,-33.782129227744,41.));
#42017=CARTESIAN_POINT('Ctrl Pts',(31.0792097130569,-33.791328684408,41.));
#42018=CARTESIAN_POINT('Ctrl Pts',(31.1421653737961,-33.8326952895796,41.));
#42019=CARTESIAN_POINT('Ctrl Pts',(31.2072783450083,-33.8703859700674,41.));
#42020=CARTESIAN_POINT('Ctrl Pts',(31.2742872744703,-33.9041214598101,41.));
#42021=CARTESIAN_POINT('Ctrl Pts',(31.3254777357978,-33.9298931785482,41.));
#42022=CARTESIAN_POINT('Ctrl Pts',(31.3777756457353,-33.9533562526433,41.));
#42023=CARTESIAN_POINT('Ctrl Pts',(31.4310783175737,-33.9743709615764,41.));
#42024=CARTESIAN_POINT('Ctrl Pts',(31.4435634323603,-33.9792932486624,41.));
#42025=CARTESIAN_POINT('Ctrl Pts',(31.4561037167888,-33.9840811412651,41.));
#42026=CARTESIAN_POINT('Ctrl Pts',(31.4686972148566,-33.9887352337365,41.));
#42027=CARTESIAN_POINT('Ctrl Pts',(33.6673070425528,-32.0013037875835,42.1285196366098));
#42028=CARTESIAN_POINT('Ctrl Pts',(33.6680432508362,-32.0869536148502,42.1227790551389));
#42029=CARTESIAN_POINT('Ctrl Pts',(33.6620131902561,-32.1724994405965,42.1170384736681));
#42030=CARTESIAN_POINT('Ctrl Pts',(33.6488560459642,-32.2569345941976,42.1112978921973));
#42031=CARTESIAN_POINT('Ctrl Pts',(33.5639546192058,-32.8017842097567,42.074254629124));
#42032=CARTESIAN_POINT('Ctrl Pts',(33.1822841728743,-33.3003858651474,42.0372113660508));
#42033=CARTESIAN_POINT('Ctrl Pts',(32.6784946149966,-33.5245912715416,42.0001681029776));
#42034=CARTESIAN_POINT('Ctrl Pts',(32.1747050571189,-33.7487966779359,41.9631248399043));
#42035=CARTESIAN_POINT('Ctrl Pts',(31.5487963876951,-33.6986058353337,41.9260815768311));
#42036=CARTESIAN_POINT('Ctrl Pts',(31.0871818488499,-33.3969677369612,41.8890383137578));
#42037=CARTESIAN_POINT('Ctrl Pts',(30.6255673100048,-33.0953296385888,41.8519950506846));
#42038=CARTESIAN_POINT('Ctrl Pts',(30.3282469017383,-32.542244284446,41.8149517876113));
#42039=CARTESIAN_POINT('Ctrl Pts',(30.3312711899686,-31.9908362937928,41.7779085245381));
#42040=CARTESIAN_POINT('Ctrl Pts',(30.3342954781989,-31.4394283031396,41.7408652614648));
#42041=CARTESIAN_POINT('Ctrl Pts',(30.6376644629259,-30.889697675976,41.7038219983916));
#42042=CARTESIAN_POINT('Ctrl Pts',(31.1025613892782,-30.59312737402,41.6667787353184));
#42043=CARTESIAN_POINT('Ctrl Pts',(31.5674583156305,-30.296557072064,41.6297354722451));
#42044=CARTESIAN_POINT('Ctrl Pts',(32.1938831836081,-30.2531470953156,41.5926922091719));
#42045=CARTESIAN_POINT('Ctrl Pts',(32.6951809468332,-30.4829017702283,41.5556489460986));
#42046=CARTESIAN_POINT('Ctrl Pts',(33.1964787100584,-30.7126564451409,41.5186056830254));
#42047=CARTESIAN_POINT('Ctrl Pts',(33.5726493685311,-31.2155757717146,41.4815624199521));
#42048=CARTESIAN_POINT('Ctrl Pts',(33.6515719182498,-31.7612489585941,41.4445191568789));
#42049=CARTESIAN_POINT('Ctrl Pts',(33.6629345145688,-31.839810335117,41.4391859834559));
#42050=CARTESIAN_POINT('Ctrl Pts',(33.6681358153543,-31.9192579045568,41.4338528100328));
#42051=CARTESIAN_POINT('Ctrl Pts',(33.6674738845699,-31.9987897819954,41.4285196366098));
#42052=CARTESIAN_POINT('Ctrl Pts',(32.5301702171886,-33.9851743256717,41.));
#42053=CARTESIAN_POINT('Ctrl Pts',(33.1902397907527,-33.8088929660699,41.0370432630732));
#42054=CARTESIAN_POINT('Ctrl Pts',(34.309243415742,-32.7487884047516,41.1111297892197));
#42055=CARTESIAN_POINT('Ctrl Pts',(33.8813839462517,-30.4619629566307,41.2222595784394));
#42056=CARTESIAN_POINT('Ctrl Pts',(31.7284038562778,-29.5872042670172,41.3333893676592));
#42057=CARTESIAN_POINT('Ctrl Pts',(29.825627898444,-30.918441305227,41.4445191568789));
#42058=CARTESIAN_POINT('Ctrl Pts',(29.9119860544063,-33.2405970018638,41.5556489460987));
#42059=CARTESIAN_POINT('Ctrl Pts',(31.9096898625478,-34.4268228681169,41.6667787353183));
#42060=CARTESIAN_POINT('Ctrl Pts',(33.9898334202982,-33.3923239957753,41.7779085245381));
#42061=CARTESIAN_POINT('Ctrl Pts',(34.2490096530018,-31.0834452595862,41.8890383137578));
#42062=CARTESIAN_POINT('Ctrl Pts',(32.4498627695247,-29.6134582253175,42.0001681029775));
#42063=CARTESIAN_POINT('Ctrl Pts',(30.2390335714705,-30.327572605785,42.1112978921973));
#42064=CARTESIAN_POINT('Ctrl Pts',(29.6398080047623,-32.5722924533201,42.222427681417));
#42065=CARTESIAN_POINT('Ctrl Pts',(31.200611501379,-34.2932473343971,42.3335574706367));
#42066=CARTESIAN_POINT('Ctrl Pts',(33.4930031748503,-33.9154517310286,42.4446872598565));
#42067=CARTESIAN_POINT('Ctrl Pts',(34.4190163057797,-31.7846531484843,42.5558170490762));
#42068=CARTESIAN_POINT('Ctrl Pts',(33.1311710515888,-29.8509388446871,42.6669468382959));
#42069=CARTESIAN_POINT('Ctrl Pts',(30.8080907702464,-29.8840214107802,42.7780766275156));
#42070=CARTESIAN_POINT('Ctrl Pts',(29.5758326618125,-31.8536249348858,42.8892064167354));
#42071=CARTESIAN_POINT('Ctrl Pts',(30.5621463276885,-33.9571891796694,43.0003362059551));
#42072=CARTESIAN_POINT('Ctrl Pts',(32.8643680232945,-34.2695551886057,43.1114659951748));
#42073=CARTESIAN_POINT('Ctrl Pts',(34.3755295071108,-32.5048488625596,43.2225957843945));
#42074=CARTESIAN_POINT('Ctrl Pts',(33.7126321326879,-30.2781103518923,43.3337255736142));
#42075=CARTESIAN_POINT('Ctrl Pts',(31.4823524106659,-29.6272265641889,43.444855362834));
#42076=CARTESIAN_POINT('Ctrl Pts',(29.725818144952,-31.1478792982686,43.5559851520537));
#42077=CARTESIAN_POINT('Ctrl Pts',(30.0505904524204,-33.4483836551904,43.6671149412735));
#42078=CARTESIAN_POINT('Ctrl Pts',(32.1594412363987,-34.4233429992207,43.7782447304931));
#42079=CARTESIAN_POINT('Ctrl Pts',(34.1223731303825,-33.1804851097821,43.8893745197129));
#42080=CARTESIAN_POINT('Ctrl Pts',(34.1429321513712,-30.8572600500235,44.0005043089326));
#42081=CARTESIAN_POINT('Ctrl Pts',(32.2023029066813,-29.5798581998207,44.1116340981523));
#42082=CARTESIAN_POINT('Ctrl Pts',(30.0765282356173,-30.5173438798798,44.2227638873721));
#42083=CARTESIAN_POINT('Ctrl Pts',(29.7110940641655,-32.8117403622951,44.3338936765918));
#42084=CARTESIAN_POINT('Ctrl Pts',(31.4404417830221,-34.3632408681166,44.4450234658115));
#42085=CARTESIAN_POINT('Ctrl Pts',(33.6818911139087,-33.7519289597072,44.5561532550313));
#42086=CARTESIAN_POINT('Ctrl Pts',(34.3840919366917,-31.5372706662576,44.667283044251));
#42087=CARTESIAN_POINT('Ctrl Pts',(32.9043976734169,-29.7460972409556,44.7784128334707));
#42088=CARTESIAN_POINT('Ctrl Pts',(30.5970084672143,-30.0176711781749,44.8895426226904));
#42089=CARTESIAN_POINT('Ctrl Pts',(29.573621897008,-32.1034509556668,45.0006724119102));
#42090=CARTESIAN_POINT('Ctrl Pts',(30.770830253685,-34.0945535404118,45.1118022011299));
#42091=CARTESIAN_POINT('Ctrl Pts',(33.0929614323987,-34.168743439459,45.2229319903496));
#42092=CARTESIAN_POINT('Ctrl Pts',(34.4148261608542,-32.2581228617566,45.3340617795694));
#42093=CARTESIAN_POINT('Ctrl Pts',(33.5266681745953,-30.1112710402004,45.445191568789));
#42094=CARTESIAN_POINT('Ctrl Pts',(31.2413200309736,-29.6929634802401,45.5563213580089));
#42095=CARTESIAN_POINT('Ctrl Pts',(29.6503075674633,-31.3860307243948,45.6674511472285));
#42096=CARTESIAN_POINT('Ctrl Pts',(30.2097081368571,-33.6409959913638,45.7785809364483));
#42097=CARTESIAN_POINT('Ctrl Pts',(32.4075644044926,-34.3941395228971,45.8897107256679));
#42098=CARTESIAN_POINT('Ctrl Pts',(34.2324221489883,-32.956192526437,46.0008405148877));
#42099=CARTESIAN_POINT('Ctrl Pts',(34.01419135234,-30.6431484992579,46.1119703041074));
#42100=CARTESIAN_POINT('Ctrl Pts',(31.9525944730258,-29.5718802511161,46.2231000933272));
#42101=CARTESIAN_POINT('Ctrl Pts',(29.9343826179068,-30.7228008652907,46.3342298825469));
#42102=CARTESIAN_POINT('Ctrl Pts',(29.8066013901918,-33.0426002769034,46.4453596717666));
#42103=CARTESIAN_POINT('Ctrl Pts',(31.6861947837558,-34.4082232216233,46.5564894609863));
#42104=CARTESIAN_POINT('Ctrl Pts',(33.8529793081506,-33.5698663900069,46.6676192502061));
#42105=CARTESIAN_POINT('Ctrl Pts',(34.3239372644498,-31.2947848627483,46.7787490394257));
#42106=CARTESIAN_POINT('Ctrl Pts',(32.6680530383748,-29.6651085813628,46.8898788286456));
#42107=CARTESIAN_POINT('Ctrl Pts',(30.4007739163126,-30.172299605471,47.0010086178652));
#42108=CARTESIAN_POINT('Ctrl Pts',(29.5970891631565,-32.3521822100667,47.112138407085));
#42109=CARTESIAN_POINT('Ctrl Pts',(30.9925223493965,-34.2097514752664,47.2232681963047));
#42110=CARTESIAN_POINT('Ctrl Pts',(33.3099881558288,-34.0449801540592,47.3343979855244));
#42111=CARTESIAN_POINT('Ctrl Pts',(34.4285670082764,-32.0086651727433,47.4455277747442));
#42112=CARTESIAN_POINT('Ctrl Pts',(33.324547671462,-29.9644199193026,47.5566575639638));
#42113=CARTESIAN_POINT('Ctrl Pts',(31.008316669847,-29.7831154807695,47.6677873531836));
#42114=CARTESIAN_POINT('Ctrl Pts',(29.59966349763,-31.6306797131245,47.7789171424033));
#42115=CARTESIAN_POINT('Ctrl Pts',(30.3877722618167,-33.8162418669164,47.8900469316231));
#42116=CARTESIAN_POINT('Ctrl Pts',(32.6513743681069,-34.3395991604291,48.0011767208428));
#42117=CARTESIAN_POINT('Ctrl Pts',(34.3188457165666,-32.7217806742136,48.1123065100625));
#42118=CARTESIAN_POINT('Ctrl Pts',(33.8641346120592,-30.4433963423432,48.2234362992822));
#42119=CARTESIAN_POINT('Ctrl Pts',(31.7033877262933,-29.5895987972966,48.334566088502));
#42120=CARTESIAN_POINT('Ctrl Pts',(29.8140971767976,-30.9417742932515,48.4456958777216));
#42121=CARTESIAN_POINT('Ctrl Pts',(29.9253211859677,-33.2624264800428,48.5568256669414));
#42122=CARTESIAN_POINT('Ctrl Pts',(31.9352687467854,-34.427719642744,48.6679554561611));
#42123=CARTESIAN_POINT('Ctrl Pts',(34.0044576485638,-33.3711901159291,48.7790852453809));
#42124=CARTESIAN_POINT('Ctrl Pts',(34.2391886478147,-31.0597622649535,48.8902150346006));
#42125=CARTESIAN_POINT('Ctrl Pts',(32.4246384795753,-29.6088297926389,49.0013448238203));
#42126=CARTESIAN_POINT('Ctrl Pts',(30.2214637798412,-30.34627036294,49.1124746130401));
#42127=CARTESIAN_POINT('Ctrl Pts',(29.6459861413742,-32.5971863631273,49.2236044022597));
#42128=CARTESIAN_POINT('Ctrl Pts',(31.2248764581043,-34.3015638799969,49.3347341914795));
#42129=CARTESIAN_POINT('Ctrl Pts',(33.5131514345126,-33.8995750933143,49.4458639806993));
#42130=CARTESIAN_POINT('Ctrl Pts',(34.4166066274989,-31.7591157812645,49.5569937699189));
#42131=CARTESIAN_POINT('Ctrl Pts',(33.1084096420059,-29.8391110939209,49.6681235591387));
#42132=CARTESIAN_POINT('Ctrl Pts',(30.785808172351,-29.8967284995564,49.7792533483584));
#42133=CARTESIAN_POINT('Ctrl Pts',(29.5744218959985,-31.8792371733684,49.8903831375781));
#42134=CARTESIAN_POINT('Ctrl Pts',(30.5828983961289,-33.9722666764952,50.0015129267979));
#42135=CARTESIAN_POINT('Ctrl Pts',(32.8882909162952,-34.2602991056352,50.1126427160176));
#42136=CARTESIAN_POINT('Ctrl Pts',(34.3807292229819,-32.4797303052207,50.2237725052373));
#42137=CARTESIAN_POINT('Ctrl Pts',(33.6943499627291,-30.2601175319272,50.334902294457));
#42138=CARTESIAN_POINT('Ctrl Pts',(31.4573199910465,-29.6328263251734,50.4460320836768));
#42139=CARTESIAN_POINT('Ctrl Pts',(29.7169448784392,-31.1719467946929,50.5571618728964));
#42140=CARTESIAN_POINT('Ctrl Pts',(30.0659970543811,-33.4688925778434,50.6682916621163));
#42141=CARTESIAN_POINT('Ctrl Pts',(32.1850277527679,-34.4215238032342,50.7794214513359));
#42142=CARTESIAN_POINT('Ctrl Pts',(34.1347230583577,-33.1580027042254,50.8905512405557));
#42143=CARTESIAN_POINT('Ctrl Pts',(34.1307429710586,-30.8346900883493,51.0016810297754));
#42144=CARTESIAN_POINT('Ctrl Pts',(32.1767300235671,-29.5778564663098,51.1128108189952));
#42145=CARTESIAN_POINT('Ctrl Pts',(30.0609756751137,-30.5377423393424,51.2239406082148));
#42146=CARTESIAN_POINT('Ctrl Pts',(29.7197953608552,-32.8358705657033,51.3350703974346));
#42147=CARTESIAN_POINT('Ctrl Pts',(31.465433604746,-34.3690191153306,51.4462001866543));
#42148=CARTESIAN_POINT('Ctrl Pts',(33.7003012160588,-33.7340670608388,51.5573299758741));
#42149=CARTESIAN_POINT('Ctrl Pts',(34.3790715941924,-31.5121156388489,51.6684597650937));
#42150=CARTESIAN_POINT('Ctrl Pts',(32.8805414477757,-29.736670690513,51.7795895543136));
#42151=CARTESIAN_POINT('Ctrl Pts',(30.5761493204034,-30.0326001869503,51.8907193435332));
#42152=CARTESIAN_POINT('Ctrl Pts',(29.5748498880924,-32.1290726458106,52.001849132753));
#42153=CARTESIAN_POINT('Ctrl Pts',(30.7930215501968,-34.1074192405717,52.1129789219727));
#42154=CARTESIAN_POINT('Ctrl Pts',(33.1158067773521,-34.1570785575888,52.2241087111924));
#42155=CARTESIAN_POINT('Ctrl Pts',(34.4174177879696,-32.2326030559352,52.3352385004122));
#42156=CARTESIAN_POINT('Ctrl Pts',(33.506634164426,-30.0952515923113,52.4463682896318));
#42157=CARTESIAN_POINT('Ctrl Pts',(31.2169954713513,-29.7011055471504,52.5574980788516));
#42158=CARTESIAN_POINT('Ctrl Pts',(29.6439536772523,-31.4108821177788,52.6686278680713));
#42159=CARTESIAN_POINT('Ctrl Pts',(30.2271406288629,-33.6598142860527,52.779757657291));
#42160=CARTESIAN_POINT('Ctrl Pts',(32.432827862626,-34.3896998451232,52.8908874465108));
#42161=CARTESIAN_POINT('Ctrl Pts',(34.2423984788832,-32.9325631176565,53.0020172357305));
#42162=CARTESIAN_POINT('Ctrl Pts',(33.9997448841109,-30.6219446492246,53.1131470249503));
#42163=CARTESIAN_POINT('Ctrl Pts',(31.9269572285084,-29.572527465193,53.2242768141699));
#42164=CARTESIAN_POINT('Ctrl Pts',(29.9209962036954,-30.7446672845728,53.3354066033898));
#42165=CARTESIAN_POINT('Ctrl Pts',(29.8177591150446,-33.0657522553465,53.4465363926093));
#42166=CARTESIAN_POINT('Ctrl Pts',(31.7116016656226,-34.4113173899075,53.5576661818292));
#42167=CARTESIAN_POINT('Ctrl Pts',(33.8695486450878,-33.5503777029091,53.6687959710488));
#42168=CARTESIAN_POINT('Ctrl Pts',(34.3161775453905,-31.269941903344,53.7799257602686));
#42169=CARTESIAN_POINT('Ctrl Pts',(32.6437141768078,-29.658850758076,53.8910555494883));
#42170=CARTESIAN_POINT('Ctrl Pts',(30.3808457446301,-30.1879561271019,54.002185338708));
#42171=CARTESIAN_POINT('Ctrl Pts',(29.6023721664291,-32.3803550971457,54.1133151279277));
#42172=CARTESIAN_POINT('Ctrl Pts',(30.5427968191103,-33.6016627022545,54.1874016540742));
#42173=CARTESIAN_POINT('Ctrl Pts',(31.1673980508611,-33.878502477185,54.2244449171475));
#42174=CARTESIAN_POINT('Ctrl Pts',(32.4967348970877,-33.8599788000028,40.9251850276175));
#42175=CARTESIAN_POINT('Ctrl Pts',(33.1151770144774,-33.6948146693493,40.9622282906908));
#42176=CARTESIAN_POINT('Ctrl Pts',(34.163610390172,-32.7015658728382,41.0363148168372));
#42177=CARTESIAN_POINT('Ctrl Pts',(33.7627339873589,-30.5589596554359,41.147444606057));
#42178=CARTESIAN_POINT('Ctrl Pts',(31.7455321364208,-29.7393678459112,41.2585743952766));
#42179=CARTESIAN_POINT('Ctrl Pts',(29.9627552301519,-30.9866500804378,41.3697041844965));
#42180=CARTESIAN_POINT('Ctrl Pts',(30.0436671869608,-33.1623584352134,41.4808339737161));
#42181=CARTESIAN_POINT('Ctrl Pts',(31.9153852944227,-34.2737746643645,41.5919637629359));
#42182=CARTESIAN_POINT('Ctrl Pts',(33.8643440676371,-33.3045167275176,41.7030935521556));
#42183=CARTESIAN_POINT('Ctrl Pts',(34.1071752850569,-31.1412480182893,41.8142233413753));
#42184=CARTESIAN_POINT('Ctrl Pts',(32.4214920591134,-29.7639660916285,41.925353130595));
#42185=CARTESIAN_POINT('Ctrl Pts',(30.3500893688654,-30.4330446663765,42.0364829198148));
#42186=CARTESIAN_POINT('Ctrl Pts',(29.7886541155055,-32.5362006836436,42.1476127090345));
#42187=CARTESIAN_POINT('Ctrl Pts',(31.2510251411306,-34.1486231057811,42.2587424982542));
#42188=CARTESIAN_POINT('Ctrl Pts',(33.3988465484605,-33.7946532785911,42.369872287474));
#42189=CARTESIAN_POINT('Ctrl Pts',(34.2664604248743,-31.7982340526538,42.4810020766937));
#42190=CARTESIAN_POINT('Ctrl Pts',(33.0598334604292,-29.9864699351082,42.5921318659135));
#42191=CARTESIAN_POINT('Ctrl Pts',(30.8832588301186,-30.0174661407245,42.7032616551331));
#42192=CARTESIAN_POINT('Ctrl Pts',(29.7287133938919,-31.8628561157372,42.8143914443529));
#42193=CARTESIAN_POINT('Ctrl Pts',(30.6528249366209,-33.8337585443777,42.9255212335725));
#42194=CARTESIAN_POINT('Ctrl Pts',(32.8098564332299,-34.1264251112126,43.0366510227924));
#42195=CARTESIAN_POINT('Ctrl Pts',(34.2257161322656,-32.473010440153,43.147780812012));
#42196=CARTESIAN_POINT('Ctrl Pts',(33.6046245500003,-30.3867017621533,43.2589106012318));
#42197=CARTESIAN_POINT('Ctrl Pts',(31.5149979880441,-29.776866126694,43.3700403904514));
#42198=CARTESIAN_POINT('Ctrl Pts',(29.8692400042455,-31.2016185078721,43.4811701796713));
#42199=CARTESIAN_POINT('Ctrl Pts',(30.1735304632281,-33.3570409701995,43.5922999688909));
#42200=CARTESIAN_POINT('Ctrl Pts',(32.1493860341195,-34.2705142542887,43.7034297581108));
#42201=CARTESIAN_POINT('Ctrl Pts',(33.9885251270672,-33.1060375149526,43.8145595473303));
#42202=CARTESIAN_POINT('Ctrl Pts',(34.0077875881485,-30.9293272367134,43.9256893365502));
#42203=CARTESIAN_POINT('Ctrl Pts',(32.189544622223,-29.7324850603179,44.0368191257698));
#42204=CARTESIAN_POINT('Ctrl Pts',(30.1978324735058,-30.6108479666214,44.1479489149896));
#42205=CARTESIAN_POINT('Ctrl Pts',(29.8554445013729,-32.7605477491074,44.2590787042093));
#42206=CARTESIAN_POINT('Ctrl Pts',(31.4757304648326,-34.214202479427,44.370208493429));
#42207=CARTESIAN_POINT('Ctrl Pts',(33.5758222214187,-33.641443112591,44.4813382826487));
#42208=CARTESIAN_POINT('Ctrl Pts',(34.233738570039,-31.5664528098261,44.5924680718685));
#42209=CARTESIAN_POINT('Ctrl Pts',(32.8473616032476,-29.8882401938823,44.7035978610882));
#42210=CARTESIAN_POINT('Ctrl Pts',(30.685488486417,-30.1426872514172,44.8147276503079));
#42211=CARTESIAN_POINT('Ctrl Pts',(29.7266420515343,-32.0969267947364,44.9258574395277));
#42212=CARTESIAN_POINT('Ctrl Pts',(30.8483481575467,-33.9624599866405,45.0369872287473));
#42213=CARTESIAN_POINT('Ctrl Pts',(33.0240335406284,-34.0319710807634,45.1481170179672));
#42214=CARTESIAN_POINT('Ctrl Pts',(34.2625345325082,-32.2418442775805,45.2592468071868));
#42215=CARTESIAN_POINT('Ctrl Pts',(33.4303884564018,-30.2303842142479,45.3703765964066));
#42216=CARTESIAN_POINT('Ctrl Pts',(31.2891663769134,-29.8384573273516,45.4815063856263));
#42217=CARTESIAN_POINT('Ctrl Pts',(29.7984915206042,-31.4247508535089,45.592636174846));
#42218=CARTESIAN_POINT('Ctrl Pts',(30.3226133502727,-33.5375061602177,45.7037659640658));
#42219=CARTESIAN_POINT('Ctrl Pts',(32.3818612512709,-34.2431525026552,45.8148957532854));
#42220=CARTESIAN_POINT('Ctrl Pts',(34.0916338762188,-32.8958900006387,45.9260255425053));
#42221=CARTESIAN_POINT('Ctrl Pts',(33.8871658604762,-30.7287186855601,46.0371553317249));
#42222=CARTESIAN_POINT('Ctrl Pts',(31.9555841146872,-29.7250102429852,46.1482851209447));
#42223=CARTESIAN_POINT('Ctrl Pts',(30.0646513054664,-30.8033477547936,46.2594149101644));
#42224=CARTESIAN_POINT('Ctrl Pts',(29.9449286335,-32.9768484242617,46.3705446993841));
#42225=CARTESIAN_POINT('Ctrl Pts',(31.7059849898336,-34.2563480093256,46.4816744886039));
#42226=CARTESIAN_POINT('Ctrl Pts',(33.7361206950114,-33.4708623653299,46.5928042778235));
#42227=CARTESIAN_POINT('Ctrl Pts',(34.1773775675597,-31.3392594354224,46.7039340670433));
#42228=CARTESIAN_POINT('Ctrl Pts',(32.6259221029539,-29.8123591047833,46.815063856263));
#42229=CARTESIAN_POINT('Ctrl Pts',(30.5016295175672,-30.2875639974689,46.9261936454828));
#42230=CARTESIAN_POINT('Ctrl Pts',(29.7486293485517,-32.3299717490758,47.0373234347024));
#42231=CARTESIAN_POINT('Ctrl Pts',(31.0560591846437,-34.0703929343231,47.1484532239223));
#42232=CARTESIAN_POINT('Ctrl Pts',(33.2273734183378,-33.9160129585544,47.2595830131419));
#42233=CARTESIAN_POINT('Ctrl Pts',(34.2754088098797,-32.008118701412,47.3707128023617));
#42234=CARTESIAN_POINT('Ctrl Pts',(33.2410147344006,-30.092794296781,47.4818425915813));
#42235=CARTESIAN_POINT('Ctrl Pts',(31.0708574322425,-29.9229238689514,47.5929723808012));
#42236=CARTESIAN_POINT('Ctrl Pts',(29.7510413319645,-31.6539709913048,47.7041021700207));
#42237=CARTESIAN_POINT('Ctrl Pts',(30.4894478157314,-33.7017001098877,47.8152319592406));
#42238=CARTESIAN_POINT('Ctrl Pts',(32.6102952772846,-34.1920517420706,47.9263617484602));
#42239=CARTESIAN_POINT('Ctrl Pts',(34.1726071194436,-32.6762613917217,48.0374915376801));
#42240=CARTESIAN_POINT('Ctrl Pts',(33.746572486831,-30.5415639494185,48.1486213268997));
#42241=CARTESIAN_POINT('Ctrl Pts',(31.7220936550605,-29.7416113645272,48.2597511161195));
#42242=CARTESIAN_POINT('Ctrl Pts',(29.9519516964098,-31.0085115676156,48.3708809053392));
#42243=CARTESIAN_POINT('Ctrl Pts',(30.0561613350459,-33.1828112317779,48.4820106945589));
#42244=CARTESIAN_POINT('Ctrl Pts',(31.9393510397954,-34.2746148836708,48.5931404837787));
#42245=CARTESIAN_POINT('Ctrl Pts',(33.8780460152136,-33.2847156611994,48.7042702729983));
#42246=CARTESIAN_POINT('Ctrl Pts',(34.0979736440693,-31.1190585977596,48.8154000622182));
#42247=CARTESIAN_POINT('Ctrl Pts',(32.3978585454495,-29.7596295522384,48.9265298514378));
#42248=CARTESIAN_POINT('Ctrl Pts',(30.3336276206307,-30.4505632447029,49.0376596406576));
#42249=CARTESIAN_POINT('Ctrl Pts',(29.7944426263546,-32.5595246526734,49.1487894298773));
#42250=CARTESIAN_POINT('Ctrl Pts',(31.2737598221652,-34.1564151663094,49.259919219097));
#42251=CARTESIAN_POINT('Ctrl Pts',(33.4177241529833,-33.7797779050877,49.3710490083168));
#42252=CARTESIAN_POINT('Ctrl Pts',(34.2642027135694,-31.7743072060174,49.4821787975364));
#42253=CARTESIAN_POINT('Ctrl Pts',(33.0385075049527,-29.9753881044636,49.5933085867562));
#42254=CARTESIAN_POINT('Ctrl Pts',(30.8623814899483,-30.0293718537029,49.7044383759759));
#42255=CARTESIAN_POINT('Ctrl Pts',(29.7273915983841,-31.886853111861,49.8155681651957));
#42256=CARTESIAN_POINT('Ctrl Pts',(30.672268270567,-33.8478851750169,49.9266979544154));
#42257=CARTESIAN_POINT('Ctrl Pts',(32.832270622876,-34.1177527654777,50.0378277436351));
#42258=CARTESIAN_POINT('Ctrl Pts',(34.2305879267278,-32.4494759910455,50.1489575328549));
#42259=CARTESIAN_POINT('Ctrl Pts',(33.5874953497574,-30.369843663973,50.2600873220745));
#42260=CARTESIAN_POINT('Ctrl Pts',(31.4915442443588,-29.7821127373223,50.3712171112943));
#42261=CARTESIAN_POINT('Ctrl Pts',(29.8609263325507,-31.2241681814899,50.482346900514));
#42262=CARTESIAN_POINT('Ctrl Pts',(30.1879654439028,-33.3762564924093,50.5934766897338));
#42263=CARTESIAN_POINT('Ctrl Pts',(32.1733589303015,-34.2688097863616,50.7046064789534));
#42264=CARTESIAN_POINT('Ctrl Pts',(34.0000962036816,-33.0849729680422,50.8157362681732));
#42265=CARTESIAN_POINT('Ctrl Pts',(33.9963671216043,-30.9081806554344,50.9268660573929));
#42266=CARTESIAN_POINT('Ctrl Pts',(32.1655844995112,-29.7306095666419,51.0379958466127));
#42267=CARTESIAN_POINT('Ctrl Pts',(30.1832607392009,-30.6299599920302,51.1491256358323));
#42268=CARTESIAN_POINT('Ctrl Pts',(29.8635970485653,-32.7831561750772,51.2602554250521));
#42269=CARTESIAN_POINT('Ctrl Pts',(31.499146170939,-34.2196163200051,51.3713852142718));
#42270=CARTESIAN_POINT('Ctrl Pts',(33.5930712857764,-33.6247076789349,51.4825150034915));
#42271=CARTESIAN_POINT('Ctrl Pts',(34.2290348367211,-31.5428841906432,51.5936447927113));
#42272=CARTESIAN_POINT('Ctrl Pts',(32.8250098765671,-29.87940813125,51.704774581931));
#42273=CARTESIAN_POINT('Ctrl Pts',(30.6659448270252,-30.1566747584428,51.8159043711507));
#42274=CARTESIAN_POINT('Ctrl Pts',(29.7277925990474,-32.12093264645,51.9270341603704));
#42275=CARTESIAN_POINT('Ctrl Pts',(30.8691399542786,-33.9745143081351,52.0381639495902));
#42276=CARTESIAN_POINT('Ctrl Pts',(33.0454381380698,-34.0210418476463,52.1492937388099));
#42277=CARTESIAN_POINT('Ctrl Pts',(34.2649627179979,-32.2179338848285,52.2604235280296));
#42278=CARTESIAN_POINT('Ctrl Pts',(33.4116178961986,-30.2153750369296,52.3715533172493));
#42279=CARTESIAN_POINT('Ctrl Pts',(31.2663758518537,-29.8460859127335,52.4826831064691));
#42280=CARTESIAN_POINT('Ctrl Pts',(29.7925383401015,-31.4480349874244,52.5938128956888));
#42281=CARTESIAN_POINT('Ctrl Pts',(30.3389464577195,-33.5551376743476,52.7049426849085));
#42282=CARTESIAN_POINT('Ctrl Pts',(32.4055314629674,-34.2389928142936,52.8160724741283));
#42283=CARTESIAN_POINT('Ctrl Pts',(34.1009810463219,-32.8737507865556,52.927202263348));
#42284=CARTESIAN_POINT('Ctrl Pts',(33.8736304624541,-30.7088520617425,53.0383320525678));
#42285=CARTESIAN_POINT('Ctrl Pts',(31.9315636895405,-29.7256166403411,53.1494618417874));
#42286=CARTESIAN_POINT('Ctrl Pts',(30.0521091088848,-30.8238351627611,53.2605916310072));
#42287=CARTESIAN_POINT('Ctrl Pts',(29.9553826935864,-32.9985403172736,53.3717214202268));
#42288=CARTESIAN_POINT('Ctrl Pts',(31.7297895802091,-34.259247043097,53.4828512094467));
#42289=CARTESIAN_POINT('Ctrl Pts',(33.7516450824844,-33.4526027372595,53.5939809986663));
#42290=CARTESIAN_POINT('Ctrl Pts',(34.1701072171639,-31.3159832035954,53.7051107878861));
#42291=CARTESIAN_POINT('Ctrl Pts',(32.6031181779054,-29.8064959327199,53.8162405771057));
#42292=CARTESIAN_POINT('Ctrl Pts',(30.4829581211195,-30.302233136566,53.9273703663256));
#42293=CARTESIAN_POINT('Ctrl Pts',(29.7535791778743,-32.3563679058385,54.0385001555452));
#42294=CARTESIAN_POINT('Ctrl Pts',(30.634695709741,-33.5006534350279,54.1125866816917));
#42295=CARTESIAN_POINT('Ctrl Pts',(31.2199063053491,-33.7600342388744,54.149629944765));
#42296=CARTESIAN_POINT('Ctrl Pts',(32.4632995769868,-33.7347832743338,40.850370055235));
#42297=CARTESIAN_POINT('Ctrl Pts',(33.0401142382021,-33.5807363726288,40.8874133183083));
#42298=CARTESIAN_POINT('Ctrl Pts',(34.017977364602,-32.6543433409248,40.9614998444548));
#42299=CARTESIAN_POINT('Ctrl Pts',(33.6440840284661,-30.6559563542411,41.0726296336744));
#42300=CARTESIAN_POINT('Ctrl Pts',(31.7626604165639,-29.8915314248051,41.1837594228942));
#42301=CARTESIAN_POINT('Ctrl Pts',(30.0998825618597,-31.0548588556486,41.2948892121139));
#42302=CARTESIAN_POINT('Ctrl Pts',(30.1753483195154,-33.084119868563,41.4060190013337));
#42303=CARTESIAN_POINT('Ctrl Pts',(31.9210807262976,-34.1207264606122,41.5171487905533));
#42304=CARTESIAN_POINT('Ctrl Pts',(33.7388547149761,-33.2167094592598,41.6282785797731));
#42305=CARTESIAN_POINT('Ctrl Pts',(33.965340917112,-31.1990507769925,41.7394083689929));
#42306=CARTESIAN_POINT('Ctrl Pts',(32.3931213487021,-29.9144739579396,41.8505381582125));
#42307=CARTESIAN_POINT('Ctrl Pts',(30.4611451662601,-30.5385167269679,41.9616679474324));
#42308=CARTESIAN_POINT('Ctrl Pts',(29.9375002262487,-32.5001089139672,42.0727977366519));
#42309=CARTESIAN_POINT('Ctrl Pts',(31.3014387808822,-34.0039988771649,42.1839275258718));
#42310=CARTESIAN_POINT('Ctrl Pts',(33.3046899220708,-33.6738548261537,42.2950573150914));
#42311=CARTESIAN_POINT('Ctrl Pts',(34.1139045439687,-31.8118149568232,42.4061871043112));
#42312=CARTESIAN_POINT('Ctrl Pts',(32.9884958692697,-30.1220010255292,42.5173168935309));
#42313=CARTESIAN_POINT('Ctrl Pts',(30.9584268899907,-30.1509108706688,42.6284466827506));
#42314=CARTESIAN_POINT('Ctrl Pts',(29.8815941259713,-31.8720872965886,42.7395764719704));
#42315=CARTESIAN_POINT('Ctrl Pts',(30.7435035455532,-33.7103279090861,42.8507062611901));
#42316=CARTESIAN_POINT('Ctrl Pts',(32.7553448431653,-33.9832950338195,42.9618360504099));
#42317=CARTESIAN_POINT('Ctrl Pts',(34.0759027574205,-32.4411720177464,43.0729658396295));
#42318=CARTESIAN_POINT('Ctrl Pts',(33.4966169673125,-30.4952931724144,43.1840956288493));
#42319=CARTESIAN_POINT('Ctrl Pts',(31.5476435654224,-29.926505689199,43.295225418069));
#42320=CARTESIAN_POINT('Ctrl Pts',(30.012661863539,-31.2553577174755,43.4063552072887));
#42321=CARTESIAN_POINT('Ctrl Pts',(30.2964704740359,-33.2656982852085,43.5174849965084));
#42322=CARTESIAN_POINT('Ctrl Pts',(32.1393308318402,-34.1176855093567,43.6286147857282));
#42323=CARTESIAN_POINT('Ctrl Pts',(33.8546771237519,-33.0315899201231,43.7397445749479));
#42324=CARTESIAN_POINT('Ctrl Pts',(33.8726430249258,-31.0013944234033,43.8508743641676));
#42325=CARTESIAN_POINT('Ctrl Pts',(32.1767863377647,-29.8851119208151,43.9620041533874));
#42326=CARTESIAN_POINT('Ctrl Pts',(30.3191367113942,-30.7043520533629,44.0731339426071));
#42327=CARTESIAN_POINT('Ctrl Pts',(29.9997949385803,-32.7093551359197,44.1842637318268));
#42328=CARTESIAN_POINT('Ctrl Pts',(31.511019146643,-34.0651640907373,44.2953935210465));
#42329=CARTESIAN_POINT('Ctrl Pts',(33.4697533289286,-33.5309572654748,44.4065233102663));
#42330=CARTESIAN_POINT('Ctrl Pts',(34.0833852033863,-31.5956349533947,44.5176530994859));
#42331=CARTESIAN_POINT('Ctrl Pts',(32.7903255330784,-30.030383146809,44.6287828887058));
#42332=CARTESIAN_POINT('Ctrl Pts',(30.7739685056197,-30.2677033246597,44.7399126779254));
#42333=CARTESIAN_POINT('Ctrl Pts',(29.8796622060605,-32.0904026338059,44.8510424671452));
#42334=CARTESIAN_POINT('Ctrl Pts',(30.9258660614085,-33.8303664328691,44.9621722563649));
#42335=CARTESIAN_POINT('Ctrl Pts',(32.9551056488581,-33.8951987220677,45.0733020455846));
#42336=CARTESIAN_POINT('Ctrl Pts',(34.1102429041622,-32.2255656934043,45.1844318348044));
#42337=CARTESIAN_POINT('Ctrl Pts',(33.3341087382084,-30.3494973882954,45.295561624024));
#42338=CARTESIAN_POINT('Ctrl Pts',(31.3370127228531,-29.983951174463,45.4066914132439));
#42339=CARTESIAN_POINT('Ctrl Pts',(29.946675473745,-31.463470982623,45.5178212024635));
#42340=CARTESIAN_POINT('Ctrl Pts',(30.4355185636883,-33.4340163290715,45.6289509916833));
#42341=CARTESIAN_POINT('Ctrl Pts',(32.3561580980493,-34.0921654824133,45.740080780903));
#42342=CARTESIAN_POINT('Ctrl Pts',(33.9508456034494,-32.8355874748403,45.8512105701227));
#42343=CARTESIAN_POINT('Ctrl Pts',(33.7601403686122,-30.8142888718623,45.9623403593424));
#42344=CARTESIAN_POINT('Ctrl Pts',(31.9585737563486,-29.8781402348542,46.0734701485622));
#42345=CARTESIAN_POINT('Ctrl Pts',(30.1949199930259,-30.8838946442965,46.1845999377819));
#42346=CARTESIAN_POINT('Ctrl Pts',(30.0832558768083,-32.9110965716201,46.2957297270016));
#42347=CARTESIAN_POINT('Ctrl Pts',(31.7257751959113,-34.1044727970279,46.4068595162214));
#42348=CARTESIAN_POINT('Ctrl Pts',(33.6192620818722,-33.3718583406529,46.5179893054411));
#42349=CARTESIAN_POINT('Ctrl Pts',(34.0308178706696,-31.3837340080966,46.6291190946608));
#42350=CARTESIAN_POINT('Ctrl Pts',(32.583791167533,-29.9596096282039,46.7402488838806));
#42351=CARTESIAN_POINT('Ctrl Pts',(30.6024851188217,-30.4028283894668,46.8513786731002));
#42352=CARTESIAN_POINT('Ctrl Pts',(29.9001695339471,-32.3077612880849,46.96250846232));
#42353=CARTESIAN_POINT('Ctrl Pts',(31.1195960198908,-33.9310343933798,47.0736382515397));
#42354=CARTESIAN_POINT('Ctrl Pts',(33.1447586808469,-33.7870457630496,47.1847680407594));
#42355=CARTESIAN_POINT('Ctrl Pts',(34.1222506114829,-32.0075722300807,47.2958978299792));
#42356=CARTESIAN_POINT('Ctrl Pts',(33.1574817973392,-30.2211686742594,47.4070276191988));
#42357=CARTESIAN_POINT('Ctrl Pts',(31.1333981946381,-30.0627322571335,47.5181574084187));
#42358=CARTESIAN_POINT('Ctrl Pts',(29.902419166299,-31.6772622694852,47.6292871976383));
#42359=CARTESIAN_POINT('Ctrl Pts',(30.5911233696461,-33.5871583528591,47.740416986858));
#42360=CARTESIAN_POINT('Ctrl Pts',(32.5692161864623,-34.044504323712,47.8515467760779));
#42361=CARTESIAN_POINT('Ctrl Pts',(34.0263685223206,-32.6307421092299,47.9626765652975));
#42362=CARTESIAN_POINT('Ctrl Pts',(33.6290103616028,-30.6397315564939,48.0738063545173));
#42363=CARTESIAN_POINT('Ctrl Pts',(31.7407995838277,-29.8936239317577,48.1849361437369));
#42364=CARTESIAN_POINT('Ctrl Pts',(30.0898062160221,-31.0752488419796,48.2960659329567));
#42365=CARTESIAN_POINT('Ctrl Pts',(30.187001484124,-33.1031959835131,48.4071957221764));
#42366=CARTESIAN_POINT('Ctrl Pts',(31.9434333328055,-34.1215101245977,48.5183255113962));
#42367=CARTESIAN_POINT('Ctrl Pts',(33.7516343818633,-33.1982412064697,48.6294553006159));
#42368=CARTESIAN_POINT('Ctrl Pts',(33.9567586403238,-31.1783549305655,48.7405850898356));
#42369=CARTESIAN_POINT('Ctrl Pts',(32.3710786113237,-29.910429311838,48.8517148790553));
#42370=CARTESIAN_POINT('Ctrl Pts',(30.4457914614202,-30.5548561264658,48.9628446682751));
#42371=CARTESIAN_POINT('Ctrl Pts',(29.9428991113351,-32.5218629422194,49.0739744574948));
#42372=CARTESIAN_POINT('Ctrl Pts',(31.3226431862259,-34.0112664526218,49.1851042467145));
#42373=CARTESIAN_POINT('Ctrl Pts',(33.3222968714541,-33.6599807168611,49.2962340359343));
#42374=CARTESIAN_POINT('Ctrl Pts',(34.1117987996398,-31.7894986307704,49.4073638251539));
#42375=CARTESIAN_POINT('Ctrl Pts',(32.9686053678996,-30.1116651150064,49.5184936143737));
#42376=CARTESIAN_POINT('Ctrl Pts',(30.9389548075454,-30.1620152078494,49.6296234035934));
#42377=CARTESIAN_POINT('Ctrl Pts',(29.8803613007697,-31.8944690503536,49.7407531928132));
#42378=CARTESIAN_POINT('Ctrl Pts',(30.7616381450051,-33.7235036735387,49.8518829820329));
#42379=CARTESIAN_POINT('Ctrl Pts',(32.7762503294566,-33.9752064253202,49.9630127712526));
#42380=CARTESIAN_POINT('Ctrl Pts',(34.0804466304738,-32.4192216768704,50.0741425604724));
#42381=CARTESIAN_POINT('Ctrl Pts',(33.4806407367856,-30.4795697960187,50.185272349692));
#42382=CARTESIAN_POINT('Ctrl Pts',(31.5257684976712,-29.9313991494713,50.2964021389118));
#42383=CARTESIAN_POINT('Ctrl Pts',(30.0049077866622,-31.2763895682868,50.4075319281314));
#42384=CARTESIAN_POINT('Ctrl Pts',(30.3099338334245,-33.2836204069753,50.5186617173513));
#42385=CARTESIAN_POINT('Ctrl Pts',(32.1616901078351,-34.1160957694889,50.6297915065709));
#42386=CARTESIAN_POINT('Ctrl Pts',(33.8654693490056,-33.0119432318589,50.7409212957907));
#42387=CARTESIAN_POINT('Ctrl Pts',(33.8619912721499,-30.9816712225195,50.8520510850104));
#42388=CARTESIAN_POINT('Ctrl Pts',(32.1544389754553,-29.883362666974,50.9631808742301));
#42389=CARTESIAN_POINT('Ctrl Pts',(30.3055458032881,-30.722177644718,51.0743106634499));
#42390=CARTESIAN_POINT('Ctrl Pts',(30.0073987362756,-32.730441784451,51.1854404526696));
#42391=CARTESIAN_POINT('Ctrl Pts',(31.5328587371319,-34.0702135246797,51.2965702418894));
#42392=CARTESIAN_POINT('Ctrl Pts',(33.4858413554941,-33.515348297031,51.4077000311091));
#42393=CARTESIAN_POINT('Ctrl Pts',(34.0789980792498,-31.5736527424373,51.5188298203288));
#42394=CARTESIAN_POINT('Ctrl Pts',(32.7694783053585,-30.022145571987,51.6299596095485));
#42395=CARTESIAN_POINT('Ctrl Pts',(30.7557403336469,-30.2807493299354,51.7410893987682));
#42396=CARTESIAN_POINT('Ctrl Pts',(29.8807353100023,-32.1127926470893,51.8522191879879));
#42397=CARTESIAN_POINT('Ctrl Pts',(30.9452583583604,-33.8416093756986,51.9633489772077));
#42398=CARTESIAN_POINT('Ctrl Pts',(32.9750694987876,-33.8850051377039,52.0744787664274));
#42399=CARTESIAN_POINT('Ctrl Pts',(34.1125076480262,-32.2032647137217,52.1856085556471));
#42400=CARTESIAN_POINT('Ctrl Pts',(33.3166016279713,-30.3354984815481,52.2967383448669));
#42401=CARTESIAN_POINT('Ctrl Pts',(31.3157562323562,-29.9910662783164,52.4078681340865));
#42402=CARTESIAN_POINT('Ctrl Pts',(29.9411230029507,-31.4851878570702,52.5189979233064));
#42403=CARTESIAN_POINT('Ctrl Pts',(30.4507522865762,-33.4504610626425,52.630127712526));
#42404=CARTESIAN_POINT('Ctrl Pts',(32.3782350633087,-34.0882857834639,52.7412575017459));
#42405=CARTESIAN_POINT('Ctrl Pts',(33.9595636137607,-32.8149384554547,52.8523872909654));
#42406=CARTESIAN_POINT('Ctrl Pts',(33.7475160407973,-30.7957594742605,52.9635170801853));
#42407=CARTESIAN_POINT('Ctrl Pts',(31.9361701505726,-29.8787058154891,53.0746468694049));
#42408=CARTESIAN_POINT('Ctrl Pts',(30.1832220140741,-30.9030030409494,53.1857766586248));
#42409=CARTESIAN_POINT('Ctrl Pts',(30.0930062721282,-32.9313283792007,53.2969064478443));
#42410=CARTESIAN_POINT('Ctrl Pts',(31.7479774947954,-34.1071766962865,53.4080362370641));
#42411=CARTESIAN_POINT('Ctrl Pts',(33.6337415198811,-33.3548277716098,53.5191660262838));
#42412=CARTESIAN_POINT('Ctrl Pts',(34.0240368889374,-31.3620245038469,53.6302958155036));
#42413=CARTESIAN_POINT('Ctrl Pts',(32.562522179003,-29.9541411073636,53.7414256047233));
#42414=CARTESIAN_POINT('Ctrl Pts',(30.585070497609,-30.4165101460301,53.8525553939431));
#42415=CARTESIAN_POINT('Ctrl Pts',(29.9047861893194,-32.3323807145313,53.9636851831628));
#42416=CARTESIAN_POINT('Ctrl Pts',(30.7265946003719,-33.3996441678013,54.0377717093093));
#42417=CARTESIAN_POINT('Ctrl Pts',(31.2724145598371,-33.6415660005639,54.0748149723825));
#42418=CARTESIAN_POINT('Ctrl Pts',(32.4298642568859,-33.6095877486649,40.7755550828525));
#42419=CARTESIAN_POINT('Ctrl Pts',(32.9650514619268,-33.4666580759082,40.8125983459258));
#42420=CARTESIAN_POINT('Ctrl Pts',(33.8723443390321,-32.6071208090114,40.8866848720722));
#42421=CARTESIAN_POINT('Ctrl Pts',(33.5254340695732,-30.7529530530463,40.997814661292));
#42422=CARTESIAN_POINT('Ctrl Pts',(31.779788696707,-30.0436950036991,41.1089444505117));
#42423=CARTESIAN_POINT('Ctrl Pts',(30.2370098935675,-31.1230676308593,41.2200742397315));
#42424=CARTESIAN_POINT('Ctrl Pts',(30.30702945207,-33.0058813019126,41.3312040289512));
#42425=CARTESIAN_POINT('Ctrl Pts',(31.9267761581724,-33.9676782568598,41.4423338181709));
#42426=CARTESIAN_POINT('Ctrl Pts',(33.613365362315,-33.1289021910022,41.5534636073906));
#42427=CARTESIAN_POINT('Ctrl Pts',(33.8235065491671,-31.2568535356956,41.6645933966104));
#42428=CARTESIAN_POINT('Ctrl Pts',(32.3647506382908,-30.0649818242506,41.77572318583));
#42429=CARTESIAN_POINT('Ctrl Pts',(30.5722009636549,-30.6439887875594,41.8868529750498));
#42430=CARTESIAN_POINT('Ctrl Pts',(30.0863463369919,-32.4640171442907,41.9979827642695));
#42431=CARTESIAN_POINT('Ctrl Pts',(31.3518524206338,-33.8593746485488,42.1091125534892));
#42432=CARTESIAN_POINT('Ctrl Pts',(33.210533295681,-33.5530563737163,42.220242342709));
#42433=CARTESIAN_POINT('Ctrl Pts',(33.9613486630632,-31.8253958609927,42.3313721319287));
#42434=CARTESIAN_POINT('Ctrl Pts',(32.9171582781102,-30.2575321159502,42.4425019211484));
#42435=CARTESIAN_POINT('Ctrl Pts',(31.0335949498628,-30.2843556006131,42.5536317103682));
#42436=CARTESIAN_POINT('Ctrl Pts',(30.0344748580507,-31.8813184774399,42.6647614995879));
#42437=CARTESIAN_POINT('Ctrl Pts',(30.8341821544855,-33.5868972737945,42.7758912888076));
#42438=CARTESIAN_POINT('Ctrl Pts',(32.7008332531007,-33.8401649564264,42.8870210780274));
#42439=CARTESIAN_POINT('Ctrl Pts',(33.9260893825753,-32.4093335953397,42.998150867247));
#42440=CARTESIAN_POINT('Ctrl Pts',(33.3886093846249,-30.6038845826755,43.1092806564668));
#42441=CARTESIAN_POINT('Ctrl Pts',(31.5802891428005,-30.076145251704,43.2204104456865));
#42442=CARTESIAN_POINT('Ctrl Pts',(30.1560837228325,-31.309096927079,43.3315402349062));
#42443=CARTESIAN_POINT('Ctrl Pts',(30.4194104848436,-33.1743556002176,43.442670024126));
#42444=CARTESIAN_POINT('Ctrl Pts',(32.1292756295609,-33.9648567644247,43.5537998133457));
#42445=CARTESIAN_POINT('Ctrl Pts',(33.7208291204366,-32.9571423252936,43.6649296025654));
#42446=CARTESIAN_POINT('Ctrl Pts',(33.7374984617031,-31.0734616100933,43.7760593917851));
#42447=CARTESIAN_POINT('Ctrl Pts',(32.1640280533063,-30.0377387813122,43.8871891810049));
#42448=CARTESIAN_POINT('Ctrl Pts',(30.4404409492826,-30.7978561401045,43.9983189702246));
#42449=CARTESIAN_POINT('Ctrl Pts',(30.1441453757877,-32.658162522732,44.1094487594443));
#42450=CARTESIAN_POINT('Ctrl Pts',(31.5463078284535,-33.9161257020476,44.2205785486641));
#42451=CARTESIAN_POINT('Ctrl Pts',(33.3636844364385,-33.4204714183585,44.3317083378837));
#42452=CARTESIAN_POINT('Ctrl Pts',(33.9330318367336,-31.6248170969632,44.4428381271036));
#42453=CARTESIAN_POINT('Ctrl Pts',(32.7332894629091,-30.1725260997357,44.5539679163232));
#42454=CARTESIAN_POINT('Ctrl Pts',(30.8624485248225,-30.3927193979021,44.665097705543));
#42455=CARTESIAN_POINT('Ctrl Pts',(30.0326823605866,-32.0838784728755,44.7762274947626));
#42456=CARTESIAN_POINT('Ctrl Pts',(31.0033839652703,-33.6982728790978,44.8873572839824));
#42457=CARTESIAN_POINT('Ctrl Pts',(32.8861777570878,-33.758426363372,44.9984870732021));
#42458=CARTESIAN_POINT('Ctrl Pts',(33.9579512758162,-32.2092871092282,45.1096168624219));
#42459=CARTESIAN_POINT('Ctrl Pts',(33.2378290200149,-30.4686105623428,45.2207466516415));
#42460=CARTESIAN_POINT('Ctrl Pts',(31.3848590687928,-30.1294450215744,45.3318764408614));
#42461=CARTESIAN_POINT('Ctrl Pts',(30.0948594268859,-31.5021911117371,45.443006230081));
#42462=CARTESIAN_POINT('Ctrl Pts',(30.5484237771038,-33.3305264979253,45.5541360193008));
#42463=CARTESIAN_POINT('Ctrl Pts',(32.3304549448276,-33.9411784621714,45.6652658085204));
#42464=CARTESIAN_POINT('Ctrl Pts',(33.81005733068,-32.775284949042,45.7763955977403));
#42465=CARTESIAN_POINT('Ctrl Pts',(33.6331148767482,-30.8998590581646,45.8875253869598));
#42466=CARTESIAN_POINT('Ctrl Pts',(31.96156339801,-30.0312702267232,45.9986551761798));
#42467=CARTESIAN_POINT('Ctrl Pts',(30.3251886805853,-30.9644415337994,46.1097849653993));
#42468=CARTESIAN_POINT('Ctrl Pts',(30.2215831201166,-32.8453447189785,46.2209147546191));
#42469=CARTESIAN_POINT('Ctrl Pts',(31.7455654019891,-33.9525975847302,46.3320445438389));
#42470=CARTESIAN_POINT('Ctrl Pts',(33.5024034687329,-33.2728543159759,46.4431743330586));
#42471=CARTESIAN_POINT('Ctrl Pts',(33.8842581737795,-31.4282085807707,46.5543041222783));
#42472=CARTESIAN_POINT('Ctrl Pts',(32.5416602321121,-30.1068601516244,46.665433911498));
#42473=CARTESIAN_POINT('Ctrl Pts',(30.7033407200763,-30.5180927814648,46.7765637007178));
#42474=CARTESIAN_POINT('Ctrl Pts',(30.0517097193423,-32.2855508270939,46.8876934899375));
#42475=CARTESIAN_POINT('Ctrl Pts',(31.183132855138,-33.7916758524365,46.9988232791572));
#42476=CARTESIAN_POINT('Ctrl Pts',(33.062143943356,-33.6580785675447,47.109953068377));
#42477=CARTESIAN_POINT('Ctrl Pts',(33.9690924130861,-32.0070257587494,47.2210828575967));
#42478=CARTESIAN_POINT('Ctrl Pts',(33.0739488602778,-30.3495430517377,47.3322126468164));
#42479=CARTESIAN_POINT('Ctrl Pts',(31.1959389570337,-30.2025406453155,47.4433424360361));
#42480=CARTESIAN_POINT('Ctrl Pts',(30.0537970006334,-31.7005535476654,47.5544722252559));
#42481=CARTESIAN_POINT('Ctrl Pts',(30.6927989235608,-33.4726165958304,47.6656020144756));
#42482=CARTESIAN_POINT('Ctrl Pts',(32.52813709564,-33.8969569053535,47.7767318036953));
#42483=CARTESIAN_POINT('Ctrl Pts',(33.8801299251977,-32.5852228267379,47.887861592915));
#42484=CARTESIAN_POINT('Ctrl Pts',(33.5114482363745,-30.7378991635692,47.9989913821347));
#42485=CARTESIAN_POINT('Ctrl Pts',(31.759505512595,-30.0456364989882,48.1101211713545));
#42486=CARTESIAN_POINT('Ctrl Pts',(30.2276607356344,-31.1419861163437,48.2212509605742));
#42487=CARTESIAN_POINT('Ctrl Pts',(30.3178416332022,-33.0235807352482,48.3323807497939));
#42488=CARTESIAN_POINT('Ctrl Pts',(31.9475156258155,-33.9684053655245,48.4435105390137));
#42489=CARTESIAN_POINT('Ctrl Pts',(33.6252227485131,-33.11176675174,48.5546403282334));
#42490=CARTESIAN_POINT('Ctrl Pts',(33.8155436365783,-31.2376512633715,48.6657701174532));
#42491=CARTESIAN_POINT('Ctrl Pts',(32.3442986771979,-30.0612290714376,48.7768999066728));
#42492=CARTESIAN_POINT('Ctrl Pts',(30.5579553022097,-30.6591490082288,48.8880296958926));
#42493=CARTESIAN_POINT('Ctrl Pts',(30.0913555963156,-32.4842012317655,48.9991594851123));
#42494=CARTESIAN_POINT('Ctrl Pts',(31.3715265502868,-33.8661177389341,49.110289274332));
#42495=CARTESIAN_POINT('Ctrl Pts',(33.2268695899248,-33.5401835286345,49.2214190635518));
#42496=CARTESIAN_POINT('Ctrl Pts',(33.9593948857103,-31.8046900555234,49.3325488527714));
#42497=CARTESIAN_POINT('Ctrl Pts',(32.8987032308465,-30.2479421255491,49.4436786419912));
#42498=CARTESIAN_POINT('Ctrl Pts',(31.0155281251426,-30.2946585619959,49.554808431211));
#42499=CARTESIAN_POINT('Ctrl Pts',(30.0333310031554,-31.9020849888462,49.6659382204306));
#42500=CARTESIAN_POINT('Ctrl Pts',(30.8510080194431,-33.5991221720603,49.7770680096504));
#42501=CARTESIAN_POINT('Ctrl Pts',(32.7202300360374,-33.8326600851628,49.8881977988701));
#42502=CARTESIAN_POINT('Ctrl Pts',(33.9303053342196,-32.3889673626951,49.9993275880899));
#42503=CARTESIAN_POINT('Ctrl Pts',(33.373786123814,-30.5892959280646,50.1104573773095));
#42504=CARTESIAN_POINT('Ctrl Pts',(31.5599927509835,-30.0806855616201,50.2215871665293));
#42505=CARTESIAN_POINT('Ctrl Pts',(30.1488892407737,-31.3286109550838,50.332716955749));
#42506=CARTESIAN_POINT('Ctrl Pts',(30.4319022229462,-33.1909843215413,50.4438467449688));
#42507=CARTESIAN_POINT('Ctrl Pts',(32.1500212853687,-33.9633817526162,50.5549765341885));
#42508=CARTESIAN_POINT('Ctrl Pts',(33.7308424943297,-32.9389134956757,50.6661063234082));
#42509=CARTESIAN_POINT('Ctrl Pts',(33.7276154226956,-31.0551617896046,50.7772361126279));
#42510=CARTESIAN_POINT('Ctrl Pts',(32.1432934513994,-30.0361157673061,50.8883659018476));
#42511=CARTESIAN_POINT('Ctrl Pts',(30.4278308673753,-30.8143952974057,50.9994956910674));
#42512=CARTESIAN_POINT('Ctrl Pts',(30.1512004239858,-32.677727393825,51.1106254802871));
#42513=CARTESIAN_POINT('Ctrl Pts',(31.5665713033249,-33.9208107293542,51.2217552695069));
#42514=CARTESIAN_POINT('Ctrl Pts',(33.3786114252118,-33.4059889151271,51.3328850587265));
#42515=CARTESIAN_POINT('Ctrl Pts',(33.9289613217785,-31.6044212942316,51.4440148479463));
#42516=CARTESIAN_POINT('Ctrl Pts',(32.7139467341499,-30.164883012724,51.5551446371661));
#42517=CARTESIAN_POINT('Ctrl Pts',(30.8455358402687,-30.404823901428,51.6662744263857));
#42518=CARTESIAN_POINT('Ctrl Pts',(30.0336780209573,-32.1046526477287,51.7774042156055));
#42519=CARTESIAN_POINT('Ctrl Pts',(31.0213767624421,-33.7087044432619,51.8885340048252));
#42520=CARTESIAN_POINT('Ctrl Pts',(32.9047008595054,-33.7489684277615,51.9996637940449));
#42521=CARTESIAN_POINT('Ctrl Pts',(33.9600525780544,-32.1885955426149,52.1107935832646));
#42522=CARTESIAN_POINT('Ctrl Pts',(33.2215853597439,-30.4556219261665,52.2219233724845));
#42523=CARTESIAN_POINT('Ctrl Pts',(31.3651366128586,-30.1360466438995,52.333053161704));
#42524=CARTESIAN_POINT('Ctrl Pts',(30.0897076657999,-31.5223407267159,52.4441829509239));
#42525=CARTESIAN_POINT('Ctrl Pts',(30.5625581154328,-33.3457844509375,52.5553127401435));
#42526=CARTESIAN_POINT('Ctrl Pts',(32.3509386636501,-33.9375787526343,52.6664425293633));
#42527=CARTESIAN_POINT('Ctrl Pts',(33.8181461811994,-32.7561261243537,52.777572318583));
#42528=CARTESIAN_POINT('Ctrl Pts',(33.6214016191404,-30.8826668867785,52.8887021078028));
#42529=CARTESIAN_POINT('Ctrl Pts',(31.9407766116048,-30.0317949906372,52.9998318970224));
#42530=CARTESIAN_POINT('Ctrl Pts',(30.3143349192635,-30.9821709191377,53.1109616862423));
#42531=CARTESIAN_POINT('Ctrl Pts',(30.23062985067,-32.8641164411277,53.2220914754618));
#42532=CARTESIAN_POINT('Ctrl Pts',(31.7661654093819,-33.955106349476,53.3332212646817));
#42533=CARTESIAN_POINT('Ctrl Pts',(33.5158379572776,-33.2570528059602,53.4443510539013));
#42534=CARTESIAN_POINT('Ctrl Pts',(33.8779665607108,-31.4080658040983,53.5554808431211));
#42535=CARTESIAN_POINT('Ctrl Pts',(32.5219261801006,-30.1017862820074,53.6666106323408));
#42536=CARTESIAN_POINT('Ctrl Pts',(30.6871828740984,-30.5307871554942,53.7777404215606));
#42537=CARTESIAN_POINT('Ctrl Pts',(30.0559932007645,-32.3083935232241,53.8888702107803));
#42538=CARTESIAN_POINT('Ctrl Pts',(30.8184934910026,-33.2986349005747,53.9629567369268));
#42539=CARTESIAN_POINT('Ctrl Pts',(31.3249228143251,-33.5230977622534,54.));
#42540=CARTESIAN_POINT('Ctrl Pts',(33.6638410100825,-31.9990545799874,41.6214803633902));
#42541=CARTESIAN_POINT('Ctrl Pts',(33.6649611950912,-31.7834963339009,41.6358513744636));
#42542=CARTESIAN_POINT('Ctrl Pts',(33.6260908134042,-31.5683254077851,41.650222385537));
#42543=CARTESIAN_POINT('Ctrl Pts',(33.5453570328791,-31.3702163596725,41.6645933966103));
#42544=CARTESIAN_POINT('Ctrl Pts',(33.337254578875,-30.8595629652139,41.7016366596836));
#42545=CARTESIAN_POINT('Ctrl Pts',(32.8510026085829,-30.4622723947323,41.7386799227568));
#42546=CARTESIAN_POINT('Ctrl Pts',(32.3091183443309,-30.3601282700429,41.77572318583));
#42547=CARTESIAN_POINT('Ctrl Pts',(31.7672340800789,-30.2579841453535,41.8127664489033));
#42548=CARTESIAN_POINT('Ctrl Pts',(31.1697175218669,-30.4509864664565,41.8498097119765));
#42549=CARTESIAN_POINT('Ctrl Pts',(30.7899834716504,-30.8508256864632,41.8868529750498));
#42550=CARTESIAN_POINT('Ctrl Pts',(30.4102494214339,-31.2506649064699,41.923896238123));
#42551=CARTESIAN_POINT('Ctrl Pts',(30.2482978792129,-31.8573410253802,41.9609395011963));
#42552=CARTESIAN_POINT('Ctrl Pts',(30.3782397887094,-32.3932386688785,41.9979827642695));
#42553=CARTESIAN_POINT('Ctrl Pts',(30.5081816982059,-32.9291363123767,42.0350260273428));
#42554=CARTESIAN_POINT('Ctrl Pts',(30.9300170594198,-33.3942554804628,42.072069290416));
#42555=CARTESIAN_POINT('Ctrl Pts',(31.450714885868,-33.5757620187004,42.1091125534892));
#42556=CARTESIAN_POINT('Ctrl Pts',(31.9714127123162,-33.757268556938,42.1461558165625));
#42557=CARTESIAN_POINT('Ctrl Pts',(32.5909730039986,-33.6551624653271,42.1831990796357));
#42558=CARTESIAN_POINT('Ctrl Pts',(33.0258890444035,-33.3161660007344,42.220242342709));
#42559=CARTESIAN_POINT('Ctrl Pts',(33.4220927932116,-33.0073439348036,42.2539883496027));
#42560=CARTESIAN_POINT('Ctrl Pts',(33.6650600854439,-32.5019263014425,42.2877343564965));
#42561=CARTESIAN_POINT('Ctrl Pts',(33.6682077276635,-31.9991447210259,42.3214803633902));
#42562=CARTESIAN_POINT('Ctrl Pts',(32.5301702171886,-33.9851743256717,41.));
#42563=CARTESIAN_POINT('Ctrl Pts',(32.5988371200409,-33.9597495173352,41.));
#42564=CARTESIAN_POINT('Ctrl Pts',(32.6658006735426,-33.9304353732127,41.));
#42565=CARTESIAN_POINT('Ctrl Pts',(32.7308718973377,-33.8975258144197,41.));
#42566=CARTESIAN_POINT('Ctrl Pts',(32.7977522078449,-33.8637013159338,41.));
#42567=CARTESIAN_POINT('Ctrl Pts',(32.8626342777603,-33.826078018407,41.));
#42568=CARTESIAN_POINT('Ctrl Pts',(32.925281707376,-33.7849304046057,41.));
#42569=CARTESIAN_POINT('Ctrl Pts',(32.9782123635771,-33.7501648888779,41.));
#42570=CARTESIAN_POINT('Ctrl Pts',(33.0295474834986,-33.7128824829906,41.));
#42571=CARTESIAN_POINT('Ctrl Pts',(33.0791217504879,-33.6732307266858,41.));
#42572=CARTESIAN_POINT('Ctrl Pts',(33.1011524559357,-33.6556095652105,41.));
#42573=CARTESIAN_POINT('Ctrl Pts',(33.1228351080429,-33.6375203027614,41.));
#42574=CARTESIAN_POINT('Ctrl Pts',(33.1441536442999,-33.6189751639077,41.));
#42575=CARTESIAN_POINT('Ctrl Pts',(33.1558677305351,-33.6087850010767,41.));
#42576=CARTESIAN_POINT('Ctrl Pts',(33.1674718626525,-33.5984571902042,41.));
#42577=CARTESIAN_POINT('Ctrl Pts',(33.178963241537,-33.5879937176865,41.));
#42578=CARTESIAN_POINT('Ctrl Pts',(33.1895552130653,-33.5783492003393,41.));
#42579=CARTESIAN_POINT('Ctrl Pts',(33.2000528216363,-33.5685879135171,41.));
#42580=CARTESIAN_POINT('Ctrl Pts',(33.210437993979,-33.5587268613668,41.));
#42581=CARTESIAN_POINT('Ctrl Pts',(33.2635230443273,-33.5083209140594,41.));
#42582=CARTESIAN_POINT('Ctrl Pts',(33.3137681124905,-33.4552266753419,41.));
#42583=CARTESIAN_POINT('Ctrl Pts',(33.360954505967,-33.3997034771336,41.));
#42584=CARTESIAN_POINT('Ctrl Pts',(33.4077743219468,-33.3446116226562,41.));
#42585=CARTESIAN_POINT('Ctrl Pts',(33.451583310905,-33.2871275187766,41.));
#42586=CARTESIAN_POINT('Ctrl Pts',(33.4921230471312,-33.2274802596658,41.));
#42587=CARTESIAN_POINT('Ctrl Pts',(33.5258091626199,-33.1779169263528,41.));
#42588=CARTESIAN_POINT('Ctrl Pts',(33.5572373380051,-33.1268593641302,41.));
#42589=CARTESIAN_POINT('Ctrl Pts',(33.5862317099631,-33.0744325355151,41.));
#42590=CARTESIAN_POINT('Ctrl Pts',(33.5983395910643,-33.0525393967949,41.));
#42591=CARTESIAN_POINT('Ctrl Pts',(33.6100227318467,-33.0304074395486,41.));
#42592=CARTESIAN_POINT('Ctrl Pts',(33.6212668835334,-33.0080456806059,41.));
#42593=CARTESIAN_POINT('Ctrl Pts',(33.626466482389,-32.9977050004506,41.));
#42594=CARTESIAN_POINT('Ctrl Pts',(33.6315721959925,-32.9873151798452,41.));
#42595=CARTESIAN_POINT('Ctrl Pts',(33.636582550181,-32.9768771123835,41.));
#42596=CARTESIAN_POINT('Ctrl Pts',(33.6418163462648,-32.9659735485738,41.));
#42597=CARTESIAN_POINT('Ctrl Pts',(33.646942482252,-32.9550247828872,41.));
#42598=CARTESIAN_POINT('Ctrl Pts',(33.6519578880443,-32.9440361447188,41.));
#42599=CARTESIAN_POINT('Ctrl Pts',(33.6804982443946,-32.8815048836164,41.));
#42600=CARTESIAN_POINT('Ctrl Pts',(33.7054776090138,-32.817640230646,41.));
#42601=CARTESIAN_POINT('Ctrl Pts',(33.7266725048855,-32.7526465165606,41.));
#42602=CARTESIAN_POINT('Ctrl Pts',(33.7458696726495,-32.6937787948011,41.));
#42603=CARTESIAN_POINT('Ctrl Pts',(33.7619618380551,-32.6339842234184,41.));
#42604=CARTESIAN_POINT('Ctrl Pts',(33.7747462836708,-32.5734098051776,41.));
#42605=CARTESIAN_POINT('Ctrl Pts',(33.789880467178,-32.5017020136112,41.));
#42606=CARTESIAN_POINT('Ctrl Pts',(33.8003799022934,-32.4288998459686,41.));
#42607=CARTESIAN_POINT('Ctrl Pts',(33.8063197386492,-32.3554264965557,41.));
#42608=CARTESIAN_POINT('Ctrl Pts',(33.8076266775032,-32.3392601967906,41.));
#42609=CARTESIAN_POINT('Ctrl Pts',(33.808712649019,-32.3230614848392,41.));
#42610=CARTESIAN_POINT('Ctrl Pts',(33.809578084761,-32.3068350328842,41.));
#42611=CARTESIAN_POINT('Ctrl Pts',(33.8104757224762,-32.2900048113543,41.));
#42612=CARTESIAN_POINT('Ctrl Pts',(33.8111361175212,-32.2731385190501,41.));
#42613=CARTESIAN_POINT('Ctrl Pts',(33.8115591884844,-32.2562757703559,41.));
#42614=CARTESIAN_POINT('Ctrl Pts',(33.8132793631208,-32.1877131056438,41.));
#42615=CARTESIAN_POINT('Ctrl Pts',(33.8110879096862,-32.1191225382936,41.));
#42616=CARTESIAN_POINT('Ctrl Pts',(33.8051054090175,-32.0508425096977,41.));
#42617=CARTESIAN_POINT('Ctrl Pts',(33.799124181534,-31.9825770123365,41.));
#42618=CARTESIAN_POINT('Ctrl Pts',(33.7893530665424,-31.9146208497202,41.));
#42619=CARTESIAN_POINT('Ctrl Pts',(33.7758629639258,-31.8473272796643,41.));
#42620=CARTESIAN_POINT('Ctrl Pts',(33.7661049760548,-31.7986508641426,41.));
#42621=CARTESIAN_POINT('Ctrl Pts',(33.7544000640131,-31.7503214006864,41.));
#42622=CARTESIAN_POINT('Ctrl Pts',(33.7407608724217,-31.7024822288915,41.));
#42623=CARTESIAN_POINT('Ctrl Pts',(33.7305262530612,-31.6665845211305,41.));
#42624=CARTESIAN_POINT('Ctrl Pts',(33.7192022406327,-31.6309630389482,41.));
#42625=CARTESIAN_POINT('Ctrl Pts',(33.7067902653119,-31.59568252048,41.));
#42626=CARTESIAN_POINT('Ctrl Pts',(33.7026575477152,-31.5839354443118,41.));
#42627=CARTESIAN_POINT('Ctrl Pts',(33.6984073995683,-31.5722353381128,41.));
#42628=CARTESIAN_POINT('Ctrl Pts',(33.6940404882691,-31.560584828957,41.));
#42629=CARTESIAN_POINT('Ctrl Pts',(33.6709167177176,-31.4988927811749,41.));
#42630=CARTESIAN_POINT('Ctrl Pts',(33.6445204253536,-31.4385842551238,41.));
#42631=CARTESIAN_POINT('Ctrl Pts',(33.6149016066083,-31.3799934310527,41.));
#42632=CARTESIAN_POINT('Ctrl Pts',(33.5940761832706,-31.3387973683238,41.));
#42633=CARTESIAN_POINT('Ctrl Pts',(33.5716567844582,-31.2984510155133,41.));
#42634=CARTESIAN_POINT('Ctrl Pts',(33.5476503990608,-31.2590818683295,41.));
#42635=CARTESIAN_POINT('Ctrl Pts',(33.5399365575065,-31.2464315938929,41.));
#42636=CARTESIAN_POINT('Ctrl Pts',(33.5320577131048,-31.2338806239069,41.));
#42637=CARTESIAN_POINT('Ctrl Pts',(33.5240173880638,-31.221438771236,41.));
#42638=CARTESIAN_POINT('Ctrl Pts',(33.4897744370523,-31.168450148347,41.));
#42639=CARTESIAN_POINT('Ctrl Pts',(33.452675776676,-31.117545406851,41.));
#42640=CARTESIAN_POINT('Ctrl Pts',(33.412755652156,-31.0690398416308,41.));
#42641=CARTESIAN_POINT('Ctrl Pts',(33.3759796503983,-31.0243545914407,41.));
#42642=CARTESIAN_POINT('Ctrl Pts',(33.3368085344288,-30.9817053877508,41.));
#42643=CARTESIAN_POINT('Ctrl Pts',(33.295247657559,-30.9413716077237,41.));
#42644=CARTESIAN_POINT('Ctrl Pts',(33.2874058185866,-30.9337613013024,41.));
#42645=CARTESIAN_POINT('Ctrl Pts',(33.279478847569,-30.9262335309294,41.));
#42646=CARTESIAN_POINT('Ctrl Pts',(33.2714683511891,-30.9187889684226,41.));
#42647=CARTESIAN_POINT('Origin',(32.,-32.,48.));
#42648=CARTESIAN_POINT('Origin',(32.,-32.,55.));
#42649=CARTESIAN_POINT('Origin',(-32.,-32.,55.));
#42650=CARTESIAN_POINT('Origin',(-32.,32.,55.));
#42651=CARTESIAN_POINT('Origin',(32.,32.,55.));
#42652=CARTESIAN_POINT('Origin',(-45.,-3.,179.));
#42653=CARTESIAN_POINT('',(-49.9099188538711,-3.,179.));
#42654=CARTESIAN_POINT('',(-49.9099188538711,-3.,41.));
#42655=CARTESIAN_POINT('',(-49.9099188538711,-3.,41.));
#42656=CARTESIAN_POINT('',(-45.,-3.,179.));
#42657=CARTESIAN_POINT('',(-22.5,-3.,179.));
#42658=CARTESIAN_POINT('',(-45.,-3.,41.));
#42659=CARTESIAN_POINT('',(-45.,-3.,179.));
#42660=CARTESIAN_POINT('',(-22.5,-3.,41.));
#42661=CARTESIAN_POINT('Origin',(-45.,3.,179.));
#42662=CARTESIAN_POINT('',(-45.,3.,179.));
#42663=CARTESIAN_POINT('',(-45.,1.5,179.));
#42664=CARTESIAN_POINT('',(-45.,3.,41.));
#42665=CARTESIAN_POINT('',(-45.,3.,179.));
#42666=CARTESIAN_POINT('',(-45.,1.5,41.));
#42667=CARTESIAN_POINT('Origin',(-53.,3.,179.));
#42668=CARTESIAN_POINT('',(-49.9099188538711,3.,41.));
#42669=CARTESIAN_POINT('',(-49.9099188538711,3.,179.));
#42670=CARTESIAN_POINT('',(-49.9099188538711,3.,41.));
#42671=CARTESIAN_POINT('',(-26.5,3.,41.));
#42672=CARTESIAN_POINT('',(-26.5,3.,179.));
#42673=CARTESIAN_POINT('Origin',(0.,0.,41.));
#42674=CARTESIAN_POINT('Origin',(0.,0.,41.));
#42675=CARTESIAN_POINT('',(-40.,-4.89858719658941E-15,41.));
#42676=CARTESIAN_POINT('Origin',(0.,0.,41.));
#42677=CARTESIAN_POINT('Origin',(80.,0.,57.8647410325605));
#42678=CARTESIAN_POINT('Ctrl Pts',(73.8864642614677,0.000114121245111225,
53.4897410325605));
#42679=CARTESIAN_POINT('Ctrl Pts',(73.88634736256,0.135162929769602,53.4835872578684));
#42680=CARTESIAN_POINT('Ctrl Pts',(73.9231853293536,1.26913664614987,53.4319125319522));
#42681=CARTESIAN_POINT('Ctrl Pts',(74.5968874696183,3.36192360377817,53.3347168548118));
#42682=CARTESIAN_POINT('Ctrl Pts',(76.8165950932171,5.51017981513921,53.1981540011394));
#42683=CARTESIAN_POINT('Ctrl Pts',(79.7864084401088,6.36007322196442,53.0615911474669));
#42684=CARTESIAN_POINT('Ctrl Pts',(82.8065504208398,5.71134182197275,52.9250282937945));
#42685=CARTESIAN_POINT('Ctrl Pts',(85.1653847950113,3.71684696339025,52.7884654401221));
#42686=CARTESIAN_POINT('Ctrl Pts',(86.3070993591023,0.846551199044585,52.6519025864497));
#42687=CARTESIAN_POINT('Ctrl Pts',(85.9626718510223,-2.22321740518142,52.5153397327772));
#42688=CARTESIAN_POINT('Ctrl Pts',(84.2132597448983,-4.769129230128,52.3787768791048));
#42689=CARTESIAN_POINT('Ctrl Pts',(81.4710770800909,-6.19129093756104,52.2422140254323));
#42690=CARTESIAN_POINT('Ctrl Pts',(78.3822644661494,-6.15459852582288,52.1056511717599));
#42691=CARTESIAN_POINT('Ctrl Pts',(75.6746389387688,-4.66769782144369,51.9690883180875));
#42692=CARTESIAN_POINT('Ctrl Pts',(74.1666214617889,-2.35736179104307,51.8471182716877));
#42693=CARTESIAN_POINT('Ctrl Pts',(73.8875345335937,-0.678780393631098,
51.7706691765121));
#42694=CARTESIAN_POINT('Ctrl Pts',(73.8869923021753,0.000128310058932178,
51.7397410325606));
#42695=CARTESIAN_POINT('Ctrl Pts',(73.8870077577991,0.000138281717805347,
53.6352589674395));
#42696=CARTESIAN_POINT('Ctrl Pts',(73.8867593267721,0.329017176271155,53.6202764579539));
#42697=CARTESIAN_POINT('Ctrl Pts',(73.9922018351304,1.65695988743391,53.5597729972442));
#42698=CARTESIAN_POINT('Ctrl Pts',(74.9405084533092,3.85979119586914,53.4537485853103));
#42699=CARTESIAN_POINT('Ctrl Pts',(77.3541911747203,5.78754789219838,53.3171857316378));
#42700=CARTESIAN_POINT('Ctrl Pts',(80.391275596298,6.35162199178929,53.1806228779654));
#42701=CARTESIAN_POINT('Ctrl Pts',(83.3361779879638,5.41904570738785,53.044060024293));
#42702=CARTESIAN_POINT('Ctrl Pts',(85.4949699527806,3.20958767782661,52.9074971706206));
#42703=CARTESIAN_POINT('Ctrl Pts',(86.3589850655242,0.243850535977484,52.7709343169481));
#42704=CARTESIAN_POINT('Ctrl Pts',(85.7246308116887,-2.7793433146957,52.6343714632757));
#42705=CARTESIAN_POINT('Ctrl Pts',(83.7413822653001,-5.14764123692896,52.4978086096033));
#42706=CARTESIAN_POINT('Ctrl Pts',(80.8765513474216,-6.30299985802483,52.3612457559308));
#42707=CARTESIAN_POINT('Ctrl Pts',(77.8051787527545,-5.9731825630531,52.2246829022584));
#42708=CARTESIAN_POINT('Ctrl Pts',(75.2509719030383,-4.23590394123515,52.0881200485859));
#42709=CARTESIAN_POINT('Ctrl Pts',(74.0619250280353,-1.96965792532052,51.9749787369797));
#42710=CARTESIAN_POINT('Ctrl Pts',(73.8871918657965,-0.485173931894543,
51.9073583765975));
#42711=CARTESIAN_POINT('Ctrl Pts',(73.8872279103786,-1.26095903429935E-5,
51.8852589674395));
#42712=CARTESIAN_POINT('Ctrl Pts',(83.8799476118145,3.36633437021264,54.));
#42713=CARTESIAN_POINT('Ctrl Pts',(84.4301347069223,2.73220333302164,53.9544790487759));
#42714=CARTESIAN_POINT('Ctrl Pts',(85.2131282914198,1.18960825322011,53.8634371463276));
#42715=CARTESIAN_POINT('Ctrl Pts',(85.1591137460442,-1.40568202732916,53.7268742926551));
#42716=CARTESIAN_POINT('Ctrl Pts',(83.8893923039574,-3.66938767399442,53.5903114389827));
#42717=CARTESIAN_POINT('Ctrl Pts',(81.7032246129214,-5.06866334381662,53.4537485853103));
#42718=CARTESIAN_POINT('Ctrl Pts',(79.1157173213369,-5.27352492015549,53.3171857316378));
#42719=CARTESIAN_POINT('Ctrl Pts',(76.7365771085195,-4.23582589027655,53.1806228779654));
#42720=CARTESIAN_POINT('Ctrl Pts',(75.1263956128531,-2.20002026082073,53.044060024293));
#42721=CARTESIAN_POINT('Ctrl Pts',(74.6645825100926,0.354167410375346,52.9074971706205));
#42722=CARTESIAN_POINT('Ctrl Pts',(75.4599536596021,2.82490673074183,52.7709343169481));
#42723=CARTESIAN_POINT('Ctrl Pts',(77.3250962818604,4.63001123222775,52.6343714632757));
#42724=CARTESIAN_POINT('Ctrl Pts',(79.8205264883211,5.3441469141497,52.4978086096033));
#42725=CARTESIAN_POINT('Ctrl Pts',(82.3582460842022,4.79904062552954,52.3612457559308));
#42726=CARTESIAN_POINT('Ctrl Pts',(84.3402920452745,3.12313640685312,52.2246829022584));
#42727=CARTESIAN_POINT('Ctrl Pts',(85.2996348313694,0.711327341707319,52.088120048586));
#42728=CARTESIAN_POINT('Ctrl Pts',(85.0102244519263,-1.86809176887346,51.9515571949135));
#42729=CARTESIAN_POINT('Ctrl Pts',(83.5402546917934,-4.00733236377704,51.8149943412411));
#42730=CARTESIAN_POINT('Ctrl Pts',(81.2360945799954,-5.2023250682561,51.6784314875687));
#42731=CARTESIAN_POINT('Ctrl Pts',(78.6406734546261,-5.17149371897446,51.5418686338963));
#42732=CARTESIAN_POINT('Ctrl Pts',(76.3655504958444,-3.92210310134558,51.4053057802238));
#42733=CARTESIAN_POINT('Ctrl Pts',(74.9468130152413,-1.74854717831912,51.2687429265514));
#42734=CARTESIAN_POINT('Ctrl Pts',(74.7187581804446,0.837018984838123,51.132180072879));
#42735=CARTESIAN_POINT('Ctrl Pts',(75.7351225611137,3.22535833181042,50.9956172192065));
#42736=CARTESIAN_POINT('Ctrl Pts',(77.7564201786535,4.8537063696547,50.8590543655341));
#42737=CARTESIAN_POINT('Ctrl Pts',(80.306372596804,5.33837538670167,50.7224915118616));
#42738=CARTESIAN_POINT('Ctrl Pts',(82.7841344280458,4.5651628036752,50.5859286581892));
#42739=CARTESIAN_POINT('Ctrl Pts',(84.6058705556718,2.71626073156826,50.4493658045168));
#42740=CARTESIAN_POINT('Ctrl Pts',(85.3423252250402,0.227326037591453,50.3128029508444));
#42741=CARTESIAN_POINT('Ctrl Pts',(84.8199675937518,-2.31517349947107,50.176240097172));
#42742=CARTESIAN_POINT('Ctrl Pts',(83.1618808107925,-4.31214861476392,50.0396772434995));
#42743=CARTESIAN_POINT('Ctrl Pts',(80.7587599293508,-5.29305198416577,49.9031143898271));
#42744=CARTESIAN_POINT('Ctrl Pts',(78.1768524162312,-5.02675330857473,49.7665515361547));
#42745=CARTESIAN_POINT('Ctrl Pts',(76.0245332392176,-3.57600055528289,49.6299886824822));
#42746=CARTESIAN_POINT('Ctrl Pts',(74.8089534497408,-1.28263465200007,49.4934258288098));
#42747=CARTESIAN_POINT('Ctrl Pts',(74.8165401608961,1.31295850424349,49.3568629751374));
#42748=CARTESIAN_POINT('Ctrl Pts',(76.0455057156385,3.59917919704222,49.2203001214649));
#42749=CARTESIAN_POINT('Ctrl Pts',(78.2062689124828,5.03732515559033,49.0837372677925));
#42750=CARTESIAN_POINT('Ctrl Pts',(80.7896890352764,5.28852599171387,48.9471744141201));
#42751=CARTESIAN_POINT('Ctrl Pts',(83.1870346999595,4.29359124262232,48.8106115604476));
#42752=CARTESIAN_POINT('Ctrl Pts',(84.8334192542769,2.2869574219591,48.6740487067752));
#42753=CARTESIAN_POINT('Ctrl Pts',(85.3409050416308,-0.258552265030627,
48.5374858531028));
#42754=CARTESIAN_POINT('Ctrl Pts',(84.5899131661994,-2.74313927175038,48.4009229994303));
#42755=CARTESIAN_POINT('Ctrl Pts',(82.7573998728133,-4.58136026512633,48.2643601457579));
#42756=CARTESIAN_POINT('Ctrl Pts',(80.2751603401001,-5.34007516096028,48.1277972920854));
#42757=CARTESIAN_POINT('Ctrl Pts',(77.7280847657421,-4.84050793882374,47.9912344384131));
#42758=CARTESIAN_POINT('Ctrl Pts',(75.7163406664372,-3.20037164270791,47.8546715847406));
#42759=CARTESIAN_POINT('Ctrl Pts',(74.7139553825858,-0.806131651887682,
47.7181087310682));
#42760=CARTESIAN_POINT('Ctrl Pts',(74.9571209976267,1.77805717143511,47.5815458773958));
#42761=CARTESIAN_POINT('Ctrl Pts',(76.3885403882258,3.94328231426472,47.4449830237233));
#42762=CARTESIAN_POINT('Ctrl Pts',(78.6709281476767,5.17935169194281,47.3084201700509));
#42763=CARTESIAN_POINT('Ctrl Pts',(81.2664851594074,5.19501022890906,47.1718573163784));
#42764=CARTESIAN_POINT('Ctrl Pts',(83.5636202237454,3.98656830348881,47.035294462706));
#42765=CARTESIAN_POINT('Ctrl Pts',(85.0210593160944,1.83877113359181,46.8987316090335));
#42766=CARTESIAN_POINT('Ctrl Pts',(85.2953860064122,-0.742295750063858,
46.7621687553612));
#42767=CARTESIAN_POINT('Ctrl Pts',(84.3219606859846,-3.14845545724768,46.6256059016887));
#42768=CARTESIAN_POINT('Ctrl Pts',(82.3301516009419,-4.81274448252728,46.4890430480163));
#42769=CARTESIAN_POINT('Ctrl Pts',(79.7892888034983,-5.34300633811507,46.3524801943438));
#42770=CARTESIAN_POINT('Ctrl Pts',(77.2980758934855,-4.61429540234531,46.2159173406714));
#42771=CARTESIAN_POINT('Ctrl Pts',(75.4435174658283,-2.79831786136907,46.079354486999));
#42772=CARTESIAN_POINT('Ctrl Pts',(74.6626031950001,-0.322972573830058,
45.9427916333266));
#42773=CARTESIAN_POINT('Ctrl Pts',(75.1393399410234,2.22847475384808,45.8062287796541));
#42774=CARTESIAN_POINT('Ctrl Pts',(76.7613942058816,4.25482648856233,45.6696659259817));
#42775=CARTESIAN_POINT('Ctrl Pts',(79.1465612800289,5.27861329221261,45.5331030723093));
#42776=CARTESIAN_POINT('Ctrl Pts',(81.7328241529721,5.05860024041677,45.3965402186368));
#42777=CARTESIAN_POINT('Ctrl Pts',(83.9107816033226,3.64662901713134,45.2599773649644));
#42778=CARTESIAN_POINT('Ctrl Pts',(85.1672414323057,1.37540245664025,45.123414511292));
#42779=CARTESIAN_POINT('Ctrl Pts',(85.2061439615261,-1.21991023822647,44.9868516576195));
#42780=CARTESIAN_POINT('Ctrl Pts',(84.0183225865111,-3.52777543619547,44.8502888039471));
#42781=CARTESIAN_POINT('Ctrl Pts',(81.8836637040732,-5.00439077085035,44.7137259502747));
#42782=CARTESIAN_POINT('Ctrl Pts',(79.3051570697518,-5.30182131346047,44.5771630966022));
#42783=CARTESIAN_POINT('Ctrl Pts',(76.8903763021125,-4.34998349362811,44.4406002429298));
#42784=CARTESIAN_POINT('Ctrl Pts',(75.20831628743,-2.37315889402526,44.3040373892574));
#42785=CARTESIAN_POINT('Ctrl Pts',(74.6553208923488,0.162853228334741,44.1674745355849));
#42786=CARTESIAN_POINT('Ctrl Pts',(75.3616924434739,2.66049223770987,44.0309116819125));
#42787=CARTESIAN_POINT('Ctrl Pts',(77.1609885844208,4.53123935855979,43.8943488282401));
#42788=CARTESIAN_POINT('Ctrl Pts',(79.6292410961376,5.33429037095907,43.7577859745677));
#42789=CARTESIAN_POINT('Ctrl Pts',(82.1848555418488,4.88042234010467,43.6212231208952));
#42790=CARTESIAN_POINT('Ctrl Pts',(84.2256523932433,3.2765801939049,43.4846602672228));
#42791=CARTESIAN_POINT('Ctrl Pts',(85.2707586024651,0.900677349257217,43.3480974135504));
#42792=CARTESIAN_POINT('Ctrl Pts',(85.0739157663178,-1.68745217721733,43.2115345598779));
#42793=CARTESIAN_POINT('Ctrl Pts',(83.6815059410305,-3.87796718981677,43.0749717062055));
#42794=CARTESIAN_POINT('Ctrl Pts',(81.4216227696065,-5.15471683823141,42.9384088525331));
#42795=CARTESIAN_POINT('Ctrl Pts',(78.8267624800316,-5.21685994000325,42.8018459988606));
#42796=CARTESIAN_POINT('Ctrl Pts',(76.5083523841484,-4.04975502185875,42.6652831451882));
#42797=CARTESIAN_POINT('Ctrl Pts',(75.0126789436487,-1.92840426961145,42.5287202915158));
#42798=CARTESIAN_POINT('Ctrl Pts',(74.6921690274326,0.647332400775962,42.3921574378433));
#42799=CARTESIAN_POINT('Ctrl Pts',(75.6223416665355,3.07054676838256,42.2555945841709));
#42800=CARTESIAN_POINT('Ctrl Pts',(77.5840260405478,4.77022963457038,42.1190317304985));
#42801=CARTESIAN_POINT('Ctrl Pts',(80.1149778044545,5.34594259971938,41.9824688768261));
#42802=CARTESIAN_POINT('Ctrl Pts',(82.6188542837379,4.66190740327312,41.8459060231536));
#42803=CARTESIAN_POINT('Ctrl Pts',(84.5056048859645,2.87956962377209,41.7093431694812));
#42804=CARTESIAN_POINT('Ctrl Pts',(85.3307462672301,0.418352259874965,41.5727803158088));
#42805=CARTESIAN_POINT('Ctrl Pts',(85.0431484786228,-1.28750999880251,41.4817384133605));
#42806=CARTESIAN_POINT('Ctrl Pts',(84.7069873520512,-2.056810791038,41.4362174621363));
#42807=CARTESIAN_POINT('Ctrl Pts',(84.1258079218638,3.57964859370108,54.1879275126212));
#42808=CARTESIAN_POINT('Ctrl Pts',(84.7108586757943,2.90533462905485,54.1424065613971));
#42809=CARTESIAN_POINT('Ctrl Pts',(85.5434681481107,1.26499005814018,54.0513646589488));
#42810=CARTESIAN_POINT('Ctrl Pts',(85.4860308676361,-1.49475576070059,53.9148018052764));
#42811=CARTESIAN_POINT('Ctrl Pts',(84.1358510950097,-3.90190545038712,53.7782389516039));
#42812=CARTESIAN_POINT('Ctrl Pts',(81.8111527019866,-5.38984890246992,53.6416760979315));
#42813=CARTESIAN_POINT('Ctrl Pts',(79.0596830561099,-5.60769192487844,53.5051132442591));
#42814=CARTESIAN_POINT('Ctrl Pts',(76.5297840679439,-4.50423710890409,53.3685503905866));
#42815=CARTESIAN_POINT('Ctrl Pts',(74.8175703385033,-2.33942875741822,53.2319875369142));
#42816=CARTESIAN_POINT('Ctrl Pts',(74.3264935641706,0.376609906521191,53.0954246832418));
#42817=CARTESIAN_POINT('Ctrl Pts',(75.1722649296075,3.00391235508727,52.9588618295694));
#42818=CARTESIAN_POINT('Ctrl Pts',(77.1555958856459,4.9234007598649,52.8222989758969));
#42819=CARTESIAN_POINT('Ctrl Pts',(79.8091538055837,5.68278901675461,52.6857361222245));
#42820=CARTESIAN_POINT('Ctrl Pts',(82.5076808630813,5.10314102434395,52.5491732685521));
#42821=CARTESIAN_POINT('Ctrl Pts',(84.6153229618534,3.32103992569883,52.4126104148796));
#42822=CARTESIAN_POINT('Ctrl Pts',(85.6354563406138,0.756401960819743,52.2760475612072));
#42823=CARTESIAN_POINT('Ctrl Pts',(85.3277069182916,-1.98646698097611,52.1394847075348));
#42824=CARTESIAN_POINT('Ctrl Pts',(83.7645897094951,-4.26126465256069,52.0029218538623));
#42825=CARTESIAN_POINT('Ctrl Pts',(81.3144220800272,-5.53198035802442,51.8663590001899));
#42826=CARTESIAN_POINT('Ctrl Pts',(78.5545371251339,-5.49919532125727,51.7297961465174));
#42827=CARTESIAN_POINT('Ctrl Pts',(76.1352466434858,-4.17063467471162,51.5932332928451));
#42828=CARTESIAN_POINT('Ctrl Pts',(74.6266081457151,-1.85934721852798,51.4566704391726));
#42829=CARTESIAN_POINT('Ctrl Pts',(74.3841021796143,0.890058295601701,51.3201075855002));
#42830=CARTESIAN_POINT('Ctrl Pts',(75.4648704354783,3.42973933867357,51.1835447318277));
#42831=CARTESIAN_POINT('Ctrl Pts',(77.6142514470921,5.16127076802383,51.0469818781553));
#42832=CARTESIAN_POINT('Ctrl Pts',(80.3257864830666,5.67665176541806,50.9104190244829));
#42833=CARTESIAN_POINT('Ctrl Pts',(82.960556437357,4.85444308646029,50.7738561708105));
#42834=CARTESIAN_POINT('Ctrl Pts',(84.8977303631125,2.88838179413223,50.637293317138));
#42835=CARTESIAN_POINT('Ctrl Pts',(85.6808518928265,0.241730987265083,50.5007304634656));
#42836=CARTESIAN_POINT('Ctrl Pts',(85.1253940699802,-2.46187890154005,50.3641676097932));
#42837=CARTESIAN_POINT('Ctrl Pts',(83.3622394429846,-4.58539616897732,50.2276047561207));
#42838=CARTESIAN_POINT('Ctrl Pts',(80.8068402052069,-5.62845635869168,50.0910419024483));
#42839=CARTESIAN_POINT('Ctrl Pts',(78.0613251784804,-5.34528315759231,49.9544790487759));
#42840=CARTESIAN_POINT('Ctrl Pts',(75.7726201753865,-3.80260067807349,49.8179161951034));
#42841=CARTESIAN_POINT('Ctrl Pts',(74.4800128448624,-1.36391125281304,49.681353341431));
#42842=CARTESIAN_POINT('Ctrl Pts',(74.4880803024976,1.39615663402034,49.5447904877586));
#42843=CARTESIAN_POINT('Ctrl Pts',(75.7949216129355,3.82724807885216,49.4082276340861));
#42844=CARTESIAN_POINT('Ctrl Pts',(78.0926057073459,5.35652490993785,49.2716647804137));
#42845=CARTESIAN_POINT('Ctrl Pts',(80.8397291931549,5.62364356806135,49.1351019267413));
#42846=CARTESIAN_POINT('Ctrl Pts',(83.3889872565054,4.56566287341486,48.9985390730688));
#42847=CARTESIAN_POINT('Ctrl Pts',(85.1396981207328,2.43187485824618,48.8619762193964));
#42848=CARTESIAN_POINT('Ctrl Pts',(85.6793417167757,-0.274935924400359,
48.725413365724));
#42849=CARTESIAN_POINT('Ctrl Pts',(84.8807618030997,-2.91696354448211,48.5888505120515));
#42850=CARTESIAN_POINT('Ctrl Pts',(82.9321277958387,-4.87166693107243,48.4522876583791));
#42851=CARTESIAN_POINT('Ctrl Pts',(80.292596401949,-5.67845924912743,48.3157248047067));
#42852=CARTESIAN_POINT('Ctrl Pts',(77.5841205064826,-5.14723599334988,48.1791619510343));
#42853=CARTESIAN_POINT('Ctrl Pts',(75.4448983900806,-3.40316932016962,48.0425990973618));
#42854=CARTESIAN_POINT('Ctrl Pts',(74.3789950432723,-0.857213727653378,
47.9060362436894));
#42855=CARTESIAN_POINT('Ctrl Pts',(74.6375693131429,1.8907271688658,47.7694733900169));
#42856=CARTESIAN_POINT('Ctrl Pts',(76.1596933344209,4.19315594901299,47.6329105363445));
#42857=CARTESIAN_POINT('Ctrl Pts',(78.5867089647436,5.50755122972981,47.4963476826721));
#42858=CARTESIAN_POINT('Ctrl Pts',(81.3467384166979,5.52420199987513,47.3597848289997));
#42859=CARTESIAN_POINT('Ctrl Pts',(83.7894358431213,4.23918483783166,47.2232219753272));
#42860=CARTESIAN_POINT('Ctrl Pts',(85.3392283543752,1.9552883874944,47.0866591216548));
#42861=CARTESIAN_POINT('Ctrl Pts',(85.6309382807271,-0.789332741672519,
46.9500962679824));
#42862=CARTESIAN_POINT('Ctrl Pts',(84.5958300008798,-3.34796336620454,46.8135334143099));
#42863=CARTESIAN_POINT('Ctrl Pts',(82.4778061190918,-5.11771325248156,46.6769705606375));
#42864=CARTESIAN_POINT('Ctrl Pts',(79.7759366850458,-5.68157616593548,46.540407706965));
#42865=CARTESIAN_POINT('Ctrl Pts',(77.126863298621,-4.90668906632807,46.4038448532927));
#42866=CARTESIAN_POINT('Ctrl Pts',(75.154787224942,-2.97563863109226,46.2672819996202));
#42867=CARTESIAN_POINT('Ctrl Pts',(74.3243888259871,-0.343438349423903,
46.1307191459478));
#42868=CARTESIAN_POINT('Ctrl Pts',(74.8313349088149,2.36968632388313,45.9941562922753));
#42869=CARTESIAN_POINT('Ctrl Pts',(76.556173748202,4.52444171648408,45.8575934386029));
#42870=CARTESIAN_POINT('Ctrl Pts',(79.0924815013068,5.61310273137458,45.7210305849305));
#42871=CARTESIAN_POINT('Ctrl Pts',(81.8426278735721,5.37914813125352,45.5844677312581));
#42872=CARTESIAN_POINT('Ctrl Pts',(84.1585957682871,3.87770464765186,45.4479048775857));
#42873=CARTESIAN_POINT('Ctrl Pts',(85.4946735803011,1.46255746703329,45.3113420239132));
#42874=CARTESIAN_POINT('Ctrl Pts',(85.5360412427791,-1.29721218645108,45.1747791702407));
#42875=CARTESIAN_POINT('Ctrl Pts',(84.2729512918033,-3.75131968196986,45.0382163165683));
#42876=CARTESIAN_POINT('Ctrl Pts',(82.003025661668,-5.32150357484349,44.9016534628959));
#42877=CARTESIAN_POINT('Ctrl Pts',(79.2611270169371,-5.63778137332934,44.7650906092235));
#42878=CARTESIAN_POINT('Ctrl Pts',(76.6933290419456,-4.62562852738992,44.628527755551));
#42879=CARTESIAN_POINT('Ctrl Pts',(74.9046820734928,-2.52353865165512,44.4919649018786));
#42880=CARTESIAN_POINT('Ctrl Pts',(74.3166450662836,0.173172734992249,44.3554020482062));
#42881=CARTESIAN_POINT('Ctrl Pts',(75.0677772033611,2.82907942287063,44.2188391945338));
#42882=CARTESIAN_POINT('Ctrl Pts',(76.9810891897119,4.81837001728588,44.0822763408613));
#42883=CARTESIAN_POINT('Ctrl Pts',(79.6057472482362,5.67230789483062,43.9457134871889));
#42884=CARTESIAN_POINT('Ctrl Pts',(82.32330309699,5.18967964709919,43.8091506335164));
#42885=CARTESIAN_POINT('Ctrl Pts',(84.4934189487503,3.48420697214328,43.672587779844));
#42886=CARTESIAN_POINT('Ctrl Pts',(85.6047503141703,0.957750494180222,43.5360249261716));
#42887=CARTESIAN_POINT('Ctrl Pts',(85.3954341547806,-1.7943808156919,43.3994620724992));
#42888=CARTESIAN_POINT('Ctrl Pts',(83.9147916146189,-4.12370200663389,43.2628992188267));
#42889=CARTESIAN_POINT('Ctrl Pts',(81.5117066186369,-5.48135534134026,43.1263363651543));
#42890=CARTESIAN_POINT('Ctrl Pts',(78.7524180379719,-5.54743625975233,42.9897735114818));
#42891=CARTESIAN_POINT('Ctrl Pts',(76.2870974468905,-4.30637550360597,42.8532106578094));
#42892=CARTESIAN_POINT('Ctrl Pts',(74.6966477948012,-2.05060129881445,42.716647804137));
#42893=CARTESIAN_POINT('Ctrl Pts',(74.3558281540067,0.688351857913759,42.5800849504646));
#42894=CARTESIAN_POINT('Ctrl Pts',(75.3449429635535,3.26511784408383,42.4435220967921));
#42895=CARTESIAN_POINT('Ctrl Pts',(77.4309332243115,5.07250436977312,42.3069592431197));
#42896=CARTESIAN_POINT('Ctrl Pts',(80.1222635932022,5.68469848937892,42.1703963894473));
#42897=CARTESIAN_POINT('Ctrl Pts',(82.7848030002136,4.95731809286584,42.0338335357748));
#42898=CARTESIAN_POINT('Ctrl Pts',(84.7911111672477,3.06203906700717,41.8972706821024));
#42899=CARTESIAN_POINT('Ctrl Pts',(85.6685392121824,0.444861951915516,41.76070782843));
#42900=CARTESIAN_POINT('Ctrl Pts',(85.3627172389852,-1.36909553530131,41.6696659259817));
#42901=CARTESIAN_POINT('Ctrl Pts',(85.0052546189208,-2.18714454535403,41.6241449747575));
#42902=CARTESIAN_POINT('Ctrl Pts',(84.371668231913,3.79296281718951,54.3758550252424));
#42903=CARTESIAN_POINT('Ctrl Pts',(84.9915826446663,3.07846592508805,54.3303340740183));
#42904=CARTESIAN_POINT('Ctrl Pts',(85.8738080048016,1.34037186306025,54.23929217157));
#42905=CARTESIAN_POINT('Ctrl Pts',(85.812947989228,-1.58382949407201,54.1027293178976));
#42906=CARTESIAN_POINT('Ctrl Pts',(84.3823098860621,-4.13442322677981,53.9661664642251));
#42907=CARTESIAN_POINT('Ctrl Pts',(81.9190807910518,-5.71103446112322,53.8296036105527));
#42908=CARTESIAN_POINT('Ctrl Pts',(79.0036487908829,-5.94185892960139,53.6930407568803));
#42909=CARTESIAN_POINT('Ctrl Pts',(76.3229910273682,-4.77264832753163,53.5564779032079));
#42910=CARTESIAN_POINT('Ctrl Pts',(74.5087450641535,-2.47883725401571,53.4199150495354));
#42911=CARTESIAN_POINT('Ctrl Pts',(73.9884046182486,0.399052402667041,53.283352195863));
#42912=CARTESIAN_POINT('Ctrl Pts',(74.884576199613,3.18291797943272,53.1467893421906));
#42913=CARTESIAN_POINT('Ctrl Pts',(76.9860954894315,5.21679028750206,53.0102264885181));
#42914=CARTESIAN_POINT('Ctrl Pts',(79.7977811228463,6.02143111935951,52.8736636348457));
#42915=CARTESIAN_POINT('Ctrl Pts',(82.6571156419606,5.40724142315835,52.7371007811733));
#42916=CARTESIAN_POINT('Ctrl Pts',(84.8903538784323,3.51894344454454,52.6005379275008));
#42917=CARTESIAN_POINT('Ctrl Pts',(85.971277849858,0.801476579932164,52.4639750738284));
#42918=CARTESIAN_POINT('Ctrl Pts',(85.6451893846569,-2.10484219307877,52.3274122201559));
#42919=CARTESIAN_POINT('Ctrl Pts',(83.9889247271966,-4.51519694134435,52.1908493664836));
#42920=CARTESIAN_POINT('Ctrl Pts',(81.392749580059,-5.86163564779273,52.0542865128111));
#42921=CARTESIAN_POINT('Ctrl Pts',(78.4684007956417,-5.82689692354007,51.9177236591387));
#42922=CARTESIAN_POINT('Ctrl Pts',(75.9049427911273,-4.41916624807766,51.7811608054662));
#42923=CARTESIAN_POINT('Ctrl Pts',(74.3064032761888,-1.97014725873684,51.6445979517938));
#42924=CARTESIAN_POINT('Ctrl Pts',(74.0494461787839,0.943097606365279,51.5080350981214));
#42925=CARTESIAN_POINT('Ctrl Pts',(75.194618309843,3.63412034553672,51.371472244449));
#42926=CARTESIAN_POINT('Ctrl Pts',(77.4720827155306,5.46883516639296,51.2349093907765));
#42927=CARTESIAN_POINT('Ctrl Pts',(80.3452003693293,6.01492814413444,51.0983465371041));
#42928=CARTESIAN_POINT('Ctrl Pts',(83.1369784466681,5.14372336924537,50.9617836834317));
#42929=CARTESIAN_POINT('Ctrl Pts',(85.1895901705532,3.06050285669621,50.8252208297592));
#42930=CARTESIAN_POINT('Ctrl Pts',(86.0193785606126,0.256135936938712,50.6886579760868));
#42931=CARTESIAN_POINT('Ctrl Pts',(85.4308205462086,-2.60858430360903,50.5520951224144));
#42932=CARTESIAN_POINT('Ctrl Pts',(83.5625980751767,-4.85864372319071,50.415532268742));
#42933=CARTESIAN_POINT('Ctrl Pts',(80.854920481063,-5.96386073321759,50.2789694150695));
#42934=CARTESIAN_POINT('Ctrl Pts',(77.9457979407295,-5.6638130066099,50.1424065613971));
#42935=CARTESIAN_POINT('Ctrl Pts',(75.5207071115553,-4.02920080086409,50.0058437077247));
#42936=CARTESIAN_POINT('Ctrl Pts',(74.1510722399839,-1.44518785362601,49.8692808540522));
#42937=CARTESIAN_POINT('Ctrl Pts',(74.1596204440991,1.4793547637972,49.7327180003798));
#42938=CARTESIAN_POINT('Ctrl Pts',(75.5443375102325,4.05531696066211,49.5961551467073));
#42939=CARTESIAN_POINT('Ctrl Pts',(77.9789425022089,5.67572466428538,49.4595922930349));
#42940=CARTESIAN_POINT('Ctrl Pts',(80.8897693510335,5.95876114440882,49.3230294393625));
#42941=CARTESIAN_POINT('Ctrl Pts',(83.5909398130512,4.8377345042074,49.1864665856901));
#42942=CARTESIAN_POINT('Ctrl Pts',(85.4459769871887,2.57679229453327,49.0499037320176));
#42943=CARTESIAN_POINT('Ctrl Pts',(86.0177783919207,-0.29131958377009,48.9133408783452));
#42944=CARTESIAN_POINT('Ctrl Pts',(85.17161044,-3.09078781721385,48.7767780246728));
#42945=CARTESIAN_POINT('Ctrl Pts',(83.1068557188642,-5.16197359701852,48.6402151710003));
#42946=CARTESIAN_POINT('Ctrl Pts',(80.310032463798,-6.01684333729458,48.5036523173279));
#42947=CARTESIAN_POINT('Ctrl Pts',(77.4401562472232,-5.45396404787602,48.3670894636555));
#42948=CARTESIAN_POINT('Ctrl Pts',(75.173456113724,-3.60596699763133,48.2305266099831));
#42949=CARTESIAN_POINT('Ctrl Pts',(74.0440347039589,-0.908295803419074,
48.0939637563106));
#42950=CARTESIAN_POINT('Ctrl Pts',(74.318017628659,2.0033971662965,47.9574009026382));
#42951=CARTESIAN_POINT('Ctrl Pts',(75.930846280616,4.44302958376126,47.8208380489657));
#42952=CARTESIAN_POINT('Ctrl Pts',(78.5024897818106,5.83575076751681,47.6842751952933));
#42953=CARTESIAN_POINT('Ctrl Pts',(81.4269916739885,5.85339377084119,47.5477123416209));
#42954=CARTESIAN_POINT('Ctrl Pts',(84.0152514624972,4.49180137217451,47.4111494879485));
#42955=CARTESIAN_POINT('Ctrl Pts',(85.657397392656,2.07180564139699,47.274586634276));
#42956=CARTESIAN_POINT('Ctrl Pts',(85.966490555042,-0.83636973328118,47.1380237806036));
#42957=CARTESIAN_POINT('Ctrl Pts',(84.869699315775,-3.5474712751614,47.0014609269311));
#42958=CARTESIAN_POINT('Ctrl Pts',(82.6254606372418,-5.42268202243584,46.8648980732587));
#42959=CARTESIAN_POINT('Ctrl Pts',(79.7625845665931,-6.02014599375589,46.7283352195863));
#42960=CARTESIAN_POINT('Ctrl Pts',(76.9556507037564,-5.19908273031082,46.5917723659139));
#42961=CARTESIAN_POINT('Ctrl Pts',(74.8660569840556,-3.15295940081547,46.4552095122415));
#42962=CARTESIAN_POINT('Ctrl Pts',(73.9861744569741,-0.363904125017746,
46.318646658569));
#42963=CARTESIAN_POINT('Ctrl Pts',(74.5233298766064,2.51089789391818,46.1820838048966));
#42964=CARTESIAN_POINT('Ctrl Pts',(76.3509532905225,4.79405694440583,46.0455209512242));
#42965=CARTESIAN_POINT('Ctrl Pts',(79.0384017225848,5.94759217053654,45.9089580975517));
#42966=CARTESIAN_POINT('Ctrl Pts',(81.9524315941722,5.69969602209027,45.7723952438793));
#42967=CARTESIAN_POINT('Ctrl Pts',(84.4064099332516,4.10878027817237,45.6358323902068));
#42968=CARTESIAN_POINT('Ctrl Pts',(85.8221057282965,1.54971247742632,45.4992695365344));
#42969=CARTESIAN_POINT('Ctrl Pts',(85.8659385240322,-1.37451413467567,45.362706682862));
#42970=CARTESIAN_POINT('Ctrl Pts',(84.5275799970954,-3.97486392774426,45.2261438291896));
#42971=CARTESIAN_POINT('Ctrl Pts',(82.122387619263,-5.63861637883664,45.0895809755171));
#42972=CARTESIAN_POINT('Ctrl Pts',(79.2170969641224,-5.97374143319821,44.9530181218447));
#42973=CARTESIAN_POINT('Ctrl Pts',(76.4962817817787,-4.90127356115173,44.8164552681723));
#42974=CARTESIAN_POINT('Ctrl Pts',(74.6010478595557,-2.67391840928499,44.6798924144998));
#42975=CARTESIAN_POINT('Ctrl Pts',(73.9779692402184,0.183492241649758,44.5433295608274));
#42976=CARTESIAN_POINT('Ctrl Pts',(74.7738619632483,2.9976666080314,44.406766707155));
#42977=CARTESIAN_POINT('Ctrl Pts',(76.801189795003,5.10550067601197,44.2702038534825));
#42978=CARTESIAN_POINT('Ctrl Pts',(79.5822534003349,6.01032541870217,44.1336409998101));
#42979=CARTESIAN_POINT('Ctrl Pts',(82.4617506521313,5.49893695409371,43.9970781461377));
#42980=CARTESIAN_POINT('Ctrl Pts',(84.7611855042573,3.69183375038168,43.8605152924653));
#42981=CARTESIAN_POINT('Ctrl Pts',(85.9387420258757,1.01482363910322,43.7239524387928));
#42982=CARTESIAN_POINT('Ctrl Pts',(85.7169525432435,-1.90130945416647,43.5873895851204));
#42983=CARTESIAN_POINT('Ctrl Pts',(84.1480772882073,-4.36943682345102,43.450826731448));
#42984=CARTESIAN_POINT('Ctrl Pts',(81.6017904676673,-5.8079938444491,43.3142638777755));
#42985=CARTESIAN_POINT('Ctrl Pts',(78.6780735959123,-5.87801257950141,43.1777010241031));
#42986=CARTESIAN_POINT('Ctrl Pts',(76.0658425096326,-4.56299598535319,43.0411381704307));
#42987=CARTESIAN_POINT('Ctrl Pts',(74.3806166459536,-2.17279832801746,42.9045753167582));
#42988=CARTESIAN_POINT('Ctrl Pts',(74.0194872805808,0.729371315051554,42.7680124630858));
#42989=CARTESIAN_POINT('Ctrl Pts',(75.0675442605715,3.45968891978511,42.6314496094134));
#42990=CARTESIAN_POINT('Ctrl Pts',(77.2778404080753,5.37477910497586,42.4948867557409));
#42991=CARTESIAN_POINT('Ctrl Pts',(80.1295493819499,6.02345437903847,42.3583239020685));
#42992=CARTESIAN_POINT('Ctrl Pts',(82.9507517166893,5.25272878245856,42.2217610483961));
#42993=CARTESIAN_POINT('Ctrl Pts',(85.0766174485309,3.24450851024225,42.0851981947236));
#42994=CARTESIAN_POINT('Ctrl Pts',(86.0063321571346,0.471371643956068,41.9486353410512));
#42995=CARTESIAN_POINT('Ctrl Pts',(85.6822859993477,-1.45068107180012,41.8575934386029));
#42996=CARTESIAN_POINT('Ctrl Pts',(85.3035218857904,-2.31747829967006,41.8120724873788));
#42997=CARTESIAN_POINT('Ctrl Pts',(84.6175285419623,4.00627704067795,54.5637825378637));
#42998=CARTESIAN_POINT('Ctrl Pts',(85.2723066135383,3.25159722112125,54.5182615866395));
#42999=CARTESIAN_POINT('Ctrl Pts',(86.2041478614926,1.41575366798031,54.4272196841912));
#43000=CARTESIAN_POINT('Ctrl Pts',(86.13986511082,-1.67290322744343,54.2906568305188));
#43001=CARTESIAN_POINT('Ctrl Pts',(84.6287686771144,-4.36694100317251,54.1540939768463));
#43002=CARTESIAN_POINT('Ctrl Pts',(82.0270088801171,-6.03222001977652,54.0175311231739));
#43003=CARTESIAN_POINT('Ctrl Pts',(78.9476145256559,-6.27602593432435,53.8809682695015));
#43004=CARTESIAN_POINT('Ctrl Pts',(76.1161979867926,-5.04105954615917,53.7444054158291));
#43005=CARTESIAN_POINT('Ctrl Pts',(74.1999197898036,-2.6182457506132,53.6078425621567));
#43006=CARTESIAN_POINT('Ctrl Pts',(73.6503156723266,0.421494898812886,53.4712797084842));
#43007=CARTESIAN_POINT('Ctrl Pts',(74.5968874696183,3.36192360377817,53.3347168548118));
#43008=CARTESIAN_POINT('Ctrl Pts',(76.8165950932171,5.51017981513921,53.1981540011394));
#43009=CARTESIAN_POINT('Ctrl Pts',(79.7864084401088,6.36007322196442,53.0615911474669));
#43010=CARTESIAN_POINT('Ctrl Pts',(82.8065504208398,5.71134182197275,52.9250282937945));
#43011=CARTESIAN_POINT('Ctrl Pts',(85.1653847950113,3.71684696339025,52.7884654401221));
#43012=CARTESIAN_POINT('Ctrl Pts',(86.3070993591023,0.846551199044585,52.6519025864497));
#43013=CARTESIAN_POINT('Ctrl Pts',(85.9626718510223,-2.22321740518142,52.5153397327772));
#43014=CARTESIAN_POINT('Ctrl Pts',(84.2132597448983,-4.769129230128,52.3787768791048));
#43015=CARTESIAN_POINT('Ctrl Pts',(81.4710770800909,-6.19129093756104,52.2422140254323));
#43016=CARTESIAN_POINT('Ctrl Pts',(78.3822644661494,-6.15459852582288,52.1056511717599));
#43017=CARTESIAN_POINT('Ctrl Pts',(75.6746389387688,-4.66769782144369,51.9690883180875));
#43018=CARTESIAN_POINT('Ctrl Pts',(73.9861984066626,-2.0809472989457,51.832525464415));
#43019=CARTESIAN_POINT('Ctrl Pts',(73.7147901779535,0.996136917128858,51.6959626107427));
#43020=CARTESIAN_POINT('Ctrl Pts',(74.9243661842076,3.83850135239988,51.5593997570702));
#43021=CARTESIAN_POINT('Ctrl Pts',(77.3299139839692,5.77639956476208,51.4228369033978));
#43022=CARTESIAN_POINT('Ctrl Pts',(80.3646142555919,6.35320452285083,51.2862740497253));
#43023=CARTESIAN_POINT('Ctrl Pts',(83.3134004559793,5.43300365203046,51.1497111960529));
#43024=CARTESIAN_POINT('Ctrl Pts',(85.481449977994,3.23262391926018,51.0131483423805));
#43025=CARTESIAN_POINT('Ctrl Pts',(86.3579052283988,0.270540886612342,50.8765854887081));
#43026=CARTESIAN_POINT('Ctrl Pts',(85.736247022437,-2.75528970567801,50.7400226350356));
#43027=CARTESIAN_POINT('Ctrl Pts',(83.7629567073689,-5.13189127740411,50.6034597813632));
#43028=CARTESIAN_POINT('Ctrl Pts',(80.903000756919,-6.2992651077435,50.4668969276907));
#43029=CARTESIAN_POINT('Ctrl Pts',(77.8302707029787,-5.98234285562748,50.3303340740183));
#43030=CARTESIAN_POINT('Ctrl Pts',(75.2687940477242,-4.25580092365468,50.1937712203459));
#43031=CARTESIAN_POINT('Ctrl Pts',(73.8221316351055,-1.52646445443898,50.0572083666734));
#43032=CARTESIAN_POINT('Ctrl Pts',(73.8311605857006,1.56255289357405,49.920645513001));
#43033=CARTESIAN_POINT('Ctrl Pts',(75.2937534075295,4.28338584247207,49.7840826593286));
#43034=CARTESIAN_POINT('Ctrl Pts',(77.8652792970721,5.99492441863291,49.6475198056562));
#43035=CARTESIAN_POINT('Ctrl Pts',(80.939809508912,6.2938787207563,49.5109569519837));
#43036=CARTESIAN_POINT('Ctrl Pts',(83.792892369597,5.10980613499994,49.3743940983113));
#43037=CARTESIAN_POINT('Ctrl Pts',(85.7522558536446,2.72170973082036,49.2378312446388));
#43038=CARTESIAN_POINT('Ctrl Pts',(86.3562150670656,-0.307703243139823,
49.1012683909664));
#43039=CARTESIAN_POINT('Ctrl Pts',(85.4624590769004,-3.26461208994559,48.964705537294));
#43040=CARTESIAN_POINT('Ctrl Pts',(83.2815836418895,-5.45228026296463,48.8281426836216));
#43041=CARTESIAN_POINT('Ctrl Pts',(80.3274685256469,-6.35522742546172,48.6915798299491));
#43042=CARTESIAN_POINT('Ctrl Pts',(77.2961919879637,-5.76069210240215,48.5550169762767));
#43043=CARTESIAN_POINT('Ctrl Pts',(74.9020138373674,-3.80876467509304,48.4184541226043));
#43044=CARTESIAN_POINT('Ctrl Pts',(73.7090743646455,-0.959377879184771,
48.2818912689318));
#43045=CARTESIAN_POINT('Ctrl Pts',(73.9984659441751,2.1160671637272,48.1453284152594));
#43046=CARTESIAN_POINT('Ctrl Pts',(75.701999226811,4.69290321850953,48.008765561587));
#43047=CARTESIAN_POINT('Ctrl Pts',(78.4182705988775,6.16395030530382,47.8722027079146));
#43048=CARTESIAN_POINT('Ctrl Pts',(81.507244931279,6.18258554180725,47.7356398542421));
#43049=CARTESIAN_POINT('Ctrl Pts',(84.2410670818731,4.74441790651735,47.5990770005697));
#43050=CARTESIAN_POINT('Ctrl Pts',(85.9755664309368,2.18832289529958,47.4625141468972));
#43051=CARTESIAN_POINT('Ctrl Pts',(86.3020428293569,-0.88340672488984,47.3259512932248));
#43052=CARTESIAN_POINT('Ctrl Pts',(85.1435686306702,-3.74697918411825,47.1893884395524));
#43053=CARTESIAN_POINT('Ctrl Pts',(82.7731151553917,-5.72765079239012,47.05282558588));
#43054=CARTESIAN_POINT('Ctrl Pts',(79.7492324481405,-6.35871582157629,46.9162627322075));
#43055=CARTESIAN_POINT('Ctrl Pts',(76.7844381088919,-5.49147639429357,46.7796998785351));
#43056=CARTESIAN_POINT('Ctrl Pts',(74.5773267431693,-3.33028017053867,46.6431370248627));
#43057=CARTESIAN_POINT('Ctrl Pts',(73.6479600879612,-0.384369900611591,
46.5065741711902));
#43058=CARTESIAN_POINT('Ctrl Pts',(74.2153248443979,2.65210946395323,46.3700113175178));
#43059=CARTESIAN_POINT('Ctrl Pts',(76.1457328328429,5.06367217232759,46.2334484638453));
#43060=CARTESIAN_POINT('Ctrl Pts',(78.9843219438627,6.2820816096985,46.0968856101729));
#43061=CARTESIAN_POINT('Ctrl Pts',(82.0622353147722,6.02024391292702,45.9603227565005));
#43062=CARTESIAN_POINT('Ctrl Pts',(84.6542240982161,4.33985590869289,45.8237599028281));
#43063=CARTESIAN_POINT('Ctrl Pts',(86.149537876292,1.63686748781935,45.6871970491556));
#43064=CARTESIAN_POINT('Ctrl Pts',(86.1958358052853,-1.45181608290028,45.5506341954832));
#43065=CARTESIAN_POINT('Ctrl Pts',(84.7822087023876,-4.19840817351866,45.4140713418108));
#43066=CARTESIAN_POINT('Ctrl Pts',(82.2417495768579,-5.95572918282979,45.2775084881383));
#43067=CARTESIAN_POINT('Ctrl Pts',(79.1730669113078,-6.30970149306707,45.140945634466));
#43068=CARTESIAN_POINT('Ctrl Pts',(76.2992345216118,-5.17691859491353,45.0043827807935));
#43069=CARTESIAN_POINT('Ctrl Pts',(74.2974136456185,-2.82429816691486,44.867819927121));
#43070=CARTESIAN_POINT('Ctrl Pts',(73.6392934141531,0.193811748307269,44.7312570734486));
#43071=CARTESIAN_POINT('Ctrl Pts',(74.4799467231356,3.16625379319216,44.5946942197762));
#43072=CARTESIAN_POINT('Ctrl Pts',(76.621290400294,5.39263133473806,44.4581313661038));
#43073=CARTESIAN_POINT('Ctrl Pts',(79.5587595524336,6.34834294257372,44.3215685124313));
#43074=CARTESIAN_POINT('Ctrl Pts',(82.6001982072725,5.80819426108823,44.1850056587589));
#43075=CARTESIAN_POINT('Ctrl Pts',(85.0289520597644,3.89946052862007,44.0484428050865));
#43076=CARTESIAN_POINT('Ctrl Pts',(86.272733737581,1.07189678402622,43.911879951414));
#43077=CARTESIAN_POINT('Ctrl Pts',(86.0384709317063,-2.00823809264104,43.7753170977416));
#43078=CARTESIAN_POINT('Ctrl Pts',(84.3813629617958,-4.61517164026814,43.6387542440692));
#43079=CARTESIAN_POINT('Ctrl Pts',(81.6918743166977,-6.13463234755794,43.5021913903967));
#43080=CARTESIAN_POINT('Ctrl Pts',(78.6037291538527,-6.20858889925048,43.3656285367243));
#43081=CARTESIAN_POINT('Ctrl Pts',(75.8445875723747,-4.81961646710041,43.2290656830519));
#43082=CARTESIAN_POINT('Ctrl Pts',(74.0645854971062,-2.29499535722046,43.0925028293794));
#43083=CARTESIAN_POINT('Ctrl Pts',(73.6831464071548,0.770390772189351,42.955939975707));
#43084=CARTESIAN_POINT('Ctrl Pts',(74.7901455575896,3.65425999548639,42.8193771220346));
#43085=CARTESIAN_POINT('Ctrl Pts',(77.1247475918389,5.6770538401786,42.6828142683621));
#43086=CARTESIAN_POINT('Ctrl Pts',(80.1368351706977,6.36221026869802,42.5462514146897));
#43087=CARTESIAN_POINT('Ctrl Pts',(83.1167004331651,5.54813947205128,42.4096885610173));
#43088=CARTESIAN_POINT('Ctrl Pts',(85.3621237298141,3.42697795347734,42.2731257073449));
#43089=CARTESIAN_POINT('Ctrl Pts',(86.3441251020869,0.497881335996617,42.1365628536724));
#43090=CARTESIAN_POINT('Ctrl Pts',(86.0018547597101,-1.53226660829892,42.0455209512241));
#43091=CARTESIAN_POINT('Ctrl Pts',(85.6017891526601,-2.4478120539861,42.));
#43092=CARTESIAN_POINT('Ctrl Pts',(85.6017891526601,-2.4478120539861,42.));
#43093=CARTESIAN_POINT('Ctrl Pts',(85.6569254810043,-2.28851462898893,42.));
#43094=CARTESIAN_POINT('Ctrl Pts',(85.705210066224,-2.12723744746175,42.));
#43095=CARTESIAN_POINT('Ctrl Pts',(85.7466571421988,-1.96442654482131,42.));
#43096=CARTESIAN_POINT('Ctrl Pts',(85.788432837758,-1.80032477063183,42.));
#43097=CARTESIAN_POINT('Ctrl Pts',(85.8232622239843,-1.63466409832166,42.));
#43098=CARTESIAN_POINT('Ctrl Pts',(85.851107925251,-1.46789149284502,42.));
#43099=CARTESIAN_POINT('Ctrl Pts',(85.8787722019253,-1.30220546987841,42.));
#43100=CARTESIAN_POINT('Ctrl Pts',(85.8995434395036,-1.13542121242627,42.));
#43101=CARTESIAN_POINT('Ctrl Pts',(85.9133341464194,-0.967978688103236,
42.));
#43102=CARTESIAN_POINT('Ctrl Pts',(85.926960703886,-0.80252921593562,42.));
#43103=CARTESIAN_POINT('Ctrl Pts',(85.9337718247844,-0.636436380822634,
42.));
#43104=CARTESIAN_POINT('Ctrl Pts',(85.9336345128749,-0.470136750206304,
42.));
#43105=CARTESIAN_POINT('Ctrl Pts',(85.9335702448832,-0.392301234639418,
42.));
#43106=CARTESIAN_POINT('Ctrl Pts',(85.9319831293793,-0.314420653493014,
42.));
#43107=CARTESIAN_POINT('Ctrl Pts',(85.9288558891231,-0.236541327327588,
42.));
#43108=CARTESIAN_POINT('Ctrl Pts',(85.9277529940179,-0.209075344356874,
42.));
#43109=CARTESIAN_POINT('Ctrl Pts',(85.9264585191432,-0.181609528300492,
42.));
#43110=CARTESIAN_POINT('Ctrl Pts',(85.9249716376403,-0.154145948317355,
42.));
#43111=CARTESIAN_POINT('Ctrl Pts',(85.9237407875316,-0.131411419477627,
42.));
#43112=CARTESIAN_POINT('Ctrl Pts',(85.922378510943,-0.108686724224631,42.));
#43113=CARTESIAN_POINT('Ctrl Pts',(85.9208851246716,-0.0859796899287691,
42.));
#43114=CARTESIAN_POINT('Ctrl Pts',(85.9100466443096,0.0788201009962529,
42.));
#43115=CARTESIAN_POINT('Ctrl Pts',(85.892300375058,0.242802290608795,42.));
#43116=CARTESIAN_POINT('Ctrl Pts',(85.8675999298121,0.405551851065137,42.));
#43117=CARTESIAN_POINT('Ctrl Pts',(85.8648424370719,0.423720783931401,42.));
#43118=CARTESIAN_POINT('Ctrl Pts',(85.8619982222532,0.441874346367681,42.));
#43119=CARTESIAN_POINT('Ctrl Pts',(85.8590671810102,0.46001195351897,42.));
#43120=CARTESIAN_POINT('Ctrl Pts',(85.8327238923556,0.623027135182727,42.));
#43121=CARTESIAN_POINT('Ctrl Pts',(85.7993709501763,0.784754959977138,42.));
#43122=CARTESIAN_POINT('Ctrl Pts',(85.7591902245475,0.944778915634052,42.));
#43123=CARTESIAN_POINT('Ctrl Pts',(85.7190590371889,1.10460557993238,42.));
#43124=CARTESIAN_POINT('Ctrl Pts',(85.6721165102442,1.26273325668429,42.));
#43125=CARTESIAN_POINT('Ctrl Pts',(85.6184980647307,1.4187228208717,42.));
#43126=CARTESIAN_POINT('Ctrl Pts',(85.5685831655387,1.56393783590737,42.));
#43127=CARTESIAN_POINT('Ctrl Pts',(85.5128820688434,1.70730010798767,42.));
#43128=CARTESIAN_POINT('Ctrl Pts',(85.451472575904,1.84842874304492,42.));
#43129=CARTESIAN_POINT('Ctrl Pts',(85.4364074129714,1.88305084754089,42.));
#43130=CARTESIAN_POINT('Ctrl Pts',(85.4209985669166,1.91753838332473,42.));
#43131=CARTESIAN_POINT('Ctrl Pts',(85.4052469350423,1.95188543849552,42.));
#43132=CARTESIAN_POINT('Ctrl Pts',(85.3941405753051,1.97610329437745,42.));
#43133=CARTESIAN_POINT('Ctrl Pts',(85.3828637956616,2.00025130705317,42.));
#43134=CARTESIAN_POINT('Ctrl Pts',(85.3714168828596,2.02432736674011,42.));
#43135=CARTESIAN_POINT('Ctrl Pts',(85.3626888510097,2.04268485922774,42.));
#43136=CARTESIAN_POINT('Ctrl Pts',(85.3538640990633,2.06099584588555,42.));
#43137=CARTESIAN_POINT('Ctrl Pts',(85.3449464057949,2.07925244694918,42.));
#43138=CARTESIAN_POINT('Ctrl Pts',(85.2740289091692,2.2244371270408,42.));
#43139=CARTESIAN_POINT('Ctrl Pts',(85.1971721039349,2.3663221572068,42.));
#43140=CARTESIAN_POINT('Ctrl Pts',(85.1145485353578,2.50451868546955,42.));
#43141=CARTESIAN_POINT('Ctrl Pts',(85.0325534073232,2.64166408143795,42.));
#43142=CARTESIAN_POINT('Ctrl Pts',(84.9448784824779,2.77517746393529,42.));
#43143=CARTESIAN_POINT('Ctrl Pts',(84.8516514430892,2.90464835133629,42.));
#43144=CARTESIAN_POINT('Ctrl Pts',(84.8193995921606,2.94943874463242,42.));
#43145=CARTESIAN_POINT('Ctrl Pts',(84.7864829254346,2.99374501823486,42.));
#43146=CARTESIAN_POINT('Ctrl Pts',(84.752905714703,3.03754912324718,42.));
#43147=CARTESIAN_POINT('Ctrl Pts',(84.65510697225,3.16513525357588,42.));
#43148=CARTESIAN_POINT('Ctrl Pts',(84.5517063684955,3.28846448836943,42.));
#43149=CARTESIAN_POINT('Ctrl Pts',(84.4430292319423,3.40721711979787,42.));
#43150=CARTESIAN_POINT('Ctrl Pts',(84.3801478011414,3.47592830977242,42.));
#43151=CARTESIAN_POINT('Ctrl Pts',(84.3154993362663,3.54310650462682,42.));
#43152=CARTESIAN_POINT('Ctrl Pts',(84.2491434596823,3.60868251821583,42.));
#43153=CARTESIAN_POINT('Ctrl Pts',(84.2089699962351,3.64838383361632,42.));
#43154=CARTESIAN_POINT('Ctrl Pts',(84.1681706577425,3.68749778106476,42.));
#43155=CARTESIAN_POINT('Ctrl Pts',(84.1267583557391,3.726007975968,42.));
#43156=CARTESIAN_POINT('Ctrl Pts',(84.1075910362983,3.74383208068396,42.));
#43157=CARTESIAN_POINT('Ctrl Pts',(84.088292403684,3.76152683711411,42.));
#43158=CARTESIAN_POINT('Ctrl Pts',(84.0688637244686,3.77909056167488,42.));
#43159=CARTESIAN_POINT('Ctrl Pts',(84.0541228012848,3.79241650687679,42.));
#43160=CARTESIAN_POINT('Ctrl Pts',(84.0393144271957,3.80566031870826,42.));
#43161=CARTESIAN_POINT('Ctrl Pts',(84.0244399044793,3.81882101986992,42.));
#43162=CARTESIAN_POINT('Ctrl Pts',(83.9064001150324,3.92326043105106,42.));
#43163=CARTESIAN_POINT('Ctrl Pts',(83.7841852346065,4.02248016159722,42.));
#43164=CARTESIAN_POINT('Ctrl Pts',(83.6581398297667,4.1162287172709,42.));
#43165=CARTESIAN_POINT('Ctrl Pts',(83.5324837634402,4.20968769536464,42.));
#43166=CARTESIAN_POINT('Ctrl Pts',(83.4030201308865,4.2977096203736,42.));
#43167=CARTESIAN_POINT('Ctrl Pts',(83.2700643854091,4.38000074382011,42.));
#43168=CARTESIAN_POINT('Ctrl Pts',(83.1392403663464,4.46097246462693,42.));
#43169=CARTESIAN_POINT('Ctrl Pts',(83.0050346764522,4.53639592031169,42.));
#43170=CARTESIAN_POINT('Ctrl Pts',(82.8677324475143,4.60594364255217,42.));
#43171=CARTESIAN_POINT('Ctrl Pts',(82.7949213954891,4.64282463757642,42.));
#43172=CARTESIAN_POINT('Ctrl Pts',(82.721239345296,4.67805245546147,42.));
#43173=CARTESIAN_POINT('Ctrl Pts',(82.6467279335914,4.71157233605123,42.));
#43174=CARTESIAN_POINT('Ctrl Pts',(82.5480059693877,4.75598363327391,42.));
#43175=CARTESIAN_POINT('Ctrl Pts',(82.4478279782409,4.79739714128736,42.));
#43176=CARTESIAN_POINT('Ctrl Pts',(82.3463374882128,4.83575688226234,42.));
#43177=CARTESIAN_POINT('Ctrl Pts',(82.3210480836265,4.84531536413657,42.));
#43178=CARTESIAN_POINT('Ctrl Pts',(82.2956771925386,4.85468417743707,42.));
#43179=CARTESIAN_POINT('Ctrl Pts',(82.2702270542163,4.86386234007145,42.));
#43180=CARTESIAN_POINT('Ctrl Pts',(82.2479671578636,4.87188999581004,42.));
#43181=CARTESIAN_POINT('Ctrl Pts',(82.2256545985108,4.87976890597722,42.));
#43182=CARTESIAN_POINT('Ctrl Pts',(82.2032959008903,4.88749708030084,42.));
#43183=CARTESIAN_POINT('Ctrl Pts',(82.0573143762485,4.93795487930184,42.));
#43184=CARTESIAN_POINT('Ctrl Pts',(81.9092993450614,4.98201550564599,42.));
#43185=CARTESIAN_POINT('Ctrl Pts',(81.7596854975444,5.01959244081141,42.));
#43186=CARTESIAN_POINT('Ctrl Pts',(81.6253698886421,5.05332707842144,42.));
#43187=CARTESIAN_POINT('Ctrl Pts',(81.4897651591011,5.08183552641375,42.));
#43188=CARTESIAN_POINT('Ctrl Pts',(81.3531856950333,5.10501933912427,42.));
#43189=CARTESIAN_POINT('Ctrl Pts',(81.2870765067884,5.11624110697331,42.));
#43190=CARTESIAN_POINT('Ctrl Pts',(81.2207389937343,5.12621485843111,42.));
#43191=CARTESIAN_POINT('Ctrl Pts',(81.154209309988,5.13492653924264,42.));
#43192=CARTESIAN_POINT('Ctrl Pts',(81.1165245578612,5.13986114156606,42.));
#43193=CARTESIAN_POINT('Ctrl Pts',(81.0787781560059,5.14439077566049,42.));
#43194=CARTESIAN_POINT('Ctrl Pts',(81.0409767524365,5.14851261661839,42.));
#43195=CARTESIAN_POINT('Ctrl Pts',(81.0182097045005,5.15099512101801,42.));
#43196=CARTESIAN_POINT('Ctrl Pts',(80.995425948708,5.15332930886033,42.));
#43197=CARTESIAN_POINT('Ctrl Pts',(80.9726350572463,5.15551398645696,42.));
#43198=CARTESIAN_POINT('Ctrl Pts',(80.8229478859385,5.16986262263071,42.));
#43199=CARTESIAN_POINT('Ctrl Pts',(80.6728487059268,5.17777748899213,42.));
#43200=CARTESIAN_POINT('Ctrl Pts',(80.5227445915659,5.17914634612362,42.));
#43201=CARTESIAN_POINT('Ctrl Pts',(80.385433598572,5.18039853786262,42.));
#43202=CARTESIAN_POINT('Ctrl Pts',(80.2481180770058,5.17617242893916,42.));
#43203=CARTESIAN_POINT('Ctrl Pts',(80.111118248695,5.16634484417903,42.));
#43204=CARTESIAN_POINT('Ctrl Pts',(80.0029202747275,5.15858333985344,42.));
#43205=CARTESIAN_POINT('Ctrl Pts',(79.894919291723,5.14732714412843,42.));
#43206=CARTESIAN_POINT('Ctrl Pts',(79.7872818445162,5.13260507264869,42.));
#43207=CARTESIAN_POINT('Ctrl Pts',(83.8799476118145,3.36633437021264,54.));
#43208=CARTESIAN_POINT('Ctrl Pts',(83.9867208778113,3.26433819512922,54.));
#43209=CARTESIAN_POINT('Ctrl Pts',(84.0887720625524,3.15785064545971,54.));
#43210=CARTESIAN_POINT('Ctrl Pts',(84.1859774524887,3.04731119162579,54.));
#43211=CARTESIAN_POINT('Ctrl Pts',(84.2849060809427,2.93481211554574,54.));
#43212=CARTESIAN_POINT('Ctrl Pts',(84.3788160767822,2.81811580143815,54.));
#43213=CARTESIAN_POINT('Ctrl Pts',(84.4675539561856,2.69763654749194,54.));
#43214=CARTESIAN_POINT('Ctrl Pts',(84.5575854668602,2.57540093277315,54.));
#43215=CARTESIAN_POINT('Ctrl Pts',(84.6422935095527,2.44927079503114,54.));
#43216=CARTESIAN_POINT('Ctrl Pts',(84.7214863046654,2.31963561596069,54.));
#43217=CARTESIAN_POINT('Ctrl Pts',(84.8005661343855,2.19018535635012,54.));
#43218=CARTESIAN_POINT('Ctrl Pts',(84.8741469255614,2.0572394347727,54.));
#43219=CARTESIAN_POINT('Ctrl Pts',(84.9419988953608,1.92115133237301,54.));
#43220=CARTESIAN_POINT('Ctrl Pts',(84.9589203834966,1.88721255038936,54.));
#43221=CARTESIAN_POINT('Ctrl Pts',(84.9754853611401,1.85307820023649,54.));
#43222=CARTESIAN_POINT('Ctrl Pts',(84.991689831896,1.81875350067991,54.));
#43223=CARTESIAN_POINT('Ctrl Pts',(85.0049215662956,1.79072572274637,54.));
#43224=CARTESIAN_POINT('Ctrl Pts',(85.0179129290737,1.76257102716215,54.));
#43225=CARTESIAN_POINT('Ctrl Pts',(85.0306616523005,1.73429221126858,54.));
#43226=CARTESIAN_POINT('Ctrl Pts',(85.0386661539721,1.71653687804293,54.));
#43227=CARTESIAN_POINT('Ctrl Pts',(85.0465747847197,1.69873297209936,54.));
#43228=CARTESIAN_POINT('Ctrl Pts',(85.0543816393726,1.68089376031065,54.));
#43229=CARTESIAN_POINT('Ctrl Pts',(85.116794780348,1.53827534485887,54.));
#43230=CARTESIAN_POINT('Ctrl Pts',(85.1727981491917,1.39320033760763,54.));
#43231=CARTESIAN_POINT('Ctrl Pts',(85.2222276344322,1.24609759053344,54.));
#43232=CARTESIAN_POINT('Ctrl Pts',(85.2279053057752,1.22920077181355,54.));
#43233=CARTESIAN_POINT('Ctrl Pts',(85.2334962056225,1.21227715721916,54.));
#43234=CARTESIAN_POINT('Ctrl Pts',(85.239000055387,1.19532736479374,54.));
#43235=CARTESIAN_POINT('Ctrl Pts',(85.2863939183891,1.04937204724304,54.));
#43236=CARTESIAN_POINT('Ctrl Pts',(85.3273366473861,0.901478132634383,54.));
#43237=CARTESIAN_POINT('Ctrl Pts',(85.361892379472,0.75208834072346,54.));
#43238=CARTESIAN_POINT('Ctrl Pts',(85.3968699097081,0.600875049958123,54.));
#43239=CARTESIAN_POINT('Ctrl Pts',(85.4253037941124,0.448128478050284,54.));
#43240=CARTESIAN_POINT('Ctrl Pts',(85.4472134338793,0.294282568467623,54.));
#43241=CARTESIAN_POINT('Ctrl Pts',(85.4680624160397,0.147884423247048,54.));
#43242=CARTESIAN_POINT('Ctrl Pts',(85.4830033161768,0.000490076344759782,
54.));
#43243=CARTESIAN_POINT('Ctrl Pts',(85.4920112832216,-0.147538780000658,
54.));
#43244=CARTESIAN_POINT('Ctrl Pts',(85.494164608261,-0.182924593618131,54.));
#43245=CARTESIAN_POINT('Ctrl Pts',(85.4959787192161,-0.218346695891146,
54.));
#43246=CARTESIAN_POINT('Ctrl Pts',(85.4974529220841,-0.25380018882677,54.));
#43247=CARTESIAN_POINT('Ctrl Pts',(85.4983096377735,-0.27440357001597,54.));
#43248=CARTESIAN_POINT('Ctrl Pts',(85.4990515565517,-0.29501755266055,54.));
#43249=CARTESIAN_POINT('Ctrl Pts',(85.4996785205849,-0.315641176049658,
54.));
#43250=CARTESIAN_POINT('Ctrl Pts',(85.5002766428774,-0.335316066873864,
54.));
#43251=CARTESIAN_POINT('Ctrl Pts',(85.5007698615858,-0.354990703538879,
54.));
#43252=CARTESIAN_POINT('Ctrl Pts',(85.5011582956561,-0.374662168734253,
54.));
#43253=CARTESIAN_POINT('Ctrl Pts',(85.5042977154338,-0.533651792992443,
54.));
#43254=CARTESIAN_POINT('Ctrl Pts',(85.5005974827858,-0.692475378903122,
54.));
#43255=CARTESIAN_POINT('Ctrl Pts',(85.4901267378284,-0.850671112988953,
54.));
#43256=CARTESIAN_POINT('Ctrl Pts',(85.4795441308475,-1.01055689825874,54.));
#43257=CARTESIAN_POINT('Ctrl Pts',(85.4620457764301,-1.1698020853449,54.));
#43258=CARTESIAN_POINT('Ctrl Pts',(85.4376534301819,-1.32794813514256,54.));
#43259=CARTESIAN_POINT('Ctrl Pts',(85.4300871316483,-1.37700369595264,54.));
#43260=CARTESIAN_POINT('Ctrl Pts',(85.4218571333759,-1.42595358576316,54.));
#43261=CARTESIAN_POINT('Ctrl Pts',(85.4129630820678,-1.4747842949477,54.));
#43262=CARTESIAN_POINT('Ctrl Pts',(85.3844600874515,-1.63127332258914,54.));
#43263=CARTESIAN_POINT('Ctrl Pts',(85.3491410875078,-1.78653855181248,54.));
#43264=CARTESIAN_POINT('Ctrl Pts',(85.3072293605156,-1.9402107254356,54.));
#43265=CARTESIAN_POINT('Ctrl Pts',(85.2815881273281,-2.03422603621094,54.));
#43266=CARTESIAN_POINT('Ctrl Pts',(85.2534782669258,-2.12764507941347,54.));
#43267=CARTESIAN_POINT('Ctrl Pts',(85.2229414321389,-2.2203819677405,54.));
#43268=CARTESIAN_POINT('Ctrl Pts',(85.2062836803499,-2.27096966218257,54.));
#43269=CARTESIAN_POINT('Ctrl Pts',(85.1889036183782,-2.32135434404811,54.));
#43270=CARTESIAN_POINT('Ctrl Pts',(85.1708071415319,-2.37152182596523,54.));
#43271=CARTESIAN_POINT('Ctrl Pts',(85.1621804631312,-2.3954369082408,54.));
#43272=CARTESIAN_POINT('Ctrl Pts',(85.1533909724132,-2.41930262938926,54.));
#43273=CARTESIAN_POINT('Ctrl Pts',(85.144439260286,-2.44311743472982,54.));
#43274=CARTESIAN_POINT('Ctrl Pts',(85.1369936391982,-2.46292549092338,54.));
#43275=CARTESIAN_POINT('Ctrl Pts',(85.1294387812218,-2.48269031816802,54.));
#43276=CARTESIAN_POINT('Ctrl Pts',(85.121776982974,-2.50240686339091,54.));
#43277=CARTESIAN_POINT('Ctrl Pts',(85.0627970435496,-2.65418332699488,54.));
#43278=CARTESIAN_POINT('Ctrl Pts',(84.9974542852625,-2.80317877950254,54.));
#43279=CARTESIAN_POINT('Ctrl Pts',(84.9260417665538,-2.94901892145395,54.));
#43280=CARTESIAN_POINT('Ctrl Pts',(84.8539555738348,-3.09623485458405,54.));
#43281=CARTESIAN_POINT('Ctrl Pts',(84.7756843890024,-3.24023637487642,54.));
#43282=CARTESIAN_POINT('Ctrl Pts',(84.6914762047118,-3.38063566136618,54.));
#43283=CARTESIAN_POINT('Ctrl Pts',(84.6071559667504,-3.52122177358501,54.));
#43284=CARTESIAN_POINT('Ctrl Pts',(84.5168826728383,-3.65819679106705,54.));
#43285=CARTESIAN_POINT('Ctrl Pts',(84.4208552373469,-3.79115765968197,54.));
#43286=CARTESIAN_POINT('Ctrl Pts',(84.3666732455324,-3.86617876857727,54.));
#43287=CARTESIAN_POINT('Ctrl Pts',(84.3106584773921,-3.93992162294824,54.));
#43288=CARTESIAN_POINT('Ctrl Pts',(84.2528400935798,-4.01231054808743,54.));
#43289=CARTESIAN_POINT('Ctrl Pts',(84.1767127434739,-4.10762239675047,54.));
#43290=CARTESIAN_POINT('Ctrl Pts',(84.0974590287316,-4.2005874878607,54.));
#43291=CARTESIAN_POINT('Ctrl Pts',(84.0152183541386,-4.29110409180728,54.));
#43292=CARTESIAN_POINT('Ctrl Pts',(83.9998522812934,-4.30801646195529,54.));
#43293=CARTESIAN_POINT('Ctrl Pts',(83.9843818987029,-4.32484332582238,54.));
#43294=CARTESIAN_POINT('Ctrl Pts',(83.9688080694945,-4.34158397855754,54.));
#43295=CARTESIAN_POINT('Ctrl Pts',(83.9526295296066,-4.35897464814822,54.));
#43296=CARTESIAN_POINT('Ctrl Pts',(83.9363458803576,-4.37626524708654,54.));
#43297=CARTESIAN_POINT('Ctrl Pts',(83.9199606112101,-4.39345287359883,54.));
#43298=CARTESIAN_POINT('Ctrl Pts',(83.8056108457966,-4.51340214278705,54.));
#43299=CARTESIAN_POINT('Ctrl Pts',(83.686281282956,-4.62837513484254,54.));
#43300=CARTESIAN_POINT('Ctrl Pts',(83.5623913145015,-4.73816763663545,54.));
#43301=CARTESIAN_POINT('Ctrl Pts',(83.4420179244782,-4.8448437122275,54.));
#43302=CARTESIAN_POINT('Ctrl Pts',(83.3173386901459,-4.94662952648338,54.));
#43303=CARTESIAN_POINT('Ctrl Pts',(83.1886992789893,-5.0433133030905,54.));
#43304=CARTESIAN_POINT('Ctrl Pts',(83.1301826943935,-5.08729363805938,54.));
#43305=CARTESIAN_POINT('Ctrl Pts',(83.0708461719817,-5.13021787326625,54.));
#43306=CARTESIAN_POINT('Ctrl Pts',(83.0107200033352,-5.17206406404072,54.));
#43307=CARTESIAN_POINT('Ctrl Pts',(82.9801270201334,-5.19335595474724,54.));
#43308=CARTESIAN_POINT('Ctrl Pts',(82.9493295839171,-5.2143687281097,54.));
#43309=CARTESIAN_POINT('Ctrl Pts',(82.9183315612049,-5.23509935358629,54.));
#43310=CARTESIAN_POINT('Ctrl Pts',(82.889668794743,-5.25426822387709,54.));
#43311=CARTESIAN_POINT('Ctrl Pts',(82.8608313052831,-5.27319782388591,54.));
#43312=CARTESIAN_POINT('Ctrl Pts',(82.8318448455755,-5.29187134074881,54.));
#43313=CARTESIAN_POINT('Ctrl Pts',(82.6883558129876,-5.38430915125419,54.));
#43314=CARTESIAN_POINT('Ctrl Pts',(82.5411173174573,-5.47054475376944,54.));
#43315=CARTESIAN_POINT('Ctrl Pts',(82.39054444323,-5.55034300499343,54.));
#43316=CARTESIAN_POINT('Ctrl Pts',(82.242702024046,-5.62869421246123,54.));
#43317=CARTESIAN_POINT('Ctrl Pts',(82.0916444097254,-5.70083979834345,54.));
#43318=CARTESIAN_POINT('Ctrl Pts',(81.9377302789933,-5.76652227351167,54.));
#43319=CARTESIAN_POINT('Ctrl Pts',(81.8197903384035,-5.81685285188211,54.));
#43320=CARTESIAN_POINT('Ctrl Pts',(81.700172382812,-5.86338783920109,54.));
#43321=CARTESIAN_POINT('Ctrl Pts',(81.5790669755173,-5.90611323035059,54.));
#43322=CARTESIAN_POINT('Ctrl Pts',(74.8634535980369,0.000107814451578703,
51.1759584946969));
#43323=CARTESIAN_POINT('Ctrl Pts',(74.8639092161186,-0.570355406205201,
51.2068866386484));
#43324=CARTESIAN_POINT('Ctrl Pts',(74.9587810459553,-1.14096646897359,51.2378147825999));
#43325=CARTESIAN_POINT('Ctrl Pts',(75.1452601228757,-1.67987880496399,51.2687429265514));
#43326=CARTESIAN_POINT('Ctrl Pts',(75.4197255087757,-2.47306581932794,51.3142638777755));
#43327=CARTESIAN_POINT('Ctrl Pts',(75.89263800231,-3.19758446033676,51.3597848289997));
#43328=CARTESIAN_POINT('Ctrl Pts',(76.5082814088742,-3.76807555044598,51.4053057802238));
#43329=CARTESIAN_POINT('Ctrl Pts',(77.1239248154383,-4.33856664055521,51.450826731448));
#43330=CARTESIAN_POINT('Ctrl Pts',(77.8822991350322,-4.75503017976483,51.4963476826721));
#43331=CARTESIAN_POINT('Ctrl Pts',(78.6940564823907,-4.96840050758325,51.5418686338963));
#43332=CARTESIAN_POINT('Ctrl Pts',(79.5058138297492,-5.18177083540168,51.5873895851204));
#43333=CARTESIAN_POINT('Ctrl Pts',(80.3709542048723,-5.19204795182889,51.6329105363446));
#43334=CARTESIAN_POINT('Ctrl Pts',(81.1875510777335,-4.99802105929599,51.6784314875687));
#43335=CARTESIAN_POINT('Ctrl Pts',(82.0041479505947,-4.80399416676308,51.7239524387928));
#43336=CARTESIAN_POINT('Ctrl Pts',(82.7722013211941,-4.40566326527006,51.769473390017));
#43337=CARTESIAN_POINT('Ctrl Pts',(83.4012229665159,-3.84995771537295,51.8149943412411));
#43338=CARTESIAN_POINT('Ctrl Pts',(84.0302446118377,-3.29425216547584,51.8605152924653));
#43339=CARTESIAN_POINT('Ctrl Pts',(84.520234531882,-2.58117196717465,51.9060362436894));
#43340=CARTESIAN_POINT('Ctrl Pts',(84.8134645551446,-1.79472868292726,51.9515571949135));
#43341=CARTESIAN_POINT('Ctrl Pts',(85.1066945784073,-1.00828539867987,51.9970781461377));
#43342=CARTESIAN_POINT('Ctrl Pts',(85.2031647048884,-0.148479028486275,
52.0425990973618));
#43343=CARTESIAN_POINT('Ctrl Pts',(85.0915093037797,0.683392334134824,52.088120048586));
#43344=CARTESIAN_POINT('Ctrl Pts',(84.9798539026711,1.51526369675592,52.1336409998101));
#43345=CARTESIAN_POINT('Ctrl Pts',(84.6600729739728,2.31920005180453,52.1791619510343));
#43346=CARTESIAN_POINT('Ctrl Pts',(84.1698415161116,3.00048559910823,52.2246829022584));
#43347=CARTESIAN_POINT('Ctrl Pts',(83.6796100582504,3.68177114641193,52.2702038534825));
#43348=CARTESIAN_POINT('Ctrl Pts',(83.0189280712263,4.24040588597073,52.3157248047067));
#43349=CARTESIAN_POINT('Ctrl Pts',(82.265633811734,4.6105743038535,52.3612457559308));
#43350=CARTESIAN_POINT('Ctrl Pts',(81.5123395522418,4.98074272173626,52.406766707155));
#43351=CARTESIAN_POINT('Ctrl Pts',(80.6664330202815,5.16244481794298,52.4522876583791));
#43352=CARTESIAN_POINT('Ctrl Pts',(79.8275747198911,5.13427325239268,52.4978086096033));
#43353=CARTESIAN_POINT('Ctrl Pts',(78.9887164195008,5.10610168684238,52.5433295608274));
#43354=CARTESIAN_POINT('Ctrl Pts',(78.1569063506806,4.86805645953507,52.5888505120516));
#43355=CARTESIAN_POINT('Ctrl Pts',(77.4301442125608,4.44818309563375,52.6343714632757));
#43356=CARTESIAN_POINT('Ctrl Pts',(76.7033820744409,4.02830973173244,52.6798924144998));
#43357=CARTESIAN_POINT('Ctrl Pts',(76.0816678670215,3.42660823123714,52.725413365724));
#43358=CARTESIAN_POINT('Ctrl Pts',(75.6382489050602,2.71396759426174,52.7709343169481));
#43359=CARTESIAN_POINT('Ctrl Pts',(75.1948299430989,2.00132695728634,52.8164552681723));
#43360=CARTESIAN_POINT('Ctrl Pts',(74.9297062265958,1.17774718383084,52.8619762193964));
#43361=CARTESIAN_POINT('Ctrl Pts',(74.8741132188043,0.340259351903744,52.9074971706205));
#43362=CARTESIAN_POINT('Ctrl Pts',(74.8665978476355,0.227043101222055,52.9136509453126));
#43363=CARTESIAN_POINT('Ctrl Pts',(74.8629116778522,0.113572678934222,52.9198047200048));
#43364=CARTESIAN_POINT('Ctrl Pts',(74.8630099039127,9.58920879684522E-5,
52.9259584946969));
#43365=CARTESIAN_POINT('Ctrl Pts',(78.4211181181246,-5.90584097022479,54.));
#43366=CARTESIAN_POINT('Ctrl Pts',(77.455879038986,-5.647791608345,53.9544790487759));
#43367=CARTESIAN_POINT('Ctrl Pts',(75.6552430725963,-4.64961437394933,53.8634371463276));
#43368=CARTESIAN_POINT('Ctrl Pts',(73.9774513743918,-2.05559122386841,53.7268742926551));
#43369=CARTESIAN_POINT('Ctrl Pts',(73.7190590194211,1.02247359936586,53.5903114389827));
#43370=CARTESIAN_POINT('Ctrl Pts',(74.9405084533092,3.85979119586914,53.4537485853103));
#43371=CARTESIAN_POINT('Ctrl Pts',(77.3541911747203,5.78754789219838,53.3171857316378));
#43372=CARTESIAN_POINT('Ctrl Pts',(80.391275596298,6.35162199178929,53.1806228779654));
#43373=CARTESIAN_POINT('Ctrl Pts',(83.3361779879638,5.41904570738785,53.044060024293));
#43374=CARTESIAN_POINT('Ctrl Pts',(85.4949699527806,3.20958767782661,52.9074971706206));
#43375=CARTESIAN_POINT('Ctrl Pts',(86.3589850655242,0.243850535977484,52.7709343169481));
#43376=CARTESIAN_POINT('Ctrl Pts',(85.7246308116887,-2.7793433146957,52.6343714632757));
#43377=CARTESIAN_POINT('Ctrl Pts',(83.7413822653001,-5.14764123692896,52.4978086096033));
#43378=CARTESIAN_POINT('Ctrl Pts',(80.8765513474216,-6.30299985802483,52.3612457559308));
#43379=CARTESIAN_POINT('Ctrl Pts',(77.8051787527545,-5.9731825630531,52.2246829022584));
#43380=CARTESIAN_POINT('Ctrl Pts',(75.2509719030383,-4.23590394123515,52.0881200485859));
#43381=CARTESIAN_POINT('Ctrl Pts',(73.8157787618652,-1.5005191497456,51.9515571949136));
#43382=CARTESIAN_POINT('Ctrl Pts',(73.8377738960802,1.58843304652964,51.8149943412411));
#43383=CARTESIAN_POINT('Ctrl Pts',(75.3117746142583,4.30310269326682,51.6784314875687));
#43384=CARTESIAN_POINT('Ctrl Pts',(77.8904620590793,6.00383208915477,51.5418686338962));
#43385=CARTESIAN_POINT('Ctrl Pts',(80.9662200126132,6.28987829428071,51.4053057802239));
#43386=CARTESIAN_POINT('Ctrl Pts',(83.8143075062239,5.09384023309799,51.2687429265514));
#43387=CARTESIAN_POINT('Ctrl Pts',(85.7636295740737,2.6975403991448,51.132180072879));
#43388=CARTESIAN_POINT('Ctrl Pts',(86.354867380944,-0.334380983822473,50.9956172192065));
#43389=CARTESIAN_POINT('Ctrl Pts',(85.4487075396391,-3.28751216265552,50.8590543655341));
#43390=CARTESIAN_POINT('Ctrl Pts',(83.258668528712,-5.46600672263342,50.7224915118617));
#43391=CARTESIAN_POINT('Ctrl Pts',(80.3007893255799,-6.35654590588445,50.5859286581892));
#43392=CARTESIAN_POINT('Ctrl Pts',(77.2720351219492,-5.74929192997566,50.4493658045168));
#43393=CARTESIAN_POINT('Ctrl Pts',(74.8860713886881,-3.78733207289439,50.3128029508444));
#43394=CARTESIAN_POINT('Ctrl Pts',(73.7051028531023,-0.932963012101885,
50.1762400971719));
#43395=CARTESIAN_POINT('Ctrl Pts',(74.0074011771884,2.14124015953471,50.0396772434995));
#43396=CARTESIAN_POINT('Ctrl Pts',(75.7217357950776,4.71090282906051,49.9031143898271));
#43397=CARTESIAN_POINT('Ctrl Pts',(78.4441579740491,6.17053528166351,49.7665515361547));
#43398=CARTESIAN_POINT('Ctrl Pts',(81.5331832701364,6.17620426573987,49.6299886824822));
#43399=CARTESIAN_POINT('Ctrl Pts',(84.2609445326221,4.72657399835094,49.4934258288098));
#43400=CARTESIAN_POINT('Ctrl Pts',(85.9846992690839,2.16322091580975,49.3568629751373));
#43401=CARTESIAN_POINT('Ctrl Pts',(86.2982790838942,-0.909851995299122,
49.2203001214649));
#43402=CARTESIAN_POINT('Ctrl Pts',(85.1277951530875,-3.76853644535141,49.0837372677925));
#43403=CARTESIAN_POINT('Ctrl Pts',(82.7490486508255,-5.73924050614397,48.94717441412));
#43404=CARTESIAN_POINT('Ctrl Pts',(79.7225437079984,-6.35760710314802,48.8106115604476));
#43405=CARTESIAN_POINT('Ctrl Pts',(76.7614158020519,-5.47793049104956,48.6740487067752));
#43406=CARTESIAN_POINT('Ctrl Pts',(74.563395616688,-3.3074889041874,48.5374858531028));
#43407=CARTESIAN_POINT('Ctrl Pts',(73.6464027337136,-0.357703578130303,
48.4009229994303));
#43408=CARTESIAN_POINT('Ctrl Pts',(74.2265082218259,2.67636745596063,48.2643601457579));
#43409=CARTESIAN_POINT('Ctrl Pts',(76.1670218022879,5.07980592226054,48.1277972920855));
#43410=CARTESIAN_POINT('Ctrl Pts',(79.0107001846261,6.28628952143238,47.991234438413));
#43411=CARTESIAN_POINT('Ctrl Pts',(82.0874873209564,6.01153447605647,47.8546715847406));
#43412=CARTESIAN_POINT('Ctrl Pts',(84.6723997386214,4.32028132816605,47.7181087310682));
#43413=CARTESIAN_POINT('Ctrl Pts',(86.1563544240622,1.61104012280873,47.5815458773957));
#43414=CARTESIAN_POINT('Ctrl Pts',(86.1896870770046,-1.47781052937492,47.4449830237233));
#43415=CARTESIAN_POINT('Ctrl Pts',(84.7645435231389,-4.21844462901729,47.3084201700509));
#43416=CARTESIAN_POINT('Ctrl Pts',(82.2167303935176,-5.96508645657586,47.1718573163784));
#43417=CARTESIAN_POINT('Ctrl Pts',(79.1465889950142,-6.30617473025753,47.035294462706));
#43418=CARTESIAN_POINT('Ctrl Pts',(76.2775368648236,-5.1613388068622,46.8987316090336));
#43419=CARTESIAN_POINT('Ctrl Pts',(74.2856088680233,-2.80033641956749,46.7621687553612));
#43420=CARTESIAN_POINT('Ctrl Pts',(73.6401630760097,0.220509347236804,46.6256059016887));
#43421=CARTESIAN_POINT('Ctrl Pts',(74.4932859058703,3.18939648797121,46.4890430480163));
#43422=CARTESIAN_POINT('Ctrl Pts',(76.6439559920085,5.40676601013892,46.3524801943438));
#43423=CARTESIAN_POINT('Ctrl Pts',(79.5854108583403,6.35013904694908,46.2159173406715));
#43424=CARTESIAN_POINT('Ctrl Pts',(82.624555380254,5.79722857302948,46.079354486999));
#43425=CARTESIAN_POINT('Ctrl Pts',(85.0452758157915,3.87831690486471,45.9427916333266));
#43426=CARTESIAN_POINT('Ctrl Pts',(86.2771777145318,1.04555727349326,45.8062287796541));
#43427=CARTESIAN_POINT('Ctrl Pts',(86.0299879841389,-2.03356705891616,45.6696659259817));
#43428=CARTESIAN_POINT('Ctrl Pts',(84.3619519504042,-4.63352190610293,45.5331030723093));
#43429=CARTESIAN_POINT('Ctrl Pts',(81.6661090088627,-6.14167980625449,45.3965402186368));
#43430=CARTESIAN_POINT('Ctrl Pts',(78.5776807367317,-6.20267345467319,45.2599773649644));
#43431=CARTESIAN_POINT('Ctrl Pts',(75.8243936079491,-4.80213091560737,45.123414511292));
#43432=CARTESIAN_POINT('Ctrl Pts',(74.0550047758089,-2.27006208203801,44.9868516576196));
#43433=CARTESIAN_POINT('Ctrl Pts',(73.6864353996727,0.7969015682589,44.8502888039471));
#43434=CARTESIAN_POINT('Ctrl Pts',(74.8055314959948,3.67609127100912,44.7137259502747));
#43435=CARTESIAN_POINT('Ctrl Pts',(77.1486004080237,5.68908344454576,44.5771630966022));
#43436=CARTESIAN_POINT('Ctrl Pts',(80.1635447169054,6.36155666463022,44.4406002429298));
#43437=CARTESIAN_POINT('Ctrl Pts',(83.1399529776901,5.53505604037131,44.3040373892574));
#43438=CARTESIAN_POINT('Ctrl Pts',(85.3764939963492,3.4043299457581,44.167474535585));
#43439=CARTESIAN_POINT('Ctrl Pts',(86.3461715250332,0.471441453942473,44.0309116819125));
#43440=CARTESIAN_POINT('Ctrl Pts',(85.8205004111942,-2.57253280683391,43.8943488282401));
#43441=CARTESIAN_POINT('Ctrl Pts',(83.9233445571365,-5.0103410604769,43.7577859745677));
#43442=CARTESIAN_POINT('Ctrl Pts',(81.1017308763422,-6.26756245882339,43.6212231208953));
#43443=CARTESIAN_POINT('Ctrl Pts',(78.020516297909,-6.04795786312262,43.4846602672228));
#43444=CARTESIAN_POINT('Ctrl Pts',(75.40572755909,-4.40327273783911,43.3480974135504));
#43445=CARTESIAN_POINT('Ctrl Pts',(73.8734873761917,-1.72104424964613,43.211534559878));
#43446=CARTESIAN_POINT('Ctrl Pts',(73.784837682508,1.36671388452568,43.0749717062055));
#43447=CARTESIAN_POINT('Ctrl Pts',(75.1606667541984,4.13243333827823,42.9384088525331));
#43448=CARTESIAN_POINT('Ctrl Pts',(77.6767884766317,5.92442701100857,42.8018459988606));
#43449=CARTESIAN_POINT('Ctrl Pts',(80.7403278321772,6.32044846892683,42.6652831451882));
#43450=CARTESIAN_POINT('Ctrl Pts',(83.6294253939595,5.22718080357853,42.5287202915158));
#43451=CARTESIAN_POINT('Ctrl Pts',(85.6633177227071,2.90223574469819,42.3921574378434));
#43452=CARTESIAN_POINT('Ctrl Pts',(86.3627699345494,-0.106570534545254,
42.2555945841709));
#43453=CARTESIAN_POINT('Ctrl Pts',(85.5629461401894,-3.09025001994495,42.1190317304985));
#43454=CARTESIAN_POINT('Ctrl Pts',(83.45236018166,-5.34580695151189,41.9824688768261));
#43455=CARTESIAN_POINT('Ctrl Pts',(80.5282216380884,-6.34166017411614,41.8459060231536));
#43456=CARTESIAN_POINT('Ctrl Pts',(77.4797852514363,-5.84337786289595,41.7093431694812));
#43457=CARTESIAN_POINT('Ctrl Pts',(75.0248946938219,-3.96789034338118,41.5727803158088));
#43458=CARTESIAN_POINT('Ctrl Pts',(74.1705695184084,-2.09471758856737,41.4817384133605));
#43459=CARTESIAN_POINT('Ctrl Pts',(73.988784526404,-1.1122563070174,41.4362174621363));
#43460=CARTESIAN_POINT('Ctrl Pts',(78.5051856848936,-5.59138446414239,54.1879275126212));
#43461=CARTESIAN_POINT('Ctrl Pts',(77.5913407611158,-5.34707494069419,54.1424065613971));
#43462=CARTESIAN_POINT('Ctrl Pts',(75.8865796578611,-4.40204565375622,54.0513646589488));
#43463=CARTESIAN_POINT('Ctrl Pts',(74.2981219796566,-1.94614126789259,53.9148018052764));
#43464=CARTESIAN_POINT('Ctrl Pts',(74.0534877257849,0.968031991940416,53.7782389516039));
#43465=CARTESIAN_POINT('Ctrl Pts',(75.2099010838163,3.6542766112774,53.6416760979315));
#43466=CARTESIAN_POINT('Ctrl Pts',(77.4950672672453,5.47938990112807,53.5051132442591));
#43467=CARTESIAN_POINT('Ctrl Pts',(80.3704421269332,6.01342987494025,53.3685503905866));
#43468=CARTESIAN_POINT('Ctrl Pts',(83.1585431889481,5.13050861537382,53.2319875369142));
#43469=CARTESIAN_POINT('Ctrl Pts',(85.202390274274,3.0386931799519,53.0954246832418));
#43470=CARTESIAN_POINT('Ctrl Pts',(86.0204009018096,0.23086671403978,52.9588618295694));
#43471=CARTESIAN_POINT('Ctrl Pts',(85.4198228406087,-2.63135717819982,52.8222989758969));
#43472=CARTESIAN_POINT('Ctrl Pts',(83.5421723642892,-4.873555076111,52.6857361222245));
#43473=CARTESIAN_POINT('Ctrl Pts',(80.8298793703903,-5.9673966267179,52.549173268552));
#43474=CARTESIAN_POINT('Ctrl Pts',(77.9220420114104,-5.65514045381926,52.4126104148797));
#43475=CARTESIAN_POINT('Ctrl Pts',(75.5038339069743,-4.01036323328569,52.2760475612072));
#43476=CARTESIAN_POINT('Ctrl Pts',(74.1450576254833,-1.42062400669694,52.1394847075348));
#43477=CARTESIAN_POINT('Ctrl Pts',(74.1658816287634,1.50385692799279,52.0029218538623));
#43478=CARTESIAN_POINT('Ctrl Pts',(75.561399177798,4.07398398772421,51.8663590001899));
#43479=CARTESIAN_POINT('Ctrl Pts',(78.0027844080377,5.68415804588484,51.7297961465174));
#43480=CARTESIAN_POINT('Ctrl Pts',(80.9147736274489,5.95497372064338,51.593233292845));
#43481=CARTESIAN_POINT('Ctrl Pts',(83.6112147007152,4.82261870676202,51.4566704391726));
#43482=CARTESIAN_POINT('Ctrl Pts',(85.4567451138666,2.5539098589376,51.3201075855002));
#43483=CARTESIAN_POINT('Ctrl Pts',(86.0165024633475,-0.316576868133725,
51.1835447318278));
#43484=CARTESIAN_POINT('Ctrl Pts',(85.1585911033486,-3.1124685755383,51.0469818781553));
#43485=CARTESIAN_POINT('Ctrl Pts',(83.0851607209018,-5.17496919133383,50.9104190244829));
#43486=CARTESIAN_POINT('Ctrl Pts',(80.284773797755,-6.01809161522638,50.7738561708104));
#43487=CARTESIAN_POINT('Ctrl Pts',(77.4172856135544,-5.44317087763737,50.6372933171381));
#43488=CARTESIAN_POINT('Ctrl Pts',(75.1583625207344,-3.5856755743499,50.5007304634656));
#43489=CARTESIAN_POINT('Ctrl Pts',(74.0402746555502,-0.883287395950221,
50.3641676097932));
#43490=CARTESIAN_POINT('Ctrl Pts',(74.326477105185,2.02722982592681,50.2276047561207));
#43491=CARTESIAN_POINT('Ctrl Pts',(75.9495319752931,4.46007080503741,50.0910419024483));
#43492=CARTESIAN_POINT('Ctrl Pts',(78.5269987836753,5.84198512680619,49.9544790487759));
#43493=CARTESIAN_POINT('Ctrl Pts',(81.4515489259775,5.84735226582193,49.8179161951034));
#43494=CARTESIAN_POINT('Ctrl Pts',(84.0340705383689,4.47490756290936,49.681353341431));
#43495=CARTESIAN_POINT('Ctrl Pts',(85.6660439528304,2.04804021682049,49.5447904877586));
#43496=CARTESIAN_POINT('Ctrl Pts',(85.9629272102087,-0.861406925251295,
49.4082276340861));
#43497=CARTESIAN_POINT('Ctrl Pts',(84.8547656970158,-3.56788072000698,49.2716647804137));
#43498=CARTESIAN_POINT('Ctrl Pts',(82.602675553726,-5.43365464187376,49.1351019267412));
#43499=CARTESIAN_POINT('Ctrl Pts',(79.7373168684362,-6.01909630904101,48.9985390730689));
#43500=CARTESIAN_POINT('Ctrl Pts',(76.9338542196583,-5.18625807869333,48.8619762193964));
#43501=CARTESIAN_POINT('Ctrl Pts',(74.8528676204124,-3.13138165545505,48.725413365724));
#43502=CARTESIAN_POINT('Ctrl Pts',(73.9847000240544,-0.338657650893332,
48.5888505120515));
#43503=CARTESIAN_POINT('Ctrl Pts',(74.5339177950964,2.53386426912626,48.4522876583791));
#43504=CARTESIAN_POINT('Ctrl Pts',(76.3711087287763,4.80933165281371,48.3157248047067));
#43505=CARTESIAN_POINT('Ctrl Pts',(79.0633754539025,5.95157603200757,48.1791619510343));
#43506=CARTESIAN_POINT('Ctrl Pts',(81.9763390572716,5.69145031919123,48.0425990973618));
#43507=CARTESIAN_POINT('Ctrl Pts',(84.4236178116724,4.09024794619769,47.9060362436894));
#43508=CARTESIAN_POINT('Ctrl Pts',(85.8285593289765,1.52526029048154,47.7694733900169));
#43509=CARTESIAN_POINT('Ctrl Pts',(85.8601171847926,-1.39912450683183,47.6329105363445));
#43510=CARTESIAN_POINT('Ctrl Pts',(84.5108554003267,-3.99383354215757,47.4963476826721));
#43511=CARTESIAN_POINT('Ctrl Pts',(82.0987005823549,-5.64747542453636,47.3597848289997));
#43512=CARTESIAN_POINT('Ctrl Pts',(79.1920288644982,-5.97040245287662,47.2232219753272));
#43513=CARTESIAN_POINT('Ctrl Pts',(76.4757394167395,-4.88652331892474,47.0866591216548));
#43514=CARTESIAN_POINT('Ctrl Pts',(74.5898716273508,-2.65123250518983,46.9500962679824));
#43515=CARTESIAN_POINT('Ctrl Pts',(73.9787925969288,0.208768326907914,46.8135334143099));
#43516=CARTESIAN_POINT('Ctrl Pts',(74.7864909011902,3.01957707001274,46.6769705606375));
#43517=CARTESIAN_POINT('Ctrl Pts',(76.8226485572726,5.11888275061244,46.5404077069651));
#43518=CARTESIAN_POINT('Ctrl Pts',(79.6074856574423,6.01202588949896,46.4038448532926));
#43519=CARTESIAN_POINT('Ctrl Pts',(82.4848109274224,5.48855513410238,46.2672819996202));
#43520=CARTESIAN_POINT('Ctrl Pts',(84.7766401018847,3.67181591888614,46.1307191459478));
#43521=CARTESIAN_POINT('Ctrl Pts',(85.942949383271,0.989886575824742,45.9941562922754));
#43522=CARTESIAN_POINT('Ctrl Pts',(85.7089212702245,-1.92528977961673,45.8575934386029));
#43523=CARTESIAN_POINT('Ctrl Pts',(84.1296998161292,-4.38681002937017,45.7210305849305));
#43524=CARTESIAN_POINT('Ctrl Pts',(81.5773970336638,-5.81466606120303,45.5844677312581));
#43525=CARTESIAN_POINT('Ctrl Pts',(78.6534121267769,-5.87241210277425,45.4479048775856));
#43526=CARTESIAN_POINT('Ctrl Pts',(76.0467237728552,-4.54644145206012,45.3113420239132));
#43527=CARTESIAN_POINT('Ctrl Pts',(74.3715460501678,-2.14919262508739,45.1747791702408));
#43528=CARTESIAN_POINT('Ctrl Pts',(74.02260115069,0.754470543768118,45.0382163165683));
#43529=CARTESIAN_POINT('Ctrl Pts',(75.082110974677,3.48035778902924,44.9016534628959));
#43530=CARTESIAN_POINT('Ctrl Pts',(77.3004231810475,5.38616819305111,44.7650906092235));
#43531=CARTESIAN_POINT('Ctrl Pts',(80.1548367783535,6.02283557611966,44.6285277555511));
#43532=CARTESIAN_POINT('Ctrl Pts',(82.9727661794669,5.24034197810641,44.4919649018786));
#43533=CARTESIAN_POINT('Ctrl Pts',(85.0902225702155,3.22306639570792,44.3554020482062));
#43534=CARTESIAN_POINT('Ctrl Pts',(86.0082696182899,0.446339553438113,44.2188391945338));
#43535=CARTESIAN_POINT('Ctrl Pts',(85.5105878632297,-2.43555829595599,44.0822763408613));
#43536=CARTESIAN_POINT('Ctrl Pts',(83.7144460737851,-4.74356544763836,43.9457134871889));
#43537=CARTESIAN_POINT('Ctrl Pts',(81.0430692151556,-5.93384609185868,43.8091506335164));
#43538=CARTESIAN_POINT('Ctrl Pts',(78.1259139088411,-5.72593434299071,43.672587779844));
#43539=CARTESIAN_POINT('Ctrl Pts',(75.6503495980245,-4.1688204782118,43.5360249261716));
#43540=CARTESIAN_POINT('Ctrl Pts',(74.1996935446045,-1.629407247518,43.3994620724992));
#43541=CARTESIAN_POINT('Ctrl Pts',(74.1157640039154,1.29394320290574,43.2628992188267));
#43542=CARTESIAN_POINT('Ctrl Pts',(75.4183370558397,3.91240192264668,43.1263363651543));
#43543=CARTESIAN_POINT('Ctrl Pts',(77.8004878756186,5.60898089117325,42.9897735114819));
#43544=CARTESIAN_POINT('Ctrl Pts',(80.7009090762987,5.98391618632172,42.8532106578094));
#43545=CARTESIAN_POINT('Ctrl Pts',(83.4361766366318,4.94885955848552,42.716647804137));
#43546=CARTESIAN_POINT('Ctrl Pts',(85.3617743670875,2.74770620069144,42.5800849504646));
#43547=CARTESIAN_POINT('Ctrl Pts',(86.0239842454813,-0.100896186368019,
42.4435220967921));
#43548=CARTESIAN_POINT('Ctrl Pts',(85.2667470695425,-2.92570965573735,42.3069592431197));
#43549=CARTESIAN_POINT('Ctrl Pts',(83.2685392616698,-5.06116945709941,42.1703963894473));
#43550=CARTESIAN_POINT('Ctrl Pts',(80.5000964766443,-6.0039984742552,42.0338335357748));
#43551=CARTESIAN_POINT('Ctrl Pts',(77.6139740872696,-5.5322472050016,41.8972706821024));
#43552=CARTESIAN_POINT('Ctrl Pts',(75.2897941789012,-3.75662001961385,41.76070782843));
#43553=CARTESIAN_POINT('Ctrl Pts',(74.4809575479766,-1.98318434927916,41.6696659259817));
#43554=CARTESIAN_POINT('Ctrl Pts',(74.308851697983,-1.05303421926797,41.6241449747576));
#43555=CARTESIAN_POINT('Ctrl Pts',(78.5892532516625,-5.27692795806,54.3758550252424));
#43556=CARTESIAN_POINT('Ctrl Pts',(77.7268024832456,-5.04635827304338,54.3303340740183));
#43557=CARTESIAN_POINT('Ctrl Pts',(76.1179162431258,-4.15447693356311,54.23929217157));
#43558=CARTESIAN_POINT('Ctrl Pts',(74.6187925849215,-1.83669131191678,54.1027293178976));
#43559=CARTESIAN_POINT('Ctrl Pts',(74.3879164321487,0.913590384514973,53.9661664642252));
#43560=CARTESIAN_POINT('Ctrl Pts',(75.4792937143235,3.44876202668567,53.8296036105527));
#43561=CARTESIAN_POINT('Ctrl Pts',(77.6359433597704,5.17123191005776,53.6930407568803));
#43562=CARTESIAN_POINT('Ctrl Pts',(80.3496086575683,5.6752377580912,53.5564779032078));
#43563=CARTESIAN_POINT('Ctrl Pts',(82.9809083899325,4.84197152335979,53.4199150495354));
#43564=CARTESIAN_POINT('Ctrl Pts',(84.9098105957675,2.86779868207719,53.283352195863));
#43565=CARTESIAN_POINT('Ctrl Pts',(85.681816738095,0.217882892102075,53.1467893421906));
#43566=CARTESIAN_POINT('Ctrl Pts',(85.1150148695287,-2.48337104170394,53.0102264885181));
#43567=CARTESIAN_POINT('Ctrl Pts',(83.3429624632783,-4.59946891529305,52.8736636348457));
#43568=CARTESIAN_POINT('Ctrl Pts',(80.7832073933592,-5.63179339541097,52.7371007811733));
#43569=CARTESIAN_POINT('Ctrl Pts',(78.0389052700664,-5.33709834458541,52.6005379275009));
#43570=CARTESIAN_POINT('Ctrl Pts',(75.7566959109101,-3.78482252533623,52.4639750738284));
#43571=CARTESIAN_POINT('Ctrl Pts',(74.4743364891013,-1.34072886364829,52.327412220156));
#43572=CARTESIAN_POINT('Ctrl Pts',(74.4939893614466,1.41928080945594,52.1908493664835));
#43573=CARTESIAN_POINT('Ctrl Pts',(75.8110237413377,3.8448652821816,52.0542865128111));
#43574=CARTESIAN_POINT('Ctrl Pts',(78.115106756996,5.36448400261491,51.9177236591387));
#43575=CARTESIAN_POINT('Ctrl Pts',(80.8633272422847,5.62006914700605,51.7811608054663));
#43576=CARTESIAN_POINT('Ctrl Pts',(83.4081218952066,4.55139718042604,51.6445979517938));
#43577=CARTESIAN_POINT('Ctrl Pts',(85.1498606536595,2.41027931873041,51.5080350981214));
#43578=CARTESIAN_POINT('Ctrl Pts',(85.6781375457509,-0.298772752444985,
51.371472244449));
#43579=CARTESIAN_POINT('Ctrl Pts',(84.8684746670582,-2.93742498842107,51.2349093907766));
#43580=CARTESIAN_POINT('Ctrl Pts',(82.9116529130915,-4.88393166003425,51.0983465371041));
#43581=CARTESIAN_POINT('Ctrl Pts',(80.2687582699299,-5.67963732456832,50.9617836834317));
#43582=CARTESIAN_POINT('Ctrl Pts',(77.5625361051596,-5.13704982529907,50.8252208297592));
#43583=CARTESIAN_POINT('Ctrl Pts',(75.4306536527807,-3.3840190758054,50.6886579760868));
#43584=CARTESIAN_POINT('Ctrl Pts',(74.3754464579983,-0.833611779798555,
50.5520951224143));
#43585=CARTESIAN_POINT('Ctrl Pts',(74.6455530331815,1.91321949231889,50.4155322687419));
#43586=CARTESIAN_POINT('Ctrl Pts',(76.1773281555086,4.20923878101431,50.2789694150695));
#43587=CARTESIAN_POINT('Ctrl Pts',(78.6098395933014,5.51343497194888,50.1424065613971));
#43588=CARTESIAN_POINT('Ctrl Pts',(81.3699145818185,5.51850026590399,50.0058437077246));
#43589=CARTESIAN_POINT('Ctrl Pts',(83.8071965441157,4.22324112746778,49.8692808540522));
#43590=CARTESIAN_POINT('Ctrl Pts',(85.3473886365768,1.93285951783123,49.7327180003798));
#43591=CARTESIAN_POINT('Ctrl Pts',(85.6275753365233,-0.812961855203473,
49.5961551467073));
#43592=CARTESIAN_POINT('Ctrl Pts',(84.5817362409442,-3.36722499466254,49.4595922930349));
#43593=CARTESIAN_POINT('Ctrl Pts',(82.4563024566265,-5.12806877760354,49.3230294393625));
#43594=CARTESIAN_POINT('Ctrl Pts',(79.752090028874,-5.680585514934,49.1864665856901));
#43595=CARTESIAN_POINT('Ctrl Pts',(77.1062926372646,-4.89458566633712,49.0499037320176));
#43596=CARTESIAN_POINT('Ctrl Pts',(75.1423396241368,-2.95527440672271,48.9133408783452));
#43597=CARTESIAN_POINT('Ctrl Pts',(74.3229973143953,-0.319611723656359,
48.7767780246728));
#43598=CARTESIAN_POINT('Ctrl Pts',(74.8413273683668,2.39136108229189,48.6402151710003));
#43599=CARTESIAN_POINT('Ctrl Pts',(76.5751956552648,4.53885738336689,48.5036523173279));
#43600=CARTESIAN_POINT('Ctrl Pts',(79.1160507231789,5.61686254258275,48.3670894636555));
#43601=CARTESIAN_POINT('Ctrl Pts',(81.8651907935868,5.37136616232601,48.2305266099831));
#43602=CARTESIAN_POINT('Ctrl Pts',(84.1748358847232,3.86021456422933,48.0939637563106));
#43603=CARTESIAN_POINT('Ctrl Pts',(85.5007642338909,1.43948045815434,47.9574009026382));
#43604=CARTESIAN_POINT('Ctrl Pts',(85.5305472925806,-1.32043848428875,47.8208380489658));
#43605=CARTESIAN_POINT('Ctrl Pts',(84.2571672775145,-3.76922245529786,47.6842751952933));
#43606=CARTESIAN_POINT('Ctrl Pts',(81.9806707711923,-5.32986439249687,47.5477123416209));
#43607=CARTESIAN_POINT('Ctrl Pts',(79.2374687339821,-5.63463017549571,47.4111494879484));
#43608=CARTESIAN_POINT('Ctrl Pts',(76.6739419686554,-4.61170783098729,47.274586634276));
#43609=CARTESIAN_POINT('Ctrl Pts',(74.8941343866782,-2.50212859081217,47.1380237806036));
#43610=CARTESIAN_POINT('Ctrl Pts',(74.3174221178479,0.197027306579024,47.0014609269311));
#43611=CARTESIAN_POINT('Ctrl Pts',(75.0796958965101,2.84975765205427,46.8648980732588));
#43612=CARTESIAN_POINT('Ctrl Pts',(77.0013411225368,4.83099949108596,46.7283352195863));
#43613=CARTESIAN_POINT('Ctrl Pts',(79.6295604565443,5.67391273204884,46.5917723659139));
#43614=CARTESIAN_POINT('Ctrl Pts',(82.3450664745908,5.17988169517528,46.4552095122414));
#43615=CARTESIAN_POINT('Ctrl Pts',(84.5080043879781,3.46531493290757,46.318646658569));
#43616=CARTESIAN_POINT('Ctrl Pts',(85.6087210520102,0.934215878156226,46.1820838048966));
#43617=CARTESIAN_POINT('Ctrl Pts',(85.3878545563101,-1.8170125003173,46.0455209512241));
#43618=CARTESIAN_POINT('Ctrl Pts',(83.8974476818542,-4.14009815263742,45.9089580975517));
#43619=CARTESIAN_POINT('Ctrl Pts',(81.4886850584649,-5.48765231615157,45.7723952438793));
#43620=CARTESIAN_POINT('Ctrl Pts',(78.7291435168221,-5.54215075087533,45.6358323902069));
#43621=CARTESIAN_POINT('Ctrl Pts',(76.2690539377614,-4.29075198851288,45.4992695365344));
#43622=CARTESIAN_POINT('Ctrl Pts',(74.6880873245266,-2.02832316813677,45.362706682862));
#43623=CARTESIAN_POINT('Ctrl Pts',(74.3587669017073,0.712039519277336,45.2261438291895));
#43624=CARTESIAN_POINT('Ctrl Pts',(75.3586904533591,3.28462430704937,45.0895809755172));
#43625=CARTESIAN_POINT('Ctrl Pts',(77.4522459540714,5.08325294155646,44.9530181218447));
#43626=CARTESIAN_POINT('Ctrl Pts',(80.1461288398016,5.68411448760911,44.8164552681723));
#43627=CARTESIAN_POINT('Ctrl Pts',(82.8055793812436,4.94562791584151,44.6798924144999));
#43628=CARTESIAN_POINT('Ctrl Pts',(84.8039511440818,3.04180284565774,44.5433295608274));
#43629=CARTESIAN_POINT('Ctrl Pts',(85.6703677115467,0.421237652933754,44.406766707155));
#43630=CARTESIAN_POINT('Ctrl Pts',(85.2006753152652,-2.29858378507807,44.2702038534825));
#43631=CARTESIAN_POINT('Ctrl Pts',(83.5055475904337,-4.47678983479981,44.1336409998101));
#43632=CARTESIAN_POINT('Ctrl Pts',(80.9844075539689,-5.60012972489397,43.9970781461377));
#43633=CARTESIAN_POINT('Ctrl Pts',(78.2313115197731,-5.40391082285879,43.8605152924653));
#43634=CARTESIAN_POINT('Ctrl Pts',(75.894971636959,-3.93436821858449,43.7239524387928));
#43635=CARTESIAN_POINT('Ctrl Pts',(74.5258997130174,-1.53777024538986,43.5873895851204));
#43636=CARTESIAN_POINT('Ctrl Pts',(74.4466903253228,1.22117252128579,43.4508267314479));
#43637=CARTESIAN_POINT('Ctrl Pts',(75.6760073574809,3.69237050701514,43.3142638777755));
#43638=CARTESIAN_POINT('Ctrl Pts',(77.9241872746054,5.29353477133792,43.1777010241031));
#43639=CARTESIAN_POINT('Ctrl Pts',(80.6614903204203,5.6473839037166,43.0411381704306));
#43640=CARTESIAN_POINT('Ctrl Pts',(83.2429278793041,4.67053831339252,42.9045753167582));
#43641=CARTESIAN_POINT('Ctrl Pts',(85.060231011468,2.59317665668469,42.7680124630858));
#43642=CARTESIAN_POINT('Ctrl Pts',(85.6851985564131,-0.0952218381907853,
42.6314496094134));
#43643=CARTESIAN_POINT('Ctrl Pts',(84.9705479988958,-2.76116929152976,42.4948867557409));
#43644=CARTESIAN_POINT('Ctrl Pts',(83.0847183416795,-4.77653196268692,42.3583239020685));
#43645=CARTESIAN_POINT('Ctrl Pts',(80.4719713152003,-5.66633677439428,42.2217610483961));
#43646=CARTESIAN_POINT('Ctrl Pts',(77.7481629231028,-5.22111654710725,42.0851981947237));
#43647=CARTESIAN_POINT('Ctrl Pts',(75.5546936639805,-3.54534969584653,41.9486353410512));
#43648=CARTESIAN_POINT('Ctrl Pts',(74.7913455775449,-1.87165110999094,41.8575934386029));
#43649=CARTESIAN_POINT('Ctrl Pts',(74.6289188695621,-0.993812131518549,
41.8120724873788));
#43650=CARTESIAN_POINT('Ctrl Pts',(78.6733208184315,-4.96247145197761,54.5637825378637));
#43651=CARTESIAN_POINT('Ctrl Pts',(77.8622642053754,-4.74564160539257,54.5182615866395));
#43652=CARTESIAN_POINT('Ctrl Pts',(76.3492528283906,-3.90690821337,54.4272196841912));
#43653=CARTESIAN_POINT('Ctrl Pts',(74.9394631901864,-1.72724135594096,54.2906568305188));
#43654=CARTESIAN_POINT('Ctrl Pts',(74.7223451385125,0.85914877708953,54.1540939768464));
#43655=CARTESIAN_POINT('Ctrl Pts',(75.7486863448307,3.24324744209394,54.017531123174));
#43656=CARTESIAN_POINT('Ctrl Pts',(77.7768194522954,4.86307391898745,53.8809682695015));
#43657=CARTESIAN_POINT('Ctrl Pts',(80.3287751882034,5.33704564124216,53.7444054158291));
#43658=CARTESIAN_POINT('Ctrl Pts',(82.8032735909169,4.55343443134576,53.6078425621567));
#43659=CARTESIAN_POINT('Ctrl Pts',(84.617230917261,2.69690418420248,53.4712797084842));
#43660=CARTESIAN_POINT('Ctrl Pts',(85.3432325743804,0.204899070164371,53.3347168548118));
#43661=CARTESIAN_POINT('Ctrl Pts',(84.8102068984487,-2.33538490520805,53.1981540011394));
#43662=CARTESIAN_POINT('Ctrl Pts',(83.1437525622673,-4.32538275447508,53.0615911474669));
#43663=CARTESIAN_POINT('Ctrl Pts',(80.7365354163281,-5.29619016410404,52.9250282937945));
#43664=CARTESIAN_POINT('Ctrl Pts',(78.1557685287222,-5.01905623535157,52.7884654401221));
#43665=CARTESIAN_POINT('Ctrl Pts',(76.0095579148461,-3.55928181738677,52.6519025864496));
#43666=CARTESIAN_POINT('Ctrl Pts',(74.8036153527193,-1.26083372059963,52.5153397327772));
#43667=CARTESIAN_POINT('Ctrl Pts',(74.8220970941299,1.33470469091909,52.3787768791048));
#43668=CARTESIAN_POINT('Ctrl Pts',(76.0606483048774,3.61574657663899,52.2422140254324));
#43669=CARTESIAN_POINT('Ctrl Pts',(78.2274291059544,5.04480995934498,52.1056511717599));
#43670=CARTESIAN_POINT('Ctrl Pts',(80.8118808571204,5.28516457336873,51.9690883180875));
#43671=CARTESIAN_POINT('Ctrl Pts',(83.2050290896979,4.28017565409007,51.832525464415));
#43672=CARTESIAN_POINT('Ctrl Pts',(84.8429761934525,2.26664877852321,51.6959626107426));
#43673=CARTESIAN_POINT('Ctrl Pts',(85.3397726281543,-0.280968636756239,
51.5593997570702));
#43674=CARTESIAN_POINT('Ctrl Pts',(84.5783582307678,-2.76238140130385,51.4228369033978));
#43675=CARTESIAN_POINT('Ctrl Pts',(82.7381451052813,-4.59289412873466,51.2862740497253));
#43676=CARTESIAN_POINT('Ctrl Pts',(80.2527427421049,-5.34118303391026,51.1497111960529));
#43677=CARTESIAN_POINT('Ctrl Pts',(77.7077865967648,-4.83092877296077,51.0131483423805));
#43678=CARTESIAN_POINT('Ctrl Pts',(75.702944784827,-3.18236257726091,50.876585488708));
#43679=CARTESIAN_POINT('Ctrl Pts',(74.7106182604463,-0.783936163646889,
50.7400226350356));
#43680=CARTESIAN_POINT('Ctrl Pts',(74.9646289611781,1.79920915871098,50.6034597813632));
#43681=CARTESIAN_POINT('Ctrl Pts',(76.405124335724,3.95840675699122,50.4668969276907));
#43682=CARTESIAN_POINT('Ctrl Pts',(78.6926804029276,5.18488481709156,50.3303340740183));
#43683=CARTESIAN_POINT('Ctrl Pts',(81.2882802376596,5.18964826598606,50.1937712203459));
#43684=CARTESIAN_POINT('Ctrl Pts',(83.5803225498624,3.97157469202619,50.0572083666735));
#43685=CARTESIAN_POINT('Ctrl Pts',(85.0287333203233,1.81767881884198,49.920645513001));
#43686=CARTESIAN_POINT('Ctrl Pts',(85.2922234628379,-0.764516785155648,
49.7840826593286));
#43687=CARTESIAN_POINT('Ctrl Pts',(84.3087067848726,-3.1665692693181,49.6475198056562));
#43688=CARTESIAN_POINT('Ctrl Pts',(82.3099293595269,-4.82248291333333,49.5109569519837));
#43689=CARTESIAN_POINT('Ctrl Pts',(79.7668631893118,-5.34207472082699,49.3743940983113));
#43690=CARTESIAN_POINT('Ctrl Pts',(77.278731054871,-4.6029132539809,49.2378312446389));
#43691=CARTESIAN_POINT('Ctrl Pts',(75.4318116278612,-2.77916715799037,49.1012683909664));
#43692=CARTESIAN_POINT('Ctrl Pts',(74.6612946047361,-0.300565796419388,
48.964705537294));
#43693=CARTESIAN_POINT('Ctrl Pts',(75.1487369416373,2.24885789545753,48.8281426836216));
#43694=CARTESIAN_POINT('Ctrl Pts',(76.7792825817531,4.26838311392006,48.6915798299491));
#43695=CARTESIAN_POINT('Ctrl Pts',(79.1687259924554,5.28214905315793,48.5550169762767));
#43696=CARTESIAN_POINT('Ctrl Pts',(81.7540425299019,5.05128200546077,48.4184541226042));
#43697=CARTESIAN_POINT('Ctrl Pts',(83.9260539577742,3.63018118226098,48.2818912689319));
#43698=CARTESIAN_POINT('Ctrl Pts',(85.1729691388052,1.35370062582714,48.1453284152594));
#43699=CARTESIAN_POINT('Ctrl Pts',(85.2009774003686,-1.24175246174566,48.008765561587));
#43700=CARTESIAN_POINT('Ctrl Pts',(84.0034791547023,-3.54461136843815,47.8722027079146));
#43701=CARTESIAN_POINT('Ctrl Pts',(81.8626409600297,-5.01225336045737,47.7356398542421));
#43702=CARTESIAN_POINT('Ctrl Pts',(79.282908603466,-5.2988578981148,47.5990770005697));
#43703=CARTESIAN_POINT('Ctrl Pts',(76.8721445205713,-4.33689234304983,47.4625141468972));
#43704=CARTESIAN_POINT('Ctrl Pts',(75.1983971460056,-2.35302467643452,47.3259512932248));
#43705=CARTESIAN_POINT('Ctrl Pts',(74.6560516387671,0.185286286250136,47.1893884395524));
#43706=CARTESIAN_POINT('Ctrl Pts',(75.37290089183,2.6799382340958,47.05282558588));
#43707=CARTESIAN_POINT('Ctrl Pts',(77.180033687801,4.54311623155949,46.9162627322075));
#43708=CARTESIAN_POINT('Ctrl Pts',(79.6516352556463,5.33579957459872,46.7796998785351));
#43709=CARTESIAN_POINT('Ctrl Pts',(82.2053220217592,4.87120825624818,46.6431370248627));
#43710=CARTESIAN_POINT('Ctrl Pts',(84.2393686740714,3.25881394692901,46.5065741711902));
#43711=CARTESIAN_POINT('Ctrl Pts',(85.2744927207494,0.87854518048771,46.3700113175178));
#43712=CARTESIAN_POINT('Ctrl Pts',(85.0667878423957,-1.70873522101788,46.2334484638454));
#43713=CARTESIAN_POINT('Ctrl Pts',(83.6651955475792,-3.89338627590466,46.0968856101729));
#43714=CARTESIAN_POINT('Ctrl Pts',(81.399973083266,-5.16063857110011,45.9603227565005));
#43715=CARTESIAN_POINT('Ctrl Pts',(78.8048749068673,-5.21188939897639,45.8237599028281));
#43716=CARTESIAN_POINT('Ctrl Pts',(76.4913841026675,-4.03506252496563,45.6871970491556));
#43717=CARTESIAN_POINT('Ctrl Pts',(75.0046285988854,-1.90745371118615,45.5506341954832));
#43718=CARTESIAN_POINT('Ctrl Pts',(74.6949326527246,0.669608494786554,45.4140713418108));
#43719=CARTESIAN_POINT('Ctrl Pts',(75.6352699320413,3.08889082506949,45.2775084881384));
#43720=CARTESIAN_POINT('Ctrl Pts',(77.6040687270953,4.78033769006181,45.1409456344659));
#43721=CARTESIAN_POINT('Ctrl Pts',(80.1374209012496,5.34539339909855,45.0043827807935));
#43722=CARTESIAN_POINT('Ctrl Pts',(82.6383925830204,4.65091385357662,44.8678199271211));
#43723=CARTESIAN_POINT('Ctrl Pts',(84.5176797179481,2.86053929560756,44.7312570734486));
#43724=CARTESIAN_POINT('Ctrl Pts',(85.3324658048034,0.396135752429396,44.5946942197762));
#43725=CARTESIAN_POINT('Ctrl Pts',(84.8907627673008,-2.16160927420015,44.4581313661037));
#43726=CARTESIAN_POINT('Ctrl Pts',(83.2966491070823,-4.21001422196126,44.3215685124314));
#43727=CARTESIAN_POINT('Ctrl Pts',(80.9257458927823,-5.26641335792926,44.1850056587589));
#43728=CARTESIAN_POINT('Ctrl Pts',(78.3367091307052,-5.08188730272688,44.0484428050865));
#43729=CARTESIAN_POINT('Ctrl Pts',(76.1395936758935,-3.69991595895718,43.9118799514141));
#43730=CARTESIAN_POINT('Ctrl Pts',(74.8521058814301,-1.44613324326173,43.7753170977416));
#43731=CARTESIAN_POINT('Ctrl Pts',(74.7776166467301,1.14840183966585,43.6387542440692));
#43732=CARTESIAN_POINT('Ctrl Pts',(75.9336776591222,3.47233909138358,43.5021913903967));
#43733=CARTESIAN_POINT('Ctrl Pts',(78.0478866735923,4.97808865150259,43.3656285367243));
#43734=CARTESIAN_POINT('Ctrl Pts',(80.622071564542,5.31085162111149,43.2290656830519));
#43735=CARTESIAN_POINT('Ctrl Pts',(83.0496791219762,4.39221706829951,43.0925028293795));
#43736=CARTESIAN_POINT('Ctrl Pts',(84.7586876558485,2.43864711267794,42.955939975707));
#43737=CARTESIAN_POINT('Ctrl Pts',(85.3464128673449,-0.0895474900135507,
42.8193771220346));
#43738=CARTESIAN_POINT('Ctrl Pts',(84.674348928249,-2.59662892732216,42.6828142683622));
#43739=CARTESIAN_POINT('Ctrl Pts',(82.9008974216893,-4.49189446827444,42.5462514146897));
#43740=CARTESIAN_POINT('Ctrl Pts',(80.4438461537563,-5.32867507453335,42.4096885610173));
#43741=CARTESIAN_POINT('Ctrl Pts',(77.882351758936,-4.9099858892129,42.2731257073449));
#43742=CARTESIAN_POINT('Ctrl Pts',(75.8195931490597,-3.33407937207921,42.1365628536724));
#43743=CARTESIAN_POINT('Ctrl Pts',(75.1017336071131,-1.76011787070273,42.0455209512241));
#43744=CARTESIAN_POINT('Ctrl Pts',(74.9489860411411,-0.934590043769125,
42.));
#43745=CARTESIAN_POINT('Ctrl Pts',(74.9489860411411,-0.934590043769125,
42.));
#43746=CARTESIAN_POINT('Ctrl Pts',(74.9621578377196,-1.08166252357025,42.));
#43747=CARTESIAN_POINT('Ctrl Pts',(74.9817852992141,-1.22784345789557,42.));
#43748=CARTESIAN_POINT('Ctrl Pts',(75.0076019736251,-1.37276211585687,42.));
#43749=CARTESIAN_POINT('Ctrl Pts',(75.0338763132224,-1.52024981983637,42.));
#43750=CARTESIAN_POINT('Ctrl Pts',(75.0665612512022,-1.66643073229691,42.));
#43751=CARTESIAN_POINT('Ctrl Pts',(75.1054285779647,-1.81092654194609,42.));
#43752=CARTESIAN_POINT('Ctrl Pts',(75.1448624859236,-1.95752871227154,42.));
#43753=CARTESIAN_POINT('Ctrl Pts',(75.1906603781215,-2.10239702200426,42.));
#43754=CARTESIAN_POINT('Ctrl Pts',(75.2426373250352,-2.24513869268825,42.));
#43755=CARTESIAN_POINT('Ctrl Pts',(75.29454010169,-2.38767667332699,42.));
#43756=CARTESIAN_POINT('Ctrl Pts',(75.3526044873427,-2.5280948419444,42.));
#43757=CARTESIAN_POINT('Ctrl Pts',(75.4166973936328,-2.66599315453721,42.));
#43758=CARTESIAN_POINT('Ctrl Pts',(75.4326815052143,-2.70038357530239,42.));
#43759=CARTESIAN_POINT('Ctrl Pts',(75.449040803215,-2.7346171978847,42.));
#43760=CARTESIAN_POINT('Ctrl Pts',(75.4657736992349,-2.76868764381097,42.));
#43761=CARTESIAN_POINT('Ctrl Pts',(75.4794370599443,-2.79650809949688,42.));
#43762=CARTESIAN_POINT('Ctrl Pts',(75.4933495262802,-2.82421975339959,42.));
#43763=CARTESIAN_POINT('Ctrl Pts',(75.5075103252484,-2.85181908809118,42.));
#43764=CARTESIAN_POINT('Ctrl Pts',(75.5164010622901,-2.86914709534701,42.));
#43765=CARTESIAN_POINT('Ctrl Pts',(75.5253895443675,-2.88643043349627,42.));
#43766=CARTESIAN_POINT('Ctrl Pts',(75.5344690816879,-2.90365621558174,42.));
#43767=CARTESIAN_POINT('Ctrl Pts',(75.6070587324555,-3.04137397163715,42.));
#43768=CARTESIAN_POINT('Ctrl Pts',(75.6855654691879,-3.17561201831191,42.));
#43769=CARTESIAN_POINT('Ctrl Pts',(75.7697563305504,-3.30597466154241,42.));
#43770=CARTESIAN_POINT('Ctrl Pts',(75.7794264538999,-3.32094805437625,42.));
#43771=CARTESIAN_POINT('Ctrl Pts',(75.7891716226622,-3.33587031738042,42.));
#43772=CARTESIAN_POINT('Ctrl Pts',(75.7989915273745,-3.35074084747145,42.));
#43773=CARTESIAN_POINT('Ctrl Pts',(75.8835543044775,-3.47879639977254,42.));
#43774=CARTESIAN_POINT('Ctrl Pts',(75.973654962357,-3.60301695222072,42.));
#43775=CARTESIAN_POINT('Ctrl Pts',(76.0689073761605,-3.7231766192315,42.));
#43776=CARTESIAN_POINT('Ctrl Pts',(76.1653225040828,-3.84480303480804,42.));
#43777=CARTESIAN_POINT('Ctrl Pts',(76.2670163041758,-3.96226941007647,42.));
#43778=CARTESIAN_POINT('Ctrl Pts',(76.373637405052,-4.07532035528121,42.));
#43779=CARTESIAN_POINT('Ctrl Pts',(76.4750970144414,-4.18289854240666,42.));
#43780=CARTESIAN_POINT('Ctrl Pts',(76.5810191264453,-4.28647872276781,42.));
#43781=CARTESIAN_POINT('Ctrl Pts',(76.6911364486616,-4.38581595590781,42.));
#43782=CARTESIAN_POINT('Ctrl Pts',(76.7174590185628,-4.40956164105969,42.));
#43783=CARTESIAN_POINT('Ctrl Pts',(76.7440214458089,-4.43306475471181,42.));
#43784=CARTESIAN_POINT('Ctrl Pts',(76.7708203338762,-4.45632170068001,42.));
#43785=CARTESIAN_POINT('Ctrl Pts',(76.7863924722136,-4.46983570838862,42.));
#43786=CARTESIAN_POINT('Ctrl Pts',(76.8020444525746,-4.4832665963797,42.));
#43787=CARTESIAN_POINT('Ctrl Pts',(76.8177756225022,-4.49661364255217,42.));
#43788=CARTESIAN_POINT('Ctrl Pts',(76.8327874920505,-4.50935040128779,42.));
#43789=CARTESIAN_POINT('Ctrl Pts',(76.8478645955037,-4.52200496353173,42.));
#43790=CARTESIAN_POINT('Ctrl Pts',(76.8630045687877,-4.53457559580324,42.));
#43791=CARTESIAN_POINT('Ctrl Pts',(76.9853501941721,-4.63615846110177,42.));
#43792=CARTESIAN_POINT('Ctrl Pts',(77.1118304566725,-4.73229035624535,42.));
#43793=CARTESIAN_POINT('Ctrl Pts',(77.2420411835477,-4.82273740245613,42.));
#43794=CARTESIAN_POINT('Ctrl Pts',(77.3736430569181,-4.91415076760505,42.));
#43795=CARTESIAN_POINT('Ctrl Pts',(77.5090559855352,-4.9997577814759,42.));
#43796=CARTESIAN_POINT('Ctrl Pts',(77.647907899746,-5.07928955985309,42.));
#43797=CARTESIAN_POINT('Ctrl Pts',(77.6909792789766,-5.10396003996012,42.));
#43798=CARTESIAN_POINT('Ctrl Pts',(77.7343818612472,-5.12804571555085,42.));
#43799=CARTESIAN_POINT('Ctrl Pts',(77.7781053039389,-5.15153788690001,42.));
#43800=CARTESIAN_POINT('Ctrl Pts',(77.9182247422167,-5.22682266894667,42.));
#43801=CARTESIAN_POINT('Ctrl Pts',(78.06163707807,-5.29601545637256,42.));
#43802=CARTESIAN_POINT('Ctrl Pts',(78.2079144047746,-5.35906058683497,42.));
#43803=CARTESIAN_POINT('Ctrl Pts',(78.2974055901389,-5.39763104463341,42.));
#43804=CARTESIAN_POINT('Ctrl Pts',(78.3879697557877,-5.43389968577381,42.));
#43805=CARTESIAN_POINT('Ctrl Pts',(78.4795137827033,-5.46784552584796,42.));
#43806=CARTESIAN_POINT('Ctrl Pts',(78.5294507402801,-5.48636286698762,42.));
#43807=CARTESIAN_POINT('Ctrl Pts',(78.579679328162,-5.50418890812706,42.));
#43808=CARTESIAN_POINT('Ctrl Pts',(78.6301847786606,-5.52131941272422,42.));
#43809=CARTESIAN_POINT('Ctrl Pts',(78.6542608776631,-5.5294855753972,42.));
#43810=CARTESIAN_POINT('Ctrl Pts',(78.6783998956819,-5.53749367161001,42.));
#43811=CARTESIAN_POINT('Ctrl Pts',(78.7026002488239,-5.54534319403179,42.));
#43812=CARTESIAN_POINT('Ctrl Pts',(78.7227291790244,-5.55187212722577,42.));
#43813=CARTESIAN_POINT('Ctrl Pts',(78.7428924200437,-5.55828870175179,42.));
#43814=CARTESIAN_POINT('Ctrl Pts',(78.7630845889307,-5.56459156251722,42.));
#43815=CARTESIAN_POINT('Ctrl Pts',(78.9185216410264,-5.61311027799698,42.));
#43816=CARTESIAN_POINT('Ctrl Pts',(79.0757515599109,-5.65492040660673,42.));
#43817=CARTESIAN_POINT('Ctrl Pts',(79.2342989894222,-5.69001769854474,42.));
#43818=CARTESIAN_POINT('Ctrl Pts',(79.3943420666046,-5.72544607868212,42.));
#43819=CARTESIAN_POINT('Ctrl Pts',(79.5557282918266,-5.75403468223215,42.));
#43820=CARTESIAN_POINT('Ctrl Pts',(79.7179998356104,-5.77573559499886,42.));
#43821=CARTESIAN_POINT('Ctrl Pts',(79.8804872888693,-5.79746538179104,42.));
#43822=CARTESIAN_POINT('Ctrl Pts',(80.0438631437588,-5.81228940141547,42.));
#43823=CARTESIAN_POINT('Ctrl Pts',(80.2076882609928,-5.82011187102181,42.));
#43824=CARTESIAN_POINT('Ctrl Pts',(80.3001239970504,-5.82452557600221,42.));
#43825=CARTESIAN_POINT('Ctrl Pts',(80.3927030712261,-5.8267093823107,42.));
#43826=CARTESIAN_POINT('Ctrl Pts',(80.4853481377936,-5.82663890625317,42.));
#43827=CARTESIAN_POINT('Ctrl Pts',(80.6073305659698,-5.82654611296212,42.));
#43828=CARTESIAN_POINT('Ctrl Pts',(80.7294274833697,-5.82254585001131,42.));
#43829=CARTESIAN_POINT('Ctrl Pts',(80.8514724367705,-5.81468368107405,42.));
#43830=CARTESIAN_POINT('Ctrl Pts',(80.8742756500897,-5.8132146918989,42.));
#43831=CARTESIAN_POINT('Ctrl Pts',(80.8970770480159,-5.81161083778777,42.));
#43832=CARTESIAN_POINT('Ctrl Pts',(80.919875541321,-5.80987235409354,42.));
#43833=CARTESIAN_POINT('Ctrl Pts',(80.9435592690711,-5.80806636744516,42.));
#43834=CARTESIAN_POINT('Ctrl Pts',(80.9672302930977,-5.80611580996086,42.));
#43835=CARTESIAN_POINT('Ctrl Pts',(80.9908841690558,-5.80402160058609,42.));
#43836=CARTESIAN_POINT('Ctrl Pts',(81.155960195153,-5.78940650063313,42.));
#43837=CARTESIAN_POINT('Ctrl Pts',(81.3202504662812,-5.76779538062928,42.));
#43838=CARTESIAN_POINT('Ctrl Pts',(81.4833338348112,-5.73938880947425,42.));
#43839=CARTESIAN_POINT('Ctrl Pts',(81.6417881370958,-5.71178854923165,42.));
#43840=CARTESIAN_POINT('Ctrl Pts',(81.7991037303719,-5.67777281625275,42.));
#43841=CARTESIAN_POINT('Ctrl Pts',(81.9548995203013,-5.63747982388683,42.));
#43842=CARTESIAN_POINT('Ctrl Pts',(82.0257692259441,-5.61915100698019,42.));
#43843=CARTESIAN_POINT('Ctrl Pts',(82.0963244625258,-5.59952266952908,42.));
#43844=CARTESIAN_POINT('Ctrl Pts',(82.1665291864494,-5.57860481216614,42.));
#43845=CARTESIAN_POINT('Ctrl Pts',(82.2022502415219,-5.56796154070089,42.));
#43846=CARTESIAN_POINT('Ctrl Pts',(82.237880548397,-5.55698439518312,42.));
#43847=CARTESIAN_POINT('Ctrl Pts',(82.2734153269695,-5.54567450906375,42.));
#43848=CARTESIAN_POINT('Ctrl Pts',(82.3062731292964,-5.53521664166231,42.));
#43849=CARTESIAN_POINT('Ctrl Pts',(82.3390528004547,-5.52447298718656,42.));
#43850=CARTESIAN_POINT('Ctrl Pts',(82.3717251389673,-5.51345319731889,42.));
#43851=CARTESIAN_POINT('Ctrl Pts',(82.5334598871624,-5.45890298694057,42.));
#43852=CARTESIAN_POINT('Ctrl Pts',(82.6926833054789,-5.39755431492727,42.));
#43853=CARTESIAN_POINT('Ctrl Pts',(82.8489527497613,-5.32958509775792,42.));
#43854=CARTESIAN_POINT('Ctrl Pts',(83.0023884399965,-5.26284841869041,42.));
#43855=CARTESIAN_POINT('Ctrl Pts',(83.1529770200388,-5.18972885692545,42.));
#43856=CARTESIAN_POINT('Ctrl Pts',(83.300293543373,-5.11034629693712,42.));
#43857=CARTESIAN_POINT('Ctrl Pts',(83.4131779268302,-5.04951774126171,42.));
#43858=CARTESIAN_POINT('Ctrl Pts',(83.5241410217568,-4.98501074834143,42.));
#43859=CARTESIAN_POINT('Ctrl Pts',(83.6330530644636,-4.91696557452329,42.));
#43860=CARTESIAN_POINT('Ctrl Pts',(74.8636515713633,-1.05953972605244E-5,
52.4490415053031));
#43861=CARTESIAN_POINT('Ctrl Pts',(74.8636836703329,0.432042645208333,52.425619963237));
#43862=CARTESIAN_POINT('Ctrl Pts',(74.9176467693691,0.864103762023963,52.4021984211709));
#43863=CARTESIAN_POINT('Ctrl Pts',(75.025442005686,1.28228860328595,52.3787768791048));
#43864=CARTESIAN_POINT('Ctrl Pts',(75.2349474977124,2.09505198615906,52.3332559278806));
#43865=CARTESIAN_POINT('Ctrl Pts',(75.6477979012949,2.85539928139903,52.2877349766565));
#43866=CARTESIAN_POINT('Ctrl Pts',(76.215353236599,3.47375015947001,52.2422140254324));
#43867=CARTESIAN_POINT('Ctrl Pts',(76.7829085719031,4.09210103754099,52.1966930742082));
#43868=CARTESIAN_POINT('Ctrl Pts',(77.5051688389287,4.56845549844299,52.1511721229841));
#43869=CARTESIAN_POINT('Ctrl Pts',(78.2970409309692,4.84669183123127,52.1056511717599));
#43870=CARTESIAN_POINT('Ctrl Pts',(79.0889130230097,5.12492816401956,52.0601302205358));
#43871=CARTESIAN_POINT('Ctrl Pts',(79.950396940065,5.20504636869414,52.0146092693116));
#43872=CARTESIAN_POINT('Ctrl Pts',(80.7799969373556,5.07760731781833,51.9690883180875));
#43873=CARTESIAN_POINT('Ctrl Pts',(81.6095969346462,4.95016826694251,51.9235673668633));
#43874=CARTESIAN_POINT('Ctrl Pts',(82.407313012172,4.61517196051629,51.8780464156392));
#43875=CARTESIAN_POINT('Ctrl Pts',(83.0791622348941,4.11208599470871,51.832525464415));
#43876=CARTESIAN_POINT('Ctrl Pts',(83.7510114576161,3.60900002890112,51.7870045131909));
#43877=CARTESIAN_POINT('Ctrl Pts',(84.2969938255343,2.93782440371217,51.7414835619668));
#43878=CARTESIAN_POINT('Ctrl Pts',(84.652784415277,2.17763368857111,51.6959626107426));
#43879=CARTESIAN_POINT('Ctrl Pts',(85.0085750050198,1.41744297343006,51.6504416595185));
#43880=CARTESIAN_POINT('Ctrl Pts',(85.174173816587,0.568237168336915,51.6049207082943));
#43881=CARTESIAN_POINT('Ctrl Pts',(85.1300708228062,-0.269934528300925,
51.5593997570702));
#43882=CARTESIAN_POINT('Ctrl Pts',(85.0859678290255,-1.10810622493877,51.513878805846));
#43883=CARTESIAN_POINT('Ctrl Pts',(84.8321630298966,-1.93524381312131,51.4683578546219));
#43884=CARTESIAN_POINT('Ctrl Pts',(84.3985584427511,-2.65389806178438,51.4228369033978));
#43885=CARTESIAN_POINT('Ctrl Pts',(83.9649538556056,-3.37255231044745,51.3773159521736));
#43886=CARTESIAN_POINT('Ctrl Pts',(83.3515494804435,-3.98272321959106,51.3317950009495));
#43887=CARTESIAN_POINT('Ctrl Pts',(82.6306135656663,-4.41252349169213,51.2862740497253));
#43888=CARTESIAN_POINT('Ctrl Pts',(81.9096776508892,-4.84232376379319,51.2407530985012));
#43889=CARTESIAN_POINT('Ctrl Pts',(81.0812101964971,-5.09175339885173,51.1952321472771));
#43890=CARTESIAN_POINT('Ctrl Pts',(80.2428171117443,-5.13142583955608,51.1497111960529));
#43891=CARTESIAN_POINT('Ctrl Pts',(79.4044240269915,-5.17109828026043,51.1041902448287));
#43892=CARTESIAN_POINT('Ctrl Pts',(78.5561053118782,-5.0010135266106,51.0586692936046));
#43893=CARTESIAN_POINT('Ctrl Pts',(77.7978056523318,-4.64121011716904,51.0131483423805));
#43894=CARTESIAN_POINT('Ctrl Pts',(77.0395059927855,-4.28140670772748,50.9676273911563));
#43895=CARTESIAN_POINT('Ctrl Pts',(76.3712253888062,-3.73188464249419,50.9221064399322));
#43896=CARTESIAN_POINT('Ctrl Pts',(75.8716973327532,-3.0573858742752,50.876585488708));
#43897=CARTESIAN_POINT('Ctrl Pts',(75.3721692767001,-2.38288710605622,50.8310645374839));
#43898=CARTESIAN_POINT('Ctrl Pts',(75.0413937685732,-1.58341163485156,50.7855435862597));
#43899=CARTESIAN_POINT('Ctrl Pts',(74.9183411312984,-0.753149678856254,
50.7400226350356));
#43900=CARTESIAN_POINT('Ctrl Pts',(74.8814142807203,-0.503996471995245,
50.7263622584581));
#43901=CARTESIAN_POINT('Ctrl Pts',(74.863193691693,-0.252070821087219,50.7127018818806));
#43902=CARTESIAN_POINT('Ctrl Pts',(74.863409785596,-0.000114188402419197,
50.6990415053031));
#43903=CARTESIAN_POINT('Ctrl Pts',(78.4211181181246,-5.90584097022479,54.));
#43904=CARTESIAN_POINT('Ctrl Pts',(78.262197315854,-5.84962792448672,54.));
#43905=CARTESIAN_POINT('Ctrl Pts',(78.1060006691959,-5.78682362442592,54.));
#43906=CARTESIAN_POINT('Ctrl Pts',(77.9528680303037,-5.71771729056826,54.));
#43907=CARTESIAN_POINT('Ctrl Pts',(77.7985213424485,-5.64806307564769,54.));
#43908=CARTESIAN_POINT('Ctrl Pts',(77.6472868104496,-5.57200607329776,54.));
#43909=CARTESIAN_POINT('Ctrl Pts',(77.4995371906765,-5.48979573308941,54.));
#43910=CARTESIAN_POINT('Ctrl Pts',(77.3527503170532,-5.40812108081466,54.));
#43911=CARTESIAN_POINT('Ctrl Pts',(77.2094025440176,-5.32037251008645,54.));
#43912=CARTESIAN_POINT('Ctrl Pts',(77.0698924031099,-5.2267559251608,54.));
#43913=CARTESIAN_POINT('Ctrl Pts',(76.9320428668315,-5.13425366879426,54.));
#43914=CARTESIAN_POINT('Ctrl Pts',(76.7979396790733,-5.03602176868112,54.));
#43915=CARTESIAN_POINT('Ctrl Pts',(76.6680070843611,-4.9322284322092,54.));
#43916=CARTESIAN_POINT('Ctrl Pts',(76.6071928831282,-4.88364855996996,54.));
#43917=CARTESIAN_POINT('Ctrl Pts',(76.5472929286395,-4.83384997802402,54.));
#43918=CARTESIAN_POINT('Ctrl Pts',(76.4883542081234,-4.78284805815547,54.));
#43919=CARTESIAN_POINT('Ctrl Pts',(76.4675681505831,-4.76486109081434,54.));
#43920=CARTESIAN_POINT('Ctrl Pts',(76.4469016708152,-4.74672444521351,54.));
#43921=CARTESIAN_POINT('Ctrl Pts',(76.4263569020757,-4.72843876494938,54.));
#43922=CARTESIAN_POINT('Ctrl Pts',(76.4093496763995,-4.71330164197465,54.));
#43923=CARTESIAN_POINT('Ctrl Pts',(76.3924320826677,-4.69806789557155,54.));
#43924=CARTESIAN_POINT('Ctrl Pts',(76.3756100433455,-4.68274265394818,54.));
#43925=CARTESIAN_POINT('Ctrl Pts',(76.253522088766,-4.57151788699861,54.));
#43926=CARTESIAN_POINT('Ctrl Pts',(76.1363802959433,-4.45540215091792,54.));
#43927=CARTESIAN_POINT('Ctrl Pts',(76.0245380696913,-4.33461793741634,54.));
#43928=CARTESIAN_POINT('Ctrl Pts',(76.0120522412589,-4.32113384453241,54.));
#43929=CARTESIAN_POINT('Ctrl Pts',(75.9996325008476,-4.30759153218521,54.));
#43930=CARTESIAN_POINT('Ctrl Pts',(75.9872793707827,-4.29399128343888,54.));
#43931=CARTESIAN_POINT('Ctrl Pts',(75.8762537634941,-4.17175701014861,54.));
#43932=CARTESIAN_POINT('Ctrl Pts',(75.7706051017538,-4.04484500574663,54.));
#43933=CARTESIAN_POINT('Ctrl Pts',(75.6705456325977,-3.91365715790437,54.));
#43934=CARTESIAN_POINT('Ctrl Pts',(75.5706095000858,-3.78263101658568,54.));
#43935=CARTESIAN_POINT('Ctrl Pts',(75.4762484938177,-3.64733884239891,54.));
#43936=CARTESIAN_POINT('Ctrl Pts',(75.3877215008782,-3.50816030674374,54.));
#43937=CARTESIAN_POINT('Ctrl Pts',(75.3053092655013,-3.3785951440857,54.));
#43938=CARTESIAN_POINT('Ctrl Pts',(75.2279532002239,-3.24566130808865,54.));
#43939=CARTESIAN_POINT('Ctrl Pts',(75.1559025908774,-3.10965711388346,54.));
#43940=CARTESIAN_POINT('Ctrl Pts',(75.1382269322467,-3.07629218149895,54.));
#43941=CARTESIAN_POINT('Ctrl Pts',(75.1208707661237,-3.04274244911447,54.));
#43942=CARTESIAN_POINT('Ctrl Pts',(75.1038381551363,-3.00901230432905,54.));
#43943=CARTESIAN_POINT('Ctrl Pts',(75.0918286612032,-2.98522957545307,54.));
#43944=CARTESIAN_POINT('Ctrl Pts',(75.0799800257135,-2.96135715462957,54.));
#43945=CARTESIAN_POINT('Ctrl Pts',(75.0682937193415,-2.93739658146396,54.));
#43946=CARTESIAN_POINT('Ctrl Pts',(75.0593831488875,-2.91912713271648,54.));
#43947=CARTESIAN_POINT('Ctrl Pts',(75.0505692407358,-2.90081106123106,54.));
#43948=CARTESIAN_POINT('Ctrl Pts',(75.0418557997086,-2.88245623475075,54.));
#43949=CARTESIAN_POINT('Ctrl Pts',(74.9725621697134,-2.73648949775383,54.));
#43950=CARTESIAN_POINT('Ctrl Pts',(74.9095514078268,-2.58793651812475,54.));
#43951=CARTESIAN_POINT('Ctrl Pts',(74.8530199493793,-2.43717464723368,54.));
#43952=CARTESIAN_POINT('Ctrl Pts',(74.7969184627566,-2.28755945393634,54.));
#43953=CARTESIAN_POINT('Ctrl Pts',(74.7471978947673,-2.13576814174227,54.));
#43954=CARTESIAN_POINT('Ctrl Pts',(74.7040995632473,-1.98215647267268,54.));
#43955=CARTESIAN_POINT('Ctrl Pts',(74.689189623633,-1.92901425975836,54.));
#43956=CARTESIAN_POINT('Ctrl Pts',(74.6750726996462,-1.8756541147206,54.));
#43957=CARTESIAN_POINT('Ctrl Pts',(74.6617602392352,-1.82209063115797,54.));
#43958=CARTESIAN_POINT('Ctrl Pts',(74.6229859141292,-1.66607980661111,54.));
#43959=CARTESIAN_POINT('Ctrl Pts',(74.5910324654638,-1.50834341117627,54.));
#43960=CARTESIAN_POINT('Ctrl Pts',(74.5659470122711,-1.34933512929417,54.));
#43961=CARTESIAN_POINT('Ctrl Pts',(74.5514323754776,-1.25733171038229,54.));
#43962=CARTESIAN_POINT('Ctrl Pts',(74.53921800968,-1.16490257794463,54.));
#43963=CARTESIAN_POINT('Ctrl Pts',(74.5293208329226,-1.07213748305002,54.));
#43964=CARTESIAN_POINT('Ctrl Pts',(74.5233288405017,-1.01597522999915,54.));
#43965=CARTESIAN_POINT('Ctrl Pts',(74.5181862975362,-0.959689866802773,
54.));
#43966=CARTESIAN_POINT('Ctrl Pts',(74.5138979638249,-0.903301703642221,
54.));
#43967=CARTESIAN_POINT('Ctrl Pts',(74.5119131404968,-0.877202862178623,
54.));
#43968=CARTESIAN_POINT('Ctrl Pts',(74.5101113192301,-0.851082003289393,
54.));
#43969=CARTESIAN_POINT('Ctrl Pts',(74.5084930266152,-0.82494116692696,54.));
#43970=CARTESIAN_POINT('Ctrl Pts',(74.5072652037706,-0.805107722861111,
54.));
#43971=CARTESIAN_POINT('Ctrl Pts',(74.5061436496233,-0.785272753142196,
54.));
#43972=CARTESIAN_POINT('Ctrl Pts',(74.5051283162844,-0.765437884984759,
54.));
#43973=CARTESIAN_POINT('Ctrl Pts',(74.4970709060958,-0.608033747192235,
54.));
#43974=CARTESIAN_POINT('Ctrl Pts',(74.4956975322905,-0.450619814120949,
54.));
#43975=CARTESIAN_POINT('Ctrl Pts',(74.5009899876326,-0.293622280698601,
54.));
#43976=CARTESIAN_POINT('Ctrl Pts',(74.5062660952276,-0.13710969345059,54.));
#43977=CARTESIAN_POINT('Ctrl Pts',(74.5181670402557,0.018989819316881,54.));
#43978=CARTESIAN_POINT('Ctrl Pts',(74.5367258029922,0.174246479217172,54.));
#43979=CARTESIAN_POINT('Ctrl Pts',(74.554987007931,0.327013865966896,54.));
#43980=CARTESIAN_POINT('Ctrl Pts',(74.5796944593158,0.478965862238273,54.));
#43981=CARTESIAN_POINT('Ctrl Pts',(74.6109264058199,0.629675371802867,54.));
#43982=CARTESIAN_POINT('Ctrl Pts',(74.6274886243206,0.709596225510156,54.));
#43983=CARTESIAN_POINT('Ctrl Pts',(74.6458864053681,0.789167314751061,54.));
#43984=CARTESIAN_POINT('Ctrl Pts',(74.6661366021754,0.868321944692978,54.));
#43985=CARTESIAN_POINT('Ctrl Pts',(74.6929665893138,0.973195873746105,54.));
#43986=CARTESIAN_POINT('Ctrl Pts',(74.7230481604637,1.07733908095142,54.));
#43987=CARTESIAN_POINT('Ctrl Pts',(74.756335592551,1.18060444965825,54.));
#43988=CARTESIAN_POINT('Ctrl Pts',(74.764630155877,1.2063361173301,54.));
#43989=CARTESIAN_POINT('Ctrl Pts',(74.7731238140521,1.23201323737033,54.));
#43990=CARTESIAN_POINT('Ctrl Pts',(74.7818159387465,1.25763344672042,54.));
#43991=CARTESIAN_POINT('Ctrl Pts',(74.7894184833493,1.28004209721328,54.));
#43992=CARTESIAN_POINT('Ctrl Pts',(74.797170156781,1.30239918000046,54.));
#43993=CARTESIAN_POINT('Ctrl Pts',(74.8050684469936,1.3246983529196,54.));
#43994=CARTESIAN_POINT('Ctrl Pts',(74.8566369434172,1.47029123289496,54.));
#43995=CARTESIAN_POINT('Ctrl Pts',(74.9144748216866,1.61348540239222,54.));
#43996=CARTESIAN_POINT('Ctrl Pts',(74.9783786997189,1.7538870626109,54.));
#43997=CARTESIAN_POINT('Ctrl Pts',(75.035748310145,1.87993244198298,54.));
#43998=CARTESIAN_POINT('Ctrl Pts',(75.0980076737178,2.00372722149472,54.));
#43999=CARTESIAN_POINT('Ctrl Pts',(75.1650377417778,2.12496422368888,54.));
#44000=CARTESIAN_POINT('Ctrl Pts',(75.1974826154779,2.18364713029786,54.));
#44001=CARTESIAN_POINT('Ctrl Pts',(75.2310455858999,2.24173042299757,54.));
#44002=CARTESIAN_POINT('Ctrl Pts',(75.2657150993742,2.2991770726025,54.));
#44003=CARTESIAN_POINT('Ctrl Pts',(75.2853531085793,2.3317168379668,54.));
#44004=CARTESIAN_POINT('Ctrl Pts',(75.3053461718748,2.36405230992688,54.));
#44005=CARTESIAN_POINT('Ctrl Pts',(75.3256923528984,2.39617652956482,54.));
#44006=CARTESIAN_POINT('Ctrl Pts',(75.3379464504319,2.41552430397864,54.));
#44007=CARTESIAN_POINT('Ctrl Pts',(75.3503269232296,2.43479266761671,54.));
#44008=CARTESIAN_POINT('Ctrl Pts',(75.3628287363761,2.45397339235937,54.));
#44009=CARTESIAN_POINT('Ctrl Pts',(75.4449389344336,2.57994976787039,54.));
#44010=CARTESIAN_POINT('Ctrl Pts',(75.5323361389007,2.70223687521552,54.));
#44011=CARTESIAN_POINT('Ctrl Pts',(75.6248542953279,2.82044646998141,54.));
#44012=CARTESIAN_POINT('Ctrl Pts',(75.7094873480668,2.92858134052372,54.));
#44013=CARTESIAN_POINT('Ctrl Pts',(75.7984063381093,3.03330408161034,54.));
#44014=CARTESIAN_POINT('Ctrl Pts',(75.8915079123733,3.13428753395923,54.));
#44015=CARTESIAN_POINT('Ctrl Pts',(75.9650364336347,3.21404089991225,54.));
#44016=CARTESIAN_POINT('Ctrl Pts',(76.0411743927007,3.29146134666981,54.));
#44017=CARTESIAN_POINT('Ctrl Pts',(76.1197954215943,3.36643663068922,54.));
#44018=CARTESIAN_POINT('Origin',(70.,0.,54.));
#44019=CARTESIAN_POINT('',(48.9897948556636,-10.,54.));
#44020=CARTESIAN_POINT('',(48.9897948556636,10.,54.));
#44021=CARTESIAN_POINT('Origin',(0.,0.,54.));
#44022=CARTESIAN_POINT('',(100.,-10.,54.));
#44023=CARTESIAN_POINT('',(40.,-10.,54.));
#44024=CARTESIAN_POINT('',(100.,10.,54.));
#44025=CARTESIAN_POINT('',(100.,-10.,54.));
#44026=CARTESIAN_POINT('',(100.,10.,54.));
#44027=CARTESIAN_POINT('Origin',(80.,0.,48.));
#44028=CARTESIAN_POINT('Origin',(40.,-10.,42.));
#44029=CARTESIAN_POINT('',(48.9897948556636,-10.,42.));
#44030=CARTESIAN_POINT('',(48.9897948556636,-10.,41.));
#44031=CARTESIAN_POINT('',(100.,-10.,42.));
#44032=CARTESIAN_POINT('',(40.,-10.,42.));
#44033=CARTESIAN_POINT('',(100.,-10.,42.));
#44034=CARTESIAN_POINT('Origin',(100.,10.,42.));
#44035=CARTESIAN_POINT('',(48.9897948556636,10.,42.));
#44036=CARTESIAN_POINT('',(48.9897948556636,10.,41.));
#44037=CARTESIAN_POINT('',(100.,10.,42.));
#44038=CARTESIAN_POINT('',(100.,10.,42.));
#44039=CARTESIAN_POINT('',(100.,10.,42.));
#44040=CARTESIAN_POINT('Origin',(100.,-10.,42.));
#44041=CARTESIAN_POINT('',(100.,-10.,42.));
#44042=CARTESIAN_POINT('Origin',(70.,0.,42.));
#44043=CARTESIAN_POINT('Origin',(0.,0.,42.));
#44044=CARTESIAN_POINT('Origin',(0.,0.,161.));
#44045=CARTESIAN_POINT('',(-40.,4.89858719658941E-15,161.));
#44046=CARTESIAN_POINT('Origin',(0.,0.,161.));
#44047=CARTESIAN_POINT('',(-35.,-4.28626379701574E-15,161.));
#44048=CARTESIAN_POINT('Origin',(0.,0.,161.));
#44049=CARTESIAN_POINT('Origin',(0.,0.,155.));
#44050=CARTESIAN_POINT('',(-40.,-4.89858719658941E-15,155.));
#44051=CARTESIAN_POINT('Origin',(0.,0.,155.));
#44052=CARTESIAN_POINT('',(-35.,-4.28626379701574E-15,155.));
#44053=CARTESIAN_POINT('Origin',(0.,0.,155.));
#44054=CARTESIAN_POINT('Origin',(0.,0.,155.));
#44055=CARTESIAN_POINT('',(-35.,-4.28626379701574E-15,155.));
#44056=CARTESIAN_POINT('Origin',(0.,0.,41.));
#44057=CARTESIAN_POINT('',(-40.,4.89858719658941E-15,65.));
#44058=CARTESIAN_POINT('',(-40.,-4.89858719658941E-15,41.));
#44059=CARTESIAN_POINT('Origin',(0.,0.,65.));
#44060=CARTESIAN_POINT('Origin',(0.,0.,65.));
#44061=CARTESIAN_POINT('',(-35.,-4.28626379701574E-15,65.));
#44062=CARTESIAN_POINT('Origin',(0.,0.,65.));
#44063=CARTESIAN_POINT('Origin',(0.,0.,59.));
#44064=CARTESIAN_POINT('',(-40.,-4.89858719658941E-15,59.));
#44065=CARTESIAN_POINT('Origin',(0.,0.,59.));
#44066=CARTESIAN_POINT('',(-35.,-4.28626379701574E-15,59.));
#44067=CARTESIAN_POINT('Origin',(0.,0.,59.));
#44068=CARTESIAN_POINT('Origin',(0.,0.,59.));
#44069=CARTESIAN_POINT('',(-35.,-4.28626379701574E-15,59.));
#44070=CARTESIAN_POINT('Origin',(0.,0.,41.));
#44071=CARTESIAN_POINT('',(-40.,-4.89858719658941E-15,41.));
#44072=CARTESIAN_POINT('Origin',(0.,0.,41.));
#44073=CARTESIAN_POINT('',(-40.,-4.89858719658941E-15,179.));
#44074=CARTESIAN_POINT('Origin',(0.,0.,179.));
#44075=CARTESIAN_POINT('',(-40.,-4.89858719658941E-15,41.));
#44076=CARTESIAN_POINT('Origin',(0.,0.,41.));
#44077=CARTESIAN_POINT('Origin',(0.,0.,179.));
#44078=CARTESIAN_POINT('Origin',(0.,0.,179.));
#63861=UNCERTAINTY_MEASURE_WITH_UNIT(LENGTH_MEASURE(0.01),#63899,
'DISTANCE_ACCURACY_VALUE',
'Maximum model space distance between geometric entities at asserted c
onnectivities');
#63878=UNCERTAINTY_MEASURE_WITH_UNIT(LENGTH_MEASURE(0.01),#63899,
'DISTANCE_ACCURACY_VALUE',
'Maximum model space distance between geometric entities at asserted c
onnectivities');
#63881=(
GEOMETRIC_REPRESENTATION_CONTEXT(3)
GLOBAL_UNCERTAINTY_ASSIGNED_CONTEXT((#63861))
GLOBAL_UNIT_ASSIGNED_CONTEXT((#63899,#63901,#63902))
REPRESENTATION_CONTEXT('','3D')
);
#63898=(
GEOMETRIC_REPRESENTATION_CONTEXT(3)
GLOBAL_UNCERTAINTY_ASSIGNED_CONTEXT((#63878))
GLOBAL_UNIT_ASSIGNED_CONTEXT((#63899,#63901,#63902))
REPRESENTATION_CONTEXT('','3D')
);
#63899=(
LENGTH_UNIT()
NAMED_UNIT(*)
SI_UNIT(.MILLI.,.METRE.)
);
#63901=(
NAMED_UNIT(*)
PLANE_ANGLE_UNIT()
SI_UNIT($,.RADIAN.)
);
#63902=(
NAMED_UNIT(*)
SI_UNIT($,.STERADIAN.)
SOLID_ANGLE_UNIT()
);
#63905=SHAPE_DEFINITION_REPRESENTATION(#63924,#63996);
#63924=PRODUCT_DEFINITION_SHAPE('',$,#64016);
#63996=SHAPE_REPRESENTATION('',(#15752),#63881);
#64013=PRODUCT_DEFINITION_CONTEXT('part definition',#64072,'design');
#64016=PRODUCT_DEFINITION('Quill','Quill',#64035,#64013);
#64035=PRODUCT_DEFINITION_FORMATION('',$,#64076);
#64072=APPLICATION_CONTEXT(
'Core Data for Automotive Mechanical Design Process');
#64073=PRODUCT_CONTEXT('part definition',#64072,'mechanical');
#64076=PRODUCT('Quill','Quill',$,(#64073));
#64095=PRESENTATION_STYLE_ASSIGNMENT((#64108));
#64108=SURFACE_STYLE_USAGE(.BOTH.,#64121);
#64121=SURFACE_SIDE_STYLE('',(#64134));
#64134=SURFACE_STYLE_FILL_AREA(#64147);
#64147=FILL_AREA_STYLE('Light blue',(#64160));
#64160=FILL_AREA_STYLE_COLOUR('Light blue',#64173);
#64173=COLOUR_RGB('Light blue',0.662745098039216,0.831372549019608,0.949019607843137);
ENDSEC;
END-ISO-10303-21;
